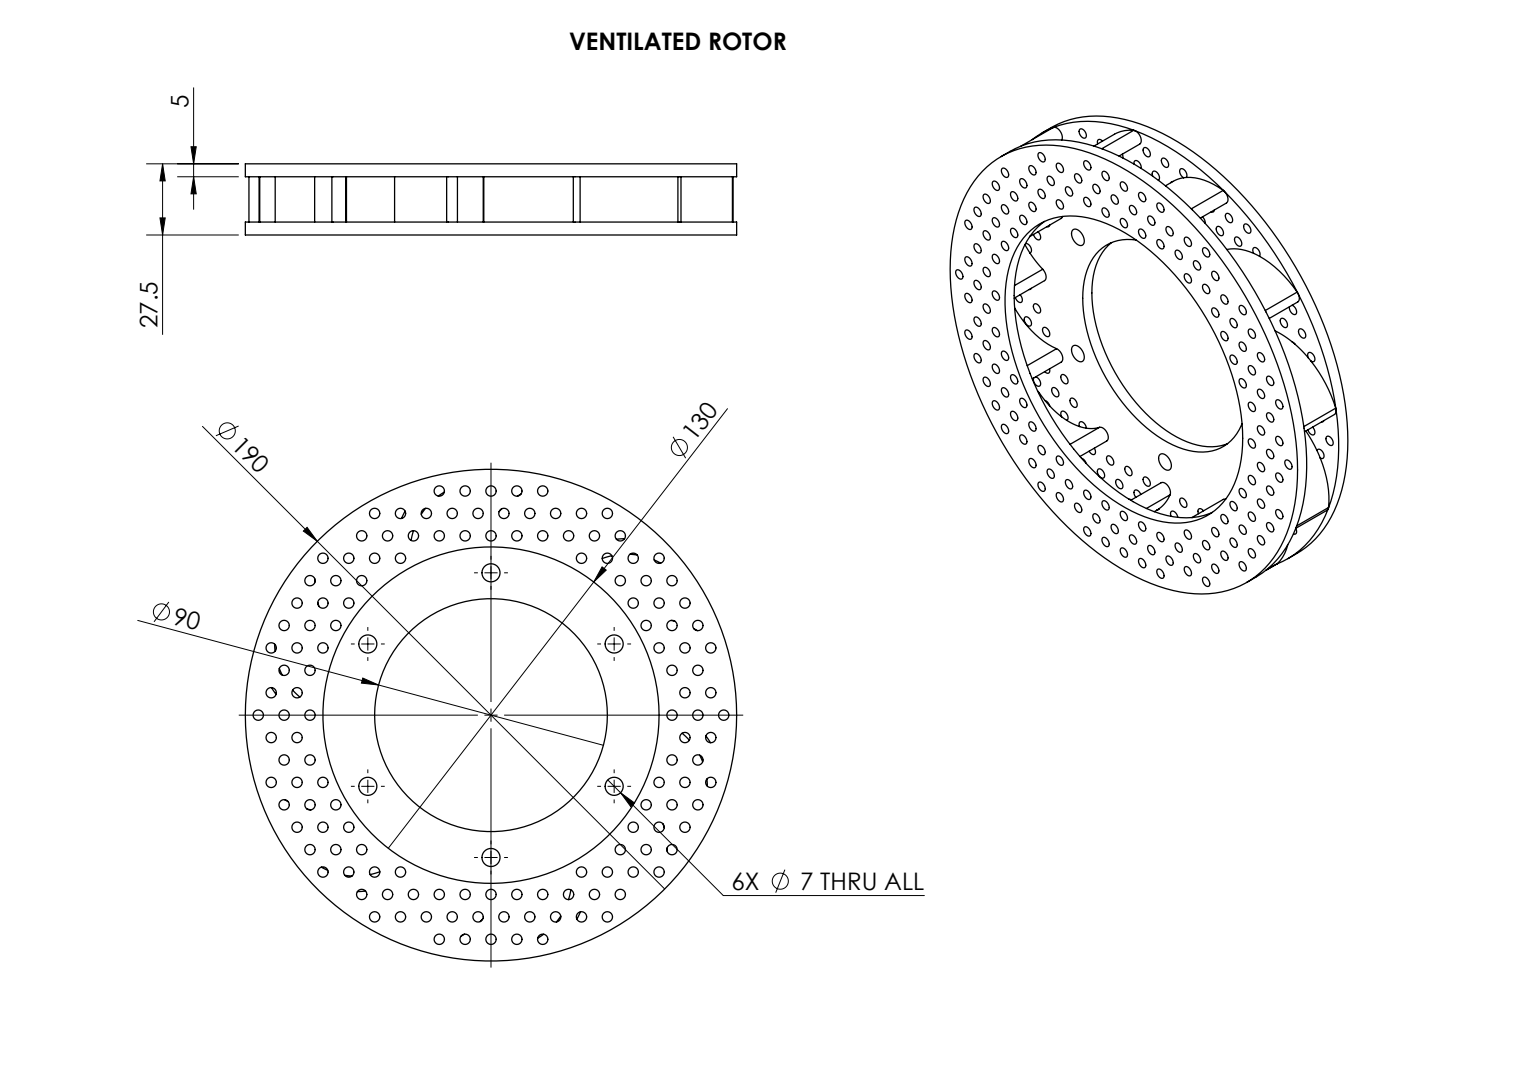
ISO-10303-21;
HEADER;
FILE_DESCRIPTION (('STEP AP214'),
    '1' );
FILE_NAME ('ventilated rotor.step',
    '2026-09-21T15:58:29',
    ( '' ),
    ( '' ),
    'SwSTEP 2.0',
    'SolidWorks 2026',
    '' );
FILE_SCHEMA (( 'AUTOMOTIVE_DESIGN' ));
ENDSEC;

DATA;
#1=ORIENTED_EDGE ( 'NONE', *, *, #25263, .F. ) ;
#2=EDGE_CURVE ( 'NONE', #26836, #23671, #14788, .T. ) ;
#4=VERTEX_POINT ( 'NONE', #16752 ) ;
#5=DIRECTION ( 'NONE',  ( 0.000000000000000000, 0.000000000000000000, 1.000000000000000000 ) ) ;
#7=CARTESIAN_POINT ( 'NONE',  ( 73.47608876694671665, 59.13646009116074964, -4.999999999999997335 ) ) ;
#9=AXIS2_PLACEMENT_3D ( 'NONE', #11158, #31391, #28593 ) ;
#10=DIRECTION ( 'NONE',  ( -1.000000000000000000, 0.000000000000000000, 0.000000000000000000 ) ) ;
#11=DIRECTION ( 'NONE',  ( 0.000000000000000000, 0.000000000000000000, 1.000000000000000000 ) ) ;
#12=FACE_OUTER_BOUND ( 'NONE', #34219, .T. ) ;
#14=ORIENTED_EDGE ( 'NONE', *, *, #31079, .F. ) ;
#15=DIRECTION ( 'NONE',  ( 0.000000000000000000, 0.000000000000000000, 1.000000000000000000 ) ) ;
#17=DIRECTION ( 'NONE',  ( 1.000000000000000000, 0.000000000000000000, 0.000000000000000000 ) ) ;
#19=AXIS2_PLACEMENT_3D ( 'NONE', #6620, #12200, #4183 ) ;
#20=FACE_OUTER_BOUND ( 'NONE', #1538, .T. ) ;
#21=CARTESIAN_POINT ( 'NONE',  ( -85.00000337463092137, -25.98076211353322051, -9.999999999999998224 ) ) ;
#24=EDGE_CURVE ( 'NONE', #14526, #29968, #7006, .T. ) ;
#25=ORIENTED_EDGE ( 'NONE', *, *, #3813, .F. ) ;
#27=EDGE_CURVE ( 'NONE', #13680, #28909, #27960, .T. ) ;
#28=CARTESIAN_POINT ( 'NONE',  ( 31.46585318596250502, 86.45172111230321832, 12.49999999999999822 ) ) ;
#29=AXIS2_PLACEMENT_3D ( 'NONE', #25718, #14617, #11988 ) ;
#30=DIRECTION ( 'NONE',  ( 0.000000000000000000, 0.000000000000000000, 1.000000000000000000 ) ) ;
#31=EDGE_CURVE ( 'NONE', #24795, #10704, #408, .T. ) ;
#32=DIRECTION ( 'NONE',  ( 0.000000000000000000, 0.000000000000000000, -1.000000000000000000 ) ) ;
#33=VERTEX_POINT ( 'NONE', #15201 ) ;
#34=ORIENTED_EDGE ( 'NONE', *, *, #16794, .F. ) ;
#35=AXIS2_PLACEMENT_3D ( 'NONE', #3567, #23609, #24168 ) ;
#36=DIRECTION ( 'NONE',  ( 0.000000000000000000, 0.000000000000000000, 1.000000000000000000 ) ) ;
#38=ORIENTED_EDGE ( 'NONE', *, *, #10995, .T. ) ;
#39=DIRECTION ( 'NONE',  ( 0.000000000000000000, 0.000000000000000000, -1.000000000000000000 ) ) ;
#44=EDGE_CURVE ( 'NONE', #12727, #16632, #5220, .T. ) ;
#45=DIRECTION ( 'NONE',  ( 0.000000000000000000, 0.000000000000000000, 1.000000000000000000 ) ) ;
#47=ORIENTED_EDGE ( 'NONE', *, *, #25069, .T. ) ;
#48=DIRECTION ( 'NONE',  ( 0.000000000000000000, 0.000000000000000000, 1.000000000000000000 ) ) ;
#49=LINE ( 'NONE', #17110, #26195 ) ;
#50=DIRECTION ( 'NONE',  ( 1.000000000000000000, 0.000000000000000000, 0.000000000000000000 ) ) ;
#51=ORIENTED_EDGE ( 'NONE', *, *, #17262, .T. ) ;
#52=CARTESIAN_POINT ( 'NONE',  ( 7.122621931239992550E-13, 68.00000000000000000, -49.86348611802629449 ) ) ;
#53=AXIS2_PLACEMENT_3D ( 'NONE', #21369, #24177, #27163 ) ;
#54=FACE_BOUND ( 'NONE', #30415, .T. ) ;
#55=EDGE_CURVE ( 'NONE', #24891, #6532, #23685, .T. ) ;
#57=CARTESIAN_POINT ( 'NONE',  ( 9.999996625368625658, 86.60254037844397601, 12.50000000000000000 ) ) ;
#58=DIRECTION ( 'NONE',  ( 1.000000000000000000, 0.000000000000000000, 0.000000000000000000 ) ) ;
#59=CYLINDRICAL_SURFACE ( 'NONE', #323, 2.000000000000001776 ) ;
#60=CARTESIAN_POINT ( 'NONE',  ( 89.99999662536828282, 0.000000000000000000, 17.49999999999999645 ) ) ;
#63=CARTESIAN_POINT ( 'NONE',  ( 34.00000000000068923, 58.88972745734143643, 12.49999999999999822 ) ) ;
#64=DIRECTION ( 'NONE',  ( 0.000000000000000000, 0.000000000000000000, -1.000000000000000000 ) ) ;
#66=EDGE_LOOP ( 'NONE', ( #17669, #12617 ) ) ;
#67=EDGE_CURVE ( 'NONE', #35240, #2856, #17838, .T. ) ;
#68=VERTEX_POINT ( 'NONE', #26089 ) ;
#69=ORIENTED_EDGE ( 'NONE', *, *, #4639, .T. ) ;
#70=EDGE_CURVE ( 'NONE', #12832, #7029, #18901, .T. ) ;
#71=EDGE_CURVE ( 'NONE', #553, #16094, #23467, .T. ) ;
#72=DIRECTION ( 'NONE',  ( 0.000000000000000000, 0.000000000000000000, 1.000000000000000000 ) ) ;
#73=FACE_OUTER_BOUND ( 'NONE', #6428, .T. ) ;
#75=EDGE_LOOP ( 'NONE', ( #16524, #10873, #23457, #7165 ) ) ;
#76=CIRCLE ( 'NONE', #28807, 2.000000000000001776 ) ;
#77=DIRECTION ( 'NONE',  ( 1.000000000000000000, 0.000000000000000000, 0.000000000000000000 ) ) ;
#78=ORIENTED_EDGE ( 'NONE', *, *, #9389, .F. ) ;
#80=EDGE_LOOP ( 'NONE', ( #13593, #3847 ) ) ;
#81=CYLINDRICAL_SURFACE ( 'NONE', #36890, 3.000000000000002665 ) ;
#82=ORIENTED_EDGE ( 'NONE', *, *, #8215, .F. ) ;
#83=ORIENTED_EDGE ( 'NONE', *, *, #27457, .T. ) ;
#85=DIRECTION ( 'NONE',  ( 1.000000000000000000, 0.000000000000000000, 0.000000000000000000 ) ) ;
#86=DIRECTION ( 'NONE',  ( 0.000000000000000000, 0.000000000000000000, 1.000000000000000000 ) ) ;
#87=ORIENTED_EDGE ( 'NONE', *, *, #14475, .T. ) ;
#88=DIRECTION ( 'NONE',  ( 0.000000000000000000, 0.000000000000000000, 1.000000000000000000 ) ) ;
#89=EDGE_CURVE ( 'NONE', #15444, #13344, #33274, .T. ) ;
#92=EDGE_LOOP ( 'NONE', ( #21704, #496, #2169, #36469 ) ) ;
#93=CYLINDRICAL_SURFACE ( 'NONE', #7565, 2.000000000000001776 ) ;
#94=DIRECTION ( 'NONE',  ( 0.000000000000000000, 0.000000000000000000, 1.000000000000000000 ) ) ;
#95=CIRCLE ( 'NONE', #3102, 2.000000000000001776 ) ;
#96=ORIENTED_EDGE ( 'NONE', *, *, #17102, .T. ) ;
#97=DIRECTION ( 'NONE',  ( 1.000000000000000000, 0.000000000000000000, 0.000000000000000000 ) ) ;
#98=CIRCLE ( 'NONE', #10881, 2.000000000000001776 ) ;
#99=FACE_OUTER_BOUND ( 'NONE', #4741, .T. ) ;
#100=CYLINDRICAL_SURFACE ( 'NONE', #2791, 2.000000000000001776 ) ;
#101=CARTESIAN_POINT ( 'NONE',  ( 77.99999662536832545, -34.64101615137759183, -9.999999999999998224 ) ) ;
#102=ORIENTED_EDGE ( 'NONE', *, *, #25257, .T. ) ;
#103=DIRECTION ( 'NONE',  ( 1.000000000000000000, 0.000000000000000000, 0.000000000000000000 ) ) ;
#104=FACE_OUTER_BOUND ( 'NONE', #24735, .T. ) ;
#106=ORIENTED_EDGE ( 'NONE', *, *, #23165, .T. ) ;
#107=EDGE_CURVE ( 'NONE', #34831, #10183, #17101, .T. ) ;
#108=FACE_OUTER_BOUND ( 'NONE', #27387, .T. ) ;
#109=CARTESIAN_POINT ( 'NONE',  ( 7.999996625368656744, -69.28203230275519786, 17.49999999999999645 ) ) ;
#110=DIRECTION ( 'NONE',  ( -1.000000000000000000, -4.625929269271482956E-15, 0.000000000000000000 ) ) ;
#111=VERTEX_POINT ( 'NONE', #9201 ) ;
#112=CIRCLE ( 'NONE', #7327, 33.00000000000002132 ) ;
#113=DIRECTION ( 'NONE',  ( 0.000000000000000000, 0.000000000000000000, 1.000000000000000000 ) ) ;
#115=CYLINDRICAL_SURFACE ( 'NONE', #8938, 2.000000000000001776 ) ;
#116=ORIENTED_EDGE ( 'NONE', *, *, #4433, .F. ) ;
#117=DIRECTION ( 'NONE',  ( 1.000000000000000000, 0.000000000000000000, 0.000000000000000000 ) ) ;
#119=CARTESIAN_POINT ( 'NONE',  ( 0.000000000000000000, 0.000000000000000000, 12.49999999999999822 ) ) ;
#121=EDGE_CURVE ( 'NONE', #28672, #5777, #21894, .T. ) ;
#123=CARTESIAN_POINT ( 'NONE',  ( -65.00000337463106348, -60.62177826491083010, -9.999999999999998224 ) ) ;
#124=DIRECTION ( 'NONE',  ( -1.000000000000000000, 0.000000000000000000, 0.000000000000000000 ) ) ;
#125=DIRECTION ( 'NONE',  ( -1.000000000000000000, 0.000000000000000000, 0.000000000000000000 ) ) ;
#126=VERTEX_POINT ( 'NONE', #20628 ) ;
#127=CARTESIAN_POINT ( 'NONE',  ( -56.67878100130369035, 27.78182860042797131, 12.49999999999999822 ) ) ;
#128=DIRECTION ( 'NONE',  ( 0.000000000000000000, 0.000000000000000000, -1.000000000000000000 ) ) ;
#129=DIRECTION ( 'NONE',  ( -1.000000000000000000, 0.000000000000000000, 0.000000000000000000 ) ) ;
#131=EDGE_CURVE ( 'NONE', #32452, #18237, #7927, .T. ) ;
#133=CIRCLE ( 'NONE', #36688, 33.00000000000001421 ) ;
#136=CARTESIAN_POINT ( 'NONE',  ( -20.00000337463123756, -86.60254037844400443, -9.999999999999998224 ) ) ;
#137=EDGE_CURVE ( 'NONE', #22617, #21874, #32058, .T. ) ;
#138=CARTESIAN_POINT ( 'NONE',  ( 71.99999662536838230, -34.64101615137759183, -9.999999999999998224 ) ) ;
#140=DIRECTION ( 'NONE',  ( -1.000000000000000000, -9.765850679573131385E-15, 0.000000000000000000 ) ) ;
#142=ORIENTED_EDGE ( 'NONE', *, *, #26390, .F. ) ;
#145=FACE_OUTER_BOUND ( 'NONE', #19323, .T. ) ;
#147=DIRECTION ( 'NONE',  ( 0.000000000000000000, 0.000000000000000000, 1.000000000000000000 ) ) ;
#148=VERTEX_POINT ( 'NONE', #32628 ) ;
#150=EDGE_CURVE ( 'NONE', #5895, #27049, #26455, .T. ) ;
#151=FACE_BOUND ( 'NONE', #17768, .T. ) ;
#153=CIRCLE ( 'NONE', #7373, 2.000000000000001776 ) ;
#154=ORIENTED_EDGE ( 'NONE', *, *, #13664, .T. ) ;
#155=EDGE_CURVE ( 'NONE', #32663, #9761, #30082, .T. ) ;
#157=CARTESIAN_POINT ( 'NONE',  ( 81.99999662536832545, -17.32050807568879591, -9.999999999999998224 ) ) ;
#158=ORIENTED_EDGE ( 'NONE', *, *, #26934, .T. ) ;
#159=ADVANCED_FACE ( 'NONE', ( #762 ), #32267, .F. ) ;
#161=CARTESIAN_POINT ( 'NONE',  ( 47.99999662536846756, 51.96152422706637708, -5.000000000000000000 ) ) ;
#163=ORIENTED_EDGE ( 'NONE', *, *, #28659, .F. ) ;
#164=ORIENTED_EDGE ( 'NONE', *, *, #35718, .T. ) ;
#165=EDGE_CURVE ( 'NONE', #35067, #9776, #18024, .T. ) ;
#166=AXIS2_PLACEMENT_3D ( 'NONE', #2144, #21659, #19396 ) ;
#167=VERTEX_POINT ( 'NONE', #9594 ) ;
#168=ORIENTED_EDGE ( 'NONE', *, *, #20538, .F. ) ;
#169=AXIS2_PLACEMENT_3D ( 'NONE', #10141, #18184, #29613 ) ;
#171=ORIENTED_EDGE ( 'NONE', *, *, #5884, .T. ) ;
#172=DIRECTION ( 'NONE',  ( 0.000000000000000000, 0.000000000000000000, 1.000000000000000000 ) ) ;
#174=DIRECTION ( 'NONE',  ( 0.000000000000000000, 0.000000000000000000, 1.000000000000000000 ) ) ;
#176=DIRECTION ( 'NONE',  ( 0.000000000000000000, 0.000000000000000000, 1.000000000000000000 ) ) ;
#177=ORIENTED_EDGE ( 'NONE', *, *, #12686, .T. ) ;
#179=CARTESIAN_POINT ( 'NONE',  ( 76.99999662536836809, -8.660254037844401509, -5.000000000000000000 ) ) ;
#180=AXIS2_PLACEMENT_3D ( 'NONE', #17663, #11656, #14493 ) ;
#181=CARTESIAN_POINT ( 'NONE',  ( -87.00000337463093558, 25.98076211353317433, -9.999999999999998224 ) ) ;
#182=VERTEX_POINT ( 'NONE', #6760 ) ;
#184=CARTESIAN_POINT ( 'NONE',  ( -67.00000337463102085, 43.30127018922198801, -9.999999999999998224 ) ) ;
#185=ORIENTED_EDGE ( 'NONE', *, *, #1729, .T. ) ;
#186=EDGE_LOOP ( 'NONE', ( #37032, #34199, #35351 ) ) ;
#189=DIRECTION ( 'NONE',  ( -1.000000000000000000, 0.000000000000000000, 0.000000000000000000 ) ) ;
#190=DIRECTION ( 'NONE',  ( 0.000000000000000000, 0.000000000000000000, 1.000000000000000000 ) ) ;
#191=FACE_OUTER_BOUND ( 'NONE', #12059, .T. ) ;
#192=ORIENTED_EDGE ( 'NONE', *, *, #24443, .F. ) ;
#193=ORIENTED_EDGE ( 'NONE', *, *, #28677, .F. ) ;
#195=FACE_OUTER_BOUND ( 'NONE', #26488, .T. ) ;
#196=EDGE_CURVE ( 'NONE', #666, #24271, #33682, .T. ) ;
#198=CYLINDRICAL_SURFACE ( 'NONE', #3922, 2.000000000000001776 ) ;
#199=CIRCLE ( 'NONE', #27130, 2.000000000000001776 ) ;
#200=VERTEX_POINT ( 'NONE', #18959 ) ;
#203=VERTEX_POINT ( 'NONE', #33394 ) ;
#204=ORIENTED_EDGE ( 'NONE', *, *, #23510, .F. ) ;
#205=CIRCLE ( 'NONE', #19978, 1.999999999999998224 ) ;
#206=CARTESIAN_POINT ( 'NONE',  ( -55.00000337463107059, 43.30127018922197379, -9.999999999999998224 ) ) ;
#207=AXIS2_PLACEMENT_3D ( 'NONE', #7351, #10726, #24618 ) ;
#208=LINE ( 'NONE', #6596, #28035 ) ;
#210=VERTEX_POINT ( 'NONE', #1504 ) ;
#211=FACE_OUTER_BOUND ( 'NONE', #12219, .T. ) ;
#213=DIRECTION ( 'NONE',  ( 0.000000000000000000, 0.000000000000000000, 1.000000000000000000 ) ) ;
#214=DIRECTION ( 'NONE',  ( -1.000000000000000000, 0.000000000000000000, 0.000000000000000000 ) ) ;
#215=EDGE_CURVE ( 'NONE', #20361, #36249, #4334, .T. ) ;
#217=CARTESIAN_POINT ( 'NONE',  ( 54.99999662536846046, -43.30127018922200222, -9.999999999999998224 ) ) ;
#218=FACE_BOUND ( 'NONE', #809, .T. ) ;
#220=DIRECTION ( 'NONE',  ( 1.000000000000000000, 0.000000000000000000, 0.000000000000000000 ) ) ;
#221=CARTESIAN_POINT ( 'NONE',  ( -13.00000337463126066, 77.94228634059957983, 17.49999999999999645 ) ) ;
#222=DIRECTION ( 'NONE',  ( 1.000000000000000000, 0.000000000000000000, 0.000000000000000000 ) ) ;
#223=CIRCLE ( 'NONE', #20559, 2.000000000000000000 ) ;
#224=DIRECTION ( 'NONE',  ( 0.000000000000000000, 0.000000000000000000, 1.000000000000000000 ) ) ;
#225=DIRECTION ( 'NONE',  ( 0.000000000000000000, 0.000000000000000000, -1.000000000000000000 ) ) ;
#226=ORIENTED_EDGE ( 'NONE', *, *, #20326, .F. ) ;
#227=CARTESIAN_POINT ( 'NONE',  ( -60.00000337463108480, -51.96152422706641971, -9.999999999999998224 ) ) ;
#228=DIRECTION ( 'NONE',  ( 0.000000000000000000, 0.000000000000000000, -1.000000000000000000 ) ) ;
#230=VECTOR ( 'NONE', #24200, 1000.000000000000000 ) ;
#232=EDGE_LOOP ( 'NONE', ( #6616, #28930, #1676, #8816 ) ) ;
#233=EDGE_CURVE ( 'NONE', #35279, #34770, #16155, .T. ) ;
#234=ORIENTED_EDGE ( 'NONE', *, *, #11721, .F. ) ;
#235=CIRCLE ( 'NONE', #13432, 1.999999999999998224 ) ;
#236=DIRECTION ( 'NONE',  ( -1.000000000000000000, 0.000000000000000000, 0.000000000000000000 ) ) ;
#237=CYLINDRICAL_SURFACE ( 'NONE', #14553, 2.000000000000001776 ) ;
#238=EDGE_CURVE ( 'NONE', #20810, #35505, #23500, .T. ) ;
#239=CARTESIAN_POINT ( 'NONE',  ( 79.99999662536833966, 34.64101615137759183, -5.000000000000000000 ) ) ;
#240=EDGE_LOOP ( 'NONE', ( #25593, #21234, #28289, #3164 ) ) ;
#241=EDGE_CURVE ( 'NONE', #35128, #3947, #28283, .T. ) ;
#242=DIRECTION ( 'NONE',  ( 0.8660254037844418162, 0.4999999999999946709, 0.000000000000000000 ) ) ;
#243=ORIENTED_EDGE ( 'NONE', *, *, #24473, .T. ) ;
#244=CARTESIAN_POINT ( 'NONE',  ( -70.00000337463099243, 51.96152422706637708, -5.000000000000000000 ) ) ;
#245=VERTEX_POINT ( 'NONE', #21754 ) ;
#246=EDGE_CURVE ( 'NONE', #24313, #6247, #31847, .T. ) ;
#249=EDGE_CURVE ( 'NONE', #20086, #13680, #36679, .T. ) ;
#251=CIRCLE ( 'NONE', #9840, 27.00000000000001421 ) ;
#253=CARTESIAN_POINT ( 'NONE',  ( -31.00000000000027356, -58.88972745734168512, -4.999999999999997335 ) ) ;
#254=CARTESIAN_POINT ( 'NONE',  ( -3.374631303565411855E-06, -86.60254037844400443, -9.999999999999998224 ) ) ;
#255=ORIENTED_EDGE ( 'NONE', *, *, #21076, .T. ) ;
#256=DIRECTION ( 'NONE',  ( 1.000000000000000000, 0.000000000000000000, 0.000000000000000000 ) ) ;
#257=EDGE_CURVE ( 'NONE', #28630, #6061, #8948, .T. ) ;
#258=AXIS2_PLACEMENT_3D ( 'NONE', #28130, #2453, #13872 ) ;
#259=CARTESIAN_POINT ( 'NONE',  ( 0.000000000000000000, 0.000000000000000000, 12.49999999999999822 ) ) ;
#260=AXIS2_PLACEMENT_3D ( 'NONE', #12321, #32216, #32783 ) ;
#262=DIRECTION ( 'NONE',  ( -1.000000000000000000, 0.000000000000000000, 0.000000000000000000 ) ) ;
#263=ADVANCED_FACE ( 'NONE', ( #24402 ), #10505, .F. ) ;
#264=EDGE_LOOP ( 'NONE', ( #8446, #2459 ) ) ;
#266=CARTESIAN_POINT ( 'NONE',  ( 51.99999662536848888, -51.96152422706640550, 12.50000000000000000 ) ) ;
#268=EDGE_CURVE ( 'NONE', #8353, #34330, #5962, .T. ) ;
#269=ORIENTED_EDGE ( 'NONE', *, *, #4961, .F. ) ;
#270=CARTESIAN_POINT ( 'NONE',  ( -40.00000337463113453, 69.28203230275516944, -9.999999999999998224 ) ) ;
#271=CARTESIAN_POINT ( 'NONE',  ( 68.00000000000000000, 0.000000000000000000, -49.86348611802629449 ) ) ;
#272=FACE_OUTER_BOUND ( 'NONE', #19222, .T. ) ;
#274=DIRECTION ( 'NONE',  ( 1.000000000000000000, 0.000000000000000000, 0.000000000000000000 ) ) ;
#275=AXIS2_PLACEMENT_3D ( 'NONE', #18372, #12551, #4489 ) ;
#279=DIRECTION ( 'NONE',  ( 0.000000000000000000, 0.000000000000000000, 1.000000000000000000 ) ) ;
#281=VERTEX_POINT ( 'NONE', #22145 ) ;
#282=CIRCLE ( 'NONE', #23627, 2.000000000000001776 ) ;
#286=DIRECTION ( 'NONE',  ( 0.000000000000000000, 0.000000000000000000, 1.000000000000000000 ) ) ;
#287=DIRECTION ( 'NONE',  ( -1.000000000000000000, 0.000000000000000000, 0.000000000000000000 ) ) ;
#288=AXIS2_PLACEMENT_3D ( 'NONE', #11552, #26000, #31627 ) ;
#289=CIRCLE ( 'NONE', #2710, 2.000000000000001776 ) ;
#290=DIRECTION ( 'NONE',  ( 0.000000000000000000, 0.000000000000000000, -1.000000000000000000 ) ) ;
#291=ORIENTED_EDGE ( 'NONE', *, *, #20174, .T. ) ;
#293=ORIENTED_EDGE ( 'NONE', *, *, #27242, .F. ) ;
#294=FACE_BOUND ( 'NONE', #33628, .T. ) ;
#295=DIRECTION ( 'NONE',  ( 1.000000000000000000, 0.000000000000000000, 0.000000000000000000 ) ) ;
#296=CIRCLE ( 'NONE', #6888, 2.000000000000001776 ) ;
#297=CARTESIAN_POINT ( 'NONE',  ( -60.00000337463104216, 34.64101615137757051, -9.999999999999998224 ) ) ;
#298=CIRCLE ( 'NONE', #6279, 95.00000000000001421 ) ;
#299=DIRECTION ( 'NONE',  ( 0.000000000000000000, 0.000000000000000000, 1.000000000000000000 ) ) ;
#301=VECTOR ( 'NONE', #9104, 1000.000000000000000 ) ;
#302=AXIS2_PLACEMENT_3D ( 'NONE', #13859, #25139, #31280 ) ;
#304=CARTESIAN_POINT ( 'NONE',  ( 64.99999662536839651, -43.30127018922199511, -9.999999999999998224 ) ) ;
#305=DIRECTION ( 'NONE',  ( 0.000000000000000000, 0.000000000000000000, 1.000000000000000000 ) ) ;
#306=EDGE_CURVE ( 'NONE', #32244, #30221, #25138, .T. ) ;
#308=CARTESIAN_POINT ( 'NONE',  ( -40.00000337463113453, -69.28203230275519786, 17.49999999999999645 ) ) ;
#309=CYLINDRICAL_SURFACE ( 'NONE', #34030, 2.000000000000001776 ) ;
#310=VECTOR ( 'NONE', #20718, 1000.000000000000000 ) ;
#311=CARTESIAN_POINT ( 'NONE',  ( -48.49679504533954599, -67.96280346788670101, 12.50000000000000000 ) ) ;
#312=AXIS2_PLACEMENT_3D ( 'NONE', #1612, #13051, #12846 ) ;
#313=CIRCLE ( 'NONE', #17111, 33.00000000000001421 ) ;
#314=EDGE_LOOP ( 'NONE', ( #13805, #27625, #5618, #19237 ) ) ;
#317=ORIENTED_EDGE ( 'NONE', *, *, #23310, .F. ) ;
#318=CYLINDRICAL_SURFACE ( 'NONE', #26736, 2.000000000000001776 ) ;
#320=VECTOR ( 'NONE', #25378, 1000.000000000000000 ) ;
#321=LINE ( 'NONE', #703, #22374 ) ;
#323=AXIS2_PLACEMENT_3D ( 'NONE', #34020, #22562, #31540 ) ;
#324=CARTESIAN_POINT ( 'NONE',  ( 34.99999662536855283, -77.94228634059960825, -9.999999999999998224 ) ) ;
#325=VECTOR ( 'NONE', #1638, 1000.000000000000000 ) ;
#326=EDGE_CURVE ( 'NONE', #14473, #5023, #12520, .T. ) ;
#327=AXIS2_PLACEMENT_3D ( 'NONE', #16910, #9026, #2860 ) ;
#328=DIRECTION ( 'NONE',  ( 1.000000000000000000, 0.000000000000000000, 0.000000000000000000 ) ) ;
#329=EDGE_CURVE ( 'NONE', #27070, #4355, #10750, .T. ) ;
#330=ORIENTED_EDGE ( 'NONE', *, *, #17401, .T. ) ;
#331=ORIENTED_EDGE ( 'NONE', *, *, #15606, .T. ) ;
#332=DIRECTION ( 'NONE',  ( 1.000000000000000000, 0.000000000000000000, 0.000000000000000000 ) ) ;
#333=DIRECTION ( 'NONE',  ( 0.000000000000000000, 0.000000000000000000, 1.000000000000000000 ) ) ;
#334=LINE ( 'NONE', #8600, #4130 ) ;
#336=AXIS2_PLACEMENT_3D ( 'NONE', #30480, #30096, #21491 ) ;
#337=EDGE_CURVE ( 'NONE', #3085, #32118, #36511, .T. ) ;
#338=FACE_BOUND ( 'NONE', #19821, .T. ) ;
#339=EDGE_LOOP ( 'NONE', ( #32117, #28572, #22647 ) ) ;
#340=ORIENTED_EDGE ( 'NONE', *, *, #13858, .F. ) ;
#341=CARTESIAN_POINT ( 'NONE',  ( 31.99999662536857770, -69.28203230275519786, 17.49999999999999645 ) ) ;
#342=ORIENTED_EDGE ( 'NONE', *, *, #22958, .F. ) ;
#344=DIRECTION ( 'NONE',  ( 1.000000000000000000, 0.000000000000000000, 0.000000000000000000 ) ) ;
#347=EDGE_CURVE ( 'NONE', #5750, #19941, #18596, .T. ) ;
#348=ORIENTED_EDGE ( 'NONE', *, *, #23113, .F. ) ;
#349=ORIENTED_EDGE ( 'NONE', *, *, #15856, .F. ) ;
#351=CIRCLE ( 'NONE', #30901, 27.00000000000001421 ) ;
#352=ORIENTED_EDGE ( 'NONE', *, *, #4867, .T. ) ;
#353=VECTOR ( 'NONE', #6522, 1000.000000000000000 ) ;
#354=AXIS2_PLACEMENT_3D ( 'NONE', #1393, #4597, #16033 ) ;
#355=EDGE_LOOP ( 'NONE', ( #5631, #10944 ) ) ;
#356=CIRCLE ( 'NONE', #29106, 2.000000000000001776 ) ;
#357=VERTEX_POINT ( 'NONE', #11426 ) ;
#358=CARTESIAN_POINT ( 'NONE',  ( 64.99999662536839651, -60.62177826491080168, 12.50000000000000000 ) ) ;
#359=DIRECTION ( 'NONE',  ( 0.000000000000000000, 0.000000000000000000, 1.000000000000000000 ) ) ;
#360=CARTESIAN_POINT ( 'NONE',  ( 61.99999662536842493, 51.96152422706639129, -9.999999999999998224 ) ) ;
#362=DIRECTION ( 'NONE',  ( 0.000000000000000000, 0.000000000000000000, 1.000000000000000000 ) ) ;
#363=ORIENTED_EDGE ( 'NONE', *, *, #17772, .T. ) ;
#364=DIRECTION ( 'NONE',  ( 4.625929269271481378E-15, 1.000000000000000000, 0.000000000000000000 ) ) ;
#365=VECTOR ( 'NONE', #5528, 1000.000000000000000 ) ;
#366=CARTESIAN_POINT ( 'NONE',  ( -3.374631289687624047E-06, -69.28203230275519786, 17.49999999999999645 ) ) ;
#367=EDGE_CURVE ( 'NONE', #31278, #23804, #18545, .T. ) ;
#369=ORIENTED_EDGE ( 'NONE', *, *, #22241, .T. ) ;
#370=DIRECTION ( 'NONE',  ( 1.000000000000000000, 0.000000000000000000, 0.000000000000000000 ) ) ;
#371=CARTESIAN_POINT ( 'NONE',  ( -50.00000337463112032, -51.96152422706641971, -9.999999999999998224 ) ) ;
#372=ORIENTED_EDGE ( 'NONE', *, *, #6789, .F. ) ;
#373=AXIS2_PLACEMENT_3D ( 'NONE', #34364, #17849, #12387 ) ;
#376=CIRCLE ( 'NONE', #15948, 2.000000000000001776 ) ;
#377=PRODUCT_DEFINITION ( 'UNKNOWN', '', #6977, #25310 ) ;
#378=DIRECTION ( 'NONE',  ( -1.000000000000000000, 0.000000000000000000, 0.000000000000000000 ) ) ;
#379=DIRECTION ( 'NONE',  ( 1.000000000000000000, 0.000000000000000000, 0.000000000000000000 ) ) ;
#380=DIRECTION ( 'NONE',  ( 0.000000000000000000, 0.000000000000000000, -1.000000000000000000 ) ) ;
#381=EDGE_CURVE ( 'NONE', #31393, #2483, #23330, .T. ) ;
#383=ORIENTED_EDGE ( 'NONE', *, *, #2638, .F. ) ;
#384=AXIS2_PLACEMENT_3D ( 'NONE', #15641, #24247, #35700 ) ;
#386=CARTESIAN_POINT ( 'NONE',  ( 44.99999662536851019, 77.94228634059959404, -9.999999999999998224 ) ) ;
#387=CARTESIAN_POINT ( 'NONE',  ( 46.99999662536849598, 60.62177826491077326, -9.999999999999998224 ) ) ;
#389=AXIS2_PLACEMENT_3D ( 'NONE', #3869, #35759, #30111 ) ;
#390=ADVANCED_FACE ( 'NONE', ( #34309 ), #8442, .F. ) ;
#393=VERTEX_POINT ( 'NONE', #19504 ) ;
#395=CIRCLE ( 'NONE', #5209, 2.000000000000001776 ) ;
#396=DIRECTION ( 'NONE',  ( 0.000000000000000000, 0.000000000000000000, 1.000000000000000000 ) ) ;
#397=CARTESIAN_POINT ( 'NONE',  ( -8.000003374631278419, -69.28203230275519786, -9.999999999999998224 ) ) ;
#398=ORIENTED_EDGE ( 'NONE', *, *, #9596, .T. ) ;
#399=ORIENTED_EDGE ( 'NONE', *, *, #27886, .T. ) ;
#402=CARTESIAN_POINT ( 'NONE',  ( 54.99999662536846046, -43.30127018922200222, -5.000000000000000000 ) ) ;
#403=FACE_OUTER_BOUND ( 'NONE', #1715, .T. ) ;
#405=CIRCLE ( 'NONE', #23176, 2.000000000000001776 ) ;
#406=VERTEX_POINT ( 'NONE', #31295 ) ;
#407=CARTESIAN_POINT ( 'NONE',  ( -75.00000337463097821, -8.660254037844422825, -5.000000000000000000 ) ) ;
#408=CIRCLE ( 'NONE', #21379, 95.00000000000000000 ) ;
#409=FACE_BOUND ( 'NONE', #25954, .T. ) ;
#410=DIRECTION ( 'NONE',  ( 0.000000000000000000, 0.000000000000000000, 1.000000000000000000 ) ) ;
#411=CARTESIAN_POINT ( 'NONE',  ( 84.99999662536832545, 25.98076211353319565, -5.000000000000000000 ) ) ;
#414=CYLINDRICAL_SURFACE ( 'NONE', #5727, 2.000000000000001776 ) ;
#415=EDGE_CURVE ( 'NONE', #9776, #6234, #17336, .T. ) ;
#416=AXIS2_PLACEMENT_3D ( 'NONE', #33124, #10826, #22083 ) ;
#417=CIRCLE ( 'NONE', #24987, 2.000000000000001776 ) ;
#418=CARTESIAN_POINT ( 'NONE',  ( -72.00000337463100664, 34.64101615137758472, -9.999999999999998224 ) ) ;
#419=EDGE_CURVE ( 'NONE', #33801, #10648, #30929, .T. ) ;
#422=DIRECTION ( 'NONE',  ( -1.000000000000000000, 0.000000000000000000, 0.000000000000000000 ) ) ;
#425=AXIS2_PLACEMENT_3D ( 'NONE', #16423, #2545, #16814 ) ;
#426=ORIENTED_EDGE ( 'NONE', *, *, #31754, .T. ) ;
#427=AXIS2_PLACEMENT_3D ( 'NONE', #36028, #27183, #30185 ) ;
#429=EDGE_LOOP ( 'NONE', ( #21064, #7984 ) ) ;
#432=CARTESIAN_POINT ( 'NONE',  ( -30.00000337463118427, 69.28203230275516944, -9.999999999999998224 ) ) ;
#433=ORIENTED_EDGE ( 'NONE', *, *, #32932, .F. ) ;
#435=CIRCLE ( 'NONE', #1059, 2.000000000000001776 ) ;
#437=EDGE_CURVE ( 'NONE', #14230, #21660, #8801, .T. ) ;
#438=AXIS2_PLACEMENT_3D ( 'NONE', #22022, #2338, #36089 ) ;
#439=ORIENTED_EDGE ( 'NONE', *, *, #25001, .T. ) ;
#442=LINE ( 'NONE', #35143, #33928 ) ;
#443=ORIENTED_EDGE ( 'NONE', *, *, #11812, .T. ) ;
#444=ORIENTED_EDGE ( 'NONE', *, *, #10489, .T. ) ;
#445=CIRCLE ( 'NONE', #21413, 2.000000000000001776 ) ;
#446=AXIS2_PLACEMENT_3D ( 'NONE', #13189, #27434, #32882 ) ;
#447=CARTESIAN_POINT ( 'NONE',  ( -65.00000337463104927, -43.30127018922202353, -9.999999999999998224 ) ) ;
#448=LINE ( 'NONE', #18241, #25630 ) ;
#449=DIRECTION ( 'NONE',  ( 0.000000000000000000, 0.000000000000000000, 1.000000000000000000 ) ) ;
#450=ORIENTED_EDGE ( 'NONE', *, *, #35879, .F. ) ;
#452=AXIS2_PLACEMENT_3D ( 'NONE', #7985, #34244, #8372 ) ;
#453=DIRECTION ( 'NONE',  ( -0.000000000000000000, 0.000000000000000000, -1.000000000000000000 ) ) ;
#454=CARTESIAN_POINT ( 'NONE',  ( 35.19434990244975126, -52.39915983220758022, 12.49999999999999822 ) ) ;
#455=EDGE_CURVE ( 'NONE', #28642, #34166, #20183, .T. ) ;
#456=ORIENTED_EDGE ( 'NONE', *, *, #33462, .T. ) ;
#457=FACE_OUTER_BOUND ( 'NONE', #6118, .T. ) ;
#458=AXIS2_PLACEMENT_3D ( 'NONE', #31556, #28758, #23130 ) ;
#459=CARTESIAN_POINT ( 'NONE',  ( -55.00000337463107059, 60.62177826491078747, -9.999999999999998224 ) ) ;
#461=EDGE_CURVE ( 'NONE', #15417, #12117, #25697, .T. ) ;
#462=CARTESIAN_POINT ( 'NONE',  ( 79.83584911142594365, 32.64776363509508883, 12.50000000000000000 ) ) ;
#463=AXIS2_PLACEMENT_3D ( 'NONE', #20717, #23541, #16991 ) ;
#464=VECTOR ( 'NONE', #22327, 1000.000000000000000 ) ;
#465=DIRECTION ( 'NONE',  ( 1.000000000000000000, 0.000000000000000000, 0.000000000000000000 ) ) ;
#466=DIRECTION ( 'NONE',  ( 0.000000000000000000, 0.000000000000000000, -1.000000000000000000 ) ) ;
#467=CARTESIAN_POINT ( 'NONE',  ( 59.99999662536845335, 34.64101615137759893, -5.000000000000000000 ) ) ;
#468=VECTOR ( 'NONE', #869, 1000.000000000000000 ) ;
#470=LINE ( 'NONE', #31594, #559 ) ;
#471=CIRCLE ( 'NONE', #6443, 2.000000000000001776 ) ;
#472=CARTESIAN_POINT ( 'NONE',  ( -37.00000337463116296, 60.62177826491077326, -5.000000000000000000 ) ) ;
#473=ORIENTED_EDGE ( 'NONE', *, *, #22699, .T. ) ;
#474=DIRECTION ( 'NONE',  ( 0.000000000000000000, 0.000000000000000000, 1.000000000000000000 ) ) ;
#475=EDGE_CURVE ( 'NONE', #21726, #32663, #25496, .T. ) ;
#476=DIRECTION ( 'NONE',  ( -1.000000000000000000, 0.000000000000000000, 0.000000000000000000 ) ) ;
#477=DIRECTION ( 'NONE',  ( -0.000000000000000000, -0.000000000000000000, 1.000000000000000000 ) ) ;
#478=ADVANCED_FACE ( 'NONE', ( #16501 ), #22494, .F. ) ;
#479=ORIENTED_EDGE ( 'NONE', *, *, #28678, .T. ) ;
#480=ORIENTED_EDGE ( 'NONE', *, *, #7602, .T. ) ;
#481=ORIENTED_EDGE ( 'NONE', *, *, #15113, .F. ) ;
#482=DIRECTION ( 'NONE',  ( 0.8660254037844347108, -0.5000000000000067724, 0.000000000000000000 ) ) ;
#484=DIRECTION ( 'NONE',  ( 0.000000000000000000, 0.000000000000000000, 1.000000000000000000 ) ) ;
#485=CIRCLE ( 'NONE', #14278, 2.000000000000001776 ) ;
#487=EDGE_CURVE ( 'NONE', #18803, #9986, #30966, .T. ) ;
#489=EDGE_CURVE ( 'NONE', #8845, #17624, #29750, .T. ) ;
#490=AXIS2_PLACEMENT_3D ( 'NONE', #34543, #3216, #9032 ) ;
#494=EDGE_CURVE ( 'NONE', #22235, #8449, #26177, .T. ) ;
#495=DIRECTION ( 'NONE',  ( 0.000000000000000000, 0.000000000000000000, 1.000000000000000000 ) ) ;
#496=ORIENTED_EDGE ( 'NONE', *, *, #6778, .F. ) ;
#497=CIRCLE ( 'NONE', #16671, 2.000000000000001776 ) ;
#498=AXIS2_PLACEMENT_3D ( 'NONE', #15560, #26807, #26606 ) ;
#499=FACE_BOUND ( 'NONE', #23878, .T. ) ;
#500=AXIS2_PLACEMENT_3D ( 'NONE', #24873, #22243, #28401 ) ;
#501=VECTOR ( 'NONE', #13470, 1000.000000000000000 ) ;
#503=CARTESIAN_POINT ( 'NONE',  ( 49.99999662536848177, -51.96152422706640550, -5.000000000000000000 ) ) ;
#504=ORIENTED_EDGE ( 'NONE', *, *, #24797, .F. ) ;
#507=AXIS2_PLACEMENT_3D ( 'NONE', #23833, #9582, #9188 ) ;
#508=DIRECTION ( 'NONE',  ( 0.000000000000000000, 0.000000000000000000, 1.000000000000000000 ) ) ;
#509=CIRCLE ( 'NONE', #25684, 33.00000000000001421 ) ;
#510=CARTESIAN_POINT ( 'NONE',  ( -65.00000337463106348, -60.62177826491083010, -5.000000000000000000 ) ) ;
#512=ORIENTED_EDGE ( 'NONE', *, *, #1242, .T. ) ;
#513=CARTESIAN_POINT ( 'NONE',  ( 46.99999662536851019, 77.94228634059959404, -9.999999999999998224 ) ) ;
#514=CARTESIAN_POINT ( 'NONE',  ( 79.99999662536833966, 34.64101615137759183, 12.50000000000000000 ) ) ;
#515=AXIS2_PLACEMENT_3D ( 'NONE', #34654, #34457, #12285 ) ;
#516=CARTESIAN_POINT ( 'NONE',  ( -77.00000337463097821, 43.30127018922197379, -9.999999999999998224 ) ) ;
#517=ORIENTED_EDGE ( 'NONE', *, *, #24288, .F. ) ;
#518=EDGE_LOOP ( 'NONE', ( #20740, #16897, #25527, #2907, #12930 ) ) ;
#519=VECTOR ( 'NONE', #3730, 1000.000000000000000 ) ;
#520=VERTEX_POINT ( 'NONE', #10263 ) ;
#522=LINE ( 'NONE', #18315, #353 ) ;
#523=FACE_OUTER_BOUND ( 'NONE', #3503, .T. ) ;
#528=CIRCLE ( 'NONE', #2341, 27.00000000000001421 ) ;
#529=CYLINDRICAL_SURFACE ( 'NONE', #4228, 2.000000000000000000 ) ;
#531=EDGE_CURVE ( 'NONE', #35883, #4900, #15393, .T. ) ;
#532=ORIENTED_EDGE ( 'NONE', *, *, #24422, .F. ) ;
#533=LINE ( 'NONE', #26023, #19487 ) ;
#534=VECTOR ( 'NONE', #24717, 1000.000000000000000 ) ;
#538=VERTEX_POINT ( 'NONE', #33526 ) ;
#539=CARTESIAN_POINT ( 'NONE',  ( -3.374631303565411855E-06, -86.60254037844400443, 12.50000000000000000 ) ) ;
#541=ORIENTED_EDGE ( 'NONE', *, *, #11291, .F. ) ;
#542=ORIENTED_EDGE ( 'NONE', *, *, #25215, .T. ) ;
#543=AXIS2_PLACEMENT_3D ( 'NONE', #29779, #32409, #21345 ) ;
#545=VERTEX_POINT ( 'NONE', #15886 ) ;
#546=CARTESIAN_POINT ( 'NONE',  ( -15.00000337463126066, 77.94228634059957983, 12.50000000000000000 ) ) ;
#547=CARTESIAN_POINT ( 'NONE',  ( -25.00000337463120914, 77.94228634059957983, -5.000000000000000000 ) ) ;
#549=AXIS2_PLACEMENT_3D ( 'NONE', #29523, #28026, #13587 ) ;
#550=VERTEX_POINT ( 'NONE', #27865 ) ;
#551=ORIENTED_EDGE ( 'NONE', *, *, #18723, .F. ) ;
#552=AXIS2_PLACEMENT_3D ( 'NONE', #10097, #4282, #15895 ) ;
#553=VERTEX_POINT ( 'NONE', #35970 ) ;
#555=ORIENTED_EDGE ( 'NONE', *, *, #20326, .T. ) ;
#556=VECTOR ( 'NONE', #15858, 1000.000000000000000 ) ;
#559=VECTOR ( 'NONE', #17364, 1000.000000000000000 ) ;
#560=ORIENTED_EDGE ( 'NONE', *, *, #23769, .T. ) ;
#561=DIRECTION ( 'NONE',  ( 0.000000000000000000, 0.000000000000000000, 1.000000000000000000 ) ) ;
#564=ORIENTED_EDGE ( 'NONE', *, *, #32404, .T. ) ;
#565=DIRECTION ( 'NONE',  ( 1.000000000000000000, 0.000000000000000000, 0.000000000000000000 ) ) ;
#567=CARTESIAN_POINT ( 'NONE',  ( 31.46585318596250502, 86.45172111230321832, -4.999999999999997335 ) ) ;
#568=VECTOR ( 'NONE', #23561, 1000.000000000000000 ) ;
#569=DIRECTION ( 'NONE',  ( 0.000000000000000000, 0.000000000000000000, 1.000000000000000000 ) ) ;
#570=EDGE_LOOP ( 'NONE', ( #30471, #6213, #2466, #12851 ) ) ;
#571=FACE_OUTER_BOUND ( 'NONE', #12516, .T. ) ;
#572=CIRCLE ( 'NONE', #33545, 2.000000000000000000 ) ;
#575=VERTEX_POINT ( 'NONE', #13630 ) ;
#577=DIRECTION ( 'NONE',  ( -0.000000000000000000, -0.000000000000000000, 1.000000000000000000 ) ) ;
#578=EDGE_CURVE ( 'NONE', #33610, #19047, #7627, .T. ) ;
#581=ORIENTED_EDGE ( 'NONE', *, *, #7822, .T. ) ;
#582=CIRCLE ( 'NONE', #23347, 2.000000000000001776 ) ;
#583=DIRECTION ( 'NONE',  ( 1.000000000000000000, 0.000000000000000000, 0.000000000000000000 ) ) ;
#584=CARTESIAN_POINT ( 'NONE',  ( -85.00000337463092137, 25.98076211353317433, -9.999999999999998224 ) ) ;
#586=AXIS2_PLACEMENT_3D ( 'NONE', #7498, #4888, #30917 ) ;
#587=ORIENTED_EDGE ( 'NONE', *, *, #4431, .F. ) ;
#590=CIRCLE ( 'NONE', #1189, 2.000000000000001776 ) ;
#592=DIRECTION ( 'NONE',  ( 1.000000000000000000, 0.000000000000000000, 0.000000000000000000 ) ) ;
#594=AXIS2_PLACEMENT_3D ( 'NONE', #28395, #2721, #11351 ) ;
#596=CARTESIAN_POINT ( 'NONE',  ( 4.279621169095998212, -62.97617850287780072, -4.999999999999997335 ) ) ;
#597=ORIENTED_EDGE ( 'NONE', *, *, #25808, .T. ) ;
#598=VERTEX_POINT ( 'NONE', #27124 ) ;
#601=DIRECTION ( 'NONE',  ( 0.000000000000000000, 0.000000000000000000, 1.000000000000000000 ) ) ;
#602=CARTESIAN_POINT ( 'NONE',  ( -5.000003374631307729, 77.94228634059957983, -5.000000000000000000 ) ) ;
#603=VERTEX_POINT ( 'NONE', #27313 ) ;
#604=CARTESIAN_POINT ( 'NONE',  ( -10.00000337463125000, -86.60254037844400443, -9.999999999999998224 ) ) ;
#605=FACE_BOUND ( 'NONE', #24109, .T. ) ;
#606=CIRCLE ( 'NONE', #19787, 27.00000000000001421 ) ;
#607=EDGE_CURVE ( 'NONE', #27018, #35698, #9402, .T. ) ;
#609=LINE ( 'NONE', #1339, #13284 ) ;
#610=DIRECTION ( 'NONE',  ( -0.000000000000000000, -0.000000000000000000, 1.000000000000000000 ) ) ;
#611=CIRCLE ( 'NONE', #14987, 2.000000000000000000 ) ;
#612=EDGE_LOOP ( 'NONE', ( #26487, #9451, #450, #4104, #36029, #18289 ) ) ;
#616=AXIS2_PLACEMENT_3D ( 'NONE', #20434, #3187, #26434 ) ;
#618=ORIENTED_EDGE ( 'NONE', *, *, #36591, .T. ) ;
#619=CARTESIAN_POINT ( 'NONE',  ( 1.999996625368710257, -69.28203230275519786, -9.999999999999998224 ) ) ;
#621=AXIS2_PLACEMENT_3D ( 'NONE', #34504, #28693, #34320 ) ;
#622=DIRECTION ( 'NONE',  ( 0.000000000000000000, 0.000000000000000000, 1.000000000000000000 ) ) ;
#624=ORIENTED_EDGE ( 'NONE', *, *, #18049, .F. ) ;
#625=VERTEX_POINT ( 'NONE', #19092 ) ;
#628=DIRECTION ( 'NONE',  ( -1.000000000000000000, 0.000000000000000000, 0.000000000000000000 ) ) ;
#629=DIRECTION ( 'NONE',  ( -0.000000000000000000, 0.000000000000000000, -1.000000000000000000 ) ) ;
#630=VERTEX_POINT ( 'NONE', #10639 ) ;
#631=EDGE_LOOP ( 'NONE', ( #37043, #1357 ) ) ;
#632=DIRECTION ( 'NONE',  ( -0.000000000000000000, -0.000000000000000000, 1.000000000000000000 ) ) ;
#633=EDGE_LOOP ( 'NONE', ( #17490, #25632, #16229, #1140, #21792 ) ) ;
#634=CYLINDRICAL_SURFACE ( 'NONE', #1798, 2.000000000000001776 ) ;
#635=ORIENTED_EDGE ( 'NONE', *, *, #13792, .F. ) ;
#636=CARTESIAN_POINT ( 'NONE',  ( 52.39915983220795681, 35.19434990244919703, 12.49999999999999822 ) ) ;
#637=ORIENTED_EDGE ( 'NONE', *, *, #2357, .T. ) ;
#638=ORIENTED_EDGE ( 'NONE', *, *, #3699, .F. ) ;
#639=EDGE_CURVE ( 'NONE', #14986, #12253, #2835, .T. ) ;
#640=FACE_OUTER_BOUND ( 'NONE', #21210, .T. ) ;
#642=EDGE_CURVE ( 'NONE', #7415, #15541, #36961, .T. ) ;
#644=CIRCLE ( 'NONE', #15017, 3.000000000000006661 ) ;
#645=ORIENTED_EDGE ( 'NONE', *, *, #31138, .F. ) ;
#647=FACE_OUTER_BOUND ( 'NONE', #33083, .T. ) ;
#649=ORIENTED_EDGE ( 'NONE', *, *, #1353, .F. ) ;
#650=CARTESIAN_POINT ( 'NONE',  ( 82.99999662536831124, -25.98076211353319565, -9.999999999999998224 ) ) ;
#652=ORIENTED_EDGE ( 'NONE', *, *, #5571, .T. ) ;
#655=CARTESIAN_POINT ( 'NONE',  ( 14.99999662536859901, 77.94228634059957983, -9.999999999999998224 ) ) ;
#656=DIRECTION ( 'NONE',  ( 0.000000000000000000, 0.000000000000000000, 1.000000000000000000 ) ) ;
#658=DIRECTION ( 'NONE',  ( -0.000000000000000000, -0.000000000000000000, 1.000000000000000000 ) ) ;
#659=EDGE_CURVE ( 'NONE', #25006, #4037, #16002, .T. ) ;
#660=LINE ( 'NONE', #31939, #34328 ) ;
#662=FACE_OUTER_BOUND ( 'NONE', #1246, .T. ) ;
#663=CARTESIAN_POINT ( 'NONE',  ( 62.99999662536841072, 25.98076211353318854, 17.49999999999999645 ) ) ;
#664=DIRECTION ( 'NONE',  ( 1.000000000000000000, 0.000000000000000000, 0.000000000000000000 ) ) ;
#665=ORIENTED_EDGE ( 'NONE', *, *, #34374, .T. ) ;
#666=VERTEX_POINT ( 'NONE', #28244 ) ;
#667=ORIENTED_EDGE ( 'NONE', *, *, #30676, .T. ) ;
#668=CIRCLE ( 'NONE', #30002, 2.000000000000000000 ) ;
#670=CARTESIAN_POINT ( 'NONE',  ( 0.000000000000000000, 0.000000000000000000, 12.49999999999999822 ) ) ;
#671=CARTESIAN_POINT ( 'NONE',  ( -78.00000337463094979, 17.32050807568878525, -5.000000000000000000 ) ) ;
#672=CARTESIAN_POINT ( 'NONE',  ( 67.99999662536836809, -51.96152422706639840, 12.50000000000000000 ) ) ;
#673=EDGE_CURVE ( 'NONE', #16100, #33530, #36691, .T. ) ;
#675=ORIENTED_EDGE ( 'NONE', *, *, #18137, .F. ) ;
#676=DIRECTION ( 'NONE',  ( 1.000000000000000000, 0.000000000000000000, 0.000000000000000000 ) ) ;
#678=FACE_BOUND ( 'NONE', #26621, .T. ) ;
#682=DIRECTION ( 'NONE',  ( 1.000000000000000000, 0.000000000000000000, 0.000000000000000000 ) ) ;
#683=EDGE_CURVE ( 'NONE', #26110, #31910, #34436, .T. ) ;
#686=CIRCLE ( 'NONE', #33621, 3.000000000000007550 ) ;
#688=CARTESIAN_POINT ( 'NONE',  ( 29.99999662536857770, -69.28203230275519786, 12.50000000000000000 ) ) ;
#690=DIRECTION ( 'NONE',  ( 0.000000000000000000, 0.000000000000000000, -1.000000000000000000 ) ) ;
#691=VERTEX_POINT ( 'NONE', #5196 ) ;
#693=DIRECTION ( 'NONE',  ( -1.000000000000000000, 0.000000000000000000, 0.000000000000000000 ) ) ;
#695=VERTEX_POINT ( 'NONE', #8386 ) ;
#696=ORIENTED_EDGE ( 'NONE', *, *, #22729, .F. ) ;
#697=EDGE_CURVE ( 'NONE', #34083, #21168, #25636, .T. ) ;
#698=VERTEX_POINT ( 'NONE', #11372 ) ;
#699=DIRECTION ( 'NONE',  ( -0.000000000000000000, -0.000000000000000000, -1.000000000000000000 ) ) ;
#700=PLANE ( 'NONE',  #28473 ) ;
#701=ORIENTED_EDGE ( 'NONE', *, *, #12852, .F. ) ;
#702=CIRCLE ( 'NONE', #28823, 2.000000000000001776 ) ;
#703=CARTESIAN_POINT ( 'NONE',  ( -83.00000337463092137, -25.98076211353322051, -9.999999999999998224 ) ) ;
#704=DIRECTION ( 'NONE',  ( -1.000000000000000000, 0.000000000000000000, 0.000000000000000000 ) ) ;
#706=EDGE_LOOP ( 'NONE', ( #6808, #12784, #32734, #8007 ) ) ;
#707=ORIENTED_EDGE ( 'NONE', *, *, #14675, .T. ) ;
#708=CARTESIAN_POINT ( 'NONE',  ( -45.00000337463112743, -60.62177826491080168, 12.50000000000000000 ) ) ;
#709=EDGE_CURVE ( 'NONE', #31147, #12977, #28614, .T. ) ;
#710=FACE_OUTER_BOUND ( 'NONE', #35150, .T. ) ;
#712=DIRECTION ( 'NONE',  ( 0.000000000000000000, 0.000000000000000000, 1.000000000000000000 ) ) ;
#713=ORIENTED_EDGE ( 'NONE', *, *, #26824, .T. ) ;
#714=FACE_BOUND ( 'NONE', #20933, .T. ) ;
#715=EDGE_LOOP ( 'NONE', ( #3359, #25390, #2714, #32200 ) ) ;
#716=VERTEX_POINT ( 'NONE', #23179 ) ;
#717=EDGE_CURVE ( 'NONE', #28135, #24339, #28066, .T. ) ;
#718=CARTESIAN_POINT ( 'NONE',  ( -65.00000337463102085, 25.98076211353317433, -9.999999999999998224 ) ) ;
#719=VERTEX_POINT ( 'NONE', #31606 ) ;
#722=CIRCLE ( 'NONE', #22285, 27.00000000000001776 ) ;
#723=CYLINDRICAL_SURFACE ( 'NONE', #543, 2.000000000000001776 ) ;
#725=VERTEX_POINT ( 'NONE', #2743 ) ;
#726=ORIENTED_EDGE ( 'NONE', *, *, #70, .F. ) ;
#728=ORIENTED_EDGE ( 'NONE', *, *, #34251, .T. ) ;
#729=EDGE_CURVE ( 'NONE', #6234, #9776, #26632, .T. ) ;
#730=ORIENTED_EDGE ( 'NONE', *, *, #12828, .F. ) ;
#731=VERTEX_POINT ( 'NONE', #2393 ) ;
#732=EDGE_CURVE ( 'NONE', #13981, #15311, #19439, .T. ) ;
#733=DIRECTION ( 'NONE',  ( -1.000000000000000000, 0.000000000000000000, -0.000000000000000000 ) ) ;
#734=EDGE_CURVE ( 'NONE', #35238, #6394, #7477, .T. ) ;
#736=ORIENTED_EDGE ( 'NONE', *, *, #15630, .T. ) ;
#740=ORIENTED_EDGE ( 'NONE', *, *, #13061, .T. ) ;
#741=CARTESIAN_POINT ( 'NONE',  ( -22.00000337463124112, 69.28203230275516944, -9.999999999999998224 ) ) ;
#742=AXIS2_PLACEMENT_3D ( 'NONE', #35133, #6623, #15055 ) ;
#744=PLANE ( 'NONE',  #1446 ) ;
#745=VERTEX_POINT ( 'NONE', #8736 ) ;
#746=CARTESIAN_POINT ( 'NONE',  ( 13.89091430021463935, 62.33939050065170306, 12.49999999999999822 ) ) ;
#747=CYLINDRICAL_SURFACE ( 'NONE', #18394, 2.000000000000001776 ) ;
#748=ORIENTED_EDGE ( 'NONE', *, *, #21903, .T. ) ;
#749=EDGE_LOOP ( 'NONE', ( #27988, #21421, #30787, #25803 ) ) ;
#751=FACE_OUTER_BOUND ( 'NONE', #21916, .T. ) ;
#752=DIRECTION ( 'NONE',  ( 0.000000000000000000, 0.000000000000000000, 1.000000000000000000 ) ) ;
#753=AXIS2_PLACEMENT_3D ( 'NONE', #3835, #26714, #32706 ) ;
#756=ADVANCED_FACE ( 'NONE', ( #5558 ), #5945, .F. ) ;
#757=CARTESIAN_POINT ( 'NONE',  ( -62.00000337463104927, 34.64101615137757051, 12.50000000000000000 ) ) ;
#758=DIRECTION ( 'NONE',  ( 1.000000000000000000, 0.000000000000000000, 0.000000000000000000 ) ) ;
#759=ORIENTED_EDGE ( 'NONE', *, *, #20397, .T. ) ;
#760=CARTESIAN_POINT ( 'NONE',  ( -68.00000337463099243, 34.64101615137758472, 17.49999999999999645 ) ) ;
#761=ORIENTED_EDGE ( 'NONE', *, *, #12359, .F. ) ;
#762=FACE_OUTER_BOUND ( 'NONE', #15936, .T. ) ;
#763=DIRECTION ( 'NONE',  ( 1.000000000000000000, 0.000000000000000000, 0.000000000000000000 ) ) ;
#766=ORIENTED_EDGE ( 'NONE', *, *, #35554, .F. ) ;
#767=LINE ( 'NONE', #10464, #5296 ) ;
#768=DIRECTION ( 'NONE',  ( 0.000000000000000000, 0.000000000000000000, 1.000000000000000000 ) ) ;
#769=LINE ( 'NONE', #35993, #5932 ) ;
#770=ORIENTED_EDGE ( 'NONE', *, *, #3390, .F. ) ;
#771=CARTESIAN_POINT ( 'NONE',  ( -72.00000337463100664, -17.32050807568882078, 17.49999999999999645 ) ) ;
#772=CIRCLE ( 'NONE', #2581, 3.000000000000002665 ) ;
#773=ADVANCED_FACE ( 'NONE', ( #14178 ), #33878, .F. ) ;
#775=FACE_BOUND ( 'NONE', #29543, .T. ) ;
#776=DIRECTION ( 'NONE',  ( 0.000000000000000000, 0.000000000000000000, 1.000000000000000000 ) ) ;
#778=DIRECTION ( 'NONE',  ( 0.000000000000000000, 0.000000000000000000, 1.000000000000000000 ) ) ;
#779=ORIENTED_EDGE ( 'NONE', *, *, #8998, .T. ) ;
#780=CARTESIAN_POINT ( 'NONE',  ( 62.99999662536839651, -43.30127018922199511, -5.000000000000000000 ) ) ;
#783=CARTESIAN_POINT ( 'NONE',  ( -32.00000337463119848, -69.28203230275522628, -9.999999999999998224 ) ) ;
#784=ORIENTED_EDGE ( 'NONE', *, *, #3551, .F. ) ;
#786=CARTESIAN_POINT ( 'NONE',  ( 36.97203788309026606, -58.48108235278833433, -4.999999999999997335 ) ) ;
#787=AXIS2_PLACEMENT_3D ( 'NONE', #34385, #9057, #8687 ) ;
#788=CARTESIAN_POINT ( 'NONE',  ( -60.00000337463108480, -51.96152422706641971, -9.999999999999998224 ) ) ;
#790=AXIS2_PLACEMENT_3D ( 'NONE', #20031, #32206, #6536 ) ;
#791=EDGE_LOOP ( 'NONE', ( #7696, #29616, #13253, #10658 ) ) ;
#792=VERTEX_POINT ( 'NONE', #3121 ) ;
#794=DIRECTION ( 'NONE',  ( 1.000000000000000000, 0.000000000000000000, 0.000000000000000000 ) ) ;
#795=DIRECTION ( 'NONE',  ( -1.000000000000000000, 0.000000000000000000, 0.000000000000000000 ) ) ;
#796=ORIENTED_EDGE ( 'NONE', *, *, #30510, .T. ) ;
#797=ORIENTED_EDGE ( 'NONE', *, *, #31619, .F. ) ;
#798=EDGE_LOOP ( 'NONE', ( #23448, #6697, #696, #2063 ) ) ;
#799=EDGE_CURVE ( 'NONE', #33595, #36282, #8557, .T. ) ;
#800=EDGE_CURVE ( 'NONE', #167, #22384, #5680, .T. ) ;
#801=AXIS2_PLACEMENT_3D ( 'NONE', #454, #8709, #11888 ) ;
#802=LINE ( 'NONE', #10191, #24500 ) ;
#803=CIRCLE ( 'NONE', #9770, 2.000000000000001776 ) ;
#804=ORIENTED_EDGE ( 'NONE', *, *, #25973, .T. ) ;
#807=VERTEX_POINT ( 'NONE', #1041 ) ;
#808=CYLINDRICAL_SURFACE ( 'NONE', #12350, 2.000000000000000000 ) ;
#809=EDGE_LOOP ( 'NONE', ( #29970, #18235 ) ) ;
#810=AXIS2_PLACEMENT_3D ( 'NONE', #9275, #29702, #32516 ) ;
#814=FACE_BOUND ( 'NONE', #2745, .T. ) ;
#817=ORIENTED_EDGE ( 'NONE', *, *, #3496, .F. ) ;
#818=CARTESIAN_POINT ( 'NONE',  ( 84.99999662536831124, -25.98076211353319565, 12.50000000000000000 ) ) ;
#819=DIRECTION ( 'NONE',  ( 0.000000000000000000, 0.000000000000000000, 1.000000000000000000 ) ) ;
#820=CARTESIAN_POINT ( 'NONE',  ( -45.00000337463111322, 60.62177826491077326, -5.000000000000000000 ) ) ;
#821=CIRCLE ( 'NONE', #26565, 2.000000000000001776 ) ;
#822=ORIENTED_EDGE ( 'NONE', *, *, #12407, .F. ) ;
#823=CARTESIAN_POINT ( 'NONE',  ( -70.00000337463102085, -51.96152422706641971, 12.50000000000000000 ) ) ;
#825=ORIENTED_EDGE ( 'NONE', *, *, #23189, .T. ) ;
#826=EDGE_CURVE ( 'NONE', #5699, #16797, #15258, .T. ) ;
#827=DIRECTION ( 'NONE',  ( 1.000000000000000000, 0.000000000000000000, 0.000000000000000000 ) ) ;
#828=LINE ( 'NONE', #12240, #30455 ) ;
#829=DIRECTION ( 'NONE',  ( 0.000000000000000000, 0.000000000000000000, -1.000000000000000000 ) ) ;
#830=CARTESIAN_POINT ( 'NONE',  ( -8.000003374631278419, -69.28203230275519786, 17.49999999999999645 ) ) ;
#831=AXIS2_PLACEMENT_3D ( 'NONE', #34408, #28226, #31762 ) ;
#832=DIRECTION ( 'NONE',  ( 1.000000000000000000, 0.000000000000000000, 0.000000000000000000 ) ) ;
#833=AXIS2_PLACEMENT_3D ( 'NONE', #2841, #5634, #5469 ) ;
#835=EDGE_LOOP ( 'NONE', ( #25371, #30049 ) ) ;
#836=CARTESIAN_POINT ( 'NONE',  ( 74.99999662536836809, -8.660254037844401509, -5.000000000000000000 ) ) ;
#837=CARTESIAN_POINT ( 'NONE',  ( -68.00000337463102085, -34.64101615137762025, -5.000000000000000000 ) ) ;
#840=EDGE_LOOP ( 'NONE', ( #9665, #15054 ) ) ;
#841=ORIENTED_EDGE ( 'NONE', *, *, #18335, .T. ) ;
#842=ADVANCED_FACE ( 'NONE', ( #26365 ), #3674, .F. ) ;
#846=AXIS2_PLACEMENT_3D ( 'NONE', #8926, #5744, #482 ) ;
#847=CARTESIAN_POINT ( 'NONE',  ( 29.99999662536856349, 69.28203230275518365, 17.49999999999999645 ) ) ;
#848=CARTESIAN_POINT ( 'NONE',  ( -72.00000337463100664, -2.404119930384582903E-14, -9.999999999999998224 ) ) ;
#849=ORIENTED_EDGE ( 'NONE', *, *, #6512, .F. ) ;
#850=CARTESIAN_POINT ( 'NONE',  ( -83.00000337463092137, -8.660254037844422825, -9.999999999999998224 ) ) ;
#851=EDGE_CURVE ( 'NONE', #36107, #18101, #12892, .T. ) ;
#852=ORIENTED_EDGE ( 'NONE', *, *, #32604, .T. ) ;
#853=FACE_BOUND ( 'NONE', #31139, .T. ) ;
#857=CIRCLE ( 'NONE', #21821, 2.000000000000001776 ) ;
#858=CARTESIAN_POINT ( 'NONE',  ( 0.000000000000000000, 0.000000000000000000, -5.000000000000000000 ) ) ;
#859=VERTEX_POINT ( 'NONE', #6113 ) ;
#860=LINE ( 'NONE', #3858, #22442 ) ;
#862=DIRECTION ( 'NONE',  ( -1.000000000000000000, 0.000000000000000000, 0.000000000000000000 ) ) ;
#863=AXIS2_PLACEMENT_3D ( 'NONE', #5084, #16525, #22516 ) ;
#864=FACE_OUTER_BOUND ( 'NONE', #1884, .T. ) ;
#865=DIRECTION ( 'NONE',  ( 1.000000000000000000, 0.000000000000000000, 0.000000000000000000 ) ) ;
#866=ORIENTED_EDGE ( 'NONE', *, *, #31804, .F. ) ;
#867=CARTESIAN_POINT ( 'NONE',  ( 51.67316999614278217, 68.18636315956837279, 12.50000000000000000 ) ) ;
#869=DIRECTION ( 'NONE',  ( 0.000000000000000000, 0.000000000000000000, 1.000000000000000000 ) ) ;
#870=CARTESIAN_POINT ( 'NONE',  ( 69.99999662536839651, -3.469446951953614189E-15, 12.50000000000000000 ) ) ;
#871=ORIENTED_EDGE ( 'NONE', *, *, #36928, .T. ) ;
#872=AXIS2_PLACEMENT_3D ( 'NONE', #12562, #12163, #34891 ) ;
#873=EDGE_CURVE ( 'NONE', #24444, #18009, #21278, .T. ) ;
#874=ORIENTED_EDGE ( 'NONE', *, *, #19101, .F. ) ;
#875=VERTEX_POINT ( 'NONE', #6840 ) ;
#876=CARTESIAN_POINT ( 'NONE',  ( 9.999996625368655856, -86.60254037844400443, -5.000000000000000000 ) ) ;
#878=VECTOR ( 'NONE', #28436, 1000.000000000000000 ) ;
#879=EDGE_CURVE ( 'NONE', #21303, #29936, #13484, .T. ) ;
#880=AXIS2_PLACEMENT_3D ( 'NONE', #11968, #17424, #28839 ) ;
#881=AXIS2_PLACEMENT_3D ( 'NONE', #8194, #34259, #31066 ) ;
#883=AXIS2_PLACEMENT_3D ( 'NONE', #35948, #19415, #7250 ) ;
#884=EDGE_CURVE ( 'NONE', #12035, #22989, #33869, .T. ) ;
#885=CARTESIAN_POINT ( 'NONE',  ( -77.00000337463097821, 43.30127018922197379, -9.999999999999998224 ) ) ;
#886=CARTESIAN_POINT ( 'NONE',  ( 57.99999662536842493, -51.96152422706639840, 12.50000000000000000 ) ) ;
#887=DIRECTION ( 'NONE',  ( 0.000000000000000000, 0.000000000000000000, 1.000000000000000000 ) ) ;
#889=ORIENTED_EDGE ( 'NONE', *, *, #8422, .F. ) ;
#892=ORIENTED_EDGE ( 'NONE', *, *, #31404, .F. ) ;
#894=ORIENTED_EDGE ( 'NONE', *, *, #9878, .T. ) ;
#896=VECTOR ( 'NONE', #1089, 1000.000000000000000 ) ;
#897=EDGE_CURVE ( 'NONE', #17193, #19877, #2112, .T. ) ;
#898=FACE_BOUND ( 'NONE', #36335, .T. ) ;
#899=ORIENTED_EDGE ( 'NONE', *, *, #233, .T. ) ;
#900=ORIENTED_EDGE ( 'NONE', *, *, #13295, .F. ) ;
#902=VERTEX_POINT ( 'NONE', #671 ) ;
#903=CARTESIAN_POINT ( 'NONE',  ( -63.10544949267008974, -59.98094631475026262, -5.000000000000000000 ) ) ;
#904=DIRECTION ( 'NONE',  ( 1.000000000000000000, 0.000000000000000000, 0.000000000000000000 ) ) ;
#905=DIRECTION ( 'NONE',  ( 0.000000000000000000, 0.000000000000000000, 1.000000000000000000 ) ) ;
#906=EDGE_LOOP ( 'NONE', ( #34279, #5541, #36794 ) ) ;
#907=ORIENTED_EDGE ( 'NONE', *, *, #26589, .T. ) ;
#908=ORIENTED_EDGE ( 'NONE', *, *, #1147, .T. ) ;
#909=EDGE_LOOP ( 'NONE', ( #21439, #34161, #11256, #12333, #4938 ) ) ;
#910=EDGE_CURVE ( 'NONE', #8144, #9228, #21096, .T. ) ;
#911=VERTEX_POINT ( 'NONE', #18278 ) ;
#912=AXIS2_PLACEMENT_3D ( 'NONE', #18681, #29729, #36300 ) ;
#913=DIRECTION ( 'NONE',  ( 0.000000000000000000, 0.000000000000000000, 1.000000000000000000 ) ) ;
#914=DIRECTION ( 'NONE',  ( 0.000000000000000000, 0.000000000000000000, 1.000000000000000000 ) ) ;
#915=EDGE_CURVE ( 'NONE', #21808, #7036, #34459, .T. ) ;
#917=AXIS2_PLACEMENT_3D ( 'NONE', #8500, #13762, #25212 ) ;
#918=CARTESIAN_POINT ( 'NONE',  ( -35.00000337463116296, 60.62177826491077326, -9.999999999999998224 ) ) ;
#919=DIRECTION ( 'NONE',  ( 0.000000000000000000, 0.000000000000000000, -1.000000000000000000 ) ) ;
#921=CIRCLE ( 'NONE', #14715, 27.00000000000001066 ) ;
#922=EDGE_LOOP ( 'NONE', ( #32769, #22190, #15278, #22129 ) ) ;
#923=AXIS2_PLACEMENT_3D ( 'NONE', #31422, #14380, #8742 ) ;
#924=FACE_OUTER_BOUND ( 'NONE', #20592, .T. ) ;
#925=EDGE_CURVE ( 'NONE', #25902, #22136, #23069, .T. ) ;
#926=AXIS2_PLACEMENT_3D ( 'NONE', #28788, #28957, #26356 ) ;
#928=AXIS2_PLACEMENT_3D ( 'NONE', #26837, #26283, #3955 ) ;
#929=CARTESIAN_POINT ( 'NONE',  ( 37.99999662536853151, -69.28203230275519786, 12.50000000000000000 ) ) ;
#930=ORIENTED_EDGE ( 'NONE', *, *, #5467, .F. ) ;
#931=PLANE ( 'NONE',  #1685 ) ;
#932=EDGE_CURVE ( 'NONE', #8794, #23016, #6904, .T. ) ;
#933=DIRECTION ( 'NONE',  ( 1.000000000000000000, 0.000000000000000000, 0.000000000000000000 ) ) ;
#934=EDGE_CURVE ( 'NONE', #953, #6746, #26534, .T. ) ;
#936=AXIS2_PLACEMENT_3D ( 'NONE', #30512, #16262, #33521 ) ;
#937=ORIENTED_EDGE ( 'NONE', *, *, #24324, .F. ) ;
#939=LINE ( 'NONE', #6031, #30693 ) ;
#940=DIRECTION ( 'NONE',  ( 0.000000000000000000, 0.000000000000000000, 1.000000000000000000 ) ) ;
#942=VERTEX_POINT ( 'NONE', #35187 ) ;
#943=EDGE_CURVE ( 'NONE', #36107, #2483, #9102, .T. ) ;
#944=DIRECTION ( 'NONE',  ( 0.000000000000000000, 0.000000000000000000, 1.000000000000000000 ) ) ;
#945=EDGE_CURVE ( 'NONE', #2623, #23562, #30850, .T. ) ;
#946=CARTESIAN_POINT ( 'NONE',  ( 64.99999662536839651, -60.62177826491080168, 17.49999999999999645 ) ) ;
#947=ADVANCED_FACE ( 'NONE', ( #26919 ), #20364, .F. ) ;
#948=ORIENTED_EDGE ( 'NONE', *, *, #26845, .F. ) ;
#949=EDGE_CURVE ( 'NONE', #34902, #24063, #3319, .T. ) ;
#951=CIRCLE ( 'NONE', #25501, 65.00000000000000000 ) ;
#952=CARTESIAN_POINT ( 'NONE',  ( -62.97617850287781494, -4.279621169095772615, 12.49999999999999822 ) ) ;
#953=VERTEX_POINT ( 'NONE', #16261 ) ;
#954=AXIS2_PLACEMENT_3D ( 'NONE', #30315, #18885, #12300 ) ;
#955=AXIS2_PLACEMENT_3D ( 'NONE', #4511, #24395, #36023 ) ;
#956=CIRCLE ( 'NONE', #34476, 2.000000000000000000 ) ;
#957=DIRECTION ( 'NONE',  ( 0.000000000000000000, 0.000000000000000000, 1.000000000000000000 ) ) ;
#959=CARTESIAN_POINT ( 'NONE',  ( -3.374631327851540519E-06, 86.60254037844397601, -5.000000000000000000 ) ) ;
#960=AXIS2_PLACEMENT_3D ( 'NONE', #19464, #27895, #25458 ) ;
#961=CARTESIAN_POINT ( 'NONE',  ( -75.00000337463097821, 8.660254037844374864, 12.50000000000000000 ) ) ;
#962=ORIENTED_EDGE ( 'NONE', *, *, #11615, .T. ) ;
#964=CIRCLE ( 'NONE', #30303, 2.000000000000001776 ) ;
#965=CIRCLE ( 'NONE', #3965, 2.000000000000001776 ) ;
#966=DIRECTION ( 'NONE',  ( 1.000000000000000000, 0.000000000000000000, 0.000000000000000000 ) ) ;
#967=EDGE_LOOP ( 'NONE', ( #28944, #3441 ) ) ;
#968=CARTESIAN_POINT ( 'NONE',  ( -68.00000337463100664, -17.32050807568882078, 17.49999999999999645 ) ) ;
#969=CARTESIAN_POINT ( 'NONE',  ( -50.00000337463110611, -69.28203230275519786, -9.999999999999998224 ) ) ;
#970=CARTESIAN_POINT ( 'NONE',  ( 17.99999662536861678, -69.28203230275519786, -5.000000000000000000 ) ) ;
#972=CYLINDRICAL_SURFACE ( 'NONE', #26727, 2.000000000000001776 ) ;
#973=ORIENTED_EDGE ( 'NONE', *, *, #22437, .F. ) ;
#974=DIRECTION ( 'NONE',  ( 0.000000000000000000, 0.000000000000000000, 1.000000000000000000 ) ) ;
#975=AXIS2_PLACEMENT_3D ( 'NONE', #823, #1018, #3654 ) ;
#977=DIRECTION ( 'NONE',  ( 0.000000000000000000, 0.000000000000000000, 1.000000000000000000 ) ) ;
#978=ORIENTED_EDGE ( 'NONE', *, *, #16782, .T. ) ;
#981=DIRECTION ( 'NONE',  ( 0.000000000000000000, 0.000000000000000000, 1.000000000000000000 ) ) ;
#982=AXIS2_PLACEMENT_3D ( 'NONE', #6069, #26123, #12207 ) ;
#984=CIRCLE ( 'NONE', #23122, 2.000000000000001776 ) ;
#985=VERTEX_POINT ( 'NONE', #2388 ) ;
#987=ORIENTED_EDGE ( 'NONE', *, *, #34811, .T. ) ;
#988=CIRCLE ( 'NONE', #389, 2.000000000000001776 ) ;
#989=CARTESIAN_POINT ( 'NONE',  ( -50.00000337463112032, -51.96152422706641971, -5.000000000000000000 ) ) ;
#990=CARTESIAN_POINT ( 'NONE',  ( 49.99999662536846756, 51.96152422706637708, -9.999999999999998224 ) ) ;
#992=ORIENTED_EDGE ( 'NONE', *, *, #21226, .F. ) ;
#993=ORIENTED_EDGE ( 'NONE', *, *, #35591, .T. ) ;
#994=ORIENTED_EDGE ( 'NONE', *, *, #17122, .F. ) ;
#995=VECTOR ( 'NONE', #19238, 1000.000000000000000 ) ;
#996=FACE_OUTER_BOUND ( 'NONE', #23548, .T. ) ;
#997=EDGE_LOOP ( 'NONE', ( #28170, #14819 ) ) ;
#999=FACE_OUTER_BOUND ( 'NONE', #16357, .T. ) ;
#1001=DIRECTION ( 'NONE',  ( -1.000000000000000000, 0.000000000000000000, 0.000000000000000000 ) ) ;
#1003=CIRCLE ( 'NONE', #23764, 2.000000000000001776 ) ;
#1004=EDGE_LOOP ( 'NONE', ( #26799, #907, #2975, #34427 ) ) ;
#1005=( NAMED_UNIT ( * ) SI_UNIT ( $, .STERADIAN. ) SOLID_ANGLE_UNIT ( ) );
#1006=FACE_OUTER_BOUND ( 'NONE', #8509, .T. ) ;
#1007=CIRCLE ( 'NONE', #6381, 2.000000000000001776 ) ;
#1008=CARTESIAN_POINT ( 'NONE',  ( 93.55673653615997409, 16.49657687835710362, 12.49999999999999822 ) ) ;
#1010=ORIENTED_EDGE ( 'NONE', *, *, #2395, .T. ) ;
#1014=CARTESIAN_POINT ( 'NONE',  ( 21.99999662536862033, -69.28203230275519786, -9.999999999999998224 ) ) ;
#1016=AXIS2_PLACEMENT_3D ( 'NONE', #1384, #21079, #21258 ) ;
#1017=ORIENTED_EDGE ( 'NONE', *, *, #32627, .F. ) ;
#1018=DIRECTION ( 'NONE',  ( 0.000000000000000000, 0.000000000000000000, 1.000000000000000000 ) ) ;
#1019=DIRECTION ( 'NONE',  ( 1.000000000000000000, 0.000000000000000000, 0.000000000000000000 ) ) ;
#1020=ORIENTED_EDGE ( 'NONE', *, *, #1892, .T. ) ;
#1021=DIRECTION ( 'NONE',  ( 0.000000000000000000, 0.000000000000000000, 1.000000000000000000 ) ) ;
#1022=CARTESIAN_POINT ( 'NONE',  ( -53.00000337463106348, 43.30127018922197379, -9.999999999999998224 ) ) ;
#1023=DIRECTION ( 'NONE',  ( 0.000000000000000000, 0.000000000000000000, 1.000000000000000000 ) ) ;
#1024=EDGE_CURVE ( 'NONE', #2754, #11413, #27298, .T. ) ;
#1025=CARTESIAN_POINT ( 'NONE',  ( -48.00000337463110611, -69.28203230275519786, -9.999999999999998224 ) ) ;
#1028=CARTESIAN_POINT ( 'NONE',  ( 9.999996625368655856, -69.28203230275519786, 17.49999999999999645 ) ) ;
#1029=ORIENTED_EDGE ( 'NONE', *, *, #11490, .T. ) ;
#1030=CARTESIAN_POINT ( 'NONE',  ( 77.99999662536833966, 17.32050807568879236, -9.999999999999998224 ) ) ;
#1031=CIRCLE ( 'NONE', #24408, 3.000000000000002665 ) ;
#1032=CARTESIAN_POINT ( 'NONE',  ( -56.67878100130369035, 27.78182860042797131, -4.999999999999997335 ) ) ;
#1034=CIRCLE ( 'NONE', #21993, 2.000000000000001776 ) ;
#1036=ORIENTED_EDGE ( 'NONE', *, *, #15845, .T. ) ;
#1037=ORIENTED_EDGE ( 'NONE', *, *, #29724, .T. ) ;
#1038=CIRCLE ( 'NONE', #14201, 2.000000000000001776 ) ;
#1039=FACE_OUTER_BOUND ( 'NONE', #15280, .T. ) ;
#1041=CARTESIAN_POINT ( 'NONE',  ( -23.00000337463121980, -77.94228634059963667, -9.999999999999998224 ) ) ;
#1042=CIRCLE ( 'NONE', #36971, 2.000000000000001776 ) ;
#1043=AXIS2_PLACEMENT_3D ( 'NONE', #27055, #12989, #4375 ) ;
#1044=DIRECTION ( 'NONE',  ( 1.000000000000000000, 0.000000000000000000, 0.000000000000000000 ) ) ;
#1045=CARTESIAN_POINT ( 'NONE',  ( 69.99999662536838230, -34.64101615137759183, 17.49999999999999645 ) ) ;
#1046=EDGE_LOOP ( 'NONE', ( #22360, #11853, #18757, #7790, #2460, #9786 ) ) ;
#1047=EDGE_CURVE ( 'NONE', #27815, #5261, #964, .T. ) ;
#1048=CARTESIAN_POINT ( 'NONE',  ( 44.99999662536851019, 77.94228634059959404, -9.999999999999998224 ) ) ;
#1049=ORIENTED_EDGE ( 'NONE', *, *, #165, .T. ) ;
#1050=FACE_BOUND ( 'NONE', #27215, .T. ) ;
#1051=CIRCLE ( 'NONE', #5850, 2.000000000000001776 ) ;
#1053=CIRCLE ( 'NONE', #33994, 95.00000000000001421 ) ;
#1054=VERTEX_POINT ( 'NONE', #13816 ) ;
#1055=CARTESIAN_POINT ( 'NONE',  ( -60.93295298010992411, -19.13981058454771755, 12.49999999999999822 ) ) ;
#1056=CIRCLE ( 'NONE', #24436, 2.000000000000001776 ) ;
#1057=AXIS2_PLACEMENT_3D ( 'NONE', #1167, #24039, #35484 ) ;
#1059=AXIS2_PLACEMENT_3D ( 'NONE', #21546, #35806, #33152 ) ;
#1060=DIRECTION ( 'NONE',  ( 0.000000000000000000, 0.000000000000000000, 1.000000000000000000 ) ) ;
#1061=AXIS2_PLACEMENT_3D ( 'NONE', #22379, #8133, #22771 ) ;
#1062=CARTESIAN_POINT ( 'NONE',  ( 47.63139720814418610, 27.49999999999988987, -10.00000000000000000 ) ) ;
#1063=CARTESIAN_POINT ( 'NONE',  ( -40.00000337463113453, -69.28203230275519786, -5.000000000000000000 ) ) ;
#1064=ADVANCED_FACE ( 'NONE', ( #19431 ), #5188, .F. ) ;
#1065=ORIENTED_EDGE ( 'NONE', *, *, #33685, .T. ) ;
#1066=CARTESIAN_POINT ( 'NONE',  ( 0.000000000000000000, 0.000000000000000000, -5.000000000000000000 ) ) ;
#1067=CYLINDRICAL_SURFACE ( 'NONE', #23786, 2.000000000000001776 ) ;
#1068=FACE_OUTER_BOUND ( 'NONE', #28300, .T. ) ;
#1069=EDGE_CURVE ( 'NONE', #7812, #13352, #36887, .T. ) ;
#1071=CIRCLE ( 'NONE', #5871, 2.000000000000001776 ) ;
#1072=VERTEX_POINT ( 'NONE', #27856 ) ;
#1074=EDGE_CURVE ( 'NONE', #17068, #21597, #33308, .T. ) ;
#1075=CARTESIAN_POINT ( 'NONE',  ( 0.000000000000000000, 55.00000000000000000, -10.00000000000000178 ) ) ;
#1076=AXIS2_PLACEMENT_3D ( 'NONE', #7946, #19931, #31356 ) ;
#1077=CARTESIAN_POINT ( 'NONE',  ( -27.00000337463120914, 77.94228634059957983, -9.999999999999998224 ) ) ;
#1079=EDGE_CURVE ( 'NONE', #21959, #18966, #18933, .T. ) ;
#1081=CARTESIAN_POINT ( 'NONE',  ( 70.47608876694671665, 59.13646009116074964, 12.49999999999999822 ) ) ;
#1083=AXIS2_PLACEMENT_3D ( 'NONE', #4604, #30814, #13385 ) ;
#1084=AXIS2_PLACEMENT_3D ( 'NONE', #2463, #36213, #13884 ) ;
#1085=DIRECTION ( 'NONE',  ( 0.000000000000000000, 0.000000000000000000, 1.000000000000000000 ) ) ;
#1086=EDGE_LOOP ( 'NONE', ( #35105, #22460, #36309, #3044 ) ) ;
#1087=AXIS2_PLACEMENT_3D ( 'NONE', #24691, #35407, #10071 ) ;
#1088=ORIENTED_EDGE ( 'NONE', *, *, #5950, .F. ) ;
#1089=DIRECTION ( 'NONE',  ( 0.000000000000000000, 0.000000000000000000, 1.000000000000000000 ) ) ;
#1090=AXIS2_PLACEMENT_3D ( 'NONE', #23449, #35457, #14620 ) ;
#1091=DIRECTION ( 'NONE',  ( 0.000000000000000000, 0.000000000000000000, -1.000000000000000000 ) ) ;
#1092=VERTEX_POINT ( 'NONE', #7438 ) ;
#1093=DIRECTION ( 'NONE',  ( -1.000000000000000000, 0.000000000000000000, 0.000000000000000000 ) ) ;
#1094=VERTEX_POINT ( 'NONE', #10981 ) ;
#1095=AXIS2_PLACEMENT_3D ( 'NONE', #24644, #4937, #10373 ) ;
#1096=ADVANCED_FACE ( 'NONE', ( #4641 ), #16081, .F. ) ;
#1099=ORIENTED_EDGE ( 'NONE', *, *, #3575, .F. ) ;
#1101=ORIENTED_EDGE ( 'NONE', *, *, #5950, .T. ) ;
#1102=AXIS2_PLACEMENT_3D ( 'NONE', #22107, #13103, #24557 ) ;
#1103=EDGE_CURVE ( 'NONE', #35240, #21723, #21928, .T. ) ;
#1105=DIRECTION ( 'NONE',  ( 0.000000000000000000, 0.000000000000000000, 1.000000000000000000 ) ) ;
#1108=DIRECTION ( 'NONE',  ( 1.000000000000000000, 0.000000000000000000, 0.000000000000000000 ) ) ;
#1109=EDGE_CURVE ( 'NONE', #15541, #7415, #6337, .T. ) ;
#1110=VERTEX_POINT ( 'NONE', #16626 ) ;
#1111=ORIENTED_EDGE ( 'NONE', *, *, #5859, .T. ) ;
#1112=AXIS2_PLACEMENT_3D ( 'NONE', #7901, #19336, #19521 ) ;
#1113=ORIENTED_EDGE ( 'NONE', *, *, #12601, .F. ) ;
#1114=CIRCLE ( 'NONE', #35845, 2.000000000000000000 ) ;
#1115=ORIENTED_EDGE ( 'NONE', *, *, #14379, .F. ) ;
#1116=VECTOR ( 'NONE', #33369, 1000.000000000000000 ) ;
#1117=ORIENTED_EDGE ( 'NONE', *, *, #28870, .T. ) ;
#1118=DIRECTION ( 'NONE',  ( 1.000000000000000000, 0.000000000000000000, 0.000000000000000000 ) ) ;
#1120=ORIENTED_EDGE ( 'NONE', *, *, #709, .T. ) ;
#1121=DIRECTION ( 'NONE',  ( -1.000000000000000000, 0.000000000000000000, 0.000000000000000000 ) ) ;
#1123=DIRECTION ( 'NONE',  ( 0.000000000000000000, 0.000000000000000000, 1.000000000000000000 ) ) ;
#1125=VERTEX_POINT ( 'NONE', #36130 ) ;
#1127=AXIS2_PLACEMENT_3D ( 'NONE', #25556, #11105, #22757 ) ;
#1128=CARTESIAN_POINT ( 'NONE',  ( 2.999996625368645198, 77.94228634059957983, 12.50000000000000000 ) ) ;
#1129=EDGE_CURVE ( 'NONE', #35481, #15444, #20708, .T. ) ;
#1130=DIRECTION ( 'NONE',  ( 0.000000000000000000, 0.000000000000000000, 1.000000000000000000 ) ) ;
#1131=ORIENTED_EDGE ( 'NONE', *, *, #27826, .T. ) ;
#1132=DIRECTION ( 'NONE',  ( 0.000000000000000000, 0.000000000000000000, 1.000000000000000000 ) ) ;
#1133=CARTESIAN_POINT ( 'NONE',  ( 21.99999662536859191, 69.28203230275516944, -9.999999999999998224 ) ) ;
#1134=ORIENTED_EDGE ( 'NONE', *, *, #35531, .T. ) ;
#1135=VERTEX_POINT ( 'NONE', #28239 ) ;
#1137=VECTOR ( 'NONE', #19117, 1000.000000000000000 ) ;
#1138=LINE ( 'NONE', #32821, #11547 ) ;
#1139=DIRECTION ( 'NONE',  ( 0.000000000000000000, 0.000000000000000000, 1.000000000000000000 ) ) ;
#1140=ORIENTED_EDGE ( 'NONE', *, *, #5610, .F. ) ;
#1141=CIRCLE ( 'NONE', #14312, 2.000000000000001776 ) ;
#1142=DIRECTION ( 'NONE',  ( 0.000000000000000000, 0.000000000000000000, 1.000000000000000000 ) ) ;
#1143=DIRECTION ( 'NONE',  ( 1.000000000000000000, 0.000000000000000000, 0.000000000000000000 ) ) ;
#1144=ADVANCED_FACE ( 'NONE', ( #2556 ), #28058, .F. ) ;
#1145=ORIENTED_EDGE ( 'NONE', *, *, #27137, .T. ) ;
#1146=AXIS2_PLACEMENT_3D ( 'NONE', #33482, #1791, #19048 ) ;
#1147=EDGE_CURVE ( 'NONE', #8445, #4612, #10257, .T. ) ;
#1148=LINE ( 'NONE', #15588, #32767 ) ;
#1149=ORIENTED_EDGE ( 'NONE', *, *, #2072, .F. ) ;
#1150=AXIS2_PLACEMENT_3D ( 'NONE', #16145, #35836, #30371 ) ;
#1151=DIRECTION ( 'NONE',  ( 1.000000000000000000, 0.000000000000000000, 0.000000000000000000 ) ) ;
#1152=EDGE_CURVE ( 'NONE', #3514, #5093, #3808, .T. ) ;
#1153=DIRECTION ( 'NONE',  ( -0.000000000000000000, -0.000000000000000000, 1.000000000000000000 ) ) ;
#1154=AXIS2_PLACEMENT_3D ( 'NONE', #29769, #23981, #32780 ) ;
#1155=DIRECTION ( 'NONE',  ( 1.000000000000000000, 0.000000000000000000, 0.000000000000000000 ) ) ;
#1156=EDGE_CURVE ( 'NONE', #30650, #21828, #6105, .T. ) ;
#1157=ORIENTED_EDGE ( 'NONE', *, *, #34773, .T. ) ;
#1158=AXIS2_PLACEMENT_3D ( 'NONE', #18655, #15470, #18473 ) ;
#1159=ORIENTED_EDGE ( 'NONE', *, *, #12376, .F. ) ;
#1160=ADVANCED_FACE ( 'NONE', ( #104 ), #36862, .F. ) ;
#1161=ADVANCED_FACE ( 'NONE', ( #2940 ), #9094, .F. ) ;
#1162=AXIS2_PLACEMENT_3D ( 'NONE', #27745, #7331, #35846 ) ;
#1165=VECTOR ( 'NONE', #23204, 1000.000000000000000 ) ;
#1167=CARTESIAN_POINT ( 'NONE',  ( 64.99999662536841072, -25.98076211353320275, 17.49999999999999645 ) ) ;
#1168=CARTESIAN_POINT ( 'NONE',  ( -73.00000337463097821, -8.660254037844422825, -5.000000000000000000 ) ) ;
#1169=CARTESIAN_POINT ( 'NONE',  ( -8.000003374631249997, -86.60254037844400443, -9.999999999999998224 ) ) ;
#1170=EDGE_CURVE ( 'NONE', #9726, #1919, #14589, .T. ) ;
#1171=ORIENTED_EDGE ( 'NONE', *, *, #26583, .T. ) ;
#1173=EDGE_CURVE ( 'NONE', #17720, #12612, #31236, .T. ) ;
#1175=EDGE_CURVE ( 'NONE', #30254, #25902, #5739, .T. ) ;
#1176=LINE ( 'NONE', #20856, #10978 ) ;
#1177=ORIENTED_EDGE ( 'NONE', *, *, #12201, .T. ) ;
#1178=CARTESIAN_POINT ( 'NONE',  ( -34.00000000000027711, -58.88972745734168512, -4.999999999999997335 ) ) ;
#1180=DIRECTION ( 'NONE',  ( -0.000000000000000000, -0.000000000000000000, 1.000000000000000000 ) ) ;
#1181=AXIS2_PLACEMENT_3D ( 'NONE', #26923, #11728, #23741 ) ;
#1182=EDGE_LOOP ( 'NONE', ( #19164, #37024 ) ) ;
#1183=ORIENTED_EDGE ( 'NONE', *, *, #215, .F. ) ;
#1184=DIRECTION ( 'NONE',  ( 1.000000000000000000, 0.000000000000000000, 0.000000000000000000 ) ) ;
#1185=CARTESIAN_POINT ( 'NONE',  ( 69.99999662536839651, 34.64101615137758472, 12.50000000000000000 ) ) ;
#1186=CARTESIAN_POINT ( 'NONE',  ( -53.00000337463109190, -60.62177826491083010, -9.999999999999998224 ) ) ;
#1189=AXIS2_PLACEMENT_3D ( 'NONE', #28308, #7717, #13883 ) ;
#1191=CARTESIAN_POINT ( 'NONE',  ( -50.00000337463109190, 69.28203230275518365, -9.999999999999998224 ) ) ;
#1192=EDGE_CURVE ( 'NONE', #12047, #25810, #10398, .T. ) ;
#1193=ORIENTED_EDGE ( 'NONE', *, *, #196, .T. ) ;
#1194=ADVANCED_FACE ( 'NONE', ( #37063 ), #17719, .F. ) ;
#1195=VERTEX_POINT ( 'NONE', #20169 ) ;
#1197=ORIENTED_EDGE ( 'NONE', *, *, #18865, .T. ) ;
#1198=ORIENTED_EDGE ( 'NONE', *, *, #21038, .T. ) ;
#1199=DIRECTION ( 'NONE',  ( 0.000000000000000000, 0.000000000000000000, 1.000000000000000000 ) ) ;
#1200=DIRECTION ( 'NONE',  ( -0.000000000000000000, -0.000000000000000000, 1.000000000000000000 ) ) ;
#1201=ORIENTED_EDGE ( 'NONE', *, *, #3906, .T. ) ;
#1202=ORIENTED_EDGE ( 'NONE', *, *, #22250, .T. ) ;
#1203=EDGE_CURVE ( 'NONE', #14529, #21657, #26559, .T. ) ;
#1205=DIRECTION ( 'NONE',  ( 1.000000000000000000, 0.000000000000000000, 0.000000000000000000 ) ) ;
#1207=CYLINDRICAL_SURFACE ( 'NONE', #4899, 95.00000000000000000 ) ;
#1210=CARTESIAN_POINT ( 'NONE',  ( -23.00000337463120559, 77.94228634059957983, -5.000000000000000000 ) ) ;
#1211=ORIENTED_EDGE ( 'NONE', *, *, #22703, .F. ) ;
#1212=AXIS2_PLACEMENT_3D ( 'NONE', #6059, #25767, #35115 ) ;
#1213=DIRECTION ( 'NONE',  ( 0.000000000000000000, 0.000000000000000000, -1.000000000000000000 ) ) ;
#1216=CYLINDRICAL_SURFACE ( 'NONE', #1016, 2.000000000000001776 ) ;
#1218=DIRECTION ( 'NONE',  ( 0.000000000000000000, 0.000000000000000000, 1.000000000000000000 ) ) ;
#1219=EDGE_CURVE ( 'NONE', #26696, #14320, #21772, .T. ) ;
#1220=CARTESIAN_POINT ( 'NONE',  ( 69.99999662536839651, -17.32050807568879947, -9.999999999999998224 ) ) ;
#1221=EDGE_CURVE ( 'NONE', #29589, #29318, #16985, .T. ) ;
#1222=EDGE_CURVE ( 'NONE', #29771, #34151, #3222, .T. ) ;
#1223=DIRECTION ( 'NONE',  ( -1.000000000000000000, 0.000000000000000000, 0.000000000000000000 ) ) ;
#1225=DIRECTION ( 'NONE',  ( 0.000000000000000000, 0.000000000000000000, 1.000000000000000000 ) ) ;
#1226=DIRECTION ( 'NONE',  ( 0.8660254037844344888, -0.5000000000000069944, 0.000000000000000000 ) ) ;
#1227=CARTESIAN_POINT ( 'NONE',  ( 82.99999662536831124, -25.98076211353319565, -5.000000000000000000 ) ) ;
#1230=ORIENTED_EDGE ( 'NONE', *, *, #7457, .F. ) ;
#1231=DIRECTION ( 'NONE',  ( -1.000000000000000000, 0.000000000000000000, 0.000000000000000000 ) ) ;
#1234=AXIS2_PLACEMENT_3D ( 'NONE', #35121, #9785, #9429 ) ;
#1235=DIRECTION ( 'NONE',  ( 1.000000000000000000, 0.000000000000000000, 0.000000000000000000 ) ) ;
#1236=FACE_OUTER_BOUND ( 'NONE', #31327, .T. ) ;
#1237=CARTESIAN_POINT ( 'NONE',  ( -75.00000337463097821, 43.30127018922197379, 17.49999999999999645 ) ) ;
#1239=FACE_OUTER_BOUND ( 'NONE', #35151, .T. ) ;
#1240=ORIENTED_EDGE ( 'NONE', *, *, #2218, .T. ) ;
#1241=FACE_BOUND ( 'NONE', #25011, .T. ) ;
#1242=EDGE_CURVE ( 'NONE', #8606, #35191, #24182, .T. ) ;
#1246=EDGE_LOOP ( 'NONE', ( #23678, #30155, #171, #5798 ) ) ;
#1247=DIRECTION ( 'NONE',  ( -0.000000000000000000, -0.000000000000000000, 1.000000000000000000 ) ) ;
#1249=DIRECTION ( 'NONE',  ( 0.000000000000000000, 0.000000000000000000, 1.000000000000000000 ) ) ;
#1250=DIRECTION ( 'NONE',  ( -1.000000000000000000, 0.000000000000000000, 0.000000000000000000 ) ) ;
#1251=DIRECTION ( 'NONE',  ( 1.000000000000000000, 0.000000000000000000, 0.000000000000000000 ) ) ;
#1252=ORIENTED_EDGE ( 'NONE', *, *, #7122, .T. ) ;
#1253=DIRECTION ( 'NONE',  ( 0.000000000000000000, 0.000000000000000000, 1.000000000000000000 ) ) ;
#1254=CARTESIAN_POINT ( 'NONE',  ( 54.99999662536844625, 60.62177826491077326, -9.999999999999998224 ) ) ;
#1255=DIRECTION ( 'NONE',  ( 0.000000000000000000, 0.000000000000000000, 1.000000000000000000 ) ) ;
#1256=ORIENTED_EDGE ( 'NONE', *, *, #13954, .F. ) ;
#1257=ORIENTED_EDGE ( 'NONE', *, *, #6342, .T. ) ;
#1258=AXIS2_PLACEMENT_3D ( 'NONE', #15742, #21175, #12552 ) ;
#1259=EDGE_CURVE ( 'NONE', #36782, #30643, #4413, .T. ) ;
#1260=ORIENTED_EDGE ( 'NONE', *, *, #23433, .T. ) ;
#1261=DIRECTION ( 'NONE',  ( 1.000000000000000000, 0.000000000000000000, 0.000000000000000000 ) ) ;
#1264=CARTESIAN_POINT ( 'NONE',  ( 0.000000000000000000, 0.000000000000000000, -5.000000000000000000 ) ) ;
#1265=CARTESIAN_POINT ( 'NONE',  ( 59.99999662536842493, -51.96152422706639840, -5.000000000000000000 ) ) ;
#1266=APPLICATION_CONTEXT ( 'automotive_design' ) ;
#1267=FACE_OUTER_BOUND ( 'NONE', #16876, .T. ) ;
#1268=EDGE_LOOP ( 'NONE', ( #35515, #24367, #17572, #340 ) ) ;
#1270=DIRECTION ( 'NONE',  ( 0.000000000000000000, 0.000000000000000000, 1.000000000000000000 ) ) ;
#1271=CARTESIAN_POINT ( 'NONE',  ( -56.29165124598871017, -32.49999999999966604, 12.49999999999999822 ) ) ;
#1272=EDGE_LOOP ( 'NONE', ( #23070, #25854, #7139 ) ) ;
#1273=DIRECTION ( 'NONE',  ( 1.000000000000000000, 0.000000000000000000, 0.000000000000000000 ) ) ;
#1274=ORIENTED_EDGE ( 'NONE', *, *, #34814, .F. ) ;
#1275=AXIS2_PLACEMENT_3D ( 'NONE', #35835, #10142, #4887 ) ;
#1276=CARTESIAN_POINT ( 'NONE',  ( 4.279621169095998212, -62.97617850287780072, -4.999999999999997335 ) ) ;
#1277=EDGE_CURVE ( 'NONE', #32298, #9210, #18783, .T. ) ;
#1278=CARTESIAN_POINT ( 'NONE',  ( 49.99999662536846756, -69.28203230275519786, 12.50000000000000000 ) ) ;
#1279=ORIENTED_EDGE ( 'NONE', *, *, #8302, .F. ) ;
#1280=ORIENTED_EDGE ( 'NONE', *, *, #25146, .F. ) ;
#1281=EDGE_CURVE ( 'NONE', #28577, #28380, #32553, .T. ) ;
#1282=DIRECTION ( 'NONE',  ( 1.000000000000000000, 0.000000000000000000, 0.000000000000000000 ) ) ;
#1286=ADVANCED_FACE ( 'NONE', ( #10030 ), #17919, .T. ) ;
#1287=DIRECTION ( 'NONE',  ( -1.000000000000000000, 0.000000000000000000, 0.000000000000000000 ) ) ;
#1288=DIRECTION ( 'NONE',  ( 0.000000000000000000, 0.000000000000000000, 1.000000000000000000 ) ) ;
#1289=ORIENTED_EDGE ( 'NONE', *, *, #35342, .F. ) ;
#1290=ORIENTED_EDGE ( 'NONE', *, *, #13014, .F. ) ;
#1291=ORIENTED_EDGE ( 'NONE', *, *, #35469, .T. ) ;
#1292=ORIENTED_EDGE ( 'NONE', *, *, #28666, .T. ) ;
#1295=EDGE_CURVE ( 'NONE', #4453, #33934, #25980, .T. ) ;
#1296=LINE ( 'NONE', #9915, #16803 ) ;
#1298=VECTOR ( 'NONE', #940, 1000.000000000000000 ) ;
#1299=CARTESIAN_POINT ( 'NONE',  ( -56.56139351304917540, -61.87160258682602176, 12.50000000000000000 ) ) ;
#1300=DIRECTION ( 'NONE',  ( 1.000000000000000000, 0.000000000000000000, 0.000000000000000000 ) ) ;
#1301=CARTESIAN_POINT ( 'NONE',  ( -80.00000337463094979, 34.64101615137757051, -9.999999999999998224 ) ) ;
#1302=ORIENTED_EDGE ( 'NONE', *, *, #17801, .T. ) ;
#1303=CARTESIAN_POINT ( 'NONE',  ( 69.99999662536841072, 51.96152422706640550, -9.999999999999998224 ) ) ;
#1304=CARTESIAN_POINT ( 'NONE',  ( 26.97173338359068850, -77.60724282659606388, 12.50000000000000000 ) ) ;
#1306=ORIENTED_EDGE ( 'NONE', *, *, #5534, .F. ) ;
#1309=ORIENTED_EDGE ( 'NONE', *, *, #28870, .F. ) ;
#1310=EDGE_CURVE ( 'NONE', #14745, #34871, #16401, .T. ) ;
#1312=DIRECTION ( 'NONE',  ( 0.000000000000000000, 0.000000000000000000, 1.000000000000000000 ) ) ;
#1313=EDGE_CURVE ( 'NONE', #11967, #18936, #28347, .T. ) ;
#1314=CARTESIAN_POINT ( 'NONE',  ( -68.19171733629717380, 52.81598405851951838, -5.000000000000000000 ) ) ;
#1315=DIRECTION ( 'NONE',  ( -0.000000000000000000, -0.000000000000000000, 1.000000000000000000 ) ) ;
#1316=DIRECTION ( 'NONE',  ( 1.000000000000000000, 0.000000000000000000, 0.000000000000000000 ) ) ;
#1317=EDGE_LOOP ( 'NONE', ( #22354, #5648 ) ) ;
#1319=EDGE_CURVE ( 'NONE', #11639, #9216, #27762, .T. ) ;
#1320=CARTESIAN_POINT ( 'NONE',  ( 56.67878100130369035, -27.78182860042797131, -4.999999999999997335 ) ) ;
#1321=DIRECTION ( 'NONE',  ( 1.000000000000000000, 0.000000000000000000, 0.000000000000000000 ) ) ;
#1322=ORIENTED_EDGE ( 'NONE', *, *, #27528, .T. ) ;
#1324=ADVANCED_FACE ( 'NONE', ( #29903 ), #23727, .F. ) ;
#1325=CARTESIAN_POINT ( 'NONE',  ( 71.99999662536841072, 51.96152422706640550, -9.999999999999998224 ) ) ;
#1326=ORIENTED_EDGE ( 'NONE', *, *, #5342, .F. ) ;
#1328=LINE ( 'NONE', #27392, #230 ) ;
#1330=DIRECTION ( 'NONE',  ( 1.000000000000000000, 0.000000000000000000, 0.000000000000000000 ) ) ;
#1331=ORIENTED_EDGE ( 'NONE', *, *, #33702, .F. ) ;
#1332=EDGE_LOOP ( 'NONE', ( #26969, #10374, #12947, #269 ) ) ;
#1333=VECTOR ( 'NONE', #12576, 1000.000000000000000 ) ;
#1334=VECTOR ( 'NONE', #7184, 1000.000000000000000 ) ;
#1335=EDGE_LOOP ( 'NONE', ( #28851, #36850, #26335, #27471 ) ) ;
#1336=CARTESIAN_POINT ( 'NONE',  ( -35.00000337463116296, -60.62177826491080168, 17.49999999999999645 ) ) ;
#1337=CARTESIAN_POINT ( 'NONE',  ( 0.000000000000000000, 0.000000000000000000, -10.00000000000000000 ) ) ;
#1338=CARTESIAN_POINT ( 'NONE',  ( -75.00000337463097821, 8.660254037844374864, -9.999999999999998224 ) ) ;
#1339=CARTESIAN_POINT ( 'NONE',  ( -53.00000337463109190, -60.62177826491083010, -9.999999999999998224 ) ) ;
#1340=CARTESIAN_POINT ( 'NONE',  ( -3.374631327851540519E-06, 86.60254037844397601, -9.999999999999998224 ) ) ;
#1341=EDGE_LOOP ( 'NONE', ( #33053, #4985, #34509, #5482 ) ) ;
#1342=CARTESIAN_POINT ( 'NONE',  ( 0.000000000000000000, 0.000000000000000000, -10.00000000000000000 ) ) ;
#1343=ADVANCED_FACE ( 'NONE', ( #20710 ), #12251, .F. ) ;
#1344=DIRECTION ( 'NONE',  ( 0.8660254037844415942, 0.4999999999999949485, 0.000000000000000000 ) ) ;
#1346=FACE_OUTER_BOUND ( 'NONE', #19597, .T. ) ;
#1347=ORIENTED_EDGE ( 'NONE', *, *, #9423, .F. ) ;
#1348=CARTESIAN_POINT ( 'NONE',  ( -30.99999999999944933, 58.88972745734214698, -4.999999999999997335 ) ) ;
#1349=CARTESIAN_POINT ( 'NONE',  ( -60.00000337463107059, -34.64101615137762025, 17.49999999999999645 ) ) ;
#1350=ORIENTED_EDGE ( 'NONE', *, *, #33790, .T. ) ;
#1351=ADVANCED_FACE ( 'NONE', ( #35723 ), #29348, .F. ) ;
#1352=ORIENTED_EDGE ( 'NONE', *, *, #28011, .F. ) ;
#1353=EDGE_CURVE ( 'NONE', #7436, #25823, #3667, .T. ) ;
#1354=CARTESIAN_POINT ( 'NONE',  ( -65.00000337463104927, -43.30127018922202353, 17.49999999999999645 ) ) ;
#1356=DIRECTION ( 'NONE',  ( 1.000000000000000000, 0.000000000000000000, 0.000000000000000000 ) ) ;
#1357=ORIENTED_EDGE ( 'NONE', *, *, #14392, .T. ) ;
#1359=EDGE_LOOP ( 'NONE', ( #6598, #23396 ) ) ;
#1360=CARTESIAN_POINT ( 'NONE',  ( 74.99999662536836809, -8.660254037844401509, -9.999999999999998224 ) ) ;
#1361=AXIS2_PLACEMENT_3D ( 'NONE', #16489, #36922, #30568 ) ;
#1362=VERTEX_POINT ( 'NONE', #9664 ) ;
#1364=DIRECTION ( 'NONE',  ( 0.000000000000000000, 0.000000000000000000, -1.000000000000000000 ) ) ;
#1365=ORIENTED_EDGE ( 'NONE', *, *, #257, .T. ) ;
#1366=ORIENTED_EDGE ( 'NONE', *, *, #25560, .T. ) ;
#1367=CARTESIAN_POINT ( 'NONE',  ( -3.108944973436880588, -78.59336093177338967, 12.50000000000000000 ) ) ;
#1369=VECTOR ( 'NONE', #22116, 1000.000000000000000 ) ;
#1370=CARTESIAN_POINT ( 'NONE',  ( 57.99999662536843914, -34.64101615137759893, -9.999999999999998224 ) ) ;
#1372=CIRCLE ( 'NONE', #19925, 2.000000000000001776 ) ;
#1373=VERTEX_POINT ( 'NONE', #20919 ) ;
#1376=FACE_OUTER_BOUND ( 'NONE', #29442, .T. ) ;
#1377=LINE ( 'NONE', #23349, #6509 ) ;
#1378=ORIENTED_EDGE ( 'NONE', *, *, #31, .F. ) ;
#1379=DIRECTION ( 'NONE',  ( 0.000000000000000000, 0.000000000000000000, 1.000000000000000000 ) ) ;
#1380=ORIENTED_EDGE ( 'NONE', *, *, #29534, .T. ) ;
#1382=CYLINDRICAL_SURFACE ( 'NONE', #34584, 2.000000000000001776 ) ;
#1384=CARTESIAN_POINT ( 'NONE',  ( 64.99999662536841072, -25.98076211353320275, -9.999999999999998224 ) ) ;
#1385=CARTESIAN_POINT ( 'NONE',  ( -85.00000337463092137, -8.660254037844422825, -9.999999999999998224 ) ) ;
#1386=DIRECTION ( 'NONE',  ( 0.000000000000000000, 0.000000000000000000, 1.000000000000000000 ) ) ;
#1387=EDGE_CURVE ( 'NONE', #4724, #15870, #6159, .T. ) ;
#1392=DIRECTION ( 'NONE',  ( 0.000000000000000000, 0.000000000000000000, -1.000000000000000000 ) ) ;
#1393=CARTESIAN_POINT ( 'NONE',  ( 74.99999662536836809, 25.98076211353319565, -9.999999999999998224 ) ) ;
#1394=DIRECTION ( 'NONE',  ( 0.000000000000000000, 0.000000000000000000, 1.000000000000000000 ) ) ;
#1395=VERTEX_POINT ( 'NONE', #24094 ) ;
#1396=EDGE_CURVE ( 'NONE', #24986, #6951, #24134, .T. ) ;
#1397=EDGE_LOOP ( 'NONE', ( #635, #19656 ) ) ;
#1399=AXIS2_PLACEMENT_3D ( 'NONE', #7948, #21648, #16029 ) ;
#1401=CARTESIAN_POINT ( 'NONE',  ( 57.99999662536842493, 51.96152422706639129, -5.000000000000000000 ) ) ;
#1404=ORIENTED_EDGE ( 'NONE', *, *, #31414, .F. ) ;
#1405=EDGE_CURVE ( 'NONE', #5493, #24286, #18269, .T. ) ;
#1406=CARTESIAN_POINT ( 'NONE',  ( -2.000003374631289521, -69.28203230275519786, -5.000000000000000000 ) ) ;
#1407=DIRECTION ( 'NONE',  ( 0.000000000000000000, 0.000000000000000000, 1.000000000000000000 ) ) ;
#1409=DIRECTION ( 'NONE',  ( 1.000000000000000000, 0.000000000000000000, 0.000000000000000000 ) ) ;
#1410=VERTEX_POINT ( 'NONE', #1227 ) ;
#1411=FACE_BOUND ( 'NONE', #34304, .T. ) ;
#1412=EDGE_CURVE ( 'NONE', #17343, #8449, #18127, .T. ) ;
#1414=CIRCLE ( 'NONE', #27771, 2.000000000000001776 ) ;
#1415=DIRECTION ( 'NONE',  ( 1.000000000000000000, 0.000000000000000000, 0.000000000000000000 ) ) ;
#1416=CARTESIAN_POINT ( 'NONE',  ( -20.00000337463123756, -69.28203230275522628, -9.999999999999998224 ) ) ;
#1417=ADVANCED_FACE ( 'NONE', ( #10941 ), #24478, .F. ) ;
#1418=ADVANCED_FACE ( 'NONE', ( #4952 ), #35918, .F. ) ;
#1421=CARTESIAN_POINT ( 'NONE',  ( 56.67878100130369035, -27.78182860042797131, -4.999999999999997335 ) ) ;
#1423=CARTESIAN_POINT ( 'NONE',  ( 42.99999662536850309, -60.62177826491080168, -9.999999999999998224 ) ) ;
#1426=DIRECTION ( 'NONE',  ( 1.000000000000000000, 0.000000000000000000, 0.000000000000000000 ) ) ;
#1427=EDGE_LOOP ( 'NONE', ( #9390, #29158 ) ) ;
#1428=DIRECTION ( 'NONE',  ( 0.000000000000000000, 0.000000000000000000, 1.000000000000000000 ) ) ;
#1431=ORIENTED_EDGE ( 'NONE', *, *, #16531, .F. ) ;
#1433=DIRECTION ( 'NONE',  ( 0.000000000000000000, 0.000000000000000000, 1.000000000000000000 ) ) ;
#1434=CARTESIAN_POINT ( 'NONE',  ( -12.97563234535667753, 90.60231327712331506, 12.49999999999999822 ) ) ;
#1435=CIRCLE ( 'NONE', #13418, 1.999999999999998224 ) ;
#1436=DIRECTION ( 'NONE',  ( -1.000000000000000000, 0.000000000000000000, 0.000000000000000000 ) ) ;
#1437=ORIENTED_EDGE ( 'NONE', *, *, #3221, .F. ) ;
#1438=DIRECTION ( 'NONE',  ( 0.000000000000000000, 0.000000000000000000, 1.000000000000000000 ) ) ;
#1439=DIRECTION ( 'NONE',  ( 0.000000000000000000, 0.000000000000000000, -1.000000000000000000 ) ) ;
#1441=DIRECTION ( 'NONE',  ( 1.000000000000000000, 0.000000000000000000, 0.000000000000000000 ) ) ;
#1443=VECTOR ( 'NONE', #18597, 1000.000000000000000 ) ;
#1444=EDGE_LOOP ( 'NONE', ( #13748, #34243, #10343, #4834 ) ) ;
#1445=CARTESIAN_POINT ( 'NONE',  ( -67.00000337463102085, 43.30127018922198801, -5.000000000000000000 ) ) ;
#1446=AXIS2_PLACEMENT_3D ( 'NONE', #12156, #3929, #12722 ) ;
#1447=CARTESIAN_POINT ( 'NONE',  ( -47.00000337463112743, -60.62177826491080168, -5.000000000000000000 ) ) ;
#1448=ORIENTED_EDGE ( 'NONE', *, *, #31242, .F. ) ;
#1449=DIRECTION ( 'NONE',  ( 1.000000000000000000, 0.000000000000000000, 0.000000000000000000 ) ) ;
#1450=VERTEX_POINT ( 'NONE', #33079 ) ;
#1451=DIRECTION ( 'NONE',  ( 0.000000000000000000, 0.000000000000000000, -1.000000000000000000 ) ) ;
#1452=FACE_BOUND ( 'NONE', #19243, .T. ) ;
#1453=EDGE_LOOP ( 'NONE', ( #36341, #23972 ) ) ;
#1454=EDGE_LOOP ( 'NONE', ( #18816, #5074, #35697, #7195 ) ) ;
#1455=ADVANCED_FACE ( 'NONE', ( #1583 ), #7952, .F. ) ;
#1457=DIRECTION ( 'NONE',  ( -1.000000000000000000, 0.000000000000000000, -0.000000000000000000 ) ) ;
#1460=DIRECTION ( 'NONE',  ( 0.000000000000000000, 0.000000000000000000, 1.000000000000000000 ) ) ;
#1461=CARTESIAN_POINT ( 'NONE',  ( 49.99999662536848177, -51.96152422706640550, -9.999999999999998224 ) ) ;
#1462=DIRECTION ( 'NONE',  ( -0.000000000000000000, -0.000000000000000000, 1.000000000000000000 ) ) ;
#1463=ORIENTED_EDGE ( 'NONE', *, *, #22294, .F. ) ;
#1464=CARTESIAN_POINT ( 'NONE',  ( -70.00000337463099243, -2.428612866367529932E-14, -5.000000000000000000 ) ) ;
#1465=CYLINDRICAL_SURFACE ( 'NONE', #16620, 2.000000000000001776 ) ;
#1466=EDGE_LOOP ( 'NONE', ( #1037, #34759 ) ) ;
#1467=CIRCLE ( 'NONE', #8064, 27.00000000000001776 ) ;
#1469=ORIENTED_EDGE ( 'NONE', *, *, #25869, .F. ) ;
#1470=DIRECTION ( 'NONE',  ( -1.000000000000000000, 0.000000000000000000, -0.000000000000000000 ) ) ;
#1471=CIRCLE ( 'NONE', #801, 33.00000000000001421 ) ;
#1472=DIRECTION ( 'NONE',  ( 0.000000000000000000, 0.000000000000000000, 1.000000000000000000 ) ) ;
#1473=VERTEX_POINT ( 'NONE', #30259 ) ;
#1474=CARTESIAN_POINT ( 'NONE',  ( 21.99999662536862033, -86.60254037844400443, -9.999999999999998224 ) ) ;
#1475=DIRECTION ( 'NONE',  ( 1.000000000000000000, 0.000000000000000000, 0.000000000000000000 ) ) ;
#1476=EDGE_CURVE ( 'NONE', #7505, #6635, #33092, .T. ) ;
#1477=ORIENTED_EDGE ( 'NONE', *, *, #35526, .F. ) ;
#1478=FACE_OUTER_BOUND ( 'NONE', #30171, .T. ) ;
#1479=EDGE_CURVE ( 'NONE', #4566, #16555, #10953, .T. ) ;
#1480=CARTESIAN_POINT ( 'NONE',  ( 47.99999662536846756, 51.96152422706637708, -9.999999999999998224 ) ) ;
#1481=AXIS2_PLACEMENT_3D ( 'NONE', #17552, #6123, #28977 ) ;
#1482=DIRECTION ( 'NONE',  ( 0.000000000000000000, 0.000000000000000000, 1.000000000000000000 ) ) ;
#1483=DIRECTION ( 'NONE',  ( 0.000000000000000000, 0.000000000000000000, 1.000000000000000000 ) ) ;
#1486=CARTESIAN_POINT ( 'NONE',  ( -63.00000337463102085, 43.30127018922198801, -9.999999999999998224 ) ) ;
#1489=ORIENTED_EDGE ( 'NONE', *, *, #31945, .T. ) ;
#1491=CARTESIAN_POINT ( 'NONE',  ( -71.20512444582767841, -36.23716251175871861, 12.50000000000000000 ) ) ;
#1492=DIRECTION ( 'NONE',  ( -1.000000000000000000, 0.000000000000000000, 0.000000000000000000 ) ) ;
#1493=DIRECTION ( 'NONE',  ( 0.000000000000000000, 0.000000000000000000, 1.000000000000000000 ) ) ;
#1494=CARTESIAN_POINT ( 'NONE',  ( 62.97617850287784336, 4.279621169095339184, -4.999999999999997335 ) ) ;
#1495=ORIENTED_EDGE ( 'NONE', *, *, #19939, .T. ) ;
#1496=CIRCLE ( 'NONE', #21248, 2.000000000000001776 ) ;
#1497=DIRECTION ( 'NONE',  ( 1.000000000000000000, 0.000000000000000000, 0.000000000000000000 ) ) ;
#1499=FACE_OUTER_BOUND ( 'NONE', #31519, .T. ) ;
#1500=VERTEX_POINT ( 'NONE', #33651 ) ;
#1501=ADVANCED_FACE ( 'NONE', ( #13578 ), #30806, .F. ) ;
#1502=DIRECTION ( 'NONE',  ( 0.8660254037844415942, 0.4999999999999949485, 0.000000000000000000 ) ) ;
#1503=ORIENTED_EDGE ( 'NONE', *, *, #8246, .T. ) ;
#1504=CARTESIAN_POINT ( 'NONE',  ( -63.00000337463102085, 60.62177826491077326, -5.000000000000000000 ) ) ;
#1506=DIRECTION ( 'NONE',  ( 0.000000000000000000, 0.000000000000000000, -1.000000000000000000 ) ) ;
#1507=ORIENTED_EDGE ( 'NONE', *, *, #7577, .F. ) ;
#1508=CIRCLE ( 'NONE', #3918, 2.000000000000001776 ) ;
#1510=CIRCLE ( 'NONE', #18899, 2.000000000000001776 ) ;
#1511=AXIS2_PLACEMENT_3D ( 'NONE', #14031, #5250, #11415 ) ;
#1514=EDGE_CURVE ( 'NONE', #5475, #15339, #27261, .T. ) ;
#1515=DIRECTION ( 'NONE',  ( 1.000000000000000000, 0.000000000000000000, 0.000000000000000000 ) ) ;
#1516=FACE_OUTER_BOUND ( 'NONE', #15122, .T. ) ;
#1517=DIRECTION ( 'NONE',  ( 0.000000000000000000, 0.000000000000000000, 1.000000000000000000 ) ) ;
#1519=EDGE_CURVE ( 'NONE', #19586, #29300, #15755, .T. ) ;
#1520=ORIENTED_EDGE ( 'NONE', *, *, #19030, .F. ) ;
#1524=DIRECTION ( 'NONE',  ( 1.000000000000000000, 0.000000000000000000, 0.000000000000000000 ) ) ;
#1525=ORIENTED_EDGE ( 'NONE', *, *, #24071, .F. ) ;
#1527=PLANE ( 'NONE',  #22645 ) ;
#1528=EDGE_CURVE ( 'NONE', #18637, #8974, #28017, .T. ) ;
#1529=CARTESIAN_POINT ( 'NONE',  ( 74.99999662536836809, -8.660254037844401509, -5.000000000000000000 ) ) ;
#1530=ORIENTED_EDGE ( 'NONE', *, *, #26753, .T. ) ;
#1532=EDGE_CURVE ( 'NONE', #203, #14513, #36712, .T. ) ;
#1533=AXIS2_PLACEMENT_3D ( 'NONE', #19025, #1573, #24260 ) ;
#1534=CARTESIAN_POINT ( 'NONE',  ( -33.21453780030408609, 78.84345928898012801, 12.50000000000000000 ) ) ;
#1535=DIRECTION ( 'NONE',  ( 0.8660254037844418162, 0.4999999999999946709, 0.000000000000000000 ) ) ;
#1536=CIRCLE ( 'NONE', #20030, 2.000000000000001776 ) ;
#1537=CARTESIAN_POINT ( 'NONE',  ( -3.374631303565411855E-06, -86.60254037844400443, -9.999999999999998224 ) ) ;
#1538=EDGE_LOOP ( 'NONE', ( #27083, #20318, #20390, #7384 ) ) ;
#1539=VERTEX_POINT ( 'NONE', #15834 ) ;
#1541=ORIENTED_EDGE ( 'NONE', *, *, #26643, .F. ) ;
#1542=AXIS2_PLACEMENT_3D ( 'NONE', #17829, #32260, #1321 ) ;
#1543=CIRCLE ( 'NONE', #22505, 2.000000000000001776 ) ;
#1544=VECTOR ( 'NONE', #1270, 1000.000000000000000 ) ;
#1545=DIRECTION ( 'NONE',  ( 0.000000000000000000, 0.000000000000000000, -1.000000000000000000 ) ) ;
#1547=ORIENTED_EDGE ( 'NONE', *, *, #35364, .T. ) ;
#1548=LINE ( 'NONE', #7553, #15964 ) ;
#1549=AXIS2_PLACEMENT_3D ( 'NONE', #1991, #5387, #13621 ) ;
#1550=ORIENTED_EDGE ( 'NONE', *, *, #8819, .T. ) ;
#1551=ORIENTED_EDGE ( 'NONE', *, *, #3941, .F. ) ;
#1552=CIRCLE ( 'NONE', #14725, 2.000000000000001776 ) ;
#1553=EDGE_CURVE ( 'NONE', #22833, #3127, #13021, .T. ) ;
#1554=DIRECTION ( 'NONE',  ( 0.000000000000000000, 0.000000000000000000, -1.000000000000000000 ) ) ;
#1555=DIRECTION ( 'NONE',  ( 0.000000000000000000, 0.000000000000000000, 1.000000000000000000 ) ) ;
#1557=ORIENTED_EDGE ( 'NONE', *, *, #9070, .F. ) ;
#1558=CYLINDRICAL_SURFACE ( 'NONE', #1759, 2.000000000000001776 ) ;
#1560=CIRCLE ( 'NONE', #34490, 33.00000000000001421 ) ;
#1561=EDGE_CURVE ( 'NONE', #14131, #20810, #27705, .T. ) ;
#1562=LINE ( 'NONE', #1014, #26450 ) ;
#1563=CARTESIAN_POINT ( 'NONE',  ( 35.19434990244975126, -52.39915983220758022, -4.999999999999997335 ) ) ;
#1564=AXIS2_PLACEMENT_3D ( 'NONE', #35486, #21209, #31310 ) ;
#1565=ORIENTED_EDGE ( 'NONE', *, *, #10566, .T. ) ;
#1566=DIRECTION ( 'NONE',  ( 1.000000000000000000, 0.000000000000000000, 0.000000000000000000 ) ) ;
#1568=ORIENTED_EDGE ( 'NONE', *, *, #6656, .T. ) ;
#1569=CARTESIAN_POINT ( 'NONE',  ( 1.999996625368665182, 69.28203230275516944, 12.50000000000000000 ) ) ;
#1571=CARTESIAN_POINT ( 'NONE',  ( 56.99999662536844625, 60.62177826491077326, -9.999999999999998224 ) ) ;
#1572=CIRCLE ( 'NONE', #34528, 2.000000000000001776 ) ;
#1573=DIRECTION ( 'NONE',  ( 0.000000000000000000, 0.000000000000000000, 1.000000000000000000 ) ) ;
#1574=AXIS2_PLACEMENT_3D ( 'NONE', #3758, #12169, #9192 ) ;
#1575=CARTESIAN_POINT ( 'NONE',  ( 57.99999662536842493, 51.96152422706639129, -9.999999999999998224 ) ) ;
#1576=AXIS2_PLACEMENT_3D ( 'NONE', #33824, #8134, #28196 ) ;
#1577=CIRCLE ( 'NONE', #9955, 2.000000000000001776 ) ;
#1580=EDGE_LOOP ( 'NONE', ( #25200, #16709 ) ) ;
#1581=DIRECTION ( 'NONE',  ( 1.000000000000000000, 0.000000000000000000, 0.000000000000000000 ) ) ;
#1582=DIRECTION ( 'NONE',  ( 1.000000000000000000, 0.000000000000000000, 0.000000000000000000 ) ) ;
#1583=FACE_OUTER_BOUND ( 'NONE', #16361, .T. ) ;
#1584=VERTEX_POINT ( 'NONE', #1949 ) ;
#1585=AXIS2_PLACEMENT_3D ( 'NONE', #25400, #37035, #11339 ) ;
#1586=ORIENTED_EDGE ( 'NONE', *, *, #29687, .F. ) ;
#1587=ORIENTED_EDGE ( 'NONE', *, *, #4704, .F. ) ;
#1588=EDGE_CURVE ( 'NONE', #27568, #6775, #22026, .T. ) ;
#1590=FACE_OUTER_BOUND ( 'NONE', #36859, .T. ) ;
#1592=AXIS2_PLACEMENT_3D ( 'NONE', #7939, #13558, #22759 ) ;
#1593=CARTESIAN_POINT ( 'NONE',  ( 76.99999662536836809, -8.660254037844401509, -9.999999999999998224 ) ) ;
#1594=VECTOR ( 'NONE', #36557, 1000.000000000000000 ) ;
#1595=DIRECTION ( 'NONE',  ( -1.000000000000000000, 0.000000000000000000, 0.000000000000000000 ) ) ;
#1596=ORIENTED_EDGE ( 'NONE', *, *, #13699, .T. ) ;
#1597=DIRECTION ( 'NONE',  ( 0.000000000000000000, 0.000000000000000000, 1.000000000000000000 ) ) ;
#1600=CARTESIAN_POINT ( 'NONE',  ( 4.999996625368676284, -77.94228634059960825, -9.999999999999998224 ) ) ;
#1602=VECTOR ( 'NONE', #7826, 1000.000000000000000 ) ;
#1603=ADVANCED_FACE ( 'NONE', ( #17489 ), #31735, .F. ) ;
#1606=LINE ( 'NONE', #24292, #33163 ) ;
#1608=EDGE_LOOP ( 'NONE', ( #5690, #20874 ) ) ;
#1610=AXIS2_PLACEMENT_3D ( 'NONE', #2864, #34538, #23465 ) ;
#1611=EDGE_CURVE ( 'NONE', #18695, #36878, #1372, .T. ) ;
#1612=CARTESIAN_POINT ( 'NONE',  ( -4.279621169095561228, 62.97617850287782915, 12.49999999999999822 ) ) ;
#1615=DIRECTION ( 'NONE',  ( 0.000000000000000000, 0.000000000000000000, 1.000000000000000000 ) ) ;
#1616=ORIENTED_EDGE ( 'NONE', *, *, #35479, .T. ) ;
#1618=EDGE_CURVE ( 'NONE', #32403, #22417, #8507, .T. ) ;
#1623=AXIS2_PLACEMENT_3D ( 'NONE', #31306, #2630, #17062 ) ;
#1625=AXIS2_PLACEMENT_3D ( 'NONE', #33468, #10027, #21825 ) ;
#1626=VERTEX_POINT ( 'NONE', #11859 ) ;
#1627=CARTESIAN_POINT ( 'NONE',  ( -65.63757354697304436, -58.72612421542294925, -5.000000000000000000 ) ) ;
#1628=LINE ( 'NONE', #1077, #31477 ) ;
#1629=EDGE_CURVE ( 'NONE', #17931, #34610, #34305, .T. ) ;
#1632=EDGE_CURVE ( 'NONE', #26415, #8015, #1965, .T. ) ;
#1633=DIRECTION ( 'NONE',  ( -0.000000000000000000, -0.000000000000000000, 1.000000000000000000 ) ) ;
#1634=AXIS2_PLACEMENT_3D ( 'NONE', #15649, #9822, #29692 ) ;
#1635=ORIENTED_EDGE ( 'NONE', *, *, #29591, .F. ) ;
#1637=CARTESIAN_POINT ( 'NONE',  ( 89.42901512340354486, -31.83425564451495404, -5.000000000000011546 ) ) ;
#1638=DIRECTION ( 'NONE',  ( 0.000000000000000000, 0.000000000000000000, 1.000000000000000000 ) ) ;
#1639=EDGE_CURVE ( 'NONE', #33094, #3043, #8408, .T. ) ;
#1640=DIRECTION ( 'NONE',  ( 0.000000000000000000, 0.000000000000000000, 1.000000000000000000 ) ) ;
#1642=DIRECTION ( 'NONE',  ( -1.000000000000000000, 0.000000000000000000, 0.000000000000000000 ) ) ;
#1644=CIRCLE ( 'NONE', #32165, 2.000000000000001776 ) ;
#1645=ORIENTED_EDGE ( 'NONE', *, *, #24791, .T. ) ;
#1646=CARTESIAN_POINT ( 'NONE',  ( -3.374631334790434423E-06, 69.28203230275516944, 17.49999999999999645 ) ) ;
#1647=AXIS2_PLACEMENT_3D ( 'NONE', #239, #23496, #11502 ) ;
#1648=DIRECTION ( 'NONE',  ( 1.000000000000000000, 0.000000000000000000, 0.000000000000000000 ) ) ;
#1649=EDGE_LOOP ( 'NONE', ( #22777, #456 ) ) ;
#1653=CARTESIAN_POINT ( 'NONE',  ( -87.00000337463093558, -25.98076211353322051, -9.999999999999998224 ) ) ;
#1655=AXIS2_PLACEMENT_3D ( 'NONE', #22166, #9973, #21972 ) ;
#1658=DIRECTION ( 'NONE',  ( 0.000000000000000000, 0.000000000000000000, 1.000000000000000000 ) ) ;
#1659=VERTEX_POINT ( 'NONE', #19776 ) ;
#1662=AXIS2_PLACEMENT_3D ( 'NONE', #10916, #2869, #19363 ) ;
#1663=DIRECTION ( 'NONE',  ( 1.000000000000000000, 0.000000000000000000, 0.000000000000000000 ) ) ;
#1664=DIRECTION ( 'NONE',  ( 0.000000000000000000, 0.000000000000000000, 1.000000000000000000 ) ) ;
#1665=ORIENTED_EDGE ( 'NONE', *, *, #11193, .F. ) ;
#1666=DIRECTION ( 'NONE',  ( 1.000000000000000000, 0.000000000000000000, 0.000000000000000000 ) ) ;
#1668=CIRCLE ( 'NONE', #11246, 2.000000000000001776 ) ;
#1669=CARTESIAN_POINT ( 'NONE',  ( 7.999996625368656744, -86.60254037844400443, -9.999999999999998224 ) ) ;
#1670=VERTEX_POINT ( 'NONE', #11496 ) ;
#1671=ORIENTED_EDGE ( 'NONE', *, *, #5157, .F. ) ;
#1672=ORIENTED_EDGE ( 'NONE', *, *, #4969, .F. ) ;
#1675=DIRECTION ( 'NONE',  ( 0.000000000000000000, 0.000000000000000000, 1.000000000000000000 ) ) ;
#1676=ORIENTED_EDGE ( 'NONE', *, *, #34306, .F. ) ;
#1678=AXIS2_PLACEMENT_3D ( 'NONE', #15413, #32459, #12757 ) ;
#1680=DIRECTION ( 'NONE',  ( 0.000000000000000000, 0.000000000000000000, 1.000000000000000000 ) ) ;
#1681=DIRECTION ( 'NONE',  ( 1.000000000000000000, 0.000000000000000000, 0.000000000000000000 ) ) ;
#1682=AXIS2_PLACEMENT_3D ( 'NONE', #32550, #32944, #19074 ) ;
#1683=EDGE_CURVE ( 'NONE', #28818, #26555, #34167, .T. ) ;
#1684=FACE_OUTER_BOUND ( 'NONE', #25442, .T. ) ;
#1685=AXIS2_PLACEMENT_3D ( 'NONE', #746, #20437, #6574 ) ;
#1686=ADVANCED_FACE ( 'NONE', ( #13938 ), #31198, .F. ) ;
#1687=ADVANCED_FACE ( 'NONE', ( #14121 ), #16779, .T. ) ;
#1688=DIRECTION ( 'NONE',  ( -0.000000000000000000, -0.000000000000000000, 1.000000000000000000 ) ) ;
#1689=FACE_OUTER_BOUND ( 'NONE', #12212, .T. ) ;
#1691=DIRECTION ( 'NONE',  ( -1.000000000000000000, 0.000000000000000000, -0.000000000000000000 ) ) ;
#1693=EDGE_LOOP ( 'NONE', ( #15183, #32670 ) ) ;
#1694=CIRCLE ( 'NONE', #8856, 33.00000000000001421 ) ;
#1695=DIRECTION ( 'NONE',  ( 0.5000000000000038858, 0.8660254037844363761, 0.000000000000000000 ) ) ;
#1696=DIRECTION ( 'NONE',  ( 0.000000000000000000, 0.000000000000000000, -1.000000000000000000 ) ) ;
#1697=DIRECTION ( 'NONE',  ( 0.000000000000000000, 0.000000000000000000, 1.000000000000000000 ) ) ;
#1698=CARTESIAN_POINT ( 'NONE',  ( -78.00000337463094979, 34.64101615137757051, 12.50000000000000000 ) ) ;
#1699=ORIENTED_EDGE ( 'NONE', *, *, #20552, .T. ) ;
#1700=CIRCLE ( 'NONE', #22657, 3.000000000000003997 ) ;
#1702=DIRECTION ( 'NONE',  ( 0.000000000000000000, 0.000000000000000000, 1.000000000000000000 ) ) ;
#1704=AXIS2_PLACEMENT_3D ( 'NONE', #36443, #2108, #22189 ) ;
#1705=ORIENTED_EDGE ( 'NONE', *, *, #11357, .F. ) ;
#1708=ORIENTED_EDGE ( 'NONE', *, *, #31388, .F. ) ;
#1709=EDGE_CURVE ( 'NONE', #6799, #27465, #31362, .T. ) ;
#1710=AXIS2_PLACEMENT_3D ( 'NONE', #11524, #12065, #25969 ) ;
#1711=CARTESIAN_POINT ( 'NONE',  ( -65.00000337463104927, -43.30127018922202353, 12.50000000000000000 ) ) ;
#1713=CIRCLE ( 'NONE', #31355, 2.000000000000000000 ) ;
#1714=CARTESIAN_POINT ( 'NONE',  ( -42.00000337463114164, -69.28203230275519786, -9.999999999999998224 ) ) ;
#1715=EDGE_LOOP ( 'NONE', ( #15994, #30159, #25758, #23139 ) ) ;
#1716=ORIENTED_EDGE ( 'NONE', *, *, #3941, .T. ) ;
#1717=VECTOR ( 'NONE', #5646, 1000.000000000000000 ) ;
#1718=CYLINDRICAL_SURFACE ( 'NONE', #25165, 2.000000000000001776 ) ;
#1719=CIRCLE ( 'NONE', #23887, 2.000000000000001776 ) ;
#1720=ORIENTED_EDGE ( 'NONE', *, *, #15375, .T. ) ;
#1721=CARTESIAN_POINT ( 'NONE',  ( -3.374631303565411855E-06, -86.60254037844400443, -9.999999999999998224 ) ) ;
#1722=FACE_BOUND ( 'NONE', #31894, .T. ) ;
#1723=DIRECTION ( 'NONE',  ( 0.000000000000000000, 0.000000000000000000, 1.000000000000000000 ) ) ;
#1724=CARTESIAN_POINT ( 'NONE',  ( 84.99999662536832545, 8.660254037844394404, 17.49999999999999645 ) ) ;
#1725=DIRECTION ( 'NONE',  ( 1.000000000000000000, 0.000000000000000000, 0.000000000000000000 ) ) ;
#1726=ORIENTED_EDGE ( 'NONE', *, *, #4042, .F. ) ;
#1728=CARTESIAN_POINT ( 'NONE',  ( 69.99999662536839651, -17.32050807568879947, 12.50000000000000000 ) ) ;
#1729=EDGE_CURVE ( 'NONE', #1410, #9726, #21578, .T. ) ;
#1730=SURFACE_STYLE_USAGE ( .BOTH. , #15979 ) ;
#1731=ORIENTED_EDGE ( 'NONE', *, *, #30960, .T. ) ;
#1732=CYLINDRICAL_SURFACE ( 'NONE', #20808, 2.000000000000001776 ) ;
#1733=AXIS2_PLACEMENT_3D ( 'NONE', #24641, #18643, #30236 ) ;
#1734=CARTESIAN_POINT ( 'NONE',  ( -14.80603122773057478, 87.83969979969877784, 12.49999999999999645 ) ) ;
#1735=ORIENTED_EDGE ( 'NONE', *, *, #31425, .F. ) ;
#1736=ORIENTED_EDGE ( 'NONE', *, *, #27714, .T. ) ;
#1737=FACE_OUTER_BOUND ( 'NONE', #10885, .T. ) ;
#1738=DIRECTION ( 'NONE',  ( 0.000000000000000000, 0.000000000000000000, 1.000000000000000000 ) ) ;
#1740=ORIENTED_EDGE ( 'NONE', *, *, #24255, .T. ) ;
#1741=ORIENTED_EDGE ( 'NONE', *, *, #33937, .F. ) ;
#1742=ORIENTED_EDGE ( 'NONE', *, *, #2060, .T. ) ;
#1743=CARTESIAN_POINT ( 'NONE',  ( 74.99999662536836809, 8.660254037844394404, 17.49999999999999645 ) ) ;
#1744=AXIS2_PLACEMENT_3D ( 'NONE', #22096, #25105, #7848 ) ;
#1745=ORIENTED_EDGE ( 'NONE', *, *, #4190, .T. ) ;
#1746=EDGE_CURVE ( 'NONE', #22366, #13981, #15602, .T. ) ;
#1747=AXIS2_PLACEMENT_3D ( 'NONE', #10474, #33910, #8230 ) ;
#1748=DIRECTION ( 'NONE',  ( -0.000000000000000000, -0.000000000000000000, 1.000000000000000000 ) ) ;
#1751=ORIENTED_EDGE ( 'NONE', *, *, #1412, .F. ) ;
#1752=DIRECTION ( 'NONE',  ( 0.8660254037844344888, -0.5000000000000071054, 0.000000000000000000 ) ) ;
#1753=AXIS2_PLACEMENT_3D ( 'NONE', #4859, #27890, #2214 ) ;
#1754=CARTESIAN_POINT ( 'NONE',  ( -32.00000337463118427, 69.28203230275516944, -9.999999999999998224 ) ) ;
#1755=VERTEX_POINT ( 'NONE', #34763 ) ;
#1756=ADVANCED_FACE ( 'NONE', ( #31013 ), #5349, .F. ) ;
#1757=VERTEX_POINT ( 'NONE', #29099 ) ;
#1758=CARTESIAN_POINT ( 'NONE',  ( 24.99999662536857059, 77.94228634059957983, -9.999999999999998224 ) ) ;
#1759=AXIS2_PLACEMENT_3D ( 'NONE', #27439, #21803, #33242 ) ;
#1761=CARTESIAN_POINT ( 'NONE',  ( -48.00000337463109190, 69.28203230275518365, -9.999999999999998224 ) ) ;
#1762=DIRECTION ( 'NONE',  ( 1.000000000000000000, 0.000000000000000000, 0.000000000000000000 ) ) ;
#1763=ADVANCED_FACE ( 'NONE', ( #15051 ), #6979, .F. ) ;
#1764=VERTEX_POINT ( 'NONE', #29856 ) ;
#1765=CARTESIAN_POINT ( 'NONE',  ( 26.99999662536856704, 77.94228634059957983, 12.50000000000000000 ) ) ;
#1766=CIRCLE ( 'NONE', #27510, 2.000000000000001776 ) ;
#1769=DIRECTION ( 'NONE',  ( 0.000000000000000000, 0.000000000000000000, 1.000000000000000000 ) ) ;
#1770=FACE_BOUND ( 'NONE', #14736, .T. ) ;
#1772=VECTOR ( 'NONE', #14188, 1000.000000000000000 ) ;
#1773=CARTESIAN_POINT ( 'NONE',  ( 62.99999662536839651, 60.62177826491078747, -9.999999999999998224 ) ) ;
#1774=AXIS2_PLACEMENT_3D ( 'NONE', #3510, #28973, #6503 ) ;
#1775=CARTESIAN_POINT ( 'NONE',  ( 77.99999662536832545, -34.64101615137759183, -9.999999999999998224 ) ) ;
#1776=EDGE_CURVE ( 'NONE', #36972, #30139, #36572, .T. ) ;
#1778=ORIENTED_EDGE ( 'NONE', *, *, #9161, .F. ) ;
#1779=LINE ( 'NONE', #24835, #26780 ) ;
#1780=LINE ( 'NONE', #21267, #16549 ) ;
#1781=DIRECTION ( 'NONE',  ( -0.000000000000000000, -0.000000000000000000, 1.000000000000000000 ) ) ;
#1782=EDGE_LOOP ( 'NONE', ( #26880, #23235, #33783, #15243, #18109 ) ) ;
#1785=CIRCLE ( 'NONE', #17947, 33.00000000000001421 ) ;
#1788=CIRCLE ( 'NONE', #22754, 3.000000000000002665 ) ;
#1790=EDGE_CURVE ( 'NONE', #17529, #13754, #14396, .T. ) ;
#1791=DIRECTION ( 'NONE',  ( 0.000000000000000000, 0.000000000000000000, -1.000000000000000000 ) ) ;
#1792=CARTESIAN_POINT ( 'NONE',  ( -10.00000337463125000, -86.60254037844400443, 12.50000000000000000 ) ) ;
#1794=EDGE_CURVE ( 'NONE', #2651, #8103, #20385, .T. ) ;
#1795=DIRECTION ( 'NONE',  ( 0.000000000000000000, 0.000000000000000000, 1.000000000000000000 ) ) ;
#1796=EDGE_LOOP ( 'NONE', ( #35672, #5088 ) ) ;
#1797=DIRECTION ( 'NONE',  ( 0.000000000000000000, 0.000000000000000000, 1.000000000000000000 ) ) ;
#1798=AXIS2_PLACEMENT_3D ( 'NONE', #12044, #3087, #23504 ) ;
#1799=CARTESIAN_POINT ( 'NONE',  ( 52.99999662536844625, -60.62177826491080168, -9.999999999999998224 ) ) ;
#1800=FACE_OUTER_BOUND ( 'NONE', #612, .T. ) ;
#1802=VECTOR ( 'NONE', #24216, 1000.000000000000000 ) ;
#1804=ORIENTED_EDGE ( 'NONE', *, *, #487, .T. ) ;
#1806=AXIS2_PLACEMENT_3D ( 'NONE', #8453, #14806, #25710 ) ;
#1808=DIRECTION ( 'NONE',  ( 0.000000000000000000, 0.000000000000000000, -1.000000000000000000 ) ) ;
#1812=ORIENTED_EDGE ( 'NONE', *, *, #16207, .T. ) ;
#1813=DIRECTION ( 'NONE',  ( -0.4999999999999980016, 0.8660254037844398178, 0.000000000000000000 ) ) ;
#1815=EDGE_LOOP ( 'NONE', ( #19953, #7949 ) ) ;
#1816=CARTESIAN_POINT ( 'NONE',  ( 34.99999662536855283, 60.62177826491078747, -9.999999999999998224 ) ) ;
#1818=CARTESIAN_POINT ( 'NONE',  ( 24.99999662536857059, 77.94228634059957983, -9.999999999999998224 ) ) ;
#1819=VERTEX_POINT ( 'NONE', #26310 ) ;
#1821=AXIS2_PLACEMENT_3D ( 'NONE', #788, #12032, #17866 ) ;
#1822=DIRECTION ( 'NONE',  ( 0.000000000000000000, 0.000000000000000000, 1.000000000000000000 ) ) ;
#1823=CARTESIAN_POINT ( 'NONE',  ( 59.99999662536842493, 51.96152422706639129, -9.999999999999998224 ) ) ;
#1824=DIRECTION ( 'NONE',  ( 1.000000000000000000, 0.000000000000000000, 0.000000000000000000 ) ) ;
#1825=EDGE_CURVE ( 'NONE', #6458, #10369, #18046, .T. ) ;
#1826=ORIENTED_EDGE ( 'NONE', *, *, #3894, .T. ) ;
#1828=FACE_OUTER_BOUND ( 'NONE', #3973, .T. ) ;
#1829=CARTESIAN_POINT ( 'NONE',  ( 11.99999662536865763, -86.60254037844400443, -9.999999999999998224 ) ) ;
#1832=EDGE_LOOP ( 'NONE', ( #22224, #2825 ) ) ;
#1833=EDGE_CURVE ( 'NONE', #34764, #68, #34928, .T. ) ;
#1834=EDGE_LOOP ( 'NONE', ( #17146, #25800, #28090, #24674 ) ) ;
#1835=DIRECTION ( 'NONE',  ( 1.000000000000000000, 0.000000000000000000, 0.000000000000000000 ) ) ;
#1836=FACE_OUTER_BOUND ( 'NONE', #32214, .T. ) ;
#1837=ORIENTED_EDGE ( 'NONE', *, *, #25740, .T. ) ;
#1838=ADVANCED_FACE ( 'NONE', ( #6231 ), #35497, .F. ) ;
#1839=CARTESIAN_POINT ( 'NONE',  ( 65.63757102168601421, 58.72612563608866765, -5.000000000000000000 ) ) ;
#1841=ORIENTED_EDGE ( 'NONE', *, *, #25449, .F. ) ;
#1842=CARTESIAN_POINT ( 'NONE',  ( 17.99999662536858125, 86.60254037844397601, 12.50000000000000000 ) ) ;
#1843=DIRECTION ( 'NONE',  ( 1.000000000000000000, 0.000000000000000000, 0.000000000000000000 ) ) ;
#1844=EDGE_LOOP ( 'NONE', ( #2809, #20964 ) ) ;
#1845=CARTESIAN_POINT ( 'NONE',  ( 32.99999662536855283, -60.62177826491080168, -5.000000000000000000 ) ) ;
#1846=ORIENTED_EDGE ( 'NONE', *, *, #30808, .F. ) ;
#1847=CARTESIAN_POINT ( 'NONE',  ( 67.99999662536838230, -17.32050807568879947, 17.49999999999999645 ) ) ;
#1848=EDGE_CURVE ( 'NONE', #9530, #25810, #9620, .T. ) ;
#1849=CARTESIAN_POINT ( 'NONE',  ( 62.99999662536839651, -43.30127018922199511, 17.49999999999999645 ) ) ;
#1850=DIRECTION ( 'NONE',  ( 1.000000000000000000, 0.000000000000000000, 0.000000000000000000 ) ) ;
#1851=AXIS2_PLACEMENT_3D ( 'NONE', #19848, #31269, #22848 ) ;
#1852=ORIENTED_EDGE ( 'NONE', *, *, #31081, .T. ) ;
#1853=DIRECTION ( 'NONE',  ( 0.000000000000000000, 0.000000000000000000, 1.000000000000000000 ) ) ;
#1855=DIRECTION ( 'NONE',  ( 0.000000000000000000, 0.000000000000000000, 1.000000000000000000 ) ) ;
#1856=CARTESIAN_POINT ( 'NONE',  ( -85.00000337463092137, 8.660254037844389075, -5.000000000000000000 ) ) ;
#1857=VERTEX_POINT ( 'NONE', #12403 ) ;
#1858=ORIENTED_EDGE ( 'NONE', *, *, #25066, .F. ) ;
#1859=ORIENTED_EDGE ( 'NONE', *, *, #14978, .F. ) ;
#1860=DIRECTION ( 'NONE',  ( 1.000000000000000000, 0.000000000000000000, 0.000000000000000000 ) ) ;
#1861=VERTEX_POINT ( 'NONE', #20657 ) ;
#1863=CARTESIAN_POINT ( 'NONE',  ( -3.374631327851540519E-06, 86.60254037844397601, 12.50000000000000000 ) ) ;
#1865=EDGE_CURVE ( 'NONE', #33610, #4180, #32091, .T. ) ;
#1866=CARTESIAN_POINT ( 'NONE',  ( -65.00000337463102085, 60.62177826491077326, -5.000000000000000000 ) ) ;
#1867=FACE_OUTER_BOUND ( 'NONE', #31906, .T. ) ;
#1869=EDGE_CURVE ( 'NONE', #14564, #13541, #16791, .T. ) ;
#1873=EDGE_CURVE ( 'NONE', #17871, #18749, #33578, .T. ) ;
#1875=DIRECTION ( 'NONE',  ( 0.000000000000000000, 0.000000000000000000, 1.000000000000000000 ) ) ;
#1876=CARTESIAN_POINT ( 'NONE',  ( -70.00000337463099243, 51.96152422706637708, 12.50000000000000000 ) ) ;
#1877=DIRECTION ( 'NONE',  ( 1.000000000000000000, 0.000000000000000000, 0.000000000000000000 ) ) ;
#1878=CARTESIAN_POINT ( 'NONE',  ( -67.00000337463106348, -60.62177826491083010, -5.000000000000000000 ) ) ;
#1879=EDGE_CURVE ( 'NONE', #29900, #36497, #18429, .T. ) ;
#1881=EDGE_CURVE ( 'NONE', #2266, #18182, #29650, .T. ) ;
#1882=CARTESIAN_POINT ( 'NONE',  ( -20.00000337463122690, 86.60254037844397601, -5.000000000000000000 ) ) ;
#1884=EDGE_LOOP ( 'NONE', ( #8577, #25517, #19032, #6250 ) ) ;
#1885=FACE_OUTER_BOUND ( 'NONE', #26315, .T. ) ;
#1886=ORIENTED_EDGE ( 'NONE', *, *, #1790, .F. ) ;
#1887=EDGE_CURVE ( 'NONE', #36225, #13221, #24051, .T. ) ;
#1889=DIRECTION ( 'NONE',  ( -1.051347561198064495E-14, -1.000000000000000000, 0.000000000000000000 ) ) ;
#1891=LINE ( 'NONE', #13317, #14018 ) ;
#1892=EDGE_CURVE ( 'NONE', #20137, #32311, #13852, .T. ) ;
#1893=AXIS2_PLACEMENT_3D ( 'NONE', #34009, #27796, #1934 ) ;
#1894=LINE ( 'NONE', #1714, #7701 ) ;
#1895=ADVANCED_FACE ( 'NONE', ( #7875 ), #13471, .F. ) ;
#1896=EDGE_LOOP ( 'NONE', ( #31675, #26615, #30467, #15596, #25576, #31376 ) ) ;
#1897=EDGE_LOOP ( 'NONE', ( #34890, #7758 ) ) ;
#1898=AXIS2_PLACEMENT_3D ( 'NONE', #15578, #12732, #35077 ) ;
#1899=CARTESIAN_POINT ( 'NONE',  ( -70.00000337463100664, -17.32050807568882078, -9.999999999999998224 ) ) ;
#1900=ORIENTED_EDGE ( 'NONE', *, *, #22499, .F. ) ;
#1902=CYLINDRICAL_SURFACE ( 'NONE', #14361, 33.00000000000001421 ) ;
#1903=CARTESIAN_POINT ( 'NONE',  ( -7.000003374631307729, 77.94228634059957983, -9.999999999999998224 ) ) ;
#1905=CARTESIAN_POINT ( 'NONE',  ( -29.97040610772328861, 71.28181329121154874, -5.000000000000000000 ) ) ;
#1906=ORIENTED_EDGE ( 'NONE', *, *, #11864, .T. ) ;
#1910=ORIENTED_EDGE ( 'NONE', *, *, #925, .T. ) ;
#1912=CARTESIAN_POINT ( 'NONE',  ( -5.000003374631269537, -77.94228634059960825, -9.999999999999998224 ) ) ;
#1913=EDGE_CURVE ( 'NONE', #33336, #3159, #606, .T. ) ;
#1914=ORIENTED_EDGE ( 'NONE', *, *, #21623, .F. ) ;
#1915=ORIENTED_EDGE ( 'NONE', *, *, #4297, .T. ) ;
#1919=VERTEX_POINT ( 'NONE', #33740 ) ;
#1921=EDGE_LOOP ( 'NONE', ( #6368, #1910 ) ) ;
#1922=DIRECTION ( 'NONE',  ( 0.000000000000000000, 0.000000000000000000, -1.000000000000000000 ) ) ;
#1923=ORIENTED_EDGE ( 'NONE', *, *, #30008, .F. ) ;
#1926=VERTEX_POINT ( 'NONE', #24935 ) ;
#1927=CARTESIAN_POINT ( 'NONE',  ( -85.00000337463092137, 8.660254037844389075, -9.999999999999998224 ) ) ;
#1930=ORIENTED_EDGE ( 'NONE', *, *, #25063, .F. ) ;
#1931=ORIENTED_EDGE ( 'NONE', *, *, #19432, .F. ) ;
#1933=CARTESIAN_POINT ( 'NONE',  ( -8.000003374631281972, 86.60254037844397601, -9.999999999999998224 ) ) ;
#1934=DIRECTION ( 'NONE',  ( 1.000000000000000000, 0.000000000000000000, 0.000000000000000000 ) ) ;
#1935=LINE ( 'NONE', #21637, #12460 ) ;
#1936=ORIENTED_EDGE ( 'NONE', *, *, #27644, .F. ) ;
#1937=DIRECTION ( 'NONE',  ( 0.000000000000000000, 0.000000000000000000, 1.000000000000000000 ) ) ;
#1938=AXIS2_PLACEMENT_3D ( 'NONE', #13117, #19130, #30160 ) ;
#1939=FACE_BOUND ( 'NONE', #20725, .T. ) ;
#1940=DIRECTION ( 'NONE',  ( 1.000000000000000000, 0.000000000000000000, 0.000000000000000000 ) ) ;
#1941=CARTESIAN_POINT ( 'NONE',  ( -43.19957991610399972, -47.04203867989563292, 12.49999999999999822 ) ) ;
#1942=DIRECTION ( 'NONE',  ( -0.000000000000000000, -0.000000000000000000, 1.000000000000000000 ) ) ;
#1943=DIRECTION ( 'NONE',  ( 0.000000000000000000, 0.000000000000000000, 1.000000000000000000 ) ) ;
#1947=LINE ( 'NONE', #30460, #25008 ) ;
#1948=PLANE ( 'NONE',  #15930 ) ;
#1949=CARTESIAN_POINT ( 'NONE',  ( -78.00000337463096400, -34.64101615137762025, -9.999999999999998224 ) ) ;
#1951=EDGE_CURVE ( 'NONE', #1659, #19499, #14122, .T. ) ;
#1953=AXIS2_PLACEMENT_3D ( 'NONE', #1354, #33045, #1184 ) ;
#1954=ORIENTED_EDGE ( 'NONE', *, *, #10337, .T. ) ;
#1955=VERTEX_POINT ( 'NONE', #11031 ) ;
#1956=DIRECTION ( 'NONE',  ( 0.000000000000000000, 0.000000000000000000, 1.000000000000000000 ) ) ;
#1958=ADVANCED_FACE ( 'NONE', ( #10682 ), #30722, .F. ) ;
#1960=CARTESIAN_POINT ( 'NONE',  ( 67.99999662536839651, 51.96152422706640550, 12.50000000000000000 ) ) ;
#1964=ORIENTED_EDGE ( 'NONE', *, *, #11063, .T. ) ;
#1965=CIRCLE ( 'NONE', #30706, 2.000000000000001776 ) ;
#1966=CYLINDRICAL_SURFACE ( 'NONE', #19181, 2.000000000000001776 ) ;
#1967=EDGE_LOOP ( 'NONE', ( #24734, #28848 ) ) ;
#1968=DIRECTION ( 'NONE',  ( 0.000000000000000000, 0.000000000000000000, 1.000000000000000000 ) ) ;
#1969=DIRECTION ( 'NONE',  ( 1.000000000000000000, 0.000000000000000000, 0.000000000000000000 ) ) ;
#1971=CARTESIAN_POINT ( 'NONE',  ( -95.00000000000000000, 0.000000000000000000, 12.49999999999999822 ) ) ;
#1976=CYLINDRICAL_SURFACE ( 'NONE', #2114, 2.000000000000001776 ) ;
#1977=LINE ( 'NONE', #2167, #12153 ) ;
#1978=AXIS2_PLACEMENT_3D ( 'NONE', #31503, #11620, #5845 ) ;
#1979=ORIENTED_EDGE ( 'NONE', *, *, #12058, .F. ) ;
#1980=LINE ( 'NONE', #13054, #7198 ) ;
#1981=DIRECTION ( 'NONE',  ( 0.000000000000000000, 0.000000000000000000, 1.000000000000000000 ) ) ;
#1982=ORIENTED_EDGE ( 'NONE', *, *, #20359, .F. ) ;
#1984=PLANE ( 'NONE',  #28039 ) ;
#1985=CARTESIAN_POINT ( 'NONE',  ( -27.00000337463120914, 77.94228634059957983, -9.999999999999998224 ) ) ;
#1986=EDGE_LOOP ( 'NONE', ( #6166, #34350 ) ) ;
#1987=AXIS2_PLACEMENT_3D ( 'NONE', #4028, #35719, #9658 ) ;
#1988=EDGE_CURVE ( 'NONE', #32887, #4892, #14714, .T. ) ;
#1989=ORIENTED_EDGE ( 'NONE', *, *, #35364, .F. ) ;
#1990=DIRECTION ( 'NONE',  ( -1.000000000000000000, 0.000000000000000000, -0.000000000000000000 ) ) ;
#1991=CARTESIAN_POINT ( 'NONE',  ( -75.00000337463100664, -43.30127018922202353, 17.49999999999999645 ) ) ;
#1993=EDGE_LOOP ( 'NONE', ( #30566, #3036, #34482, #12581 ) ) ;
#1994=EDGE_LOOP ( 'NONE', ( #28535, #32707 ) ) ;
#1996=DIRECTION ( 'NONE',  ( -1.000000000000000000, 0.000000000000000000, 0.000000000000000000 ) ) ;
#2000=AXIS2_PLACEMENT_3D ( 'NONE', #11669, #31369, #22945 ) ;
#2001=DIRECTION ( 'NONE',  ( 0.000000000000000000, 0.000000000000000000, 1.000000000000000000 ) ) ;
#2002=VERTEX_POINT ( 'NONE', #23408 ) ;
#2004=AXIS2_PLACEMENT_3D ( 'NONE', #18333, #33131, #12878 ) ;
#2005=DIRECTION ( 'NONE',  ( -1.000000000000000000, 0.000000000000000000, 0.000000000000000000 ) ) ;
#2007=DIRECTION ( 'NONE',  ( 1.000000000000000000, 0.000000000000000000, 0.000000000000000000 ) ) ;
#2008=ORIENTED_EDGE ( 'NONE', *, *, #30972, .F. ) ;
#2010=EDGE_LOOP ( 'NONE', ( #24036, #35965 ) ) ;
#2012=AXIS2_PLACEMENT_3D ( 'NONE', #30484, #2659, #25747 ) ;
#2014=DIRECTION ( 'NONE',  ( 1.000000000000000000, 0.000000000000000000, 0.000000000000000000 ) ) ;
#2015=ORIENTED_EDGE ( 'NONE', *, *, #33020, .T. ) ;
#2016=AXIS2_PLACEMENT_3D ( 'NONE', #14169, #25627, #34622 ) ;
#2019=EDGE_CURVE ( 'NONE', #12329, #33284, #26215, .T. ) ;
#2020=CARTESIAN_POINT ( 'NONE',  ( -52.39915983220772233, -35.19434990244957362, -4.999999999999997335 ) ) ;
#2022=EDGE_LOOP ( 'NONE', ( #21195, #20127, #11544, #36205 ) ) ;
#2023=DIRECTION ( 'NONE',  ( 0.000000000000000000, 0.000000000000000000, -1.000000000000000000 ) ) ;
#2024=DIRECTION ( 'NONE',  ( 0.000000000000000000, 0.000000000000000000, 1.000000000000000000 ) ) ;
#2026=VERTEX_POINT ( 'NONE', #15136 ) ;
#2027=EDGE_CURVE ( 'NONE', #25889, #26458, #28653, .T. ) ;
#2028=VERTEX_POINT ( 'NONE', #11954 ) ;
#2029=CIRCLE ( 'NONE', #11590, 2.000000000000001776 ) ;
#2032=DIRECTION ( 'NONE',  ( 1.000000000000000000, 0.000000000000000000, 0.000000000000000000 ) ) ;
#2035=CARTESIAN_POINT ( 'NONE',  ( 51.99999662536847467, -69.28203230275519786, -9.999999999999998224 ) ) ;
#2036=CYLINDRICAL_SURFACE ( 'NONE', #2448, 2.000000000000001776 ) ;
#2037=AXIS2_PLACEMENT_3D ( 'NONE', #21970, #35864, #33606 ) ;
#2038=CARTESIAN_POINT ( 'NONE',  ( -35.00000337463116296, 60.62177826491077326, -9.999999999999998224 ) ) ;
#2039=LINE ( 'NONE', #15744, #1116 ) ;
#2041=DIRECTION ( 'NONE',  ( 0.000000000000000000, 0.000000000000000000, 1.000000000000000000 ) ) ;
#2042=DIRECTION ( 'NONE',  ( 0.000000000000000000, 0.000000000000000000, 1.000000000000000000 ) ) ;
#2043=ORIENTED_EDGE ( 'NONE', *, *, #25784, .F. ) ;
#2044=ORIENTED_EDGE ( 'NONE', *, *, #19742, .F. ) ;
#2045=EDGE_CURVE ( 'NONE', #9593, #30829, #2134, .T. ) ;
#2046=CARTESIAN_POINT ( 'NONE',  ( 71.99999662536838230, -34.64101615137759183, -9.999999999999998224 ) ) ;
#2047=CARTESIAN_POINT ( 'NONE',  ( -35.00000337463116296, 77.94228634059957983, -9.999999999999998224 ) ) ;
#2048=CARTESIAN_POINT ( 'NONE',  ( 44.99999662536849598, -77.94228634059960825, 17.49999999999999645 ) ) ;
#2050=DIRECTION ( 'NONE',  ( 0.000000000000000000, 0.000000000000000000, 1.000000000000000000 ) ) ;
#2052=DIRECTION ( 'NONE',  ( 1.000000000000000000, 0.000000000000000000, 0.000000000000000000 ) ) ;
#2053=VERTEX_POINT ( 'NONE', #29200 ) ;
#2054=DIRECTION ( 'NONE',  ( 0.000000000000000000, 0.000000000000000000, 1.000000000000000000 ) ) ;
#2055=VERTEX_POINT ( 'NONE', #26402 ) ;
#2056=DIRECTION ( 'NONE',  ( 1.000000000000000000, 0.000000000000000000, 0.000000000000000000 ) ) ;
#2057=AXIS2_PLACEMENT_3D ( 'NONE', #4110, #12703, #4471 ) ;
#2058=AXIS2_PLACEMENT_3D ( 'NONE', #23236, #20239, #31827 ) ;
#2059=CARTESIAN_POINT ( 'NONE',  ( 72.99999662536835388, -43.30127018922199511, -5.000000000000000000 ) ) ;
#2060=EDGE_CURVE ( 'NONE', #30710, #7161, #18298, .T. ) ;
#2061=AXIS2_PLACEMENT_3D ( 'NONE', #29994, #36007, #10300 ) ;
#2062=DIRECTION ( 'NONE',  ( 0.000000000000000000, 0.000000000000000000, -1.000000000000000000 ) ) ;
#2063=ORIENTED_EDGE ( 'NONE', *, *, #18585, .F. ) ;
#2064=EDGE_CURVE ( 'NONE', #20328, #26329, #9919, .T. ) ;
#2065=ORIENTED_EDGE ( 'NONE', *, *, #4297, .F. ) ;
#2066=ADVANCED_FACE ( 'NONE', ( #20396 ), #20024, .T. ) ;
#2067=EDGE_LOOP ( 'NONE', ( #25119, #14983, #24161 ) ) ;
#2068=AXIS2_PLACEMENT_3D ( 'NONE', #32426, #29601, #1681 ) ;
#2069=DIRECTION ( 'NONE',  ( 1.000000000000000000, 0.000000000000000000, 0.000000000000000000 ) ) ;
#2071=AXIS2_PLACEMENT_3D ( 'NONE', #35052, #22883, #6173 ) ;
#2072=EDGE_CURVE ( 'NONE', #23588, #15633, #12303, .T. ) ;
#2073=CARTESIAN_POINT ( 'NONE',  ( -10.00000337463125000, -86.60254037844400443, -9.999999999999998224 ) ) ;
#2075=FACE_OUTER_BOUND ( 'NONE', #18889, .T. ) ;
#2076=ADVANCED_FACE ( 'NONE', ( #17574 ), #5793, .F. ) ;
#2077=ORIENTED_EDGE ( 'NONE', *, *, #14938, .T. ) ;
#2078=DIRECTION ( 'NONE',  ( 1.000000000000000000, 0.000000000000000000, 0.000000000000000000 ) ) ;
#2079=CIRCLE ( 'NONE', #21836, 2.000000000000001776 ) ;
#2080=FACE_OUTER_BOUND ( 'NONE', #27709, .T. ) ;
#2081=DIRECTION ( 'NONE',  ( 0.000000000000000000, 0.000000000000000000, 1.000000000000000000 ) ) ;
#2082=ORIENTED_EDGE ( 'NONE', *, *, #25421, .T. ) ;
#2083=LINE ( 'NONE', #27414, #13053 ) ;
#2084=DIRECTION ( 'NONE',  ( -0.000000000000000000, -0.000000000000000000, 1.000000000000000000 ) ) ;
#2087=ORIENTED_EDGE ( 'NONE', *, *, #21136, .T. ) ;
#2088=EDGE_CURVE ( 'NONE', #26833, #15434, #35682, .T. ) ;
#2089=VERTEX_POINT ( 'NONE', #26018 ) ;
#2090=DIRECTION ( 'NONE',  ( 1.000000000000000000, 0.000000000000000000, 0.000000000000000000 ) ) ;
#2094=EDGE_CURVE ( 'NONE', #27785, #30348, #7546, .T. ) ;
#2095=CARTESIAN_POINT ( 'NONE',  ( 69.99999662536839651, 17.32050807568879236, 17.49999999999999645 ) ) ;
#2097=ORIENTED_EDGE ( 'NONE', *, *, #13664, .F. ) ;
#2098=DIRECTION ( 'NONE',  ( 0.000000000000000000, 0.000000000000000000, -1.000000000000000000 ) ) ;
#2099=CIRCLE ( 'NONE', #31993, 2.000000000000000000 ) ;
#2100=VERTEX_POINT ( 'NONE', #886 ) ;
#2102=FACE_BOUND ( 'NONE', #27319, .T. ) ;
#2105=ORIENTED_EDGE ( 'NONE', *, *, #29918, .T. ) ;
#2106=CIRCLE ( 'NONE', #5114, 2.000000000000001776 ) ;
#2107=CYLINDRICAL_SURFACE ( 'NONE', #27997, 27.00000000000001421 ) ;
#2108=DIRECTION ( 'NONE',  ( 0.000000000000000000, 0.000000000000000000, 1.000000000000000000 ) ) ;
#2109=ORIENTED_EDGE ( 'NONE', *, *, #26290, .T. ) ;
#2110=ORIENTED_EDGE ( 'NONE', *, *, #799, .F. ) ;
#2111=FACE_OUTER_BOUND ( 'NONE', #35952, .T. ) ;
#2112=CIRCLE ( 'NONE', #14688, 1.999999999999998224 ) ;
#2114=AXIS2_PLACEMENT_3D ( 'NONE', #13605, #30833, #5539 ) ;
#2115=CARTESIAN_POINT ( 'NONE',  ( -47.00000337463112743, -60.62177826491080168, -9.999999999999998224 ) ) ;
#2116=AXIS2_PLACEMENT_3D ( 'NONE', #1276, #15536, #34179 ) ;
#2117=DIRECTION ( 'NONE',  ( -1.000000000000000000, 0.000000000000000000, 0.000000000000000000 ) ) ;
#2120=FACE_BOUND ( 'NONE', #34435, .T. ) ;
#2122=CARTESIAN_POINT ( 'NONE',  ( 47.04203867989577503, -43.19957991610382919, 12.49999999999999822 ) ) ;
#2123=FACE_OUTER_BOUND ( 'NONE', #19915, .T. ) ;
#2124=CARTESIAN_POINT ( 'NONE',  ( -70.00000337463099243, 34.64101615137758472, -9.999999999999998224 ) ) ;
#2125=CARTESIAN_POINT ( 'NONE',  ( 29.99999662536857770, -69.28203230275519786, 12.50000000000000000 ) ) ;
#2127=LINE ( 'NONE', #13767, #11576 ) ;
#2128=EDGE_CURVE ( 'NONE', #8511, #6351, #19510, .T. ) ;
#2129=ORIENTED_EDGE ( 'NONE', *, *, #31840, .F. ) ;
#2130=FACE_OUTER_BOUND ( 'NONE', #32941, .T. ) ;
#2131=AXIS2_PLACEMENT_3D ( 'NONE', #33816, #5677, #19380 ) ;
#2132=DIRECTION ( 'NONE',  ( 0.000000000000000000, 0.000000000000000000, 1.000000000000000000 ) ) ;
#2134=CIRCLE ( 'NONE', #29070, 27.00000000000001421 ) ;
#2135=AXIS2_PLACEMENT_3D ( 'NONE', #29869, #17883, #35337 ) ;
#2136=CIRCLE ( 'NONE', #31455, 2.000000000000000000 ) ;
#2138=CIRCLE ( 'NONE', #33893, 2.000000000000001776 ) ;
#2139=EDGE_CURVE ( 'NONE', #28708, #13783, #17130, .T. ) ;
#2140=ORIENTED_EDGE ( 'NONE', *, *, #5981, .F. ) ;
#2141=EDGE_LOOP ( 'NONE', ( #82, #30005, #22727, #24066 ) ) ;
#2142=EDGE_CURVE ( 'NONE', #5127, #11641, #23776, .T. ) ;
#2144=CARTESIAN_POINT ( 'NONE',  ( 34.99999662536853862, 77.94228634059959404, -9.999999999999998224 ) ) ;
#2145=ORIENTED_EDGE ( 'NONE', *, *, #1881, .T. ) ;
#2146=CIRCLE ( 'NONE', #23099, 2.000000000000001776 ) ;
#2147=CARTESIAN_POINT ( 'NONE',  ( 77.99999662536833966, -3.224517592124143893E-15, -5.000000000000000000 ) ) ;
#2148=DIRECTION ( 'NONE',  ( 0.000000000000000000, 0.000000000000000000, 1.000000000000000000 ) ) ;
#2149=ORIENTED_EDGE ( 'NONE', *, *, #3807, .F. ) ;
#2151=ORIENTED_EDGE ( 'NONE', *, *, #16537, .T. ) ;
#2152=CARTESIAN_POINT ( 'NONE',  ( 89.99999662536828282, 0.000000000000000000, 12.50000000000000000 ) ) ;
#2153=AXIS2_PLACEMENT_3D ( 'NONE', #23156, #6817, #9259 ) ;
#2154=CYLINDRICAL_SURFACE ( 'NONE', #9416, 2.000000000000001776 ) ;
#2156=AXIS2_PLACEMENT_3D ( 'NONE', #16768, #14489, #13760 ) ;
#2157=CIRCLE ( 'NONE', #15323, 2.000000000000001776 ) ;
#2158=ORIENTED_EDGE ( 'NONE', *, *, #27351, .F. ) ;
#2161=AXIS2_PLACEMENT_3D ( 'NONE', #15520, #17959, #12680 ) ;
#2163=AXIS2_PLACEMENT_3D ( 'NONE', #18128, #17759, #29196 ) ;
#2164=EDGE_CURVE ( 'NONE', #32910, #5560, #32664, .T. ) ;
#2165=CIRCLE ( 'NONE', #18926, 2.000000000000001776 ) ;
#2167=CARTESIAN_POINT ( 'NONE',  ( -67.00000337463104927, -25.98076211353322051, -9.999999999999998224 ) ) ;
#2168=AXIS2_PLACEMENT_3D ( 'NONE', #17752, #23565, #8412 ) ;
#2169=ORIENTED_EDGE ( 'NONE', *, *, #8510, .T. ) ;
#2172=VERTEX_POINT ( 'NONE', #35969 ) ;
#2173=DIRECTION ( 'NONE',  ( 0.000000000000000000, 0.000000000000000000, 1.000000000000000000 ) ) ;
#2174=DIRECTION ( 'NONE',  ( 0.000000000000000000, 0.000000000000000000, -1.000000000000000000 ) ) ;
#2175=DIRECTION ( 'NONE',  ( 1.000000000000000000, 0.000000000000000000, 0.000000000000000000 ) ) ;
#2176=EDGE_CURVE ( 'NONE', #9542, #29900, #16510, .T. ) ;
#2177=VERTEX_POINT ( 'NONE', #4646 ) ;
#2178=ORIENTED_EDGE ( 'NONE', *, *, #29139, .T. ) ;
#2179=LINE ( 'NONE', #36861, #9385 ) ;
#2181=AXIS2_PLACEMENT_3D ( 'NONE', #2673, #2879, #25023 ) ;
#2182=FACE_OUTER_BOUND ( 'NONE', #27550, .T. ) ;
#2183=EDGE_LOOP ( 'NONE', ( #36867, #15554, #36057, #31956 ) ) ;
#2186=EDGE_CURVE ( 'NONE', #14320, #21597, #15885, .T. ) ;
#2188=CARTESIAN_POINT ( 'NONE',  ( -38.00000337463113453, -69.28203230275519786, -9.999999999999998224 ) ) ;
#2191=AXIS2_PLACEMENT_3D ( 'NONE', #6241, #3249, #23880 ) ;
#2192=AXIS2_PLACEMENT_3D ( 'NONE', #9463, #20894, #16562 ) ;
#2195=EDGE_LOOP ( 'NONE', ( #5622, #36339, #21023, #6317 ) ) ;
#2196=CIRCLE ( 'NONE', #26147, 2.000000000000001776 ) ;
#2197=ORIENTED_EDGE ( 'NONE', *, *, #18735, .T. ) ;
#2198=FACE_OUTER_BOUND ( 'NONE', #28753, .T. ) ;
#2199=AXIS2_PLACEMENT_3D ( 'NONE', #36677, #16425, #22244 ) ;
#2200=CARTESIAN_POINT ( 'NONE',  ( -20.39230267490738768, 84.64139243425341874, -5.000000000000000000 ) ) ;
#2201=VERTEX_POINT ( 'NONE', #24139 ) ;
#2204=FACE_BOUND ( 'NONE', #6962, .T. ) ;
#2205=CIRCLE ( 'NONE', #23754, 2.000000000000001776 ) ;
#2206=CARTESIAN_POINT ( 'NONE',  ( -50.00000337463109190, 69.28203230275518365, -9.999999999999998224 ) ) ;
#2208=DIRECTION ( 'NONE',  ( -1.000000000000000000, 0.000000000000000000, 0.000000000000000000 ) ) ;
#2209=ORIENTED_EDGE ( 'NONE', *, *, #20485, .T. ) ;
#2210=EDGE_CURVE ( 'NONE', #8614, #18736, #24297, .T. ) ;
#2211=CARTESIAN_POINT ( 'NONE',  ( 67.99999662536838230, -17.32050807568879947, 12.50000000000000000 ) ) ;
#2213=CARTESIAN_POINT ( 'NONE',  ( -2.000003374631327713, 86.60254037844397601, -9.999999999999998224 ) ) ;
#2214=DIRECTION ( 'NONE',  ( 1.000000000000000000, 0.000000000000000000, 0.000000000000000000 ) ) ;
#2216=ORIENTED_EDGE ( 'NONE', *, *, #36204, .T. ) ;
#2217=CARTESIAN_POINT ( 'NONE',  ( 44.99999662536849598, 60.62177826491077326, 12.50000000000000000 ) ) ;
#2218=EDGE_CURVE ( 'NONE', #13427, #1092, #31010, .T. ) ;
#2220=CYLINDRICAL_SURFACE ( 'NONE', #20250, 2.000000000000001776 ) ;
#2221=FACE_OUTER_BOUND ( 'NONE', #3395, .T. ) ;
#2223=CIRCLE ( 'NONE', #4616, 2.000000000000001776 ) ;
#2224=EDGE_LOOP ( 'NONE', ( #6573, #23462 ) ) ;
#2225=AXIS2_PLACEMENT_3D ( 'NONE', #19870, #5267, #34141 ) ;
#2226=AXIS2_PLACEMENT_3D ( 'NONE', #13009, #30247, #28002 ) ;
#2230=ORIENTED_EDGE ( 'NONE', *, *, #23922, .T. ) ;
#2231=CARTESIAN_POINT ( 'NONE',  ( -70.00000337463102085, -51.96152422706641971, -5.000000000000000000 ) ) ;
#2232=AXIS2_PLACEMENT_3D ( 'NONE', #31970, #17750, #3522 ) ;
#2233=DIRECTION ( 'NONE',  ( 0.000000000000000000, 0.000000000000000000, 1.000000000000000000 ) ) ;
#2234=AXIS2_PLACEMENT_3D ( 'NONE', #6999, #18448, #27229 ) ;
#2236=DIRECTION ( 'NONE',  ( 0.000000000000000000, 0.000000000000000000, -1.000000000000000000 ) ) ;
#2237=DIRECTION ( 'NONE',  ( 0.000000000000000000, 0.000000000000000000, 1.000000000000000000 ) ) ;
#2240=CIRCLE ( 'NONE', #29180, 3.499999999999989342 ) ;
#2241=CARTESIAN_POINT ( 'NONE',  ( -55.00000337463107059, 43.30127018922197379, -9.999999999999998224 ) ) ;
#2242=ORIENTED_EDGE ( 'NONE', *, *, #33594, .T. ) ;
#2245=EDGE_CURVE ( 'NONE', #5952, #8794, #36404, .T. ) ;
#2247=DIRECTION ( 'NONE',  ( -1.000000000000000000, 0.000000000000000000, 0.000000000000000000 ) ) ;
#2248=DIRECTION ( 'NONE',  ( 0.000000000000000000, 0.000000000000000000, 1.000000000000000000 ) ) ;
#2249=DIRECTION ( 'NONE',  ( 1.000000000000000000, 0.000000000000000000, 0.000000000000000000 ) ) ;
#2250=ORIENTED_EDGE ( 'NONE', *, *, #306, .T. ) ;
#2253=AXIS2_PLACEMENT_3D ( 'NONE', #34288, #17766, #2795 ) ;
#2254=AXIS2_PLACEMENT_3D ( 'NONE', #33238, #4930, #18452 ) ;
#2255=CYLINDRICAL_SURFACE ( 'NONE', #8989, 2.000000000000001776 ) ;
#2257=EDGE_LOOP ( 'NONE', ( #14402, #32970 ) ) ;
#2258=EDGE_CURVE ( 'NONE', #20554, #12415, #35201, .T. ) ;
#2259=CARTESIAN_POINT ( 'NONE',  ( 61.99999662536845335, 34.64101615137759893, -5.000000000000000000 ) ) ;
#2260=VERTEX_POINT ( 'NONE', #9706 ) ;
#2261=CARTESIAN_POINT ( 'NONE',  ( 62.99999662536841072, 25.98076211353318854, -9.999999999999998224 ) ) ;
#2263=AXIS2_PLACEMENT_3D ( 'NONE', #11868, #6071, #29112 ) ;
#2264=DIRECTION ( 'NONE',  ( 0.000000000000000000, 0.000000000000000000, 1.000000000000000000 ) ) ;
#2265=ORIENTED_EDGE ( 'NONE', *, *, #13282, .T. ) ;
#2266=VERTEX_POINT ( 'NONE', #30121 ) ;
#2267=AXIS2_PLACEMENT_3D ( 'NONE', #28414, #22991, #34430 ) ;
#2269=ORIENTED_EDGE ( 'NONE', *, *, #12176, .F. ) ;
#2270=AXIS2_PLACEMENT_3D ( 'NONE', #29545, #11559, #20743 ) ;
#2272=AXIS2_PLACEMENT_3D ( 'NONE', #6781, #6424, #17863 ) ;
#2273=VERTEX_POINT ( 'NONE', #24887 ) ;
#2274=CARTESIAN_POINT ( 'NONE',  ( 52.99999662536844625, 43.30127018922198801, -9.999999999999998224 ) ) ;
#2275=CARTESIAN_POINT ( 'NONE',  ( -51.67317684408315870, -68.18636331025710717, 12.50000000000000000 ) ) ;
#2277=CARTESIAN_POINT ( 'NONE',  ( -70.00000337463102085, -34.64101615137762025, 12.50000000000000000 ) ) ;
#2279=ORIENTED_EDGE ( 'NONE', *, *, #2915, .F. ) ;
#2281=AXIS2_PLACEMENT_3D ( 'NONE', #36376, #7313, #10685 ) ;
#2282=DIRECTION ( 'NONE',  ( 0.000000000000000000, 0.000000000000000000, 1.000000000000000000 ) ) ;
#2284=VERTEX_POINT ( 'NONE', #25089 ) ;
#2285=CARTESIAN_POINT ( 'NONE',  ( 51.99999662536847467, 51.96152422706637708, -9.999999999999998224 ) ) ;
#2287=AXIS2_PLACEMENT_3D ( 'NONE', #11204, #36548, #17213 ) ;
#2288=ORIENTED_EDGE ( 'NONE', *, *, #12048, .F. ) ;
#2289=EDGE_LOOP ( 'NONE', ( #27948, #25590, #25487, #24034, #12444 ) ) ;
#2290=EDGE_CURVE ( 'NONE', #36088, #1094, #22627, .T. ) ;
#2291=CARTESIAN_POINT ( 'NONE',  ( -56.67878100130369035, 27.78182860042797131, 12.49999999999999822 ) ) ;
#2292=CARTESIAN_POINT ( 'NONE',  ( 35.19434990244975126, -52.39915983220758022, 12.49999999999999822 ) ) ;
#2295=LINE ( 'NONE', #24801, #13171 ) ;
#2297=ORIENTED_EDGE ( 'NONE', *, *, #13007, .F. ) ;
#2300=CIRCLE ( 'NONE', #30426, 2.000000000000001776 ) ;
#2301=EDGE_CURVE ( 'NONE', #19227, #13708, #19035, .T. ) ;
#2302=CARTESIAN_POINT ( 'NONE',  ( 82.99999662536831124, -8.660254037844397956, 17.49999999999999645 ) ) ;
#2304=EDGE_LOOP ( 'NONE', ( #36745, #23293, #34724, #3964 ) ) ;
#2306=EDGE_CURVE ( 'NONE', #18101, #36107, #1056, .T. ) ;
#2307=DIRECTION ( 'NONE',  ( 0.000000000000000000, 0.000000000000000000, -1.000000000000000000 ) ) ;
#2308=ORIENTED_EDGE ( 'NONE', *, *, #5946, .T. ) ;
#2309=CIRCLE ( 'NONE', #32845, 2.000000000000001776 ) ;
#2310=VERTEX_POINT ( 'NONE', #10437 ) ;
#2311=AXIS2_PLACEMENT_3D ( 'NONE', #30995, #16924, #8121 ) ;
#2312=CARTESIAN_POINT ( 'NONE',  ( -70.00000337463099243, 17.32050807568877460, 12.50000000000000000 ) ) ;
#2313=FACE_OUTER_BOUND ( 'NONE', #36206, .T. ) ;
#2314=VERTEX_POINT ( 'NONE', #19819 ) ;
#2315=ORIENTED_EDGE ( 'NONE', *, *, #25346, .T. ) ;
#2316=FACE_OUTER_BOUND ( 'NONE', #27302, .T. ) ;
#2317=CIRCLE ( 'NONE', #18458, 2.000000000000001776 ) ;
#2318=CARTESIAN_POINT ( 'NONE',  ( -48.00000337463109190, 51.96152422706637708, 12.50000000000000000 ) ) ;
#2319=EDGE_CURVE ( 'NONE', #34031, #34954, #15436, .T. ) ;
#2320=DIRECTION ( 'NONE',  ( 1.000000000000000000, 0.000000000000000000, 0.000000000000000000 ) ) ;
#2321=EDGE_CURVE ( 'NONE', #35319, #3063, #13048, .T. ) ;
#2322=LINE ( 'NONE', #2670, #35852 ) ;
#2324=VERTEX_POINT ( 'NONE', #19090 ) ;
#2325=CARTESIAN_POINT ( 'NONE',  ( -30.00000337463118427, 69.28203230275516944, -9.999999999999998224 ) ) ;
#2326=AXIS2_PLACEMENT_3D ( 'NONE', #24768, #9598, #21022 ) ;
#2327=FACE_BOUND ( 'NONE', #35983, .T. ) ;
#2328=CIRCLE ( 'NONE', #7113, 2.000000000000001776 ) ;
#2329=FACE_OUTER_BOUND ( 'NONE', #1335, .T. ) ;
#2330=FACE_BOUND ( 'NONE', #30307, .T. ) ;
#2331=CARTESIAN_POINT ( 'NONE',  ( 4.279621169095998212, -62.97617850287780072, 12.49999999999999822 ) ) ;
#2332=CARTESIAN_POINT ( 'NONE',  ( 95.00000000000001421, 0.000000000000000000, -10.00000000000000000 ) ) ;
#2333=DIRECTION ( 'NONE',  ( 0.000000000000000000, 0.000000000000000000, 1.000000000000000000 ) ) ;
#2335=AXIS2_PLACEMENT_3D ( 'NONE', #1191, #15236, #29478 ) ;
#2336=FACE_OUTER_BOUND ( 'NONE', #9314, .T. ) ;
#2337=ORIENTED_EDGE ( 'NONE', *, *, #17534, .F. ) ;
#2338=DIRECTION ( 'NONE',  ( 0.000000000000000000, 0.000000000000000000, -1.000000000000000000 ) ) ;
#2339=DIRECTION ( 'NONE',  ( 0.000000000000000000, 0.000000000000000000, -1.000000000000000000 ) ) ;
#2340=DIRECTION ( 'NONE',  ( 1.000000000000000000, 0.000000000000000000, 0.000000000000000000 ) ) ;
#2341=AXIS2_PLACEMENT_3D ( 'NONE', #34131, #36741, #8788 ) ;
#2342=ORIENTED_EDGE ( 'NONE', *, *, #14576, .F. ) ;
#2343=CIRCLE ( 'NONE', #34680, 2.000000000000001776 ) ;
#2344=VERTEX_POINT ( 'NONE', #13256 ) ;
#2345=ADVANCED_FACE ( 'NONE', ( #30859 ), #13424, .F. ) ;
#2346=VERTEX_POINT ( 'NONE', #8191 ) ;
#2347=CARTESIAN_POINT ( 'NONE',  ( -75.00000337463097821, -8.660254037844422825, -5.000000000000000000 ) ) ;
#2348=DIRECTION ( 'NONE',  ( 1.000000000000000000, 0.000000000000000000, 0.000000000000000000 ) ) ;
#2350=ORIENTED_EDGE ( 'NONE', *, *, #36591, .F. ) ;
#2352=AXIS2_PLACEMENT_3D ( 'NONE', #2770, #20383, #34652 ) ;
#2353=CARTESIAN_POINT ( 'NONE',  ( 24.99999662536857059, 77.94228634059957983, -9.999999999999998224 ) ) ;
#2354=VERTEX_POINT ( 'NONE', #2188 ) ;
#2355=CARTESIAN_POINT ( 'NONE',  ( 37.27962116909601065, -62.97617850287780072, 12.49999999999999822 ) ) ;
#2356=ORIENTED_EDGE ( 'NONE', *, *, #23989, .T. ) ;
#2357=EDGE_CURVE ( 'NONE', #7889, #2089, #16435, .T. ) ;
#2358=VECTOR ( 'NONE', #23598, 1000.000000000000000 ) ;
#2359=CARTESIAN_POINT ( 'NONE',  ( 15.97563234535730814, -90.60231327712320137, -49.86561046011506448 ) ) ;
#2361=DIRECTION ( 'NONE',  ( 0.000000000000000000, 0.000000000000000000, 1.000000000000000000 ) ) ;
#2362=VECTOR ( 'NONE', #35553, 1000.000000000000000 ) ;
#2363=VERTEX_POINT ( 'NONE', #7836 ) ;
#2365=VECTOR ( 'NONE', #28251, 1000.000000000000000 ) ;
#2367=DIRECTION ( 'NONE',  ( 0.000000000000000000, 0.000000000000000000, 1.000000000000000000 ) ) ;
#2369=CARTESIAN_POINT ( 'NONE',  ( 74.99999662536835388, -25.98076211353319565, -9.999999999999998224 ) ) ;
#2370=CIRCLE ( 'NONE', #36502, 2.000000000000001776 ) ;
#2371=ADVANCED_FACE ( 'NONE', ( #17540 ), #28613, .F. ) ;
#2373=DIRECTION ( 'NONE',  ( 0.000000000000000000, 0.000000000000000000, 1.000000000000000000 ) ) ;
#2376=ORIENTED_EDGE ( 'NONE', *, *, #15078, .F. ) ;
#2377=AXIS2_PLACEMENT_3D ( 'NONE', #18920, #27554, #1860 ) ;
#2378=CARTESIAN_POINT ( 'NONE',  ( 69.99999662536838230, -34.64101615137759183, -9.999999999999998224 ) ) ;
#2379=DIRECTION ( 'NONE',  ( -1.000000000000000000, 0.000000000000000000, 0.000000000000000000 ) ) ;
#2380=CARTESIAN_POINT ( 'NONE',  ( 4.999996625368676284, -77.94228634059960825, 17.49999999999999645 ) ) ;
#2381=CARTESIAN_POINT ( 'NONE',  ( -50.00000337463110611, -69.28203230275519786, -9.999999999999998224 ) ) ;
#2382=AXIS2_PLACEMENT_3D ( 'NONE', #1711, #32836, #7157 ) ;
#2383=ORIENTED_EDGE ( 'NONE', *, *, #14978, .T. ) ;
#2384=VECTOR ( 'NONE', #13407, 1000.000000000000000 ) ;
#2385=ORIENTED_EDGE ( 'NONE', *, *, #9349, .F. ) ;
#2388=CARTESIAN_POINT ( 'NONE',  ( -13.00000337463126066, 77.94228634059957983, -9.999999999999998224 ) ) ;
#2389=ORIENTED_EDGE ( 'NONE', *, *, #22724, .F. ) ;
#2390=ORIENTED_EDGE ( 'NONE', *, *, #26400, .T. ) ;
#2391=CARTESIAN_POINT ( 'NONE',  ( -70.00000337463102085, -51.96152422706641971, -9.999999999999998224 ) ) ;
#2392=DIRECTION ( 'NONE',  ( 1.000000000000000000, 0.000000000000000000, 0.000000000000000000 ) ) ;
#2393=CARTESIAN_POINT ( 'NONE',  ( 52.99999662536844625, 43.30127018922198801, 12.50000000000000000 ) ) ;
#2394=CIRCLE ( 'NONE', #7180, 2.000000000000001776 ) ;
#2395=EDGE_CURVE ( 'NONE', #24063, #34902, #11255, .T. ) ;
#2396=ORIENTED_EDGE ( 'NONE', *, *, #7192, .T. ) ;
#2400=VERTEX_POINT ( 'NONE', #109 ) ;
#2401=AXIS2_PLACEMENT_3D ( 'NONE', #5882, #34567, #28907 ) ;
#2402=CARTESIAN_POINT ( 'NONE',  ( 54.99999662536844625, 60.62177826491077326, -5.000000000000000000 ) ) ;
#2403=VERTEX_POINT ( 'NONE', #3120 ) ;
#2404=FACE_BOUND ( 'NONE', #33236, .T. ) ;
#2406=DIRECTION ( 'NONE',  ( 0.000000000000000000, 0.000000000000000000, 1.000000000000000000 ) ) ;
#2407=VECTOR ( 'NONE', #30394, 1000.000000000000000 ) ;
#2408=CIRCLE ( 'NONE', #22784, 2.000000000000001776 ) ;
#2409=ORIENTED_EDGE ( 'NONE', *, *, #19176, .T. ) ;
#2411=CARTESIAN_POINT ( 'NONE',  ( -75.00000337463097821, -8.660254037844422825, -9.999999999999998224 ) ) ;
#2412=CARTESIAN_POINT ( 'NONE',  ( 56.67878100130369035, -27.78182860042797131, 12.49999999999999822 ) ) ;
#2413=CARTESIAN_POINT ( 'NONE',  ( -3.374631303565411855E-06, -86.60254037844400443, -9.999999999999998224 ) ) ;
#2414=EDGE_CURVE ( 'NONE', #2314, #31389, #9440, .T. ) ;
#2415=ORIENTED_EDGE ( 'NONE', *, *, #25215, .F. ) ;
#2416=CYLINDRICAL_SURFACE ( 'NONE', #11876, 2.000000000000001776 ) ;
#2417=DIRECTION ( 'NONE',  ( -1.000000000000000000, 0.000000000000000000, 0.000000000000000000 ) ) ;
#2418=CARTESIAN_POINT ( 'NONE',  ( 39.99999662536853151, -69.28203230275519786, -9.999999999999998224 ) ) ;
#2419=AXIS2_PLACEMENT_3D ( 'NONE', #5260, #22139, #15949 ) ;
#2421=ORIENTED_EDGE ( 'NONE', *, *, #16207, .F. ) ;
#2422=VECTOR ( 'NONE', #3576, 1000.000000000000000 ) ;
#2423=CARTESIAN_POINT ( 'NONE',  ( -89.27079897466126113, 32.49191361593859284, 12.49999999999999822 ) ) ;
#2424=ORIENTED_EDGE ( 'NONE', *, *, #9001, .T. ) ;
#2426=CIRCLE ( 'NONE', #7217, 2.000000000000001776 ) ;
#2428=DIRECTION ( 'NONE',  ( -0.000000000000000000, 0.000000000000000000, -1.000000000000000000 ) ) ;
#2431=CARTESIAN_POINT ( 'NONE',  ( 84.99999662536831124, -8.660254037844397956, -9.999999999999998224 ) ) ;
#2433=EDGE_CURVE ( 'NONE', #666, #5093, #11536, .T. ) ;
#2434=DIRECTION ( 'NONE',  ( 0.000000000000000000, 0.000000000000000000, 1.000000000000000000 ) ) ;
#2435=EDGE_LOOP ( 'NONE', ( #16819, #36767, #30220, #22143 ) ) ;
#2436=EDGE_LOOP ( 'NONE', ( #3625, #23425, #29411, #17365 ) ) ;
#2438=DIRECTION ( 'NONE',  ( -1.000000000000000000, 1.516276816038986019E-14, 0.000000000000000000 ) ) ;
#2442=ORIENTED_EDGE ( 'NONE', *, *, #35938, .T. ) ;
#2444=EDGE_CURVE ( 'NONE', #17808, #17256, #28598, .T. ) ;
#2445=CARTESIAN_POINT ( 'NONE',  ( 71.99999662536839651, -17.32050807568879947, -5.000000000000000000 ) ) ;
#2446=ORIENTED_EDGE ( 'NONE', *, *, #26140, .F. ) ;
#2447=VERTEX_POINT ( 'NONE', #20363 ) ;
#2448=AXIS2_PLACEMENT_3D ( 'NONE', #13467, #24931, #36371 ) ;
#2449=FACE_OUTER_BOUND ( 'NONE', #11683, .T. ) ;
#2450=ORIENTED_EDGE ( 'NONE', *, *, #25367, .F. ) ;
#2452=CARTESIAN_POINT ( 'NONE',  ( 54.99999662536846046, -43.30127018922200222, 17.49999999999999645 ) ) ;
#2453=DIRECTION ( 'NONE',  ( 0.000000000000000000, 0.000000000000000000, 1.000000000000000000 ) ) ;
#2455=EDGE_CURVE ( 'NONE', #27413, #25343, #26217, .T. ) ;
#2456=ORIENTED_EDGE ( 'NONE', *, *, #19213, .T. ) ;
#2457=ORIENTED_EDGE ( 'NONE', *, *, #32987, .T. ) ;
#2458=ORIENTED_EDGE ( 'NONE', *, *, #19080, .T. ) ;
#2459=ORIENTED_EDGE ( 'NONE', *, *, #28810, .T. ) ;
#2460=ORIENTED_EDGE ( 'NONE', *, *, #20527, .F. ) ;
#2461=DIRECTION ( 'NONE',  ( 0.000000000000000000, 0.000000000000000000, 1.000000000000000000 ) ) ;
#2462=CARTESIAN_POINT ( 'NONE',  ( 17.99999662536858835, 69.28203230275516944, 17.49999999999999645 ) ) ;
#2463=CARTESIAN_POINT ( 'NONE',  ( -80.00000337463096400, -34.64101615137762025, 12.50000000000000000 ) ) ;
#2466=ORIENTED_EDGE ( 'NONE', *, *, #20204, .T. ) ;
#2467=CARTESIAN_POINT ( 'NONE',  ( -62.00000337463104927, 51.96152422706639129, -9.999999999999998224 ) ) ;
#2468=EDGE_CURVE ( 'NONE', #12792, #26170, #32196, .T. ) ;
#2469=CARTESIAN_POINT ( 'NONE',  ( 59.99999662536845335, 34.64101615137759893, -9.999999999999998224 ) ) ;
#2470=EDGE_CURVE ( 'NONE', #19796, #2978, #10651, .T. ) ;
#2471=AXIS2_PLACEMENT_3D ( 'NONE', #8965, #28996, #3328 ) ;
#2472=CARTESIAN_POINT ( 'NONE',  ( 19.99999662536861678, -69.28203230275519786, -9.999999999999998224 ) ) ;
#2473=ORIENTED_EDGE ( 'NONE', *, *, #24422, .T. ) ;
#2474=FACE_OUTER_BOUND ( 'NONE', #32412, .T. ) ;
#2475=CYLINDRICAL_SURFACE ( 'NONE', #28523, 2.000000000000001776 ) ;
#2476=ORIENTED_EDGE ( 'NONE', *, *, #20416, .T. ) ;
#2477=EDGE_LOOP ( 'NONE', ( #15614, #4466 ) ) ;
#2482=EDGE_CURVE ( 'NONE', #30643, #32298, #37016, .T. ) ;
#2483=VERTEX_POINT ( 'NONE', #12079 ) ;
#2484=EDGE_LOOP ( 'NONE', ( #18047, #14457, #8542, #28271, #14081, #24475, #26306, #6737, #29059, #9151, #32316, #1437, #12204, #12891, #28177, #23491 ) ) ;
#2485=DIRECTION ( 'NONE',  ( -1.000000000000000000, 0.000000000000000000, 0.000000000000000000 ) ) ;
#2486=ADVANCED_FACE ( 'NONE', ( #3495 ), #26172, .F. ) ;
#2487=EDGE_LOOP ( 'NONE', ( #32209, #3344, #1157, #21393 ) ) ;
#2488=CIRCLE ( 'NONE', #34245, 2.000000000000001776 ) ;
#2489=CARTESIAN_POINT ( 'NONE',  ( -86.45172111230354517, 31.46585318596159553, 12.49999999999999822 ) ) ;
#2490=ORIENTED_EDGE ( 'NONE', *, *, #30442, .F. ) ;
#2493=CARTESIAN_POINT ( 'NONE',  ( -12.00000337463125000, -86.60254037844400443, -9.999999999999998224 ) ) ;
#2494=ORIENTED_EDGE ( 'NONE', *, *, #4463, .T. ) ;
#2496=CARTESIAN_POINT ( 'NONE',  ( 52.39915983220795681, 35.19434990244919703, -49.22241343995293761 ) ) ;
#2498=DIRECTION ( 'NONE',  ( 0.000000000000000000, 0.000000000000000000, 1.000000000000000000 ) ) ;
#2499=CARTESIAN_POINT ( 'NONE',  ( 62.99999662536839651, -43.30127018922199511, -9.999999999999998224 ) ) ;
#2500=ADVANCED_FACE ( 'NONE', ( #26363 ), #5557, .F. ) ;
#2501=ORIENTED_EDGE ( 'NONE', *, *, #19297, .F. ) ;
#2502=DIRECTION ( 'NONE',  ( 0.000000000000000000, 0.000000000000000000, 1.000000000000000000 ) ) ;
#2503=FACE_BOUND ( 'NONE', #7547, .T. ) ;
#2504=CARTESIAN_POINT ( 'NONE',  ( -72.28378166042018904, -61.53067111003240797, 12.49999999999999822 ) ) ;
#2505=DIRECTION ( 'NONE',  ( -1.000000000000000000, 0.000000000000000000, 0.000000000000000000 ) ) ;
#2507=CYLINDRICAL_SURFACE ( 'NONE', #11702, 3.000000000000002665 ) ;
#2508=EDGE_CURVE ( 'NONE', #6746, #22301, #29793, .T. ) ;
#2509=FACE_OUTER_BOUND ( 'NONE', #29914, .T. ) ;
#2510=VECTOR ( 'NONE', #7380, 1000.000000000000000 ) ;
#2511=EDGE_CURVE ( 'NONE', #15438, #20259, #18440, .T. ) ;
#2513=ORIENTED_EDGE ( 'NONE', *, *, #6238, .F. ) ;
#2514=CARTESIAN_POINT ( 'NONE',  ( 32.99999662536855283, 60.62177826491078747, -9.999999999999998224 ) ) ;
#2515=VECTOR ( 'NONE', #19728, 1000.000000000000000 ) ;
#2517=DIRECTION ( 'NONE',  ( -0.000000000000000000, -0.000000000000000000, 1.000000000000000000 ) ) ;
#2518=ORIENTED_EDGE ( 'NONE', *, *, #4874, .T. ) ;
#2520=ORIENTED_EDGE ( 'NONE', *, *, #3027, .F. ) ;
#2521=DIRECTION ( 'NONE',  ( 0.000000000000000000, 0.000000000000000000, 1.000000000000000000 ) ) ;
#2523=ORIENTED_EDGE ( 'NONE', *, *, #6441, .T. ) ;
#2524=CARTESIAN_POINT ( 'NONE',  ( 14.99999662536859901, 77.94228634059957983, -9.999999999999998224 ) ) ;
#2525=EDGE_CURVE ( 'NONE', #18182, #17536, #4688, .T. ) ;
#2527=DIRECTION ( 'NONE',  ( 1.000000000000000000, 0.000000000000000000, 0.000000000000000000 ) ) ;
#2528=EDGE_LOOP ( 'NONE', ( #22457, #26208 ) ) ;
#2529=DIRECTION ( 'NONE',  ( -0.000000000000000000, 0.000000000000000000, -1.000000000000000000 ) ) ;
#2531=CARTESIAN_POINT ( 'NONE',  ( 44.99999662536849598, 60.62177826491077326, -9.999999999999998224 ) ) ;
#2532=DIRECTION ( 'NONE',  ( 0.000000000000000000, 0.000000000000000000, 1.000000000000000000 ) ) ;
#2533=AXIS2_PLACEMENT_3D ( 'NONE', #35485, #23660, #31889 ) ;
#2534=ORIENTED_EDGE ( 'NONE', *, *, #28079, .F. ) ;
#2535=DIRECTION ( 'NONE',  ( 1.000000000000000000, 0.000000000000000000, 0.000000000000000000 ) ) ;
#2538=LINE ( 'NONE', #5920, #10414 ) ;
#2540=VERTEX_POINT ( 'NONE', #10039 ) ;
#2541=CARTESIAN_POINT ( 'NONE',  ( -70.00000337463099243, -2.428612866367529932E-14, -9.999999999999998224 ) ) ;
#2542=DIRECTION ( 'NONE',  ( 0.000000000000000000, 0.000000000000000000, 1.000000000000000000 ) ) ;
#2543=EDGE_LOOP ( 'NONE', ( #6067, #35259 ) ) ;
#2544=EDGE_CURVE ( 'NONE', #30363, #26529, #11826, .T. ) ;
#2545=DIRECTION ( 'NONE',  ( 0.000000000000000000, 0.000000000000000000, 1.000000000000000000 ) ) ;
#2546=CARTESIAN_POINT ( 'NONE',  ( -45.00000337463111322, 60.62177826491077326, -9.999999999999998224 ) ) ;
#2547=CYLINDRICAL_SURFACE ( 'NONE', #9388, 2.000000000000001776 ) ;
#2548=DIRECTION ( 'NONE',  ( 1.000000000000000000, 0.000000000000000000, 0.000000000000000000 ) ) ;
#2549=ADVANCED_FACE ( 'NONE', ( #1590 ), #4041, .F. ) ;
#2550=AXIS2_PLACEMENT_3D ( 'NONE', #23646, #20453, #1151 ) ;
#2552=ORIENTED_EDGE ( 'NONE', *, *, #28307, .T. ) ;
#2553=VERTEX_POINT ( 'NONE', #3841 ) ;
#2554=ADVANCED_FACE ( 'NONE', ( #35548 ), #18277, .T. ) ;
#2555=DIRECTION ( 'NONE',  ( 1.000000000000000000, 0.000000000000000000, 0.000000000000000000 ) ) ;
#2556=FACE_OUTER_BOUND ( 'NONE', #35426, .T. ) ;
#2559=EDGE_LOOP ( 'NONE', ( #23582, #8615, #5048, #3963 ) ) ;
#2560=CIRCLE ( 'NONE', #10341, 1.999999999999998224 ) ;
#2561=CARTESIAN_POINT ( 'NONE',  ( -59.29837256189559724, -31.02796211690927564, -4.999999999999997335 ) ) ;
#2563=CARTESIAN_POINT ( 'NONE',  ( -92.00000337463090716, -1.016341149603137227E-14, -9.999999999999998224 ) ) ;
#2564=EDGE_CURVE ( 'NONE', #16038, #35244, #25061, .T. ) ;
#2567=VERTEX_POINT ( 'NONE', #24278 ) ;
#2568=DIRECTION ( 'NONE',  ( 0.000000000000000000, 0.000000000000000000, 1.000000000000000000 ) ) ;
#2572=EDGE_CURVE ( 'NONE', #32411, #25244, #497, .T. ) ;
#2573=DIRECTION ( 'NONE',  ( 1.000000000000000000, 0.000000000000000000, 0.000000000000000000 ) ) ;
#2574=ORIENTED_EDGE ( 'NONE', *, *, #8150, .F. ) ;
#2575=FACE_BOUND ( 'NONE', #2672, .T. ) ;
#2576=CIRCLE ( 'NONE', #16967, 27.00000000000001421 ) ;
#2577=CARTESIAN_POINT ( 'NONE',  ( 81.99999662536832545, -17.32050807568879591, 17.49999999999999645 ) ) ;
#2578=ORIENTED_EDGE ( 'NONE', *, *, #24390, .T. ) ;
#2580=FACE_OUTER_BOUND ( 'NONE', #23319, .T. ) ;
#2581=AXIS2_PLACEMENT_3D ( 'NONE', #3831, #20705, #15829 ) ;
#2583=CARTESIAN_POINT ( 'NONE',  ( 54.99999662536844625, 43.30127018922198801, 12.50000000000000000 ) ) ;
#2584=ORIENTED_EDGE ( 'NONE', *, *, #20644, .F. ) ;
#2585=DIRECTION ( 'NONE',  ( 0.000000000000000000, 0.000000000000000000, 1.000000000000000000 ) ) ;
#2586=DIRECTION ( 'NONE',  ( -0.000000000000000000, -0.000000000000000000, 1.000000000000000000 ) ) ;
#2587=FACE_OUTER_BOUND ( 'NONE', #8879, .T. ) ;
#2588=ORIENTED_EDGE ( 'NONE', *, *, #34596, .T. ) ;
#2589=VERTEX_POINT ( 'NONE', #7233 ) ;
#2590=ORIENTED_EDGE ( 'NONE', *, *, #3746, .F. ) ;
#2592=CIRCLE ( 'NONE', #30123, 2.000000000000001776 ) ;
#2593=DIRECTION ( 'NONE',  ( -0.4999999999999980571, 0.8660254037844399289, 0.000000000000000000 ) ) ;
#2594=CIRCLE ( 'NONE', #19381, 27.00000000000001421 ) ;
#2595=CARTESIAN_POINT ( 'NONE',  ( 66.99999662536841072, 25.98076211353318854, 12.50000000000000000 ) ) ;
#2596=CARTESIAN_POINT ( 'NONE',  ( -65.00000337463106348, -60.62177826491083010, -9.999999999999998224 ) ) ;
#2600=LINE ( 'NONE', #11033, #29215 ) ;
#2601=ORIENTED_EDGE ( 'NONE', *, *, #32048, .T. ) ;
#2603=ORIENTED_EDGE ( 'NONE', *, *, #35793, .F. ) ;
#2604=CARTESIAN_POINT ( 'NONE',  ( -35.00000337463117717, -77.94228634059963667, -9.999999999999998224 ) ) ;
#2608=CARTESIAN_POINT ( 'NONE',  ( -72.77422209630326222, -61.06482292022084835, -5.000000000000000000 ) ) ;
#2609=DIRECTION ( 'NONE',  ( 1.000000000000000000, 0.000000000000000000, 0.000000000000000000 ) ) ;
#2611=AXIS2_PLACEMENT_3D ( 'NONE', #8921, #25425, #22619 ) ;
#2612=FACE_BOUND ( 'NONE', #23037, .T. ) ;
#2613=ORIENTED_EDGE ( 'NONE', *, *, #8439, .F. ) ;
#2615=DIRECTION ( 'NONE',  ( 1.000000000000000000, 0.000000000000000000, 0.000000000000000000 ) ) ;
#2616=CIRCLE ( 'NONE', #25961, 2.000000000000001776 ) ;
#2617=ORIENTED_EDGE ( 'NONE', *, *, #16998, .F. ) ;
#2618=CARTESIAN_POINT ( 'NONE',  ( -75.00000337463100664, -43.30127018922202353, -5.000000000000000000 ) ) ;
#2619=VECTOR ( 'NONE', #11370, 1000.000000000000000 ) ;
#2621=CARTESIAN_POINT ( 'NONE',  ( 34.00000000000068923, 58.88972745734143643, 12.49999999999999822 ) ) ;
#2622=ORIENTED_EDGE ( 'NONE', *, *, #35748, .T. ) ;
#2623=VERTEX_POINT ( 'NONE', #12651 ) ;
#2624=EDGE_CURVE ( 'NONE', #26555, #28818, #25647, .T. ) ;
#2625=ORIENTED_EDGE ( 'NONE', *, *, #20397, .F. ) ;
#2626=EDGE_CURVE ( 'NONE', #34851, #23895, #19062, .T. ) ;
#2628=ORIENTED_EDGE ( 'NONE', *, *, #21755, .F. ) ;
#2629=ORIENTED_EDGE ( 'NONE', *, *, #36873, .F. ) ;
#2630=DIRECTION ( 'NONE',  ( 0.000000000000000000, 0.000000000000000000, -1.000000000000000000 ) ) ;
#2631=CARTESIAN_POINT ( 'NONE',  ( -10.00000337463127842, -69.28203230275519786, -9.999999999999998224 ) ) ;
#2632=DIRECTION ( 'NONE',  ( 0.000000000000000000, 0.000000000000000000, 1.000000000000000000 ) ) ;
#2634=DIRECTION ( 'NONE',  ( -0.000000000000000000, -0.000000000000000000, 1.000000000000000000 ) ) ;
#2637=CYLINDRICAL_SURFACE ( 'NONE', #22796, 2.000000000000001776 ) ;
#2638=EDGE_CURVE ( 'NONE', #29503, #29624, #18467, .T. ) ;
#2640=ORIENTED_EDGE ( 'NONE', *, *, #7808, .T. ) ;
#2641=CARTESIAN_POINT ( 'NONE',  ( 17.99999662536861678, -86.60254037844400443, -9.999999999999998224 ) ) ;
#2643=EDGE_LOOP ( 'NONE', ( #29990, #31165, #7832, #12203 ) ) ;
#2644=AXIS2_PLACEMENT_3D ( 'NONE', #25344, #19725, #20271 ) ;
#2645=ORIENTED_EDGE ( 'NONE', *, *, #29562, .T. ) ;
#2650=DIRECTION ( 'NONE',  ( 1.000000000000000000, 0.000000000000000000, 0.000000000000000000 ) ) ;
#2651=VERTEX_POINT ( 'NONE', #12465 ) ;
#2652=ORIENTED_EDGE ( 'NONE', *, *, #14446, .T. ) ;
#2653=AXIS2_PLACEMENT_3D ( 'NONE', #15028, #26456, #763 ) ;
#2655=VERTEX_POINT ( 'NONE', #21095 ) ;
#2656=DIRECTION ( 'NONE',  ( 0.000000000000000000, 0.000000000000000000, 1.000000000000000000 ) ) ;
#2657=ORIENTED_EDGE ( 'NONE', *, *, #5667, .F. ) ;
#2659=DIRECTION ( 'NONE',  ( 0.000000000000000000, 0.000000000000000000, -1.000000000000000000 ) ) ;
#2660=DIRECTION ( 'NONE',  ( 0.000000000000000000, 0.000000000000000000, 1.000000000000000000 ) ) ;
#2663=ORIENTED_EDGE ( 'NONE', *, *, #27147, .F. ) ;
#2664=CIRCLE ( 'NONE', #23622, 2.000000000000001776 ) ;
#2665=ORIENTED_EDGE ( 'NONE', *, *, #5511, .F. ) ;
#2666=CARTESIAN_POINT ( 'NONE',  ( 9.999996625368655856, -86.60254037844400443, 12.50000000000000000 ) ) ;
#2667=DIRECTION ( 'NONE',  ( 1.000000000000000000, 0.000000000000000000, 0.000000000000000000 ) ) ;
#2668=EDGE_CURVE ( 'NONE', #26530, #21698, #11856, .T. ) ;
#2669=DIRECTION ( 'NONE',  ( 1.000000000000000000, 0.000000000000000000, 0.000000000000000000 ) ) ;
#2670=CARTESIAN_POINT ( 'NONE',  ( -48.00000337463110611, -69.28203230275519786, -9.999999999999998224 ) ) ;
#2671=AXIS2_PLACEMENT_3D ( 'NONE', #5844, #5299, #36976 ) ;
#2672=EDGE_LOOP ( 'NONE', ( #25843, #32072 ) ) ;
#2673=CARTESIAN_POINT ( 'NONE',  ( -35.00000337463116296, 77.94228634059957983, 12.50000000000000000 ) ) ;
#2675=DIRECTION ( 'NONE',  ( 0.000000000000000000, 0.000000000000000000, 1.000000000000000000 ) ) ;
#2676=EDGE_CURVE ( 'NONE', #31828, #15574, #7788, .T. ) ;
#2677=DIRECTION ( 'NONE',  ( -1.000000000000000000, 0.000000000000000000, 0.000000000000000000 ) ) ;
#2679=CARTESIAN_POINT ( 'NONE',  ( -47.00000337463112743, -60.62177826491080168, -9.999999999999998224 ) ) ;
#2680=FACE_OUTER_BOUND ( 'NONE', #35498, .T. ) ;
#2681=AXIS2_PLACEMENT_3D ( 'NONE', #6004, #6721, #17426 ) ;
#2685=AXIS2_PLACEMENT_3D ( 'NONE', #8365, #25963, #262 ) ;
#2686=DIRECTION ( 'NONE',  ( -1.000000000000000000, 0.000000000000000000, 0.000000000000000000 ) ) ;
#2691=VERTEX_POINT ( 'NONE', #22388 ) ;
#2693=ORIENTED_EDGE ( 'NONE', *, *, #1222, .F. ) ;
#2694=CIRCLE ( 'NONE', #12244, 3.000000000000002665 ) ;
#2695=DIRECTION ( 'NONE',  ( 0.000000000000000000, 0.000000000000000000, -1.000000000000000000 ) ) ;
#2696=DIRECTION ( 'NONE',  ( 1.000000000000000000, 0.000000000000000000, 0.000000000000000000 ) ) ;
#2697=AXIS2_PLACEMENT_3D ( 'NONE', #13812, #14164, #5182 ) ;
#2698=VERTEX_POINT ( 'NONE', #16228 ) ;
#2700=DIRECTION ( 'NONE',  ( 0.000000000000000000, 0.000000000000000000, -1.000000000000000000 ) ) ;
#2701=ADVANCED_FACE ( 'NONE', ( #5355 ), #36653, .F. ) ;
#2704=EDGE_LOOP ( 'NONE', ( #3407, #26222, #4553, #31576 ) ) ;
#2705=FACE_OUTER_BOUND ( 'NONE', #36826, .T. ) ;
#2706=EDGE_LOOP ( 'NONE', ( #16258, #7473, #35621, #6717 ) ) ;
#2708=ORIENTED_EDGE ( 'NONE', *, *, #24153, .F. ) ;
#2710=AXIS2_PLACEMENT_3D ( 'NONE', #3464, #20496, #29321 ) ;
#2711=DIRECTION ( 'NONE',  ( 0.000000000000000000, 0.000000000000000000, 1.000000000000000000 ) ) ;
#2712=DIRECTION ( 'NONE',  ( 0.000000000000000000, 0.000000000000000000, -1.000000000000000000 ) ) ;
#2713=ADVANCED_FACE ( 'NONE', ( #16589 ), #33086, .F. ) ;
#2714=ORIENTED_EDGE ( 'NONE', *, *, #25915, .T. ) ;
#2719=ORIENTED_EDGE ( 'NONE', *, *, #8887, .T. ) ;
#2721=DIRECTION ( 'NONE',  ( 0.000000000000000000, 0.000000000000000000, -1.000000000000000000 ) ) ;
#2723=CARTESIAN_POINT ( 'NONE',  ( -53.00000337463106348, 60.62177826491078747, -9.999999999999998224 ) ) ;
#2724=AXIS2_PLACEMENT_3D ( 'NONE', #7391, #16216, #33460 ) ;
#2725=CARTESIAN_POINT ( 'NONE',  ( 67.99999662536839651, 51.96152422706640550, 17.49999999999999645 ) ) ;
#2726=LINE ( 'NONE', #16976, #33360 ) ;
#2727=AXIS2_PLACEMENT_3D ( 'NONE', #35506, #12421, #9444 ) ;
#2729=CARTESIAN_POINT ( 'NONE',  ( 86.99999662536832545, 8.660254037844394404, -9.999999999999998224 ) ) ;
#2731=ORIENTED_EDGE ( 'NONE', *, *, #4905, .T. ) ;
#2732=ADVANCED_FACE ( 'NONE', ( #19230 ), #13584, .F. ) ;
#2733=AXIS2_PLACEMENT_3D ( 'NONE', #9394, #3598, #23287 ) ;
#2736=DIRECTION ( 'NONE',  ( 0.000000000000000000, 0.000000000000000000, 1.000000000000000000 ) ) ;
#2737=AXIS2_PLACEMENT_3D ( 'NONE', #7617, #13803, #30491 ) ;
#2739=ORIENTED_EDGE ( 'NONE', *, *, #29944, .T. ) ;
#2742=CARTESIAN_POINT ( 'NONE',  ( -10.00000337463128197, 86.60254037844397601, -9.999999999999998224 ) ) ;
#2743=CARTESIAN_POINT ( 'NONE',  ( -68.00000337463102085, -51.96152422706641971, -5.000000000000000000 ) ) ;
#2744=ORIENTED_EDGE ( 'NONE', *, *, #25381, .F. ) ;
#2745=EDGE_LOOP ( 'NONE', ( #11047, #12714 ) ) ;
#2746=LINE ( 'NONE', #25640, #9925 ) ;
#2747=EDGE_CURVE ( 'NONE', #35934, #20160, #25045, .T. ) ;
#2748=CIRCLE ( 'NONE', #19506, 2.000000000000001776 ) ;
#2749=DIRECTION ( 'NONE',  ( 1.000000000000000000, 0.000000000000000000, 0.000000000000000000 ) ) ;
#2750=ORIENTED_EDGE ( 'NONE', *, *, #7367, .F. ) ;
#2751=EDGE_CURVE ( 'NONE', #2567, #26082, #13667, .T. ) ;
#2752=CIRCLE ( 'NONE', #31475, 2.000000000000001776 ) ;
#2753=DIRECTION ( 'NONE',  ( -1.000000000000000000, 0.000000000000000000, 0.000000000000000000 ) ) ;
#2754=VERTEX_POINT ( 'NONE', #28203 ) ;
#2755=LINE ( 'NONE', #22830, #30881 ) ;
#2756=AXIS2_PLACEMENT_3D ( 'NONE', #30561, #19675, #13676 ) ;
#2757=CIRCLE ( 'NONE', #17132, 2.000000000000001776 ) ;
#2759=CIRCLE ( 'NONE', #23124, 2.000000000000001776 ) ;
#2760=CIRCLE ( 'NONE', #36305, 2.000000000000001776 ) ;
#2761=DIRECTION ( 'NONE',  ( 0.000000000000000000, 0.000000000000000000, 1.000000000000000000 ) ) ;
#2762=ADVANCED_FACE ( 'NONE', ( #30268 ), #22034, .F. ) ;
#2763=AXIS2_PLACEMENT_3D ( 'NONE', #13417, #10818, #21870 ) ;
#2764=ORIENTED_EDGE ( 'NONE', *, *, #2904, .T. ) ;
#2765=EDGE_CURVE ( 'NONE', #10183, #18228, #28331, .T. ) ;
#2767=AXIS2_PLACEMENT_3D ( 'NONE', #1600, #2911, #28576 ) ;
#2768=CARTESIAN_POINT ( 'NONE',  ( -67.00000337463102085, 43.30127018922198801, 17.49999999999999645 ) ) ;
#2769=CARTESIAN_POINT ( 'NONE',  ( 86.45172111230354517, -31.46585318596159553, 12.49999999999999822 ) ) ;
#2770=CARTESIAN_POINT ( 'NONE',  ( 0.000000000000000000, 0.000000000000000000, -5.000000000000000000 ) ) ;
#2771=ORIENTED_EDGE ( 'NONE', *, *, #17662, .T. ) ;
#2772=LINE ( 'NONE', #5024, #32218 ) ;
#2773=DIRECTION ( 'NONE',  ( 0.000000000000000000, 0.000000000000000000, 1.000000000000000000 ) ) ;
#2774=DIRECTION ( 'NONE',  ( 0.000000000000000000, 0.000000000000000000, -1.000000000000000000 ) ) ;
#2775=ADVANCED_FACE ( 'NONE', ( #4959 ), #21833, .F. ) ;
#2776=CIRCLE ( 'NONE', #25526, 3.000000000000006661 ) ;
#2777=ADVANCED_FACE ( 'NONE', ( #19046 ), #27819, .F. ) ;
#2778=ORIENTED_EDGE ( 'NONE', *, *, #32946, .T. ) ;
#2779=EDGE_LOOP ( 'NONE', ( #10001, #7376, #20857, #5494 ) ) ;
#2780=EDGE_CURVE ( 'NONE', #15508, #36358, #4977, .T. ) ;
#2781=CIRCLE ( 'NONE', #23737, 2.000000000000001776 ) ;
#2787=AXIS2_PLACEMENT_3D ( 'NONE', #19013, #34008, #30619 ) ;
#2789=AXIS2_PLACEMENT_3D ( 'NONE', #11858, #34927, #20475 ) ;
#2790=CARTESIAN_POINT ( 'NONE',  ( 78.38501592334911550, 33.46125459406803060, 12.50000000000000000 ) ) ;
#2791=AXIS2_PLACEMENT_3D ( 'NONE', #20164, #34063, #34615 ) ;
#2792=CARTESIAN_POINT ( 'NONE',  ( 71.99999662536839651, 34.64101615137758472, -9.999999999999998224 ) ) ;
#2795=DIRECTION ( 'NONE',  ( 1.000000000000000000, 0.000000000000000000, 0.000000000000000000 ) ) ;
#2796=DIRECTION ( 'NONE',  ( 0.000000000000000000, 0.000000000000000000, 1.000000000000000000 ) ) ;
#2797=EDGE_LOOP ( 'NONE', ( #7959, #33060, #6471, #16756 ) ) ;
#2798=CIRCLE ( 'NONE', #23164, 33.00000000000001421 ) ;
#2799=ORIENTED_EDGE ( 'NONE', *, *, #27985, .T. ) ;
#2801=EDGE_CURVE ( 'NONE', #18680, #7314, #7387, .T. ) ;
#2802=CARTESIAN_POINT ( 'NONE',  ( 66.99999662536841072, -25.98076211353320275, 17.49999999999999645 ) ) ;
#2803=LINE ( 'NONE', #3675, #25247 ) ;
#2805=ORIENTED_EDGE ( 'NONE', *, *, #7890, .T. ) ;
#2806=AXIS2_PLACEMENT_3D ( 'NONE', #27999, #16764, #28352 ) ;
#2807=AXIS2_PLACEMENT_3D ( 'NONE', #1863, #15924, #18924 ) ;
#2808=FACE_BOUND ( 'NONE', #9716, .T. ) ;
#2809=ORIENTED_EDGE ( 'NONE', *, *, #3813, .T. ) ;
#2810=EDGE_LOOP ( 'NONE', ( #29669, #1915, #18969, #23575 ) ) ;
#2812=VERTEX_POINT ( 'NONE', #28581 ) ;
#2815=AXIS2_PLACEMENT_3D ( 'NONE', #33287, #18291, #27280 ) ;
#2816=CARTESIAN_POINT ( 'NONE',  ( -20.00000337463123756, -86.60254037844400443, -5.000000000000000000 ) ) ;
#2817=CARTESIAN_POINT ( 'NONE',  ( -82.00000337463094979, 34.64101615137757051, -9.999999999999998224 ) ) ;
#2819=CARTESIAN_POINT ( 'NONE',  ( 72.99999662536835388, -25.98076211353319565, -9.999999999999998224 ) ) ;
#2824=EDGE_CURVE ( 'NONE', #16319, #10634, #31897, .T. ) ;
#2825=ORIENTED_EDGE ( 'NONE', *, *, #28978, .T. ) ;
#2827=EDGE_CURVE ( 'NONE', #22214, #19789, #29530, .T. ) ;
#2828=LINE ( 'NONE', #3016, #25423 ) ;
#2829=EDGE_CURVE ( 'NONE', #953, #23803, #15162, .T. ) ;
#2830=DIRECTION ( 'NONE',  ( 1.000000000000000000, 0.000000000000000000, 0.000000000000000000 ) ) ;
#2831=CARTESIAN_POINT ( 'NONE',  ( 11.99999662536865763, -69.28203230275519786, 17.49999999999999645 ) ) ;
#2832=CIRCLE ( 'NONE', #33461, 2.000000000000001776 ) ;
#2834=CARTESIAN_POINT ( 'NONE',  ( 67.99999662536839651, 51.96152422706640550, -9.999999999999998224 ) ) ;
#2835=CIRCLE ( 'NONE', #30361, 2.000000000000000000 ) ;
#2836=EDGE_LOOP ( 'NONE', ( #8618, #2442, #9985, #20484 ) ) ;
#2837=CARTESIAN_POINT ( 'NONE',  ( 34.46585318596250858, 86.45172111230321832, -49.86348611802629449 ) ) ;
#2838=CIRCLE ( 'NONE', #9995, 95.00000000000001421 ) ;
#2839=DIRECTION ( 'NONE',  ( 0.000000000000000000, 0.000000000000000000, 1.000000000000000000 ) ) ;
#2840=VECTOR ( 'NONE', #31547, 1000.000000000000000 ) ;
#2841=CARTESIAN_POINT ( 'NONE',  ( -4.279621169095561228, 62.97617850287782915, 12.49999999999999822 ) ) ;
#2842=VERTEX_POINT ( 'NONE', #5898 ) ;
#2843=CARTESIAN_POINT ( 'NONE',  ( -28.00000337463119493, -69.28203230275522628, -9.999999999999998224 ) ) ;
#2844=CIRCLE ( 'NONE', #23992, 2.000000000000001776 ) ;
#2845=DIRECTION ( 'NONE',  ( 0.000000000000000000, 0.000000000000000000, 1.000000000000000000 ) ) ;
#2847=ORIENTED_EDGE ( 'NONE', *, *, #326, .F. ) ;
#2848=CIRCLE ( 'NONE', #20814, 3.499999999999987566 ) ;
#2849=EDGE_LOOP ( 'NONE', ( #5620, #4658 ) ) ;
#2850=AXIS2_PLACEMENT_3D ( 'NONE', #4208, #10365, #13354 ) ;
#2851=DIRECTION ( 'NONE',  ( 0.000000000000000000, 0.000000000000000000, 1.000000000000000000 ) ) ;
#2852=DIRECTION ( 'NONE',  ( 0.000000000000000000, 0.000000000000000000, 1.000000000000000000 ) ) ;
#2854=DIRECTION ( 'NONE',  ( 0.000000000000000000, 0.000000000000000000, 1.000000000000000000 ) ) ;
#2855=ORIENTED_EDGE ( 'NONE', *, *, #19948, .T. ) ;
#2856=VERTEX_POINT ( 'NONE', #23324 ) ;
#2857=CIRCLE ( 'NONE', #14800, 1.999999999999998224 ) ;
#2859=DIRECTION ( 'NONE',  ( -0.000000000000000000, -0.000000000000000000, 1.000000000000000000 ) ) ;
#2860=DIRECTION ( 'NONE',  ( 1.000000000000000000, 0.000000000000000000, 0.000000000000000000 ) ) ;
#2862=ORIENTED_EDGE ( 'NONE', *, *, #24667, .F. ) ;
#2864=CARTESIAN_POINT ( 'NONE',  ( 19.99999662536861678, -69.28203230275519786, 12.50000000000000000 ) ) ;
#2866=CIRCLE ( 'NONE', #22613, 27.00000000000000711 ) ;
#2867=EDGE_LOOP ( 'NONE', ( #31463, #3366, #20490, #19599, #8376 ) ) ;
#2868=DIRECTION ( 'NONE',  ( 0.000000000000000000, 0.000000000000000000, 1.000000000000000000 ) ) ;
#2869=DIRECTION ( 'NONE',  ( 0.000000000000000000, 0.000000000000000000, -1.000000000000000000 ) ) ;
#2870=AXIS2_PLACEMENT_3D ( 'NONE', #4353, #4543, #27767 ) ;
#2871=FACE_BOUND ( 'NONE', #17915, .T. ) ;
#2872=ORIENTED_EDGE ( 'NONE', *, *, #5946, .F. ) ;
#2873=ORIENTED_EDGE ( 'NONE', *, *, #24308, .T. ) ;
#2874=DIRECTION ( 'NONE',  ( 1.000000000000000000, 0.000000000000000000, 0.000000000000000000 ) ) ;
#2875=CARTESIAN_POINT ( 'NONE',  ( 31.99999662536856704, 69.28203230275518365, -9.999999999999998224 ) ) ;
#2876=DIRECTION ( 'NONE',  ( -0.000000000000000000, 0.000000000000000000, -1.000000000000000000 ) ) ;
#2877=CYLINDRICAL_SURFACE ( 'NONE', #1127, 2.000000000000000000 ) ;
#2878=VERTEX_POINT ( 'NONE', #3444 ) ;
#2879=DIRECTION ( 'NONE',  ( 0.000000000000000000, 0.000000000000000000, 1.000000000000000000 ) ) ;
#2881=FACE_BOUND ( 'NONE', #3641, .T. ) ;
#2882=CARTESIAN_POINT ( 'NONE',  ( -70.00000337463099243, 34.64101615137758472, 12.50000000000000000 ) ) ;
#2883=CYLINDRICAL_SURFACE ( 'NONE', #27068, 3.000000000000002665 ) ;
#2886=CARTESIAN_POINT ( 'NONE',  ( 0.000000000000000000, 0.000000000000000000, -5.000000000000000000 ) ) ;
#2887=CYLINDRICAL_SURFACE ( 'NONE', #20958, 2.000000000000001776 ) ;
#2889=EDGE_LOOP ( 'NONE', ( #10879, #4992, #27135, #13817, #15532 ) ) ;
#2890=LINE ( 'NONE', #19580, #10066 ) ;
#2892=AXIS2_PLACEMENT_3D ( 'NONE', #35312, #27404, #9607 ) ;
#2893=DIRECTION ( 'NONE',  ( 1.000000000000000000, 0.000000000000000000, 0.000000000000000000 ) ) ;
#2894=CARTESIAN_POINT ( 'NONE',  ( 49.99999662536846756, -69.28203230275519786, 17.49999999999999645 ) ) ;
#2895=CIRCLE ( 'NONE', #20833, 2.000000000000001776 ) ;
#2896=ORIENTED_EDGE ( 'NONE', *, *, #8998, .F. ) ;
#2897=EDGE_LOOP ( 'NONE', ( #32096, #34103, #27596, #30792, #11181 ) ) ;
#2899=AXIS2_PLACEMENT_3D ( 'NONE', #22721, #22893, #31317 ) ;
#2900=DIRECTION ( 'NONE',  ( 0.000000000000000000, 0.000000000000000000, 1.000000000000000000 ) ) ;
#2901=DIRECTION ( 'NONE',  ( -1.000000000000000000, 0.000000000000000000, 0.000000000000000000 ) ) ;
#2902=CARTESIAN_POINT ( 'NONE',  ( 60.93295298011005201, 19.13981058454729123, 12.49999999999999822 ) ) ;
#2903=ORIENTED_EDGE ( 'NONE', *, *, #15040, .T. ) ;
#2904=EDGE_CURVE ( 'NONE', #2026, #29492, #34343, .T. ) ;
#2905=AXIS2_PLACEMENT_3D ( 'NONE', #19556, #10751, #22355 ) ;
#2906=CARTESIAN_POINT ( 'NONE',  ( 59.99999662536842493, -51.96152422706639840, -9.999999999999998224 ) ) ;
#2907=ORIENTED_EDGE ( 'NONE', *, *, #18493, .F. ) ;
#2908=DIRECTION ( 'NONE',  ( 0.000000000000000000, 0.000000000000000000, 1.000000000000000000 ) ) ;
#2909=EDGE_CURVE ( 'NONE', #37038, #23091, #21134, .T. ) ;
#2910=ORIENTED_EDGE ( 'NONE', *, *, #5531, .F. ) ;
#2911=DIRECTION ( 'NONE',  ( 0.000000000000000000, 0.000000000000000000, 1.000000000000000000 ) ) ;
#2912=VECTOR ( 'NONE', #17474, 1000.000000000000000 ) ;
#2913=ORIENTED_EDGE ( 'NONE', *, *, #33665, .T. ) ;
#2914=ORIENTED_EDGE ( 'NONE', *, *, #4748, .T. ) ;
#2915=EDGE_CURVE ( 'NONE', #34742, #20792, #18159, .T. ) ;
#2916=CARTESIAN_POINT ( 'NONE',  ( 44.99999662536849598, 60.62177826491077326, 17.49999999999999645 ) ) ;
#2918=AXIS2_PLACEMENT_3D ( 'NONE', #32451, #18407, #30015 ) ;
#2919=DIRECTION ( 'NONE',  ( 1.000000000000000000, 0.000000000000000000, 0.000000000000000000 ) ) ;
#2920=ORIENTED_EDGE ( 'NONE', *, *, #20416, .F. ) ;
#2921=CARTESIAN_POINT ( 'NONE',  ( 31.83425564451589196, 89.42901512340320380, -49.86348611802629449 ) ) ;
#2922=CIRCLE ( 'NONE', #23246, 2.000000000000001776 ) ;
#2925=VECTOR ( 'NONE', #4879, 1000.000000000000000 ) ;
#2926=ORIENTED_EDGE ( 'NONE', *, *, #15793, .F. ) ;
#2928=DIRECTION ( 'NONE',  ( 1.000000000000000000, 0.000000000000000000, 0.000000000000000000 ) ) ;
#2929=ORIENTED_EDGE ( 'NONE', *, *, #20759, .T. ) ;
#2931=CYLINDRICAL_SURFACE ( 'NONE', #37007, 1.999999999999998224 ) ;
#2932=DIRECTION ( 'NONE',  ( 1.000000000000000000, 0.000000000000000000, 0.000000000000000000 ) ) ;
#2933=DIRECTION ( 'NONE',  ( 1.000000000000000000, 0.000000000000000000, 0.000000000000000000 ) ) ;
#2934=AXIS2_PLACEMENT_3D ( 'NONE', #32823, #26625, #18389 ) ;
#2935=CARTESIAN_POINT ( 'NONE',  ( -78.00000337463094979, 17.32050807568878525, -9.999999999999998224 ) ) ;
#2936=CIRCLE ( 'NONE', #17882, 2.000000000000001776 ) ;
#2938=ORIENTED_EDGE ( 'NONE', *, *, #17116, .T. ) ;
#2940=FACE_OUTER_BOUND ( 'NONE', #24265, .T. ) ;
#2942=VERTEX_POINT ( 'NONE', #22578 ) ;
#2943=ORIENTED_EDGE ( 'NONE', *, *, #29143, .F. ) ;
#2944=AXIS2_PLACEMENT_3D ( 'NONE', #18355, #4294, #4113 ) ;
#2946=DIRECTION ( 'NONE',  ( 0.000000000000000000, 0.000000000000000000, 1.000000000000000000 ) ) ;
#2948=DIRECTION ( 'NONE',  ( 0.000000000000000000, 0.000000000000000000, 1.000000000000000000 ) ) ;
#2949=EDGE_CURVE ( 'NONE', #9993, #30809, #31328, .T. ) ;
#2951=FACE_OUTER_BOUND ( 'NONE', #7690, .T. ) ;
#2952=ORIENTED_EDGE ( 'NONE', *, *, #16444, .F. ) ;
#2953=CARTESIAN_POINT ( 'NONE',  ( -43.00331345287344931, -60.50675932581249583, -5.000000000000000000 ) ) ;
#2954=EDGE_CURVE ( 'NONE', #18222, #5353, #24761, .T. ) ;
#2955=ORIENTED_EDGE ( 'NONE', *, *, #5766, .F. ) ;
#2956=CYLINDRICAL_SURFACE ( 'NONE', #17141, 2.000000000000001776 ) ;
#2957=AXIS2_PLACEMENT_3D ( 'NONE', #2997, #5991, #17417 ) ;
#2958=EDGE_CURVE ( 'NONE', #29981, #15962, #16358, .T. ) ;
#2959=LINE ( 'NONE', #36703, #14914 ) ;
#2960=DIRECTION ( 'NONE',  ( 0.000000000000000000, 0.000000000000000000, 1.000000000000000000 ) ) ;
#2961=ORIENTED_EDGE ( 'NONE', *, *, #30807, .F. ) ;
#2963=DIRECTION ( 'NONE',  ( -1.000000000000000000, 0.000000000000000000, 0.000000000000000000 ) ) ;
#2964=AXIS2_PLACEMENT_3D ( 'NONE', #5614, #8063, #14045 ) ;
#2965=CIRCLE ( 'NONE', #32913, 2.000000000000001776 ) ;
#2966=LINE ( 'NONE', #19460, #28732 ) ;
#2968=ORIENTED_EDGE ( 'NONE', *, *, #873, .F. ) ;
#2969=DIRECTION ( 'NONE',  ( 0.000000000000000000, 0.000000000000000000, 1.000000000000000000 ) ) ;
#2970=CIRCLE ( 'NONE', #13721, 2.000000000000001776 ) ;
#2971=CARTESIAN_POINT ( 'NONE',  ( -48.00000337463109190, 69.28203230275518365, 17.49999999999999645 ) ) ;
#2973=VERTEX_POINT ( 'NONE', #31904 ) ;
#2974=EDGE_CURVE ( 'NONE', #14063, #14131, #30715, .T. ) ;
#2975=ORIENTED_EDGE ( 'NONE', *, *, #8019, .F. ) ;
#2978=VERTEX_POINT ( 'NONE', #14331 ) ;
#2979=AXIS2_PLACEMENT_3D ( 'NONE', #16101, #4460, #24340 ) ;
#2980=EDGE_CURVE ( 'NONE', #27460, #32112, #2592, .T. ) ;
#2981=DIRECTION ( 'NONE',  ( 0.000000000000000000, 0.000000000000000000, 1.000000000000000000 ) ) ;
#2983=CARTESIAN_POINT ( 'NONE',  ( -65.00000337463106348, -60.62177826491083010, 12.50000000000000000 ) ) ;
#2984=ADVANCED_FACE ( 'NONE', ( #73 ), #237, .F. ) ;
#2986=CARTESIAN_POINT ( 'NONE',  ( -14.80603122773056768, 87.83969979969874942, -49.86561046011506448 ) ) ;
#2988=CARTESIAN_POINT ( 'NONE',  ( 0.000000000000000000, 55.00000000000000000, -10.00000000000000178 ) ) ;
#2989=CIRCLE ( 'NONE', #31135, 2.000000000000001776 ) ;
#2993=AXIS2_PLACEMENT_3D ( 'NONE', #459, #94, #2928 ) ;
#2994=PLANE ( 'NONE',  #29532 ) ;
#2995=CARTESIAN_POINT ( 'NONE',  ( -90.00000337463090716, -1.040834085586084257E-14, 12.50000000000000000 ) ) ;
#2997=CARTESIAN_POINT ( 'NONE',  ( 27.78182860042856461, 56.67878100130339902, -4.999999999999997335 ) ) ;
#2998=EDGE_LOOP ( 'NONE', ( #2043, #15950, #27792, #21738 ) ) ;
#2999=ADVANCED_FACE ( 'NONE', ( #20869 ), #9983, .F. ) ;
#3000=FACE_BOUND ( 'NONE', #18631, .T. ) ;
#3002=VERTEX_POINT ( 'NONE', #4359 ) ;
#3003=LINE ( 'NONE', #5809, #36811 ) ;
#3004=ORIENTED_EDGE ( 'NONE', *, *, #249, .F. ) ;
#3006=DIRECTION ( 'NONE',  ( 0.000000000000000000, 0.000000000000000000, 1.000000000000000000 ) ) ;
#3008=CIRCLE ( 'NONE', #36531, 2.000000000000001776 ) ;
#3009=EDGE_LOOP ( 'NONE', ( #33677, #13074 ) ) ;
#3010=ORIENTED_EDGE ( 'NONE', *, *, #27990, .F. ) ;
#3011=CIRCLE ( 'NONE', #13205, 2.000000000000001776 ) ;
#3012=ORIENTED_EDGE ( 'NONE', *, *, #31052, .F. ) ;
#3014=ADVANCED_FACE ( 'NONE', ( #26672 ), #23675, .F. ) ;
#3015=EDGE_LOOP ( 'NONE', ( #9068, #21045 ) ) ;
#3016=CARTESIAN_POINT ( 'NONE',  ( 82.99999662536831124, -8.660254037844397956, -9.999999999999998224 ) ) ;
#3017=AXIS2_PLACEMENT_3D ( 'NONE', #29391, #6883, #12114 ) ;
#3018=CYLINDRICAL_SURFACE ( 'NONE', #17385, 3.000000000000006217 ) ;
#3021=DIRECTION ( 'NONE',  ( 1.000000000000000000, 0.000000000000000000, 0.000000000000000000 ) ) ;
#3022=CARTESIAN_POINT ( 'NONE',  ( -3.499999999999991562, -55.00000000000000000, -10.00000000000000000 ) ) ;
#3023=DIRECTION ( 'NONE',  ( 1.000000000000000000, 0.000000000000000000, 0.000000000000000000 ) ) ;
#3024=ORIENTED_EDGE ( 'NONE', *, *, #1396, .T. ) ;
#3027=EDGE_CURVE ( 'NONE', #8351, #15508, #29304, .T. ) ;
#3028=DIRECTION ( 'NONE',  ( -1.000000000000000000, 0.000000000000000000, 0.000000000000000000 ) ) ;
#3030=EDGE_LOOP ( 'NONE', ( #30592, #21771, #3521, #11712 ) ) ;
#3031=VECTOR ( 'NONE', #32655, 1000.000000000000000 ) ;
#3032=CYLINDRICAL_SURFACE ( 'NONE', #31620, 2.000000000000001776 ) ;
#3033=EDGE_CURVE ( 'NONE', #29904, #18462, #28912, .T. ) ;
#3036=ORIENTED_EDGE ( 'NONE', *, *, #10642, .F. ) ;
#3038=CARTESIAN_POINT ( 'NONE',  ( 59.99999662536843914, -34.64101615137759893, 17.49999999999999645 ) ) ;
#3039=CARTESIAN_POINT ( 'NONE',  ( 21.99999662536857770, 86.60254037844397601, 12.50000000000000000 ) ) ;
#3040=CIRCLE ( 'NONE', #6032, 2.000000000000001776 ) ;
#3042=DIRECTION ( 'NONE',  ( 0.000000000000000000, 0.000000000000000000, 1.000000000000000000 ) ) ;
#3043=VERTEX_POINT ( 'NONE', #12775 ) ;
#3044=ORIENTED_EDGE ( 'NONE', *, *, #31062, .F. ) ;
#3045=EDGE_CURVE ( 'NONE', #6546, #20763, #32868, .T. ) ;
#3046=DIRECTION ( 'NONE',  ( 0.000000000000000000, 0.000000000000000000, 1.000000000000000000 ) ) ;
#3048=EDGE_CURVE ( 'NONE', #26912, #20671, #22370, .T. ) ;
#3050=ADVANCED_FACE ( 'NONE', ( #9231 ), #32303, .F. ) ;
#3051=VERTEX_POINT ( 'NONE', #30039 ) ;
#3052=EDGE_CURVE ( 'NONE', #30350, #1819, #6197, .T. ) ;
#3054=EDGE_LOOP ( 'NONE', ( #116, #12528, #22839, #23482 ) ) ;
#3055=ORIENTED_EDGE ( 'NONE', *, *, #32137, .F. ) ;
#3056=CARTESIAN_POINT ( 'NONE',  ( -25.00000337463121980, -77.94228634059963667, 12.50000000000000000 ) ) ;
#3058=ORIENTED_EDGE ( 'NONE', *, *, #16911, .T. ) ;
#3060=CARTESIAN_POINT ( 'NONE',  ( -2.000003374631289521, -69.28203230275519786, -9.999999999999998224 ) ) ;
#3061=CARTESIAN_POINT ( 'NONE',  ( 49.99999662536846756, -69.28203230275519786, 17.49999999999999645 ) ) ;
#3063=VERTEX_POINT ( 'NONE', #15229 ) ;
#3064=CARTESIAN_POINT ( 'NONE',  ( 79.99999662536833966, 17.32050807568879236, 12.50000000000000000 ) ) ;
#3065=AXIS2_PLACEMENT_3D ( 'NONE', #7485, #8034, #33919 ) ;
#3066=FACE_BOUND ( 'NONE', #20042, .T. ) ;
#3068=FACE_OUTER_BOUND ( 'NONE', #29152, .T. ) ;
#3069=CARTESIAN_POINT ( 'NONE',  ( 44.99999662536849598, -77.94228634059960825, -9.999999999999998224 ) ) ;
#3071=DIRECTION ( 'NONE',  ( 1.000000000000000000, 0.000000000000000000, 0.000000000000000000 ) ) ;
#3072=CARTESIAN_POINT ( 'NONE',  ( -58.48108235278846934, -36.97203788309006001, 12.49999999999999645 ) ) ;
#3073=EDGE_LOOP ( 'NONE', ( #17456, #12380, #2145, #18604 ) ) ;
#3074=DIRECTION ( 'NONE',  ( 0.000000000000000000, 0.000000000000000000, 1.000000000000000000 ) ) ;
#3076=DIRECTION ( 'NONE',  ( 0.000000000000000000, 0.000000000000000000, 1.000000000000000000 ) ) ;
#3077=ORIENTED_EDGE ( 'NONE', *, *, #30519, .F. ) ;
#3079=ORIENTED_EDGE ( 'NONE', *, *, #4809, .T. ) ;
#3080=CARTESIAN_POINT ( 'NONE',  ( 9.999996625368625658, 86.60254037844397601, -9.999999999999998224 ) ) ;
#3081=DIRECTION ( 'NONE',  ( 1.000000000000000000, 0.000000000000000000, 0.000000000000000000 ) ) ;
#3082=DIRECTION ( 'NONE',  ( 1.000000000000000000, 0.000000000000000000, 0.000000000000000000 ) ) ;
#3083=ORIENTED_EDGE ( 'NONE', *, *, #14865, .T. ) ;
#3084=DIRECTION ( 'NONE',  ( -1.000000000000000000, 0.000000000000000000, 0.000000000000000000 ) ) ;
#3085=VERTEX_POINT ( 'NONE', #12037 ) ;
#3086=ADVANCED_FACE ( 'NONE', ( #23495 ), #32100, .F. ) ;
#3087=DIRECTION ( 'NONE',  ( 0.000000000000000000, 0.000000000000000000, 1.000000000000000000 ) ) ;
#3088=ORIENTED_EDGE ( 'NONE', *, *, #20087, .F. ) ;
#3090=EDGE_LOOP ( 'NONE', ( #28997, #6446, #27276, #35613 ) ) ;
#3091=ORIENTED_EDGE ( 'NONE', *, *, #22663, .F. ) ;
#3092=DIRECTION ( 'NONE',  ( 0.000000000000000000, 0.000000000000000000, 1.000000000000000000 ) ) ;
#3093=CARTESIAN_POINT ( 'NONE',  ( 19.99999662536858835, 69.28203230275516944, -9.999999999999998224 ) ) ;
#3095=VERTEX_POINT ( 'NONE', #17875 ) ;
#3096=CARTESIAN_POINT ( 'NONE',  ( 21.99999662536862033, -86.60254037844400443, -9.999999999999998224 ) ) ;
#3097=DIRECTION ( 'NONE',  ( 0.000000000000000000, 0.000000000000000000, 1.000000000000000000 ) ) ;
#3099=ORIENTED_EDGE ( 'NONE', *, *, #14997, .F. ) ;
#3100=LINE ( 'NONE', #650, #5161 ) ;
#3102=AXIS2_PLACEMENT_3D ( 'NONE', #35158, #6644, #12626 ) ;
#3103=ORIENTED_EDGE ( 'NONE', *, *, #2827, .T. ) ;
#3104=CYLINDRICAL_SURFACE ( 'NONE', #24427, 2.000000000000000000 ) ;
#3105=DIRECTION ( 'NONE',  ( 0.000000000000000000, 0.000000000000000000, 1.000000000000000000 ) ) ;
#3107=EDGE_CURVE ( 'NONE', #17753, #29194, #9784, .T. ) ;
#3108=EDGE_CURVE ( 'NONE', #9038, #22407, #2616, .T. ) ;
#3109=CARTESIAN_POINT ( 'NONE',  ( 72.99999662536836809, 25.98076211353319565, -9.999999999999998224 ) ) ;
#3111=LINE ( 'NONE', #12452, #34095 ) ;
#3112=EDGE_LOOP ( 'NONE', ( #16665, #3669, #14434, #31474, #12126 ) ) ;
#3113=CARTESIAN_POINT ( 'NONE',  ( 79.99999662536833966, -3.469446951953614189E-15, -9.999999999999998224 ) ) ;
#3114=DIRECTION ( 'NONE',  ( 0.000000000000000000, 0.000000000000000000, 1.000000000000000000 ) ) ;
#3115=ORIENTED_EDGE ( 'NONE', *, *, #3137, .T. ) ;
#3116=ADVANCED_FACE ( 'NONE', ( #24058 ), #35501, .F. ) ;
#3117=EDGE_LOOP ( 'NONE', ( #1931, #25655, #439, #24884, #18028 ) ) ;
#3118=VERTEX_POINT ( 'NONE', #16354 ) ;
#3120=CARTESIAN_POINT ( 'NONE',  ( 46.99999662536849598, 60.62177826491077326, -5.000000000000000000 ) ) ;
#3121=CARTESIAN_POINT ( 'NONE',  ( -22.00000337463124112, 69.28203230275516944, -9.999999999999998224 ) ) ;
#3122=AXIS2_PLACEMENT_3D ( 'NONE', #13159, #35858, #21408 ) ;
#3123=CARTESIAN_POINT ( 'NONE',  ( -10.21421600225141724, -84.61404523131187716, -5.000000000000000000 ) ) ;
#3126=CARTESIAN_POINT ( 'NONE',  ( -82.00000337463094979, 17.32050807568878525, -9.999999999999998224 ) ) ;
#3127=VERTEX_POINT ( 'NONE', #13730 ) ;
#3128=FACE_BOUND ( 'NONE', #6857, .T. ) ;
#3129=CARTESIAN_POINT ( 'NONE',  ( -75.00000337463100664, -43.30127018922202353, 12.50000000000000000 ) ) ;
#3131=CARTESIAN_POINT ( 'NONE',  ( 74.99999662536835388, -43.30127018922199511, 12.50000000000000000 ) ) ;
#3133=DIRECTION ( 'NONE',  ( 1.000000000000000000, 0.000000000000000000, 0.000000000000000000 ) ) ;
#3134=CIRCLE ( 'NONE', #22915, 2.000000000000001776 ) ;
#3135=CARTESIAN_POINT ( 'NONE',  ( -53.00000337463106348, 43.30127018922197379, -9.999999999999998224 ) ) ;
#3136=CARTESIAN_POINT ( 'NONE',  ( 61.06482292022109704, -72.77422209630303485, -5.000000000000000000 ) ) ;
#3137=EDGE_CURVE ( 'NONE', #36216, #9400, #12770, .T. ) ;
#3140=DIRECTION ( 'NONE',  ( 0.000000000000000000, 0.000000000000000000, -1.000000000000000000 ) ) ;
#3141=DIRECTION ( 'NONE',  ( 1.000000000000000000, 0.000000000000000000, 0.000000000000000000 ) ) ;
#3143=EDGE_LOOP ( 'NONE', ( #16788, #5054 ) ) ;
#3144=VECTOR ( 'NONE', #23613, 1000.000000000000000 ) ;
#3145=ORIENTED_EDGE ( 'NONE', *, *, #15609, .T. ) ;
#3146=EDGE_CURVE ( 'NONE', #695, #17257, #27150, .T. ) ;
#3147=DIRECTION ( 'NONE',  ( 3.491481338843133355E-15, 1.000000000000000000, 0.000000000000000000 ) ) ;
#3148=ADVANCED_FACE ( 'NONE', ( #36055 ), #16184, .T. ) ;
#3149=DIRECTION ( 'NONE',  ( -1.000000000000000000, 0.000000000000000000, 0.000000000000000000 ) ) ;
#3150=DIRECTION ( 'NONE',  ( 0.000000000000000000, 0.000000000000000000, 1.000000000000000000 ) ) ;
#3151=DIRECTION ( 'NONE',  ( 0.000000000000000000, 0.000000000000000000, -1.000000000000000000 ) ) ;
#3152=CARTESIAN_POINT ( 'NONE',  ( -37.00000337463116296, 60.62177826491077326, -9.999999999999998224 ) ) ;
#3153=ORIENTED_EDGE ( 'NONE', *, *, #22779, .F. ) ;
#3155=CIRCLE ( 'NONE', #15140, 2.000000000000001776 ) ;
#3156=CARTESIAN_POINT ( 'NONE',  ( 47.99999662536848177, -51.96152422706640550, 17.49999999999999645 ) ) ;
#3158=FACE_OUTER_BOUND ( 'NONE', #23959, .T. ) ;
#3159=VERTEX_POINT ( 'NONE', #10186 ) ;
#3162=EDGE_LOOP ( 'NONE', ( #10503, #25222, #32784, #8227 ) ) ;
#3163=CIRCLE ( 'NONE', #31885, 3.000000000000008882 ) ;
#3164=ORIENTED_EDGE ( 'NONE', *, *, #31640, .F. ) ;
#3166=CARTESIAN_POINT ( 'NONE',  ( -77.00000337463097821, 43.30127018922197379, 12.50000000000000000 ) ) ;
#3169=ADVANCED_FACE ( 'NONE', ( #8097 ), #18991, .F. ) ;
#3170=CARTESIAN_POINT ( 'NONE',  ( 44.99999662536851019, -60.62177826491080168, -9.999999999999998224 ) ) ;
#3171=CYLINDRICAL_SURFACE ( 'NONE', #4713, 2.000000000000001776 ) ;
#3173=ORIENTED_EDGE ( 'NONE', *, *, #3048, .T. ) ;
#3175=ORIENTED_EDGE ( 'NONE', *, *, #18253, .T. ) ;
#3177=ORIENTED_EDGE ( 'NONE', *, *, #36558, .F. ) ;
#3179=ORIENTED_EDGE ( 'NONE', *, *, #31846, .F. ) ;
#3180=DIRECTION ( 'NONE',  ( 0.000000000000000000, 0.000000000000000000, 1.000000000000000000 ) ) ;
#3182=CYLINDRICAL_SURFACE ( 'NONE', #11857, 2.000000000000000000 ) ;
#3183=DIRECTION ( 'NONE',  ( 0.000000000000000000, 0.000000000000000000, -1.000000000000000000 ) ) ;
#3184=DIRECTION ( 'NONE',  ( 0.000000000000000000, 0.000000000000000000, -1.000000000000000000 ) ) ;
#3185=ORIENTED_EDGE ( 'NONE', *, *, #20789, .F. ) ;
#3187=DIRECTION ( 'NONE',  ( 0.000000000000000000, 0.000000000000000000, 1.000000000000000000 ) ) ;
#3189=AXIS2_PLACEMENT_3D ( 'NONE', #5345, #28192, #10773 ) ;
#3192=DIRECTION ( 'NONE',  ( 0.000000000000000000, 0.000000000000000000, 1.000000000000000000 ) ) ;
#3193=DIRECTION ( 'NONE',  ( 1.000000000000000000, 0.000000000000000000, 0.000000000000000000 ) ) ;
#3194=EDGE_LOOP ( 'NONE', ( #2337, #34005, #15980, #817 ) ) ;
#3195=ORIENTED_EDGE ( 'NONE', *, *, #4704, .T. ) ;
#3197=DIRECTION ( 'NONE',  ( -1.000000000000000000, 0.000000000000000000, 0.000000000000000000 ) ) ;
#3199=CARTESIAN_POINT ( 'NONE',  ( 0.000000000000000000, 0.000000000000000000, -5.000000000000000000 ) ) ;
#3200=ORIENTED_EDGE ( 'NONE', *, *, #18319, .T. ) ;
#3201=AXIS2_PLACEMENT_3D ( 'NONE', #27421, #11082, #25730 ) ;
#3202=DIRECTION ( 'NONE',  ( 1.000000000000000000, 0.000000000000000000, 0.000000000000000000 ) ) ;
#3203=LINE ( 'NONE', #387, #28521 ) ;
#3204=CARTESIAN_POINT ( 'NONE',  ( -55.88972745734202618, -33.99999999999965894, 12.49999999999999822 ) ) ;
#3205=AXIS2_PLACEMENT_3D ( 'NONE', #13860, #7882, #24943 ) ;
#3209=CARTESIAN_POINT ( 'NONE',  ( 62.99999662536839651, -60.62177826491080168, -9.999999999999998224 ) ) ;
#3212=VECTOR ( 'NONE', #18504, 1000.000000000000000 ) ;
#3213=EDGE_CURVE ( 'NONE', #36127, #20281, #24432, .T. ) ;
#3214=LINE ( 'NONE', #23289, #29559 ) ;
#3215=AXIS2_PLACEMENT_3D ( 'NONE', #33415, #7908, #1524 ) ;
#3216=DIRECTION ( 'NONE',  ( 0.000000000000000000, 0.000000000000000000, 1.000000000000000000 ) ) ;
#3219=EDGE_CURVE ( 'NONE', #23390, #21452, #21160, .T. ) ;
#3220=DIRECTION ( 'NONE',  ( 0.000000000000000000, 0.000000000000000000, -1.000000000000000000 ) ) ;
#3221=EDGE_CURVE ( 'NONE', #20810, #14063, #5003, .T. ) ;
#3222=CIRCLE ( 'NONE', #18180, 2.000000000000001776 ) ;
#3223=DIRECTION ( 'NONE',  ( 1.000000000000000000, 0.000000000000000000, 0.000000000000000000 ) ) ;
#3224=DIRECTION ( 'NONE',  ( 1.000000000000000000, 0.000000000000000000, 0.000000000000000000 ) ) ;
#3225=EDGE_LOOP ( 'NONE', ( #35673, #24923, #9340, #11117 ) ) ;
#3226=DIRECTION ( 'NONE',  ( 0.000000000000000000, 0.000000000000000000, 1.000000000000000000 ) ) ;
#3227=FACE_BOUND ( 'NONE', #35804, .T. ) ;
#3228=DIRECTION ( 'NONE',  ( 1.000000000000000000, 0.000000000000000000, 0.000000000000000000 ) ) ;
#3230=FACE_OUTER_BOUND ( 'NONE', #22273, .T. ) ;
#3231=EDGE_CURVE ( 'NONE', #3360, #29817, #17084, .T. ) ;
#3232=CARTESIAN_POINT ( 'NONE',  ( 7.999996625368656744, -86.60254037844400443, -5.000000000000000000 ) ) ;
#3234=AXIS2_PLACEMENT_3D ( 'NONE', #1081, #12507, #21693 ) ;
#3235=FACE_OUTER_BOUND ( 'NONE', #14571, .T. ) ;
#3236=EDGE_CURVE ( 'NONE', #29323, #29299, #28826, .T. ) ;
#3237=EDGE_CURVE ( 'NONE', #24381, #26240, #35447, .T. ) ;
#3238=CARTESIAN_POINT ( 'NONE',  ( 69.99999662536838230, -51.96152422706639840, 17.49999999999999645 ) ) ;
#3239=EDGE_LOOP ( 'NONE', ( #14781, #30688 ) ) ;
#3240=EDGE_CURVE ( 'NONE', #33684, #32017, #11282, .T. ) ;
#3243=DIRECTION ( 'NONE',  ( 0.000000000000000000, 0.000000000000000000, 1.000000000000000000 ) ) ;
#3244=AXIS2_PLACEMENT_3D ( 'NONE', #36753, #36584, #7892 ) ;
#3245=ORIENTED_EDGE ( 'NONE', *, *, #27611, .T. ) ;
#3247=ORIENTED_EDGE ( 'NONE', *, *, #32470, .F. ) ;
#3249=DIRECTION ( 'NONE',  ( 0.000000000000000000, 0.000000000000000000, -1.000000000000000000 ) ) ;
#3251=CYLINDRICAL_SURFACE ( 'NONE', #25031, 2.000000000000001776 ) ;
#3252=VERTEX_POINT ( 'NONE', #20442 ) ;
#3257=ORIENTED_EDGE ( 'NONE', *, *, #28542, .T. ) ;
#3259=EDGE_LOOP ( 'NONE', ( #28821, #10348 ) ) ;
#3260=ORIENTED_EDGE ( 'NONE', *, *, #35132, .F. ) ;
#3261=AXIS2_PLACEMENT_3D ( 'NONE', #29911, #13726, #27773 ) ;
#3263=CARTESIAN_POINT ( 'NONE',  ( 59.99999662536842493, 51.96152422706639129, 17.49999999999999645 ) ) ;
#3264=ORIENTED_EDGE ( 'NONE', *, *, #26845, .T. ) ;
#3265=CARTESIAN_POINT ( 'NONE',  ( 49.99999662536848177, -51.96152422706640550, -9.999999999999998224 ) ) ;
#3266=CIRCLE ( 'NONE', #24221, 2.000000000000000000 ) ;
#3268=DIRECTION ( 'NONE',  ( 0.000000000000000000, 0.000000000000000000, 1.000000000000000000 ) ) ;
#3270=AXIS2_PLACEMENT_3D ( 'NONE', #27491, #33299, #24685 ) ;
#3271=DIRECTION ( 'NONE',  ( 0.000000000000000000, 0.000000000000000000, 1.000000000000000000 ) ) ;
#3272=LINE ( 'NONE', #14707, #20967 ) ;
#3273=ORIENTED_EDGE ( 'NONE', *, *, #3350, .T. ) ;
#3274=CYLINDRICAL_SURFACE ( 'NONE', #34601, 2.000000000000001776 ) ;
#3275=CARTESIAN_POINT ( 'NONE',  ( 51.99999662536848888, -51.96152422706640550, -5.000000000000000000 ) ) ;
#3276=CYLINDRICAL_SURFACE ( 'NONE', #18962, 3.000000000000002665 ) ;
#3277=CARTESIAN_POINT ( 'NONE',  ( -56.52018970185233826, 35.83991598322119643, -4.999999999999997335 ) ) ;
#3278=EDGE_CURVE ( 'NONE', #23804, #31278, #34841, .T. ) ;
#3279=DIRECTION ( 'NONE',  ( 1.000000000000000000, 0.000000000000000000, 0.000000000000000000 ) ) ;
#3280=AXIS2_PLACEMENT_3D ( 'NONE', #34999, #32373, #14557 ) ;
#3282=ORIENTED_EDGE ( 'NONE', *, *, #19239, .F. ) ;
#3283=CARTESIAN_POINT ( 'NONE',  ( -25.00000337463120914, 77.94228634059957983, -9.999999999999998224 ) ) ;
#3284=CIRCLE ( 'NONE', #24845, 2.000000000000000000 ) ;
#3285=DIRECTION ( 'NONE',  ( -0.8660254037844383745, 0.5000000000000005551, 0.000000000000000000 ) ) ;
#3286=DIRECTION ( 'NONE',  ( -0.000000000000000000, 0.000000000000000000, -1.000000000000000000 ) ) ;
#3287=VERTEX_POINT ( 'NONE', #34175 ) ;
#3288=VECTOR ( 'NONE', #18584, 1000.000000000000000 ) ;
#3289=ORIENTED_EDGE ( 'NONE', *, *, #20583, .F. ) ;
#3290=ORIENTED_EDGE ( 'NONE', *, *, #3240, .F. ) ;
#3292=DIRECTION ( 'NONE',  ( -1.000000000000000000, 0.000000000000000000, 0.000000000000000000 ) ) ;
#3293=DIRECTION ( 'NONE',  ( 0.000000000000000000, 0.000000000000000000, 1.000000000000000000 ) ) ;
#3294=CIRCLE ( 'NONE', #6290, 2.000000000000000000 ) ;
#3295=CIRCLE ( 'NONE', #4510, 65.00000000000000000 ) ;
#3296=DIRECTION ( 'NONE',  ( -0.000000000000000000, -0.000000000000000000, -1.000000000000000000 ) ) ;
#3297=ORIENTED_EDGE ( 'NONE', *, *, #35692, .F. ) ;
#3298=DIRECTION ( 'NONE',  ( 0.000000000000000000, 0.000000000000000000, 1.000000000000000000 ) ) ;
#3299=ORIENTED_EDGE ( 'NONE', *, *, #31791, .T. ) ;
#3300=FACE_BOUND ( 'NONE', #27954, .T. ) ;
#3301=EDGE_CURVE ( 'NONE', #15339, #11692, #31814, .T. ) ;
#3302=CARTESIAN_POINT ( 'NONE',  ( -27.00000337463121625, -77.94228634059963667, -9.999999999999998224 ) ) ;
#3303=CIRCLE ( 'NONE', #21882, 2.000000000000001776 ) ;
#3304=DIRECTION ( 'NONE',  ( 1.000000000000000000, 0.000000000000000000, 0.000000000000000000 ) ) ;
#3305=AXIS2_PLACEMENT_3D ( 'NONE', #3479, #23917, #15469 ) ;
#3307=DIRECTION ( 'NONE',  ( 0.000000000000000000, 0.000000000000000000, -1.000000000000000000 ) ) ;
#3308=AXIS2_PLACEMENT_3D ( 'NONE', #36235, #25352, #16359 ) ;
#3310=AXIS2_PLACEMENT_3D ( 'NONE', #28071, #5203, #30687 ) ;
#3311=CIRCLE ( 'NONE', #16485, 2.000000000000001776 ) ;
#3312=CARTESIAN_POINT ( 'NONE',  ( 66.99999662536841072, -25.98076211353320275, 12.50000000000000000 ) ) ;
#3315=DIRECTION ( 'NONE',  ( -1.051347561198064495E-14, -1.000000000000000000, 0.000000000000000000 ) ) ;
#3316=ORIENTED_EDGE ( 'NONE', *, *, #15234, .F. ) ;
#3317=DIRECTION ( 'NONE',  ( 1.000000000000000000, 0.000000000000000000, 0.000000000000000000 ) ) ;
#3319=CIRCLE ( 'NONE', #35099, 2.000000000000001776 ) ;
#3320=DIRECTION ( 'NONE',  ( 0.000000000000000000, 0.000000000000000000, 1.000000000000000000 ) ) ;
#3322=AXIS2_PLACEMENT_3D ( 'NONE', #14632, #5851, #3202 ) ;
#3323=ORIENTED_EDGE ( 'NONE', *, *, #437, .T. ) ;
#3325=EDGE_CURVE ( 'NONE', #10822, #16313, #6097, .T. ) ;
#3326=ORIENTED_EDGE ( 'NONE', *, *, #12201, .F. ) ;
#3327=CARTESIAN_POINT ( 'NONE',  ( 69.13212189986965939, 2.778182860042805125, -4.999999999999997335 ) ) ;
#3328=DIRECTION ( 'NONE',  ( 1.000000000000000000, 0.000000000000000000, -0.000000000000000000 ) ) ;
#3329=CIRCLE ( 'NONE', #18919, 2.000000000000001776 ) ;
#3330=CARTESIAN_POINT ( 'NONE',  ( -22.00000337463122690, 86.60254037844397601, -9.999999999999998224 ) ) ;
#3332=AXIS2_PLACEMENT_3D ( 'NONE', #23108, #29461, #15045 ) ;
#3333=DIRECTION ( 'NONE',  ( 1.000000000000000000, 0.000000000000000000, 0.000000000000000000 ) ) ;
#3334=AXIS2_PLACEMENT_3D ( 'NONE', #18322, #35589, #21133 ) ;
#3336=CARTESIAN_POINT ( 'NONE',  ( -56.67878100130369035, 27.78182860042797131, 12.49999999999999822 ) ) ;
#3339=VERTEX_POINT ( 'NONE', #26075 ) ;
#3340=CARTESIAN_POINT ( 'NONE',  ( -5.000003374631307729, 77.94228634059957983, -9.999999999999998224 ) ) ;
#3341=EDGE_CURVE ( 'NONE', #792, #36127, #4902, .T. ) ;
#3342=DIRECTION ( 'NONE',  ( 0.000000000000000000, 0.000000000000000000, -1.000000000000000000 ) ) ;
#3343=DIRECTION ( 'NONE',  ( -1.000000000000000000, 0.000000000000000000, 0.000000000000000000 ) ) ;
#3344=ORIENTED_EDGE ( 'NONE', *, *, #14200, .F. ) ;
#3345=EDGE_CURVE ( 'NONE', #33803, #22230, #5645, .T. ) ;
#3346=AXIS2_PLACEMENT_3D ( 'NONE', #27136, #36342, #36149 ) ;
#3347=FACE_OUTER_BOUND ( 'NONE', #20210, .T. ) ;
#3348=ORIENTED_EDGE ( 'NONE', *, *, #1825, .F. ) ;
#3349=ORIENTED_EDGE ( 'NONE', *, *, #21588, .F. ) ;
#3350=EDGE_CURVE ( 'NONE', #14947, #35287, #13877, .T. ) ;
#3351=CARTESIAN_POINT ( 'NONE',  ( -25.00000337463120914, 77.94228634059957983, 12.50000000000000000 ) ) ;
#3352=ORIENTED_EDGE ( 'NONE', *, *, #14752, .T. ) ;
#3354=AXIS2_PLACEMENT_3D ( 'NONE', #13364, #22009, #18827 ) ;
#3357=VECTOR ( 'NONE', #17271, 1000.000000000000000 ) ;
#3359=ORIENTED_EDGE ( 'NONE', *, *, #36714, .F. ) ;
#3360=VERTEX_POINT ( 'NONE', #34339 ) ;
#3361=CIRCLE ( 'NONE', #15351, 2.000000000000001776 ) ;
#3363=EDGE_LOOP ( 'NONE', ( #25159, #14521, #17445, #32150 ) ) ;
#3364=AXIS2_PLACEMENT_3D ( 'NONE', #21386, #15946, #1497 ) ;
#3365=AXIS2_PLACEMENT_3D ( 'NONE', #24268, #21469, #32907 ) ;
#3366=ORIENTED_EDGE ( 'NONE', *, *, #1618, .T. ) ;
#3367=CIRCLE ( 'NONE', #960, 2.000000000000001776 ) ;
#3368=ORIENTED_EDGE ( 'NONE', *, *, #5978, .T. ) ;
#3369=DIRECTION ( 'NONE',  ( 1.000000000000000000, 0.000000000000000000, 0.000000000000000000 ) ) ;
#3371=CARTESIAN_POINT ( 'NONE',  ( 39.99999662536853151, -69.28203230275519786, 12.50000000000000000 ) ) ;
#3372=ORIENTED_EDGE ( 'NONE', *, *, #25765, .F. ) ;
#3373=CARTESIAN_POINT ( 'NONE',  ( -80.00000337463096400, -34.64101615137762025, -9.999999999999998224 ) ) ;
#3375=CARTESIAN_POINT ( 'NONE',  ( -45.00000337463111322, -77.94228634059960825, -9.999999999999998224 ) ) ;
#3376=EDGE_LOOP ( 'NONE', ( #9996, #17506 ) ) ;
#3377=LINE ( 'NONE', #6021, #17032 ) ;
#3379=ADVANCED_FACE ( 'NONE', ( #23832 ), #9186, .T. ) ;
#3380=CARTESIAN_POINT ( 'NONE',  ( 64.99999662536842493, 43.30127018922200222, 12.50000000000000000 ) ) ;
#3382=ORIENTED_EDGE ( 'NONE', *, *, #14250, .F. ) ;
#3383=CARTESIAN_POINT ( 'NONE',  ( -89.42901512340354486, 31.83425564451495404, 12.49999999999999822 ) ) ;
#3384=DIRECTION ( 'NONE',  ( 1.000000000000000000, 0.000000000000000000, 0.000000000000000000 ) ) ;
#3385=VERTEX_POINT ( 'NONE', #35636 ) ;
#3386=CIRCLE ( 'NONE', #24349, 95.00000000000000000 ) ;
#3387=EDGE_CURVE ( 'NONE', #34182, #4700, #23464, .T. ) ;
#3388=VERTEX_POINT ( 'NONE', #9938 ) ;
#3390=EDGE_CURVE ( 'NONE', #30431, #35240, #21051, .T. ) ;
#3391=CARTESIAN_POINT ( 'NONE',  ( -63.00000337463104927, -43.30127018922202353, -5.000000000000000000 ) ) ;
#3392=DIRECTION ( 'NONE',  ( 1.000000000000000000, 0.000000000000000000, 0.000000000000000000 ) ) ;
#3393=DIRECTION ( 'NONE',  ( 1.000000000000000000, 0.000000000000000000, 0.000000000000000000 ) ) ;
#3395=EDGE_LOOP ( 'NONE', ( #7115, #36322, #33273, #20770 ) ) ;
#3397=CIRCLE ( 'NONE', #35155, 2.000000000000001776 ) ;
#3398=CARTESIAN_POINT ( 'NONE',  ( -60.00000337463108480, -51.96152422706641971, -9.999999999999998224 ) ) ;
#3401=AXIS2_PLACEMENT_3D ( 'NONE', #10898, #33978, #11275 ) ;
#3402=DIRECTION ( 'NONE',  ( 1.000000000000000000, 0.000000000000000000, 0.000000000000000000 ) ) ;
#3403=CIRCLE ( 'NONE', #32126, 2.000000000000001776 ) ;
#3405=EDGE_CURVE ( 'NONE', #18237, #11435, #98, .T. ) ;
#3406=DIRECTION ( 'NONE',  ( 0.000000000000000000, 0.000000000000000000, 1.000000000000000000 ) ) ;
#3407=ORIENTED_EDGE ( 'NONE', *, *, #14229, .F. ) ;
#3408=DIRECTION ( 'NONE',  ( 1.000000000000000000, 0.000000000000000000, 0.000000000000000000 ) ) ;
#3409=DIRECTION ( 'NONE',  ( -1.000000000000000000, 0.000000000000000000, 0.000000000000000000 ) ) ;
#3410=EDGE_CURVE ( 'NONE', #17105, #7306, #20450, .T. ) ;
#3412=ORIENTED_EDGE ( 'NONE', *, *, #6554, .F. ) ;
#3413=ORIENTED_EDGE ( 'NONE', *, *, #6964, .T. ) ;
#3414=DIRECTION ( 'NONE',  ( 0.000000000000000000, 0.000000000000000000, 1.000000000000000000 ) ) ;
#3416=FACE_OUTER_BOUND ( 'NONE', #14902, .T. ) ;
#3418=VECTOR ( 'NONE', #15474, 1000.000000000000000 ) ;
#3419=EDGE_LOOP ( 'NONE', ( #4535, #9732 ) ) ;
#3420=DIRECTION ( 'NONE',  ( 0.000000000000000000, 0.000000000000000000, -1.000000000000000000 ) ) ;
#3422=FACE_BOUND ( 'NONE', #10202, .T. ) ;
#3424=CYLINDRICAL_SURFACE ( 'NONE', #35230, 2.000000000000000000 ) ;
#3426=CARTESIAN_POINT ( 'NONE',  ( -45.00000337463111322, -77.94228634059960825, -9.999999999999998224 ) ) ;
#3428=DIRECTION ( 'NONE',  ( 0.000000000000000000, 0.000000000000000000, -1.000000000000000000 ) ) ;
#3430=EDGE_CURVE ( 'NONE', #14001, #27785, #7303, .T. ) ;
#3433=CARTESIAN_POINT ( 'NONE',  ( 56.56138580058825482, 61.87160379013676703, -5.000000000000000000 ) ) ;
#3434=CARTESIAN_POINT ( 'NONE',  ( 32.99999662536855283, -60.62177826491080168, -9.999999999999998224 ) ) ;
#3435=CARTESIAN_POINT ( 'NONE',  ( 52.99999662536844625, -60.62177826491080168, -9.999999999999998224 ) ) ;
#3436=AXIS2_PLACEMENT_3D ( 'NONE', #32548, #33110, #10422 ) ;
#3437=ORIENTED_EDGE ( 'NONE', *, *, #34374, .F. ) ;
#3438=AXIS2_PLACEMENT_3D ( 'NONE', #19153, #22314, #2615 ) ;
#3439=EDGE_CURVE ( 'NONE', #29585, #11539, #32439, .T. ) ;
#3440=EDGE_LOOP ( 'NONE', ( #23350, #21801 ) ) ;
#3441=ORIENTED_EDGE ( 'NONE', *, *, #32369, .T. ) ;
#3442=ADVANCED_FACE ( 'NONE', ( #14829 ), #35285, .F. ) ;
#3444=CARTESIAN_POINT ( 'NONE',  ( 12.99999662536863632, -77.94228634059960825, 17.49999999999999645 ) ) ;
#3445=EDGE_CURVE ( 'NONE', #12415, #35643, #686, .T. ) ;
#3447=VERTEX_POINT ( 'NONE', #18185 ) ;
#3449=VECTOR ( 'NONE', #17851, 1000.000000000000000 ) ;
#3450=CIRCLE ( 'NONE', #10031, 2.000000000000001776 ) ;
#3451=DIRECTION ( 'NONE',  ( 0.000000000000000000, 0.000000000000000000, -1.000000000000000000 ) ) ;
#3452=CIRCLE ( 'NONE', #31019, 2.000000000000001776 ) ;
#3456=FACE_OUTER_BOUND ( 'NONE', #5639, .T. ) ;
#3458=ORIENTED_EDGE ( 'NONE', *, *, #4537, .F. ) ;
#3459=CIRCLE ( 'NONE', #9453, 2.000000000000000000 ) ;
#3460=VECTOR ( 'NONE', #2532, 1000.000000000000000 ) ;
#3463=ADVANCED_FACE ( 'NONE', ( #12564 ), #20616, .F. ) ;
#3464=CARTESIAN_POINT ( 'NONE',  ( 64.99999662536839651, -43.30127018922199511, 12.50000000000000000 ) ) ;
#3465=ORIENTED_EDGE ( 'NONE', *, *, #37075, .F. ) ;
#3466=CARTESIAN_POINT ( 'NONE',  ( 44.13139720814420031, 27.49999999999988987, -10.00000000000000178 ) ) ;
#3467=AXIS2_PLACEMENT_3D ( 'NONE', #270, #26516, #827 ) ;
#3469=DIRECTION ( 'NONE',  ( 0.4999999999999924505, -0.8660254037844429265, 0.000000000000000000 ) ) ;
#3470=VERTEX_POINT ( 'NONE', #29815 ) ;
#3471=CARTESIAN_POINT ( 'NONE',  ( 24.99999662536857059, 77.94228634059957983, -9.999999999999998224 ) ) ;
#3472=AXIS2_PLACEMENT_3D ( 'NONE', #24530, #10264, #21696 ) ;
#3473=CARTESIAN_POINT ( 'NONE',  ( 56.99999662536844625, -60.62177826491080168, 12.50000000000000000 ) ) ;
#3475=DIRECTION ( 'NONE',  ( -0.000000000000000000, -0.000000000000000000, 1.000000000000000000 ) ) ;
#3477=CARTESIAN_POINT ( 'NONE',  ( -18.00000337463123046, 86.60254037844397601, -9.999999999999998224 ) ) ;
#3478=LINE ( 'NONE', #26349, #22592 ) ;
#3479=CARTESIAN_POINT ( 'NONE',  ( -10.00000337463127842, -69.28203230275519786, 17.49999999999999645 ) ) ;
#3481=EDGE_CURVE ( 'NONE', #24271, #10050, #34822, .T. ) ;
#3482=DIRECTION ( 'NONE',  ( 1.000000000000000000, 0.000000000000000000, 0.000000000000000000 ) ) ;
#3483=AXIS2_PLACEMENT_3D ( 'NONE', #32431, #20607, #23825 ) ;
#3484=DIRECTION ( 'NONE',  ( 1.000000000000000000, 0.000000000000000000, 0.000000000000000000 ) ) ;
#3485=ORIENTED_EDGE ( 'NONE', *, *, #29941, .T. ) ;
#3489=DIRECTION ( 'NONE',  ( 0.000000000000000000, 0.000000000000000000, 1.000000000000000000 ) ) ;
#3490=EDGE_LOOP ( 'NONE', ( #31243, #21509, #9417, #11187 ) ) ;
#3493=ORIENTED_EDGE ( 'NONE', *, *, #8225, .F. ) ;
#3494=CARTESIAN_POINT ( 'NONE',  ( 67.99999662536838230, 34.64101615137758472, 12.50000000000000000 ) ) ;
#3495=FACE_OUTER_BOUND ( 'NONE', #19885, .T. ) ;
#3496=EDGE_CURVE ( 'NONE', #18808, #28322, #18055, .T. ) ;
#3497=CARTESIAN_POINT ( 'NONE',  ( 54.99999662536846046, -43.30127018922200222, 12.50000000000000000 ) ) ;
#3498=AXIS2_PLACEMENT_3D ( 'NONE', #6049, #3220, #14649 ) ;
#3499=CIRCLE ( 'NONE', #22050, 2.000000000000000000 ) ;
#3500=CARTESIAN_POINT ( 'NONE',  ( 32.99999662536853862, 77.94228634059959404, -9.999999999999998224 ) ) ;
#3502=DIRECTION ( 'NONE',  ( 0.000000000000000000, 0.000000000000000000, 1.000000000000000000 ) ) ;
#3503=EDGE_LOOP ( 'NONE', ( #19832, #16387, #30975, #20074, #33416, #34688, #17333, #26568, #26235, #1193, #10198, #1495, #16110, #25708, #16757, #13808, #27140, #16838, #31913, #3804, #10124, #19565, #36063, #26828 ) ) ;
#3504=AXIS2_PLACEMENT_3D ( 'NONE', #6565, #12148, #24002 ) ;
#3505=FACE_BOUND ( 'NONE', #35164, .T. ) ;
#3506=EDGE_CURVE ( 'NONE', #22424, #23506, #2488, .T. ) ;
#3507=AXIS2_PLACEMENT_3D ( 'NONE', #33679, #36853, #31396 ) ;
#3508=EDGE_CURVE ( 'NONE', #17720, #15986, #76, .T. ) ;
#3509=AXIS2_PLACEMENT_3D ( 'NONE', #17764, #29555, #35020 ) ;
#3510=CARTESIAN_POINT ( 'NONE',  ( -35.00000337463116296, 77.94228634059957983, -9.999999999999998224 ) ) ;
#3511=EDGE_CURVE ( 'NONE', #5353, #18222, #30609, .T. ) ;
#3512=ADVANCED_FACE ( 'NONE', ( #4322 ), #36383, .F. ) ;
#3513=CARTESIAN_POINT ( 'NONE',  ( -73.00000337463097821, 25.98076211353318854, 17.49999999999999645 ) ) ;
#3514=VERTEX_POINT ( 'NONE', #24944 ) ;
#3515=FACE_OUTER_BOUND ( 'NONE', #18788, .T. ) ;
#3517=AXIS2_PLACEMENT_3D ( 'NONE', #7695, #7884, #16491 ) ;
#3518=DIRECTION ( 'NONE',  ( -1.000000000000000000, 0.000000000000000000, 0.000000000000000000 ) ) ;
#3519=CARTESIAN_POINT ( 'NONE',  ( -50.00000337463109190, 51.96152422706637708, -9.999999999999998224 ) ) ;
#3520=LINE ( 'NONE', #12098, #568 ) ;
#3521=ORIENTED_EDGE ( 'NONE', *, *, #12132, .T. ) ;
#3522=DIRECTION ( 'NONE',  ( 1.000000000000000000, 0.000000000000000000, 0.000000000000000000 ) ) ;
#3523=DIRECTION ( 'NONE',  ( 1.000000000000000000, 0.000000000000000000, 0.000000000000000000 ) ) ;
#3524=DIRECTION ( 'NONE',  ( 1.000000000000000000, 0.000000000000000000, 0.000000000000000000 ) ) ;
#3526=ORIENTED_EDGE ( 'NONE', *, *, #1103, .T. ) ;
#3527=AXIS2_PLACEMENT_3D ( 'NONE', #29023, #34312, #20047 ) ;
#3529=AXIS2_PLACEMENT_3D ( 'NONE', #297, #2960, #14388 ) ;
#3530=DIRECTION ( 'NONE',  ( -0.000000000000000000, -0.000000000000000000, 1.000000000000000000 ) ) ;
#3531=EDGE_CURVE ( 'NONE', #6894, #10997, #10692, .T. ) ;
#3533=AXIS2_PLACEMENT_3D ( 'NONE', #25782, #31745, #14884 ) ;
#3534=DIRECTION ( 'NONE',  ( 0.000000000000000000, 0.000000000000000000, 1.000000000000000000 ) ) ;
#3537=AXIS2_PLACEMENT_3D ( 'NONE', #5802, #20034, #11040 ) ;
#3539=ORIENTED_EDGE ( 'NONE', *, *, #16911, .F. ) ;
#3540=ORIENTED_EDGE ( 'NONE', *, *, #26107, .F. ) ;
#3541=DIRECTION ( 'NONE',  ( 0.000000000000000000, 0.000000000000000000, 1.000000000000000000 ) ) ;
#3542=AXIS2_PLACEMENT_3D ( 'NONE', #14386, #17550, #31792 ) ;
#3543=DIRECTION ( 'NONE',  ( 1.000000000000000000, 0.000000000000000000, 0.000000000000000000 ) ) ;
#3544=AXIS2_PLACEMENT_3D ( 'NONE', #17912, #23920, #3279 ) ;
#3546=ORIENTED_EDGE ( 'NONE', *, *, #44, .T. ) ;
#3547=FACE_BOUND ( 'NONE', #29513, .T. ) ;
#3548=AXIS2_PLACEMENT_3D ( 'NONE', #25112, #4676, #5219 ) ;
#3549=ORIENTED_EDGE ( 'NONE', *, *, #31767, .T. ) ;
#3551=EDGE_CURVE ( 'NONE', #20954, #12074, #12643, .T. ) ;
#3552=CIRCLE ( 'NONE', #24519, 33.00000000000001421 ) ;
#3554=ORIENTED_EDGE ( 'NONE', *, *, #25836, .F. ) ;
#3555=CARTESIAN_POINT ( 'NONE',  ( -75.00000337463100664, -43.30127018922202353, -9.999999999999998224 ) ) ;
#3556=LINE ( 'NONE', #14990, #12526 ) ;
#3557=FACE_BOUND ( 'NONE', #264, .T. ) ;
#3561=VERTEX_POINT ( 'NONE', #22134 ) ;
#3564=ORIENTED_EDGE ( 'NONE', *, *, #6531, .T. ) ;
#3565=CARTESIAN_POINT ( 'NONE',  ( -45.00000337463111322, 77.94228634059959404, 17.49999999999999645 ) ) ;
#3566=CIRCLE ( 'NONE', #1076, 2.000000000000001776 ) ;
#3567=CARTESIAN_POINT ( 'NONE',  ( -86.45172111230354517, 31.46585318596159553, -49.86348611802629449 ) ) ;
#3568=ORIENTED_EDGE ( 'NONE', *, *, #23168, .T. ) ;
#3572=EDGE_CURVE ( 'NONE', #3470, #35481, #27638, .T. ) ;
#3573=ORIENTED_EDGE ( 'NONE', *, *, #3705, .F. ) ;
#3575=EDGE_CURVE ( 'NONE', #4901, #14195, #23440, .T. ) ;
#3576=DIRECTION ( 'NONE',  ( -0.000000000000000000, -0.000000000000000000, 1.000000000000000000 ) ) ;
#3577=DIRECTION ( 'NONE',  ( 1.000000000000000000, 0.000000000000000000, 0.000000000000000000 ) ) ;
#3578=ORIENTED_EDGE ( 'NONE', *, *, #8649, .T. ) ;
#3579=DIRECTION ( 'NONE',  ( 0.000000000000000000, 0.000000000000000000, 1.000000000000000000 ) ) ;
#3580=CIRCLE ( 'NONE', #7789, 2.000000000000001776 ) ;
#3581=DIRECTION ( 'NONE',  ( 0.000000000000000000, 0.000000000000000000, 1.000000000000000000 ) ) ;
#3582=VERTEX_POINT ( 'NONE', #27376 ) ;
#3583=ORIENTED_EDGE ( 'NONE', *, *, #20457, .T. ) ;
#3584=EDGE_CURVE ( 'NONE', #29631, #18343, #33577, .T. ) ;
#3586=DIRECTION ( 'NONE',  ( 1.000000000000000000, 0.000000000000000000, 0.000000000000000000 ) ) ;
#3589=ORIENTED_EDGE ( 'NONE', *, *, #33507, .F. ) ;
#3590=CARTESIAN_POINT ( 'NONE',  ( 77.99999662536833966, 17.32050807568879236, -9.999999999999998224 ) ) ;
#3591=CARTESIAN_POINT ( 'NONE',  ( 56.99999662536844625, 60.62177826491077326, -5.000000000000000000 ) ) ;
#3592=VERTEX_POINT ( 'NONE', #16490 ) ;
#3593=AXIS2_PLACEMENT_3D ( 'NONE', #60, #17317, #22933 ) ;
#3594=ADVANCED_FACE ( 'NONE', ( #7883 ), #30732, .F. ) ;
#3595=LINE ( 'NONE', #22912, #27362 ) ;
#3597=ORIENTED_EDGE ( 'NONE', *, *, #13848, .F. ) ;
#3598=DIRECTION ( 'NONE',  ( 0.000000000000000000, 0.000000000000000000, 1.000000000000000000 ) ) ;
#3600=AXIS2_PLACEMENT_3D ( 'NONE', #11159, #25613, #29142 ) ;
#3602=ORIENTED_EDGE ( 'NONE', *, *, #9371, .T. ) ;
#3603=EDGE_LOOP ( 'NONE', ( #13637, #908, #34139, #192 ) ) ;
#3605=DIRECTION ( 'NONE',  ( 0.000000000000000000, 0.000000000000000000, 1.000000000000000000 ) ) ;
#3606=CARTESIAN_POINT ( 'NONE',  ( -65.00000337463104927, -43.30127018922202353, 12.50000000000000000 ) ) ;
#3607=DIRECTION ( 'NONE',  ( 0.000000000000000000, 0.000000000000000000, 1.000000000000000000 ) ) ;
#3609=CYLINDRICAL_SURFACE ( 'NONE', #5189, 2.000000000000001776 ) ;
#3610=EDGE_CURVE ( 'NONE', #23016, #19957, #4881, .T. ) ;
#3611=FACE_BOUND ( 'NONE', #34955, .T. ) ;
#3612=FACE_OUTER_BOUND ( 'NONE', #9599, .T. ) ;
#3613=CARTESIAN_POINT ( 'NONE',  ( -75.00000337463097821, 8.660254037844374864, -5.000000000000000000 ) ) ;
#3614=CARTESIAN_POINT ( 'NONE',  ( -22.00000337463122690, 86.60254037844397601, -5.000000000000000000 ) ) ;
#3615=EDGE_LOOP ( 'NONE', ( #16192, #3857 ) ) ;
#3616=LINE ( 'NONE', #23308, #28459 ) ;
#3618=VECTOR ( 'NONE', #23063, 1000.000000000000000 ) ;
#3619=VERTEX_POINT ( 'NONE', #36188 ) ;
#3620=LINE ( 'NONE', #34760, #36407 ) ;
#3621=ADVANCED_FACE ( 'NONE', ( #10492 ), #16144, .F. ) ;
#3622=FACE_BOUND ( 'NONE', #25500, .T. ) ;
#3623=AXIS2_PLACEMENT_3D ( 'NONE', #8029, #33730, #28099 ) ;
#3624=DIRECTION ( 'NONE',  ( 0.000000000000000000, 0.000000000000000000, 1.000000000000000000 ) ) ;
#3625=ORIENTED_EDGE ( 'NONE', *, *, #8745, .F. ) ;
#3626=VERTEX_POINT ( 'NONE', #5052 ) ;
#3628=EDGE_CURVE ( 'NONE', #27334, #36171, #19253, .T. ) ;
#3629=CARTESIAN_POINT ( 'NONE',  ( -90.00000337463090716, -1.040834085586084257E-14, -5.000000000000000000 ) ) ;
#3632=ORIENTED_EDGE ( 'NONE', *, *, #9070, .T. ) ;
#3633=ORIENTED_EDGE ( 'NONE', *, *, #19962, .F. ) ;
#3634=ORIENTED_EDGE ( 'NONE', *, *, #17630, .T. ) ;
#3635=DIRECTION ( 'NONE',  ( 0.000000000000000000, 0.000000000000000000, 1.000000000000000000 ) ) ;
#3636=ORIENTED_EDGE ( 'NONE', *, *, #7763, .T. ) ;
#3638=EDGE_LOOP ( 'NONE', ( #22948, #34679 ) ) ;
#3639=DIRECTION ( 'NONE',  ( 1.000000000000000000, 0.000000000000000000, 0.000000000000000000 ) ) ;
#3641=EDGE_LOOP ( 'NONE', ( #7283, #7896 ) ) ;
#3642=ADVANCED_FACE ( 'NONE', ( #13303 ), #18755, .F. ) ;
#3643=CARTESIAN_POINT ( 'NONE',  ( -65.00000337463102085, 43.30127018922198801, -9.999999999999998224 ) ) ;
#3644=FACE_BOUND ( 'NONE', #12085, .T. ) ;
#3646=AXIS2_PLACEMENT_3D ( 'NONE', #15180, #26611, #12918 ) ;
#3647=ORIENTED_EDGE ( 'NONE', *, *, #24373, .F. ) ;
#3648=ORIENTED_EDGE ( 'NONE', *, *, #10882, .F. ) ;
#3649=CARTESIAN_POINT ( 'NONE',  ( 34.99999662536855283, -60.62177826491080168, -9.999999999999998224 ) ) ;
#3650=EDGE_CURVE ( 'NONE', #4700, #34182, #32420, .T. ) ;
#3652=DIRECTION ( 'NONE',  ( 1.000000000000000000, 0.000000000000000000, 0.000000000000000000 ) ) ;
#3653=ORIENTED_EDGE ( 'NONE', *, *, #33769, .F. ) ;
#3654=DIRECTION ( 'NONE',  ( 1.000000000000000000, 0.000000000000000000, 0.000000000000000000 ) ) ;
#3656=EDGE_CURVE ( 'NONE', #23102, #9991, #9662, .T. ) ;
#3657=EDGE_LOOP ( 'NONE', ( #3539, #19970 ) ) ;
#3660=CARTESIAN_POINT ( 'NONE',  ( 79.99999662536833966, 34.64101615137759183, 12.50000000000000000 ) ) ;
#3661=CARTESIAN_POINT ( 'NONE',  ( 7.999996625368656744, -86.60254037844400443, 12.50000000000000000 ) ) ;
#3662=CARTESIAN_POINT ( 'NONE',  ( -10.00000337463128730, 69.28203230275516944, -9.999999999999998224 ) ) ;
#3663=DIRECTION ( 'NONE',  ( 0.000000000000000000, 0.000000000000000000, 1.000000000000000000 ) ) ;
#3664=ORIENTED_EDGE ( 'NONE', *, *, #34211, .F. ) ;
#3665=CYLINDRICAL_SURFACE ( 'NONE', #7038, 3.000000000000002665 ) ;
#3666=DIRECTION ( 'NONE',  ( 1.000000000000000000, 0.000000000000000000, 0.000000000000000000 ) ) ;
#3667=LINE ( 'NONE', #23535, #34360 ) ;
#3668=ORIENTED_EDGE ( 'NONE', *, *, #26855, .T. ) ;
#3669=ORIENTED_EDGE ( 'NONE', *, *, #5032, .T. ) ;
#3670=VERTEX_POINT ( 'NONE', #18587 ) ;
#3671=EDGE_CURVE ( 'NONE', #13923, #18360, #21743, .T. ) ;
#3674=CYLINDRICAL_SURFACE ( 'NONE', #24280, 2.000000000000001776 ) ;
#3675=CARTESIAN_POINT ( 'NONE',  ( 72.99999662536835388, -43.30127018922199511, -9.999999999999998224 ) ) ;
#3676=CARTESIAN_POINT ( 'NONE',  ( 9.999996625368618552, 69.28203230275516944, -9.999999999999998224 ) ) ;
#3677=ORIENTED_EDGE ( 'NONE', *, *, #12616, .F. ) ;
#3679=FACE_OUTER_BOUND ( 'NONE', #21697, .T. ) ;
#3680=ORIENTED_EDGE ( 'NONE', *, *, #34602, .F. ) ;
#3681=FACE_BOUND ( 'NONE', #19890, .T. ) ;
#3682=ADVANCED_FACE ( 'NONE', ( #31115 ), #33748, .F. ) ;
#3683=DIRECTION ( 'NONE',  ( 1.000000000000000000, 0.000000000000000000, 0.000000000000000000 ) ) ;
#3685=EDGE_CURVE ( 'NONE', #12225, #19686, #9285, .T. ) ;
#3686=ORIENTED_EDGE ( 'NONE', *, *, #17001, .T. ) ;
#3688=VECTOR ( 'NONE', #7497, 1000.000000000000000 ) ;
#3690=EDGE_CURVE ( 'NONE', #18793, #15817, #11417, .T. ) ;
#3691=CARTESIAN_POINT ( 'NONE',  ( 29.99999662536856349, 69.28203230275518365, -9.999999999999998224 ) ) ;
#3693=CARTESIAN_POINT ( 'NONE',  ( -30.00000337463118427, 69.28203230275516944, -9.999999999999998224 ) ) ;
#3695=LINE ( 'NONE', #26386, #7025 ) ;
#3697=DIRECTION ( 'NONE',  ( -1.000000000000000000, 0.000000000000000000, 0.000000000000000000 ) ) ;
#3698=CARTESIAN_POINT ( 'NONE',  ( 26.99999662536856704, 77.94228634059957983, 17.49999999999999645 ) ) ;
#3699=EDGE_CURVE ( 'NONE', #31147, #31233, #15060, .T. ) ;
#3701=ORIENTED_EDGE ( 'NONE', *, *, #7925, .T. ) ;
#3702=ORIENTED_EDGE ( 'NONE', *, *, #23999, .T. ) ;
#3705=EDGE_CURVE ( 'NONE', #18803, #19499, #34987, .T. ) ;
#3706=EDGE_CURVE ( 'NONE', #8132, #8981, #22854, .T. ) ;
#3707=DIRECTION ( 'NONE',  ( 1.000000000000000000, 0.000000000000000000, 0.000000000000000000 ) ) ;
#3708=EDGE_CURVE ( 'NONE', #10163, #33312, #36618, .T. ) ;
#3709=AXIS2_PLACEMENT_3D ( 'NONE', #33632, #7935, #36074 ) ;
#3710=ADVANCED_FACE ( 'NONE', ( #36740 ), #28287, .F. ) ;
#3711=CARTESIAN_POINT ( 'NONE',  ( -3.374631327851540519E-06, 86.60254037844397601, -5.000000000000000000 ) ) ;
#3713=EDGE_CURVE ( 'NONE', #24720, #15837, #2803, .T. ) ;
#3714=CARTESIAN_POINT ( 'NONE',  ( 74.99999662536835388, -43.30127018922199511, -9.999999999999998224 ) ) ;
#3716=EDGE_LOOP ( 'NONE', ( #30677, #7672, #10091, #21475, #15396, #15031 ) ) ;
#3718=DIRECTION ( 'NONE',  ( 1.000000000000000000, 0.000000000000000000, 0.000000000000000000 ) ) ;
#3719=ORIENTED_EDGE ( 'NONE', *, *, #22834, .F. ) ;
#3720=CARTESIAN_POINT ( 'NONE',  ( 74.99999662536836809, 43.30127018922198801, 12.50000000000000000 ) ) ;
#3721=ORIENTED_EDGE ( 'NONE', *, *, #11363, .F. ) ;
#3722=FACE_BOUND ( 'NONE', #11433, .T. ) ;
#3723=ORIENTED_EDGE ( 'NONE', *, *, #31276, .T. ) ;
#3724=ORIENTED_EDGE ( 'NONE', *, *, #25866, .T. ) ;
#3726=ORIENTED_EDGE ( 'NONE', *, *, #24604, .F. ) ;
#3727=DIRECTION ( 'NONE',  ( 0.000000000000000000, 0.000000000000000000, -1.000000000000000000 ) ) ;
#3728=CIRCLE ( 'NONE', #34281, 2.000000000000001776 ) ;
#3730=DIRECTION ( 'NONE',  ( 0.000000000000000000, 0.000000000000000000, 1.000000000000000000 ) ) ;
#3731=ORIENTED_EDGE ( 'NONE', *, *, #16812, .F. ) ;
#3732=ORIENTED_EDGE ( 'NONE', *, *, #29115, .F. ) ;
#3733=VERTEX_POINT ( 'NONE', #15103 ) ;
#3734=ORIENTED_EDGE ( 'NONE', *, *, #934, .T. ) ;
#3735=VERTEX_POINT ( 'NONE', #2608 ) ;
#3736=CARTESIAN_POINT ( 'NONE',  ( -80.00000337463094979, -2.428612866367529932E-14, -5.000000000000000000 ) ) ;
#3737=CARTESIAN_POINT ( 'NONE',  ( 77.99999662536833966, 34.64101615137759183, -9.999999999999998224 ) ) ;
#3738=ORIENTED_EDGE ( 'NONE', *, *, #19930, .F. ) ;
#3741=LINE ( 'NONE', #6567, #6973 ) ;
#3742=ORIENTED_EDGE ( 'NONE', *, *, #18105, .F. ) ;
#3744=AXIS2_PLACEMENT_3D ( 'NONE', #2292, #5478, #8300 ) ;
#3745=CYLINDRICAL_SURFACE ( 'NONE', #36600, 2.000000000000001776 ) ;
#3746=EDGE_CURVE ( 'NONE', #716, #29611, #11438, .T. ) ;
#3747=CARTESIAN_POINT ( 'NONE',  ( 66.99999662536839651, 60.62177826491078747, -9.999999999999998224 ) ) ;
#3748=ORIENTED_EDGE ( 'NONE', *, *, #15092, .F. ) ;
#3750=CARTESIAN_POINT ( 'NONE',  ( 34.99999662536855283, -60.62177826491080168, 12.50000000000000000 ) ) ;
#3752=ORIENTED_EDGE ( 'NONE', *, *, #19894, .F. ) ;
#3753=CYLINDRICAL_SURFACE ( 'NONE', #31976, 2.000000000000001776 ) ;
#3754=DIRECTION ( 'NONE',  ( 0.000000000000000000, 0.000000000000000000, 1.000000000000000000 ) ) ;
#3755=DIRECTION ( 'NONE',  ( -1.000000000000000000, 0.000000000000000000, 0.000000000000000000 ) ) ;
#3758=CARTESIAN_POINT ( 'NONE',  ( -30.00000337463118427, 69.28203230275516944, 12.50000000000000000 ) ) ;
#3759=DIRECTION ( 'NONE',  ( 0.000000000000000000, 0.000000000000000000, 1.000000000000000000 ) ) ;
#3760=ORIENTED_EDGE ( 'NONE', *, *, #12376, .T. ) ;
#3761=DIRECTION ( 'NONE',  ( -0.000000000000000000, -0.000000000000000000, 1.000000000000000000 ) ) ;
#3762=EDGE_LOOP ( 'NONE', ( #8508, #22112 ) ) ;
#3764=DIRECTION ( 'NONE',  ( 0.000000000000000000, 0.000000000000000000, 1.000000000000000000 ) ) ;
#3765=CIRCLE ( 'NONE', #21140, 2.999999999999999556 ) ;
#3766=DIRECTION ( 'NONE',  ( -1.000000000000000000, 0.000000000000000000, 0.000000000000000000 ) ) ;
#3767=DIRECTION ( 'NONE',  ( 0.000000000000000000, 0.000000000000000000, 1.000000000000000000 ) ) ;
#3768=ORIENTED_EDGE ( 'NONE', *, *, #3231, .T. ) ;
#3771=VERTEX_POINT ( 'NONE', #672 ) ;
#3772=DIRECTION ( 'NONE',  ( 1.000000000000000000, 0.000000000000000000, 0.000000000000000000 ) ) ;
#3773=CIRCLE ( 'NONE', #1987, 2.000000000000001776 ) ;
#3774=CARTESIAN_POINT ( 'NONE',  ( 0.000000000000000000, 0.000000000000000000, 17.49999999999999645 ) ) ;
#3775=CARTESIAN_POINT ( 'NONE',  ( -31.09745072740852123, -83.47442710120346021, 12.49999999999999645 ) ) ;
#3777=CARTESIAN_POINT ( 'NONE',  ( -32.16008401677954254, -61.25926521283091830, -49.22241343995298024 ) ) ;
#3778=EDGE_LOOP ( 'NONE', ( #24758, #15893 ) ) ;
#3782=EDGE_CURVE ( 'NONE', #13768, #7831, #21651, .T. ) ;
#3784=ORIENTED_EDGE ( 'NONE', *, *, #6674, .T. ) ;
#3786=DIRECTION ( 'NONE',  ( 0.000000000000000000, 0.000000000000000000, 1.000000000000000000 ) ) ;
#3787=AXIS2_PLACEMENT_3D ( 'NONE', #33656, #7958, #36825 ) ;
#3788=DIRECTION ( 'NONE',  ( 1.000000000000000000, 0.000000000000000000, 0.000000000000000000 ) ) ;
#3790=AXIS2_PLACEMENT_3D ( 'NONE', #10491, #22133, #30731 ) ;
#3791=ORIENTED_EDGE ( 'NONE', *, *, #21551, .F. ) ;
#3793=CARTESIAN_POINT ( 'NONE',  ( -10.00000337463127842, -69.28203230275519786, -5.000000000000000000 ) ) ;
#3795=EDGE_LOOP ( 'NONE', ( #532, #22246 ) ) ;
#3798=AXIS2_PLACEMENT_3D ( 'NONE', #21850, #2868, #33290 ) ;
#3799=DIRECTION ( 'NONE',  ( -0.000000000000000000, -0.000000000000000000, 1.000000000000000000 ) ) ;
#3800=CIRCLE ( 'NONE', #4991, 2.000000000000001776 ) ;
#3801=EDGE_LOOP ( 'NONE', ( #16195, #9358 ) ) ;
#3802=EDGE_CURVE ( 'NONE', #2177, #8794, #20032, .T. ) ;
#3804=ORIENTED_EDGE ( 'NONE', *, *, #16288, .T. ) ;
#3805=DIRECTION ( 'NONE',  ( 1.000000000000000000, 0.000000000000000000, 0.000000000000000000 ) ) ;
#3807=EDGE_CURVE ( 'NONE', #21828, #12432, #26428, .T. ) ;
#3808=CIRCLE ( 'NONE', #25368, 2.000000000000001776 ) ;
#3809=ORIENTED_EDGE ( 'NONE', *, *, #15029, .F. ) ;
#3810=DIRECTION ( 'NONE',  ( -1.000000000000000000, 0.000000000000000000, 0.000000000000000000 ) ) ;
#3811=CARTESIAN_POINT ( 'NONE',  ( 66.99999662536839651, -60.62177826491080168, -9.999999999999998224 ) ) ;
#3813=EDGE_CURVE ( 'NONE', #14280, #12923, #31229, .T. ) ;
#3814=ORIENTED_EDGE ( 'NONE', *, *, #18805, .F. ) ;
#3815=CARTESIAN_POINT ( 'NONE',  ( 71.99999662536839651, -3.469446951953614189E-15, -9.999999999999998224 ) ) ;
#3817=DIRECTION ( 'NONE',  ( -0.000000000000000000, -0.000000000000000000, 1.000000000000000000 ) ) ;
#3818=DIRECTION ( 'NONE',  ( 0.000000000000000000, 0.000000000000000000, -1.000000000000000000 ) ) ;
#3820=ORIENTED_EDGE ( 'NONE', *, *, #13282, .F. ) ;
#3821=FACE_OUTER_BOUND ( 'NONE', #10290, .T. ) ;
#3823=EDGE_LOOP ( 'NONE', ( #19189, #13639, #4459, #25732, #19468 ) ) ;
#3826=PLANE ( 'NONE',  #21979 ) ;
#3830=VECTOR ( 'NONE', #20435, 1000.000000000000000 ) ;
#3831=CARTESIAN_POINT ( 'NONE',  ( -86.45172111230354517, 31.46585318596159553, -4.999999999999997335 ) ) ;
#3832=ORIENTED_EDGE ( 'NONE', *, *, #21506, .F. ) ;
#3833=DIRECTION ( 'NONE',  ( -1.000000000000000000, 0.000000000000000000, 0.000000000000000000 ) ) ;
#3834=DIRECTION ( 'NONE',  ( 0.000000000000000000, 0.000000000000000000, 1.000000000000000000 ) ) ;
#3835=CARTESIAN_POINT ( 'NONE',  ( -65.00000337463104927, -43.30127018922202353, 17.49999999999999645 ) ) ;
#3836=ORIENTED_EDGE ( 'NONE', *, *, #35591, .F. ) ;
#3837=EDGE_CURVE ( 'NONE', #7714, #8170, #23736, .T. ) ;
#3838=ORIENTED_EDGE ( 'NONE', *, *, #27411, .F. ) ;
#3839=VERTEX_POINT ( 'NONE', #1406 ) ;
#3841=CARTESIAN_POINT ( 'NONE',  ( 57.99999662536843914, -34.64101615137759893, 17.49999999999999645 ) ) ;
#3842=CARTESIAN_POINT ( 'NONE',  ( 84.99999662536831124, -8.660254037844397956, 12.50000000000000000 ) ) ;
#3843=EDGE_CURVE ( 'NONE', #21147, #5770, #23311, .T. ) ;
#3845=CARTESIAN_POINT ( 'NONE',  ( 79.99999662536833966, -3.469446951953614189E-15, 12.50000000000000000 ) ) ;
#3847=ORIENTED_EDGE ( 'NONE', *, *, #26135, .T. ) ;
#3848=ADVANCED_FACE ( 'NONE', ( #1236 ), #7235, .F. ) ;
#3850=EDGE_LOOP ( 'NONE', ( #26634, #10376, #24662, #5165, #17182, #35032, #5481, #168, #33522, #25667, #19228, #22128, #12935, #9351, #21001, #14227 ) ) ;
#3851=FACE_BOUND ( 'NONE', #26506, .T. ) ;
#3852=AXIS2_PLACEMENT_3D ( 'NONE', #28679, #25154, #8443 ) ;
#3853=VECTOR ( 'NONE', #8795, 1000.000000000000000 ) ;
#3855=AXIS2_PLACEMENT_3D ( 'NONE', #15743, #2236, #27166 ) ;
#3856=CARTESIAN_POINT ( 'NONE',  ( -59.13646009116099833, 70.47608876694653190, 12.49999999999999822 ) ) ;
#3857=ORIENTED_EDGE ( 'NONE', *, *, #3551, .T. ) ;
#3858=CARTESIAN_POINT ( 'NONE',  ( -78.00000337463094979, 34.64101615137757051, -9.999999999999998224 ) ) ;
#3860=CARTESIAN_POINT ( 'NONE',  ( -57.00000337463107059, 43.30127018922197379, 17.49999999999999645 ) ) ;
#3862=CIRCLE ( 'NONE', #863, 2.000000000000001776 ) ;
#3863=CARTESIAN_POINT ( 'NONE',  ( -72.00000337463100664, -2.404119930384582903E-14, 17.49999999999999645 ) ) ;
#3864=CARTESIAN_POINT ( 'NONE',  ( -50.00000337463112032, -51.96152422706641971, 17.49999999999999645 ) ) ;
#3865=ORIENTED_EDGE ( 'NONE', *, *, #16134, .T. ) ;
#3867=CIRCLE ( 'NONE', #18234, 2.000000000000001776 ) ;
#3869=CARTESIAN_POINT ( 'NONE',  ( 34.99999662536855283, -77.94228634059960825, 17.49999999999999645 ) ) ;
#3870=ORIENTED_EDGE ( 'NONE', *, *, #18751, .F. ) ;
#3872=VERTEX_POINT ( 'NONE', #12653 ) ;
#3873=ORIENTED_EDGE ( 'NONE', *, *, #16935, .T. ) ;
#3875=CYLINDRICAL_SURFACE ( 'NONE', #34529, 2.000000000000001776 ) ;
#3876=CIRCLE ( 'NONE', #258, 2.000000000000001776 ) ;
#3877=AXIS2_PLACEMENT_3D ( 'NONE', #33943, #31124, #25315 ) ;
#3879=EDGE_CURVE ( 'NONE', #30974, #985, #10151, .T. ) ;
#3880=DIRECTION ( 'NONE',  ( 1.000000000000000000, 0.000000000000000000, 0.000000000000000000 ) ) ;
#3884=ORIENTED_EDGE ( 'NONE', *, *, #5109, .T. ) ;
#3885=ADVANCED_FACE ( 'NONE', ( #18283 ), #35929, .F. ) ;
#3886=ORIENTED_EDGE ( 'NONE', *, *, #27351, .T. ) ;
#3887=DIRECTION ( 'NONE',  ( 1.000000000000000000, 0.000000000000000000, 0.000000000000000000 ) ) ;
#3891=CIRCLE ( 'NONE', #18267, 2.000000000000001776 ) ;
#3892=EDGE_CURVE ( 'NONE', #19957, #27668, #7152, .T. ) ;
#3894=EDGE_CURVE ( 'NONE', #23537, #9788, #17932, .T. ) ;
#3896=DIRECTION ( 'NONE',  ( 0.000000000000000000, 0.000000000000000000, 1.000000000000000000 ) ) ;
#3897=ORIENTED_EDGE ( 'NONE', *, *, #28920, .T. ) ;
#3898=ORIENTED_EDGE ( 'NONE', *, *, #12393, .T. ) ;
#3899=PLANE ( 'NONE',  #33818 ) ;
#3903=AXIS2_PLACEMENT_3D ( 'NONE', #6307, #14391, #3518 ) ;
#3904=EDGE_CURVE ( 'NONE', #21416, #30265, #32718, .T. ) ;
#3905=DIRECTION ( 'NONE',  ( 1.000000000000000000, 0.000000000000000000, 0.000000000000000000 ) ) ;
#3906=EDGE_CURVE ( 'NONE', #26494, #1764, #37102, .T. ) ;
#3907=FACE_OUTER_BOUND ( 'NONE', #34314, .T. ) ;
#3908=DIRECTION ( 'NONE',  ( 0.000000000000000000, 0.000000000000000000, 1.000000000000000000 ) ) ;
#3910=ORIENTED_EDGE ( 'NONE', *, *, #16650, .T. ) ;
#3911=ORIENTED_EDGE ( 'NONE', *, *, #21136, .F. ) ;
#3912=ORIENTED_EDGE ( 'NONE', *, *, #29505, .T. ) ;
#3913=ORIENTED_EDGE ( 'NONE', *, *, #13313, .T. ) ;
#3914=CIRCLE ( 'NONE', #28454, 2.000000000000001776 ) ;
#3915=DIRECTION ( 'NONE',  ( 0.000000000000000000, 0.000000000000000000, 1.000000000000000000 ) ) ;
#3917=VERTEX_POINT ( 'NONE', #4243 ) ;
#3918=AXIS2_PLACEMENT_3D ( 'NONE', #25029, #8331, #10934 ) ;
#3919=CARTESIAN_POINT ( 'NONE',  ( 81.99999662536833966, 17.32050807568879236, -9.999999999999998224 ) ) ;
#3921=CARTESIAN_POINT ( 'NONE',  ( 9.999996625368655856, -69.28203230275519786, 17.49999999999999645 ) ) ;
#3922=AXIS2_PLACEMENT_3D ( 'NONE', #14082, #17294, #11459 ) ;
#3924=VECTOR ( 'NONE', #26447, 1000.000000000000000 ) ;
#3926=AXIS2_PLACEMENT_3D ( 'NONE', #36875, #16997, #11184 ) ;
#3927=DIRECTION ( 'NONE',  ( 0.000000000000000000, 0.000000000000000000, 1.000000000000000000 ) ) ;
#3928=EDGE_CURVE ( 'NONE', #29624, #10165, #32920, .T. ) ;
#3929=DIRECTION ( 'NONE',  ( 0.000000000000000000, -0.000000000000000000, -1.000000000000000000 ) ) ;
#3931=DIRECTION ( 'NONE',  ( 0.000000000000000000, 0.000000000000000000, 1.000000000000000000 ) ) ;
#3932=EDGE_CURVE ( 'NONE', #35812, #19005, #32358, .T. ) ;
#3933=DIRECTION ( 'NONE',  ( 1.000000000000000000, 0.000000000000000000, 0.000000000000000000 ) ) ;
#3934=ORIENTED_EDGE ( 'NONE', *, *, #16860, .F. ) ;
#3935=CIRCLE ( 'NONE', #27272, 2.000000000000001776 ) ;
#3936=ORIENTED_EDGE ( 'NONE', *, *, #17223, .F. ) ;
#3937=CARTESIAN_POINT ( 'NONE',  ( -34.60911769017402406, 75.98085615278088767, -5.000000000000000000 ) ) ;
#3938=LINE ( 'NONE', #15382, #25940 ) ;
#3939=DIRECTION ( 'NONE',  ( -1.000000000000000000, 1.773272886554068598E-14, 0.000000000000000000 ) ) ;
#3940=DIRECTION ( 'NONE',  ( 0.000000000000000000, 0.000000000000000000, 1.000000000000000000 ) ) ;
#3941=EDGE_CURVE ( 'NONE', #12218, #22555, #1766, .T. ) ;
#3942=ORIENTED_EDGE ( 'NONE', *, *, #5104, .T. ) ;
#3943=VECTOR ( 'NONE', #19020, 1000.000000000000000 ) ;
#3944=DIRECTION ( 'NONE',  ( -0.000000000000000000, -0.000000000000000000, 1.000000000000000000 ) ) ;
#3946=AXIS2_PLACEMENT_3D ( 'NONE', #21461, #10217, #13564 ) ;
#3947=VERTEX_POINT ( 'NONE', #6673 ) ;
#3949=STYLED_ITEM ( 'NONE', ( #24763 ), #20178 ) ;
#3950=FACE_OUTER_BOUND ( 'NONE', #9162, .T. ) ;
#3951=ORIENTED_EDGE ( 'NONE', *, *, #31804, .T. ) ;
#3953=EDGE_CURVE ( 'NONE', #14173, #3447, #27472, .T. ) ;
#3955=DIRECTION ( 'NONE',  ( 1.000000000000000000, 0.000000000000000000, 0.000000000000000000 ) ) ;
#3957=EDGE_CURVE ( 'NONE', #18237, #20586, #14937, .T. ) ;
#3958=CARTESIAN_POINT ( 'NONE',  ( -70.00000337463102085, -34.64101615137762025, 12.50000000000000000 ) ) ;
#3960=EDGE_CURVE ( 'NONE', #11611, #2623, #8933, .T. ) ;
#3963=ORIENTED_EDGE ( 'NONE', *, *, #17637, .F. ) ;
#3964=ORIENTED_EDGE ( 'NONE', *, *, #23229, .F. ) ;
#3965=AXIS2_PLACEMENT_3D ( 'NONE', #13085, #24543, #35980 ) ;
#3966=CARTESIAN_POINT ( 'NONE',  ( -90.00000337463090716, -1.040834085586084257E-14, 12.50000000000000000 ) ) ;
#3967=ORIENTED_EDGE ( 'NONE', *, *, #16998, .T. ) ;
#3968=DIRECTION ( 'NONE',  ( -1.000000000000000000, 0.000000000000000000, 0.000000000000000000 ) ) ;
#3971=DIRECTION ( 'NONE',  ( 0.000000000000000000, 0.000000000000000000, 1.000000000000000000 ) ) ;
#3972=CARTESIAN_POINT ( 'NONE',  ( 67.99999662536836809, -34.64101615137759183, -9.999999999999998224 ) ) ;
#3973=EDGE_LOOP ( 'NONE', ( #10488, #18734 ) ) ;
#3974=DIRECTION ( 'NONE',  ( 0.000000000000000000, 0.000000000000000000, -1.000000000000000000 ) ) ;
#3976=DIRECTION ( 'NONE',  ( 0.000000000000000000, 0.000000000000000000, 1.000000000000000000 ) ) ;
#3977=ORIENTED_EDGE ( 'NONE', *, *, #915, .F. ) ;
#3981=CARTESIAN_POINT ( 'NONE',  ( -83.00000337463092137, -8.660254037844422825, -9.999999999999998224 ) ) ;
#3982=AXIS2_PLACEMENT_3D ( 'NONE', #12822, #10395, #12649 ) ;
#3983=AXIS2_PLACEMENT_3D ( 'NONE', #9317, #20752, #29552 ) ;
#3984=AXIS2_PLACEMENT_3D ( 'NONE', #35961, #24135, #24878 ) ;
#3985=EDGE_CURVE ( 'NONE', #9651, #7111, #5524, .T. ) ;
#3986=ORIENTED_EDGE ( 'NONE', *, *, #22968, .F. ) ;
#3989=CIRCLE ( 'NONE', #35745, 2.000000000000001776 ) ;
#3990=PLANE ( 'NONE',  #30670 ) ;
#3991=CARTESIAN_POINT ( 'NONE',  ( -68.00000337463099243, -2.428612866367529932E-14, -9.999999999999998224 ) ) ;
#3992=DIRECTION ( 'NONE',  ( 0.000000000000000000, 0.000000000000000000, 1.000000000000000000 ) ) ;
#3993=EDGE_LOOP ( 'NONE', ( #5322, #27054, #7552, #34599 ) ) ;
#3994=ORIENTED_EDGE ( 'NONE', *, *, #11003, .T. ) ;
#3995=ORIENTED_EDGE ( 'NONE', *, *, #28335, .F. ) ;
#3996=AXIS2_PLACEMENT_3D ( 'NONE', #7199, #4563, #12786 ) ;
#3997=LINE ( 'NONE', #19192, #21297 ) ;
#3998=EDGE_LOOP ( 'NONE', ( #32582, #34625, #5229, #2926 ) ) ;
#3999=ORIENTED_EDGE ( 'NONE', *, *, #10536, .T. ) ;
#4000=CARTESIAN_POINT ( 'NONE',  ( -82.00000337463094979, -17.32050807568882078, -9.999999999999998224 ) ) ;
#4001=VERTEX_POINT ( 'NONE', #28208 ) ;
#4003=ORIENTED_EDGE ( 'NONE', *, *, #37031, .T. ) ;
#4004=CARTESIAN_POINT ( 'NONE',  ( -52.00000337463112032, -51.96152422706641971, -9.999999999999998224 ) ) ;
#4005=AXIS2_PLACEMENT_3D ( 'NONE', #34878, #9169, #20601 ) ;
#4006=LINE ( 'NONE', #13190, #27831 ) ;
#4007=EDGE_CURVE ( 'NONE', #7029, #30130, #19726, .T. ) ;
#4008=ORIENTED_EDGE ( 'NONE', *, *, #19655, .F. ) ;
#4009=EDGE_LOOP ( 'NONE', ( #23883, #2603 ) ) ;
#4010=CYLINDRICAL_SURFACE ( 'NONE', #20893, 2.000000000000001776 ) ;
#4012=AXIS2_PLACEMENT_3D ( 'NONE', #11342, #12050, #12221 ) ;
#4013=AXIS2_PLACEMENT_3D ( 'NONE', #21973, #15012, #3384 ) ;
#4014=DIRECTION ( 'NONE',  ( 1.000000000000000000, 0.000000000000000000, 0.000000000000000000 ) ) ;
#4015=DIRECTION ( 'NONE',  ( -1.000000000000000000, 0.000000000000000000, 0.000000000000000000 ) ) ;
#4016=AXIS2_PLACEMENT_3D ( 'NONE', #28129, #31127, #7891 ) ;
#4017=VECTOR ( 'NONE', #17362, 1000.000000000000000 ) ;
#4018=ORIENTED_EDGE ( 'NONE', *, *, #19551, .F. ) ;
#4019=CYLINDRICAL_SURFACE ( 'NONE', #19534, 2.000000000000001776 ) ;
#4020=LINE ( 'NONE', #18077, #15568 ) ;
#4021=ORIENTED_EDGE ( 'NONE', *, *, #6713, .F. ) ;
#4022=CARTESIAN_POINT ( 'NONE',  ( 0.000000000000000000, 0.000000000000000000, 12.49999999999999822 ) ) ;
#4023=DIRECTION ( 'NONE',  ( 1.000000000000000000, 0.000000000000000000, 0.000000000000000000 ) ) ;
#4024=FACE_OUTER_BOUND ( 'NONE', #12787, .T. ) ;
#4026=AXIS2_PLACEMENT_3D ( 'NONE', #29668, #29873, #16194 ) ;
#4027=CARTESIAN_POINT ( 'NONE',  ( 2.999996625368676728, -77.94228634059960825, -5.000000000000000000 ) ) ;
#4028=CARTESIAN_POINT ( 'NONE',  ( -70.00000337463102085, -34.64101615137762025, -9.999999999999998224 ) ) ;
#4029=ORIENTED_EDGE ( 'NONE', *, *, #21897, .T. ) ;
#4030=CARTESIAN_POINT ( 'NONE',  ( -77.00000337463097821, 8.660254037844374864, 17.49999999999999645 ) ) ;
#4031=AXIS2_PLACEMENT_3D ( 'NONE', #25209, #33813, #28355 ) ;
#4032=CARTESIAN_POINT ( 'NONE',  ( -77.00000337463100664, -43.30127018922202353, -9.999999999999998224 ) ) ;
#4033=DIRECTION ( 'NONE',  ( 0.000000000000000000, 0.000000000000000000, 1.000000000000000000 ) ) ;
#4034=EDGE_CURVE ( 'NONE', #17256, #17808, #13702, .T. ) ;
#4035=AXIS2_PLACEMENT_3D ( 'NONE', #1336, #32456, #4168 ) ;
#4037=VERTEX_POINT ( 'NONE', #8349 ) ;
#4038=VERTEX_POINT ( 'NONE', #25048 ) ;
#4039=CIRCLE ( 'NONE', #33971, 2.000000000000001776 ) ;
#4040=CARTESIAN_POINT ( 'NONE',  ( -65.00000337463102085, 43.30127018922198801, 12.50000000000000000 ) ) ;
#4041=CYLINDRICAL_SURFACE ( 'NONE', #14840, 2.000000000000001776 ) ;
#4042=EDGE_CURVE ( 'NONE', #36464, #12455, #11136, .T. ) ;
#4043=DIRECTION ( 'NONE',  ( -0.000000000000000000, -0.000000000000000000, -1.000000000000000000 ) ) ;
#4044=AXIS2_PLACEMENT_3D ( 'NONE', #2531, #22227, #19408 ) ;
#4045=AXIS2_PLACEMENT_3D ( 'NONE', #10683, #5244, #4882 ) ;
#4046=VECTOR ( 'NONE', #13956, 1000.000000000000000 ) ;
#4047=CARTESIAN_POINT ( 'NONE',  ( -70.00000337463099243, 34.64101615137758472, -9.999999999999998224 ) ) ;
#4048=ADVANCED_FACE ( 'NONE', ( #24848 ), #34039, .F. ) ;
#4049=CYLINDRICAL_SURFACE ( 'NONE', #19513, 2.000000000000000000 ) ;
#4051=DIRECTION ( 'NONE',  ( 1.000000000000000000, 0.000000000000000000, 0.000000000000000000 ) ) ;
#4052=VERTEX_POINT ( 'NONE', #31207 ) ;
#4053=FACE_BOUND ( 'NONE', #15529, .T. ) ;
#4055=DIRECTION ( 'NONE',  ( 1.000000000000000000, 0.000000000000000000, 0.000000000000000000 ) ) ;
#4056=CARTESIAN_POINT ( 'NONE',  ( 34.99999662536855283, -77.94228634059960825, 12.50000000000000000 ) ) ;
#4057=AXIS2_PLACEMENT_3D ( 'NONE', #18053, #3992, #12209 ) ;
#4060=DIRECTION ( 'NONE',  ( 0.000000000000000000, 0.000000000000000000, -1.000000000000000000 ) ) ;
#4061=AXIS2_PLACEMENT_3D ( 'NONE', #8555, #20525, #25635 ) ;
#4062=AXIS2_PLACEMENT_3D ( 'NONE', #14487, #22762, #17480 ) ;
#4064=AXIS2_PLACEMENT_3D ( 'NONE', #3606, #35992, #19121 ) ;
#4066=VECTOR ( 'NONE', #8336, 1000.000000000000000 ) ;
#4067=CARTESIAN_POINT ( 'NONE',  ( 81.99999662536833966, 34.64101615137759183, -5.000000000000000000 ) ) ;
#4072=DIRECTION ( 'NONE',  ( 0.000000000000000000, 0.000000000000000000, 1.000000000000000000 ) ) ;
#4073=EDGE_CURVE ( 'NONE', #24141, #16030, #15523, .T. ) ;
#4074=ORIENTED_EDGE ( 'NONE', *, *, #20665, .T. ) ;
#4075=VECTOR ( 'NONE', #19744, 1000.000000000000000 ) ;
#4076=ORIENTED_EDGE ( 'NONE', *, *, #35356, .T. ) ;
#4078=ORIENTED_EDGE ( 'NONE', *, *, #19516, .T. ) ;
#4079=FACE_OUTER_BOUND ( 'NONE', #13353, .T. ) ;
#4080=AXIS2_PLACEMENT_3D ( 'NONE', #11523, #9262, #22977 ) ;
#4082=EDGE_CURVE ( 'NONE', #6394, #10047, #4746, .T. ) ;
#4083=DIRECTION ( 'NONE',  ( 1.000000000000000000, 0.000000000000000000, 0.000000000000000000 ) ) ;
#4085=CARTESIAN_POINT ( 'NONE',  ( -62.00000337463104927, 51.96152422706639129, -5.000000000000000000 ) ) ;
#4087=EDGE_CURVE ( 'NONE', #17344, #26458, #23911, .T. ) ;
#4088=AXIS2_PLACEMENT_3D ( 'NONE', #27269, #9491, #30088 ) ;
#4089=CIRCLE ( 'NONE', #22665, 2.000000000000001776 ) ;
#4090=DIRECTION ( 'NONE',  ( 0.000000000000000000, 0.000000000000000000, 1.000000000000000000 ) ) ;
#4091=ORIENTED_EDGE ( 'NONE', *, *, #3219, .T. ) ;
#4092=CIRCLE ( 'NONE', #12451, 2.000000000000001776 ) ;
#4093=EDGE_LOOP ( 'NONE', ( #26561, #1331, #11056, #6068 ) ) ;
#4095=EDGE_CURVE ( 'NONE', #27467, #15817, #27484, .T. ) ;
#4097=DIRECTION ( 'NONE',  ( 1.000000000000000000, 0.000000000000000000, 0.000000000000000000 ) ) ;
#4098=ORIENTED_EDGE ( 'NONE', *, *, #20113, .T. ) ;
#4101=LINE ( 'NONE', #19904, #14693 ) ;
#4102=VECTOR ( 'NONE', #19017, 1000.000000000000000 ) ;
#4103=FACE_BOUND ( 'NONE', #9350, .T. ) ;
#4104=ORIENTED_EDGE ( 'NONE', *, *, #30013, .F. ) ;
#4105=VERTEX_POINT ( 'NONE', #1960 ) ;
#4106=CARTESIAN_POINT ( 'NONE',  ( 0.000000000000000000, 0.000000000000000000, 12.49999999999999822 ) ) ;
#4107=EDGE_LOOP ( 'NONE', ( #33160, #16781 ) ) ;
#4108=AXIS2_PLACEMENT_3D ( 'NONE', #13451, #7293, #33149 ) ;
#4110=CARTESIAN_POINT ( 'NONE',  ( 56.67878100130369035, -27.78182860042797131, 12.49999999999999822 ) ) ;
#4112=DIRECTION ( 'NONE',  ( 0.000000000000000000, 0.000000000000000000, 1.000000000000000000 ) ) ;
#4113=DIRECTION ( 'NONE',  ( 1.000000000000000000, 0.000000000000000000, 0.000000000000000000 ) ) ;
#4114=ORIENTED_EDGE ( 'NONE', *, *, #35127, .T. ) ;
#4117=EDGE_LOOP ( 'NONE', ( #2456, #10368 ) ) ;
#4118=EDGE_CURVE ( 'NONE', #20117, #14572, #13114, .T. ) ;
#4119=VERTEX_POINT ( 'NONE', #2147 ) ;
#4120=AXIS2_PLACEMENT_3D ( 'NONE', #18135, #15135, #3149 ) ;
#4121=ORIENTED_EDGE ( 'NONE', *, *, #8848, .T. ) ;
#4122=CYLINDRICAL_SURFACE ( 'NONE', #11039, 2.000000000000001776 ) ;
#4123=CIRCLE ( 'NONE', #5949, 2.000000000000001776 ) ;
#4124=EDGE_CURVE ( 'NONE', #32298, #30643, #10735, .T. ) ;
#4125=CYLINDRICAL_SURFACE ( 'NONE', #20374, 2.000000000000001776 ) ;
#4126=ORIENTED_EDGE ( 'NONE', *, *, #697, .F. ) ;
#4127=FACE_OUTER_BOUND ( 'NONE', #10182, .T. ) ;
#4129=CARTESIAN_POINT ( 'NONE',  ( 4.279621169095998212, -62.97617850287780072, 12.49999999999999822 ) ) ;
#4130=VECTOR ( 'NONE', #31116, 1000.000000000000000 ) ;
#4134=DIRECTION ( 'NONE',  ( -0.000000000000000000, -0.000000000000000000, 1.000000000000000000 ) ) ;
#4135=CARTESIAN_POINT ( 'NONE',  ( 89.99999662536828282, 0.000000000000000000, 12.50000000000000000 ) ) ;
#4136=ORIENTED_EDGE ( 'NONE', *, *, #16973, .F. ) ;
#4138=DIRECTION ( 'NONE',  ( 0.000000000000000000, 0.000000000000000000, 1.000000000000000000 ) ) ;
#4140=ORIENTED_EDGE ( 'NONE', *, *, #4319, .T. ) ;
#4143=EDGE_CURVE ( 'NONE', #7742, #14131, #27649, .T. ) ;
#4144=AXIS2_PLACEMENT_3D ( 'NONE', #17594, #905, #7468 ) ;
#4145=CARTESIAN_POINT ( 'NONE',  ( -35.19434990244938888, 52.39915983220783602, -4.999999999999997335 ) ) ;
#4147=DIRECTION ( 'NONE',  ( 1.000000000000000000, 0.000000000000000000, 0.000000000000000000 ) ) ;
#4148=ORIENTED_EDGE ( 'NONE', *, *, #1310, .F. ) ;
#4150=DIRECTION ( 'NONE',  ( 0.000000000000000000, 0.000000000000000000, -1.000000000000000000 ) ) ;
#4152=VERTEX_POINT ( 'NONE', #33658 ) ;
#4154=DIRECTION ( 'NONE',  ( 0.000000000000000000, 0.000000000000000000, 1.000000000000000000 ) ) ;
#4155=ORIENTED_EDGE ( 'NONE', *, *, #5133, .T. ) ;
#4156=CARTESIAN_POINT ( 'NONE',  ( -45.00000337463112743, -60.62177826491080168, -5.000000000000000000 ) ) ;
#4157=DIRECTION ( 'NONE',  ( 0.000000000000000000, 0.000000000000000000, 1.000000000000000000 ) ) ;
#4158=AXIS2_PLACEMENT_3D ( 'NONE', #14422, #31120, #11583 ) ;
#4159=EDGE_CURVE ( 'NONE', #21363, #36216, #7737, .T. ) ;
#4161=EDGE_LOOP ( 'NONE', ( #1708, #24531, #29476, #11004 ) ) ;
#4162=CIRCLE ( 'NONE', #6538, 2.000000000000000000 ) ;
#4163=ADVANCED_FACE ( 'NONE', ( #20134 ), #11504, .F. ) ;
#4165=EDGE_CURVE ( 'NONE', #22817, #32397, #17903, .T. ) ;
#4166=VECTOR ( 'NONE', #36030, 1000.000000000000000 ) ;
#4168=DIRECTION ( 'NONE',  ( 1.000000000000000000, 0.000000000000000000, 0.000000000000000000 ) ) ;
#4169=CIRCLE ( 'NONE', #27530, 2.000000000000001776 ) ;
#4170=DIRECTION ( 'NONE',  ( 0.000000000000000000, 0.000000000000000000, -1.000000000000000000 ) ) ;
#4171=EDGE_CURVE ( 'NONE', #12033, #8275, #5344, .T. ) ;
#4172=CYLINDRICAL_SURFACE ( 'NONE', #31011, 2.000000000000001776 ) ;
#4173=CARTESIAN_POINT ( 'NONE',  ( -35.19434990244938888, 52.39915983220783602, -4.999999999999997335 ) ) ;
#4174=FACE_OUTER_BOUND ( 'NONE', #6718, .T. ) ;
#4176=ORIENTED_EDGE ( 'NONE', *, *, #238, .T. ) ;
#4177=CARTESIAN_POINT ( 'NONE',  ( 69.99999662536838230, -51.96152422706639840, 12.50000000000000000 ) ) ;
#4178=CARTESIAN_POINT ( 'NONE',  ( -43.00000337463111322, 77.94228634059959404, -9.999999999999998224 ) ) ;
#4180=VERTEX_POINT ( 'NONE', #17682 ) ;
#4182=CARTESIAN_POINT ( 'NONE',  ( -35.00000337463116296, -60.62177826491080168, -9.999999999999998224 ) ) ;
#4183=DIRECTION ( 'NONE',  ( -1.000000000000000000, 8.737866397512802015E-15, 0.000000000000000000 ) ) ;
#4184=VECTOR ( 'NONE', #21104, 1000.000000000000000 ) ;
#4186=ORIENTED_EDGE ( 'NONE', *, *, #17058, .T. ) ;
#4187=ADVANCED_FACE ( 'NONE', ( #17499 ), #32105, .F. ) ;
#4190=EDGE_CURVE ( 'NONE', #32632, #3470, #32262, .T. ) ;
#4191=ADVANCED_FACE ( 'NONE', ( #28926 ), #9062, .T. ) ;
#4192=DIRECTION ( 'NONE',  ( 0.000000000000000000, 0.000000000000000000, -1.000000000000000000 ) ) ;
#4193=AXIS2_PLACEMENT_3D ( 'NONE', #26858, #10176, #21213 ) ;
#4194=DIRECTION ( 'NONE',  ( 0.000000000000000000, 0.000000000000000000, 1.000000000000000000 ) ) ;
#4195=CARTESIAN_POINT ( 'NONE',  ( 0.000000000000000000, 0.000000000000000000, -5.000000000000000000 ) ) ;
#4196=VERTEX_POINT ( 'NONE', #8518 ) ;
#4199=ORIENTED_EDGE ( 'NONE', *, *, #31119, .F. ) ;
#4200=DIRECTION ( 'NONE',  ( 0.000000000000000000, 0.000000000000000000, -1.000000000000000000 ) ) ;
#4201=AXIS2_PLACEMENT_3D ( 'NONE', #17519, #26153, #34241 ) ;
#4202=EDGE_LOOP ( 'NONE', ( #25482, #5938, #4975, #24808, #36574 ) ) ;
#4203=ORIENTED_EDGE ( 'NONE', *, *, #11586, .F. ) ;
#4204=CIRCLE ( 'NONE', #35378, 27.00000000000001421 ) ;
#4205=DIRECTION ( 'NONE',  ( -1.000000000000000000, 0.000000000000000000, 0.000000000000000000 ) ) ;
#4206=ORIENTED_EDGE ( 'NONE', *, *, #36000, .T. ) ;
#4207=ORIENTED_EDGE ( 'NONE', *, *, #21309, .F. ) ;
#4208=CARTESIAN_POINT ( 'NONE',  ( 89.99999662536828282, 0.000000000000000000, -5.000000000000000000 ) ) ;
#4209=CARTESIAN_POINT ( 'NONE',  ( -18.00000337463123756, -69.28203230275522628, -9.999999999999998224 ) ) ;
#4211=EDGE_LOOP ( 'NONE', ( #23698, #1469, #4926, #31837, #5298, #11673 ) ) ;
#4212=DIRECTION ( 'NONE',  ( 0.000000000000000000, 0.000000000000000000, 1.000000000000000000 ) ) ;
#4215=DIRECTION ( 'NONE',  ( 1.000000000000000000, 0.000000000000000000, 0.000000000000000000 ) ) ;
#4217=VERTEX_POINT ( 'NONE', #12041 ) ;
#4218=CYLINDRICAL_SURFACE ( 'NONE', #15343, 2.000000000000001776 ) ;
#4219=ORIENTED_EDGE ( 'NONE', *, *, #851, .T. ) ;
#4222=FACE_OUTER_BOUND ( 'NONE', #17842, .T. ) ;
#4224=CARTESIAN_POINT ( 'NONE',  ( 69.99999662536838230, -34.64101615137759183, 12.50000000000000000 ) ) ;
#4225=DIRECTION ( 'NONE',  ( 0.000000000000000000, 0.000000000000000000, -1.000000000000000000 ) ) ;
#4227=DIRECTION ( 'NONE',  ( -0.000000000000000000, 0.000000000000000000, -1.000000000000000000 ) ) ;
#4228=AXIS2_PLACEMENT_3D ( 'NONE', #26769, #1085, #11957 ) ;
#4231=DIRECTION ( 'NONE',  ( 1.000000000000000000, 0.000000000000000000, 0.000000000000000000 ) ) ;
#4232=CYLINDRICAL_SURFACE ( 'NONE', #354, 2.000000000000001776 ) ;
#4235=VERTEX_POINT ( 'NONE', #5702 ) ;
#4236=ORIENTED_EDGE ( 'NONE', *, *, #7965, .T. ) ;
#4239=DIRECTION ( 'NONE',  ( 1.000000000000000000, 0.000000000000000000, 0.000000000000000000 ) ) ;
#4241=AXIS2_PLACEMENT_3D ( 'NONE', #23876, #14871, #18218 ) ;
#4242=ORIENTED_EDGE ( 'NONE', *, *, #4384, .T. ) ;
#4243=CARTESIAN_POINT ( 'NONE',  ( -55.88972745734202618, -33.99999999999965894, -4.999999999999997335 ) ) ;
#4244=CARTESIAN_POINT ( 'NONE',  ( -10.00000337463125000, -86.60254037844400443, 12.50000000000000000 ) ) ;
#4245=VERTEX_POINT ( 'NONE', #20674 ) ;
#4246=CARTESIAN_POINT ( 'NONE',  ( -62.33939050065184517, 13.89091430021398565, 12.49999999999999822 ) ) ;
#4247=ORIENTED_EDGE ( 'NONE', *, *, #1221, .F. ) ;
#4248=DIRECTION ( 'NONE',  ( -1.000000000000000000, 0.000000000000000000, 0.000000000000000000 ) ) ;
#4251=DIRECTION ( 'NONE',  ( -0.000000000000000000, -0.000000000000000000, -1.000000000000000000 ) ) ;
#4252=ORIENTED_EDGE ( 'NONE', *, *, #18480, .T. ) ;
#4254=EDGE_CURVE ( 'NONE', #16375, #21830, #9237, .T. ) ;
#4256=EDGE_CURVE ( 'NONE', #34663, #13150, #4123, .T. ) ;
#4258=DIRECTION ( 'NONE',  ( 1.000000000000000000, 0.000000000000000000, 0.000000000000000000 ) ) ;
#4259=FACE_OUTER_BOUND ( 'NONE', #232, .T. ) ;
#4260=ORIENTED_EDGE ( 'NONE', *, *, #3843, .F. ) ;
#4262=FACE_OUTER_BOUND ( 'NONE', #21189, .T. ) ;
#4263=DIRECTION ( 'NONE',  ( 0.000000000000000000, 0.000000000000000000, 1.000000000000000000 ) ) ;
#4264=EDGE_CURVE ( 'NONE', #30055, #3619, #14335, .T. ) ;
#4265=ORIENTED_EDGE ( 'NONE', *, *, #34788, .F. ) ;
#4267=ORIENTED_EDGE ( 'NONE', *, *, #17535, .T. ) ;
#4268=CARTESIAN_POINT ( 'NONE',  ( -55.00000337463109901, -60.62177826491083010, -9.999999999999998224 ) ) ;
#4269=CARTESIAN_POINT ( 'NONE',  ( 27.99999662536857414, -69.28203230275519786, -9.999999999999998224 ) ) ;
#4271=EDGE_LOOP ( 'NONE', ( #9312, #31055, #8524, #234 ) ) ;
#4273=CYLINDRICAL_SURFACE ( 'NONE', #8610, 33.00000000000001421 ) ;
#4274=DIRECTION ( 'NONE',  ( -0.000000000000000000, 0.000000000000000000, -1.000000000000000000 ) ) ;
#4275=DIRECTION ( 'NONE',  ( 1.000000000000000000, 0.000000000000000000, 0.000000000000000000 ) ) ;
#4278=ORIENTED_EDGE ( 'NONE', *, *, #30046, .T. ) ;
#4279=FACE_OUTER_BOUND ( 'NONE', #26180, .T. ) ;
#4280=CARTESIAN_POINT ( 'NONE',  ( 21.99999662536862033, -69.28203230275519786, 12.50000000000000000 ) ) ;
#4281=EDGE_LOOP ( 'NONE', ( #11633, #25273, #21587, #13740 ) ) ;
#4282=DIRECTION ( 'NONE',  ( 0.000000000000000000, 0.000000000000000000, -1.000000000000000000 ) ) ;
#4283=ORIENTED_EDGE ( 'NONE', *, *, #18796, .F. ) ;
#4284=DIRECTION ( 'NONE',  ( 0.000000000000000000, 0.000000000000000000, 1.000000000000000000 ) ) ;
#4285=FACE_BOUND ( 'NONE', #25163, .T. ) ;
#4286=ORIENTED_EDGE ( 'NONE', *, *, #19810, .T. ) ;
#4287=EDGE_LOOP ( 'NONE', ( #14624, #18513 ) ) ;
#4288=EDGE_CURVE ( 'NONE', #36402, #12408, #16124, .T. ) ;
#4289=CYLINDRICAL_SURFACE ( 'NONE', #28418, 2.000000000000001776 ) ;
#4290=VERTEX_POINT ( 'NONE', #28377 ) ;
#4293=CARTESIAN_POINT ( 'NONE',  ( 74.99999662536835388, -25.98076211353319565, -9.999999999999998224 ) ) ;
#4294=DIRECTION ( 'NONE',  ( 0.000000000000000000, 0.000000000000000000, 1.000000000000000000 ) ) ;
#4295=ORIENTED_EDGE ( 'NONE', *, *, #14257, .F. ) ;
#4296=DIRECTION ( 'NONE',  ( 0.000000000000000000, 0.000000000000000000, 1.000000000000000000 ) ) ;
#4297=EDGE_CURVE ( 'NONE', #17677, #6217, #37030, .T. ) ;
#4298=DIRECTION ( 'NONE',  ( 0.000000000000000000, 0.000000000000000000, 1.000000000000000000 ) ) ;
#4299=ORIENTED_EDGE ( 'NONE', *, *, #24390, .F. ) ;
#4300=ORIENTED_EDGE ( 'NONE', *, *, #4474, .T. ) ;
#4301=ADVANCED_FACE ( 'NONE', ( #11871 ), #23328, .F. ) ;
#4302=ORIENTED_EDGE ( 'NONE', *, *, #21889, .T. ) ;
#4303=CARTESIAN_POINT ( 'NONE',  ( -18.03953374218250971, 86.20686523360116382, -5.000000000000000000 ) ) ;
#4306=ORIENTED_EDGE ( 'NONE', *, *, #19034, .F. ) ;
#4307=AXIS2_PLACEMENT_3D ( 'NONE', #23274, #190, #22901 ) ;
#4308=DIRECTION ( 'NONE',  ( 0.000000000000000000, 0.000000000000000000, -1.000000000000000000 ) ) ;
#4309=CARTESIAN_POINT ( 'NONE',  ( -80.00000337463094979, 17.32050807568878525, -9.999999999999998224 ) ) ;
#4312=CYLINDRICAL_SURFACE ( 'NONE', #1258, 2.000000000000001776 ) ;
#4313=DIRECTION ( 'NONE',  ( 0.000000000000000000, 0.000000000000000000, 1.000000000000000000 ) ) ;
#4314=DIRECTION ( 'NONE',  ( 0.000000000000000000, 0.000000000000000000, -1.000000000000000000 ) ) ;
#4315=DIRECTION ( 'NONE',  ( 0.000000000000000000, 0.000000000000000000, 1.000000000000000000 ) ) ;
#4316=CARTESIAN_POINT ( 'NONE',  ( 62.99999662536839651, 60.62177826491078747, -5.000000000000000000 ) ) ;
#4317=ORIENTED_EDGE ( 'NONE', *, *, #14862, .F. ) ;
#4318=VERTEX_POINT ( 'NONE', #12781 ) ;
#4319=EDGE_CURVE ( 'NONE', #25810, #12047, #34672, .T. ) ;
#4320=CARTESIAN_POINT ( 'NONE',  ( -52.00000337463110611, -69.28203230275519786, -9.999999999999998224 ) ) ;
#4321=DIRECTION ( 'NONE',  ( 0.000000000000000000, 0.000000000000000000, 1.000000000000000000 ) ) ;
#4322=FACE_OUTER_BOUND ( 'NONE', #15200, .T. ) ;
#4323=CARTESIAN_POINT ( 'NONE',  ( 22.99999662536859901, -77.94228634059960825, 12.50000000000000000 ) ) ;
#4324=ORIENTED_EDGE ( 'NONE', *, *, #734, .F. ) ;
#4326=EDGE_CURVE ( 'NONE', #20492, #27413, #25099, .T. ) ;
#4328=CARTESIAN_POINT ( 'NONE',  ( 7.999996625368656744, -86.60254037844400443, 17.49999999999999645 ) ) ;
#4329=ORIENTED_EDGE ( 'NONE', *, *, #11175, .F. ) ;
#4330=CIRCLE ( 'NONE', #21692, 27.00000000000001421 ) ;
#4332=CARTESIAN_POINT ( 'NONE',  ( 0.000000000000000000, 0.000000000000000000, -5.000000000000000000 ) ) ;
#4333=EDGE_LOOP ( 'NONE', ( #24062, #32598 ) ) ;
#4334=LINE ( 'NONE', #18402, #6126 ) ;
#4335=DIRECTION ( 'NONE',  ( 1.000000000000000000, 0.000000000000000000, 0.000000000000000000 ) ) ;
#4336=CARTESIAN_POINT ( 'NONE',  ( -3.000003374631269981, -77.94228634059960825, 17.49999999999999645 ) ) ;
#4337=ORIENTED_EDGE ( 'NONE', *, *, #2751, .T. ) ;
#4338=ORIENTED_EDGE ( 'NONE', *, *, #13797, .T. ) ;
#4340=AXIS2_PLACEMENT_3D ( 'NONE', #14828, #3754, #32041 ) ;
#4341=EDGE_CURVE ( 'NONE', #27983, #10548, #6525, .T. ) ;
#4342=EDGE_LOOP ( 'NONE', ( #28730, #27086, #8884, #32843, #32594 ) ) ;
#4344=FACE_BOUND ( 'NONE', #14014, .T. ) ;
#4345=CARTESIAN_POINT ( 'NONE',  ( -75.00000337463097821, 8.660254037844374864, -5.000000000000000000 ) ) ;
#4347=DIRECTION ( 'NONE',  ( 0.000000000000000000, 0.000000000000000000, 1.000000000000000000 ) ) ;
#4348=ORIENTED_EDGE ( 'NONE', *, *, #16881, .F. ) ;
#4349=DIRECTION ( 'NONE',  ( 0.000000000000000000, 0.000000000000000000, 1.000000000000000000 ) ) ;
#4350=DIRECTION ( 'NONE',  ( 0.000000000000000000, 0.000000000000000000, 1.000000000000000000 ) ) ;
#4351=DIRECTION ( 'NONE',  ( 0.000000000000000000, 0.000000000000000000, -1.000000000000000000 ) ) ;
#4353=CARTESIAN_POINT ( 'NONE',  ( 84.99999662536831124, -8.660254037844397956, -9.999999999999998224 ) ) ;
#4354=CARTESIAN_POINT ( 'NONE',  ( -82.00000337463094979, 34.64101615137757051, -9.999999999999998224 ) ) ;
#4355=VERTEX_POINT ( 'NONE', #32875 ) ;
#4356=ORIENTED_EDGE ( 'NONE', *, *, #14523, .F. ) ;
#4357=EDGE_CURVE ( 'NONE', #29261, #36951, #802, .T. ) ;
#4358=CARTESIAN_POINT ( 'NONE',  ( -23.00000337463120559, 77.94228634059957983, -9.999999999999998224 ) ) ;
#4359=CARTESIAN_POINT ( 'NONE',  ( -57.00000337463111322, -43.30127018922202353, -5.000000000000000000 ) ) ;
#4360=EDGE_CURVE ( 'NONE', #14063, #26676, #8333, .T. ) ;
#4362=ORIENTED_EDGE ( 'NONE', *, *, #34337, .F. ) ;
#4364=ORIENTED_EDGE ( 'NONE', *, *, #23902, .T. ) ;
#4365=EDGE_CURVE ( 'NONE', #5993, #12630, #14318, .T. ) ;
#4366=DIRECTION ( 'NONE',  ( 0.000000000000000000, 0.000000000000000000, 1.000000000000000000 ) ) ;
#4367=AXIS2_PLACEMENT_3D ( 'NONE', #29257, #31860, #20441 ) ;
#4368=ORIENTED_EDGE ( 'NONE', *, *, #10515, .T. ) ;
#4371=FACE_BOUND ( 'NONE', #13107, .T. ) ;
#4372=ORIENTED_EDGE ( 'NONE', *, *, #19297, .T. ) ;
#4373=EDGE_CURVE ( 'NONE', #6775, #29382, #8107, .T. ) ;
#4374=ORIENTED_EDGE ( 'NONE', *, *, #27980, .F. ) ;
#4375=DIRECTION ( 'NONE',  ( -1.000000000000000000, 0.000000000000000000, 0.000000000000000000 ) ) ;
#4376=CIRCLE ( 'NONE', #16953, 2.000000000000001776 ) ;
#4377=DIRECTION ( 'NONE',  ( 1.000000000000000000, 0.000000000000000000, 0.000000000000000000 ) ) ;
#4378=ORIENTED_EDGE ( 'NONE', *, *, #12635, .F. ) ;
#4379=ORIENTED_EDGE ( 'NONE', *, *, #2258, .T. ) ;
#4380=DIRECTION ( 'NONE',  ( 0.000000000000000000, 0.000000000000000000, 1.000000000000000000 ) ) ;
#4381=CARTESIAN_POINT ( 'NONE',  ( -68.00000337463099243, 17.32050807568877460, 12.50000000000000000 ) ) ;
#4382=ADVANCED_FACE ( 'NONE', ( #33051 ), #12213, .F. ) ;
#4384=EDGE_CURVE ( 'NONE', #10733, #13581, #27262, .T. ) ;
#4385=CARTESIAN_POINT ( 'NONE',  ( 69.99999662536839651, 34.64101615137758472, -9.999999999999998224 ) ) ;
#4386=ADVANCED_FACE ( 'NONE', ( #996 ), #21434, .F. ) ;
#4387=EDGE_LOOP ( 'NONE', ( #20606, #16740, #34539, #1841, #12519, #27487, #21851, #31216, #21093, #3175, #33503, #28793, #8810, #16944, #10907, #34125, #10500, #894, #6028, #24981, #2421, #4699, #6332, #30781 ) ) ;
#4389=ADVANCED_FACE ( 'NONE', ( #29310 ), #32669, .F. ) ;
#4391=FACE_OUTER_BOUND ( 'NONE', #2022, .T. ) ;
#4392=ADVANCED_FACE ( 'NONE', ( #18058 ), #9632, .F. ) ;
#4393=CARTESIAN_POINT ( 'NONE',  ( -56.67878100130369035, 27.78182860042797131, -4.999999999999997335 ) ) ;
#4394=CYLINDRICAL_SURFACE ( 'NONE', #6420, 2.000000000000001776 ) ;
#4395=CARTESIAN_POINT ( 'NONE',  ( -70.00000337463099243, 34.64101615137758472, -5.000000000000000000 ) ) ;
#4397=CIRCLE ( 'NONE', #9160, 33.00000000000001421 ) ;
#4399=CARTESIAN_POINT ( 'NONE',  ( -13.00000337463125710, -77.94228634059960825, -9.999999999999998224 ) ) ;
#4403=DIRECTION ( 'NONE',  ( -1.000000000000000000, 0.000000000000000000, 0.000000000000000000 ) ) ;
#4404=CIRCLE ( 'NONE', #33136, 2.000000000000001776 ) ;
#4405=ORIENTED_EDGE ( 'NONE', *, *, #12561, .T. ) ;
#4406=ORIENTED_EDGE ( 'NONE', *, *, #11948, .T. ) ;
#4407=VERTEX_POINT ( 'NONE', #29665 ) ;
#4413=CIRCLE ( 'NONE', #34948, 1.999999999999998224 ) ;
#4414=DIRECTION ( 'NONE',  ( 0.000000000000000000, 0.000000000000000000, 1.000000000000000000 ) ) ;
#4415=DIRECTION ( 'NONE',  ( 0.000000000000000000, 0.000000000000000000, -1.000000000000000000 ) ) ;
#4416=ORIENTED_EDGE ( 'NONE', *, *, #7937, .F. ) ;
#4417=CARTESIAN_POINT ( 'NONE',  ( -32.49191361593891969, -89.27079897466117586, -5.000000000000000000 ) ) ;
#4418=EDGE_LOOP ( 'NONE', ( #36820, #36692 ) ) ;
#4419=DIRECTION ( 'NONE',  ( 1.000000000000000000, 0.000000000000000000, 0.000000000000000000 ) ) ;
#4421=CIRCLE ( 'NONE', #24193, 2.000000000000000000 ) ;
#4424=DIRECTION ( 'NONE',  ( 0.000000000000000000, 0.000000000000000000, 1.000000000000000000 ) ) ;
#4426=FACE_OUTER_BOUND ( 'NONE', #31737, .T. ) ;
#4428=AXIS2_PLACEMENT_3D ( 'NONE', #6090, #36844, #19968 ) ;
#4429=DIRECTION ( 'NONE',  ( -1.000000000000000000, 0.000000000000000000, 0.000000000000000000 ) ) ;
#4431=EDGE_CURVE ( 'NONE', #33934, #8519, #3997, .T. ) ;
#4433=EDGE_CURVE ( 'NONE', #15350, #36079, #30777, .T. ) ;
#4434=DIRECTION ( 'NONE',  ( -1.000000000000000000, 0.000000000000000000, 0.000000000000000000 ) ) ;
#4435=DIRECTION ( 'NONE',  ( 1.000000000000000000, 0.000000000000000000, 0.000000000000000000 ) ) ;
#4436=EDGE_CURVE ( 'NONE', #28556, #16244, #25191, .T. ) ;
#4437=ORIENTED_EDGE ( 'NONE', *, *, #26850, .F. ) ;
#4439=DIRECTION ( 'NONE',  ( 0.000000000000000000, 0.000000000000000000, 1.000000000000000000 ) ) ;
#4442=VERTEX_POINT ( 'NONE', #2302 ) ;
#4443=DIRECTION ( 'NONE',  ( -0.000000000000000000, 0.000000000000000000, -1.000000000000000000 ) ) ;
#4444=CYLINDRICAL_SURFACE ( 'NONE', #3983, 2.000000000000001776 ) ;
#4447=ORIENTED_EDGE ( 'NONE', *, *, #16696, .T. ) ;
#4448=DIRECTION ( 'NONE',  ( -0.000000000000000000, -0.000000000000000000, 1.000000000000000000 ) ) ;
#4452=ADVANCED_FACE ( 'NONE', ( #4755 ), #7745, .F. ) ;
#4453=VERTEX_POINT ( 'NONE', #24806 ) ;
#4454=AXIS2_PLACEMENT_3D ( 'NONE', #8067, #8261, #36398 ) ;
#4456=CARTESIAN_POINT ( 'NONE',  ( -85.00000337463092137, 8.660254037844389075, 17.49999999999999645 ) ) ;
#4459=ORIENTED_EDGE ( 'NONE', *, *, #4431, .T. ) ;
#4460=DIRECTION ( 'NONE',  ( 0.000000000000000000, 0.000000000000000000, 1.000000000000000000 ) ) ;
#4462=CARTESIAN_POINT ( 'NONE',  ( 49.99999662536846756, -69.28203230275519786, 12.50000000000000000 ) ) ;
#4463=EDGE_CURVE ( 'NONE', #6532, #21999, #8101, .T. ) ;
#4464=FACE_OUTER_BOUND ( 'NONE', #34578, .T. ) ;
#4465=EDGE_LOOP ( 'NONE', ( #2968, #15473 ) ) ;
#4466=ORIENTED_EDGE ( 'NONE', *, *, #3237, .T. ) ;
#4467=AXIS2_PLACEMENT_3D ( 'NONE', #11600, #8620, #34701 ) ;
#4468=DIRECTION ( 'NONE',  ( 0.000000000000000000, 0.000000000000000000, 1.000000000000000000 ) ) ;
#4469=ORIENTED_EDGE ( 'NONE', *, *, #22483, .T. ) ;
#4471=DIRECTION ( 'NONE',  ( -1.000000000000000000, 0.000000000000000000, 0.000000000000000000 ) ) ;
#4473=DIRECTION ( 'NONE',  ( 0.000000000000000000, 0.000000000000000000, 1.000000000000000000 ) ) ;
#4474=EDGE_CURVE ( 'NONE', #3626, #30390, #25477, .T. ) ;
#4476=LINE ( 'NONE', #24913, #29222 ) ;
#4477=FACE_OUTER_BOUND ( 'NONE', #5518, .T. ) ;
#4480=CIRCLE ( 'NONE', #6850, 2.000000000000001776 ) ;
#4482=ORIENTED_EDGE ( 'NONE', *, *, #29871, .T. ) ;
#4483=CARTESIAN_POINT ( 'NONE',  ( -70.00000337463099243, 34.64101615137758472, -9.999999999999998224 ) ) ;
#4484=CIRCLE ( 'NONE', #30135, 3.000000000000002665 ) ;
#4485=CYLINDRICAL_SURFACE ( 'NONE', #35395, 33.00000000000001421 ) ;
#4486=EDGE_LOOP ( 'NONE', ( #32721, #6364 ) ) ;
#4487=DIRECTION ( 'NONE',  ( 1.000000000000000000, 0.000000000000000000, 0.000000000000000000 ) ) ;
#4488=FACE_OUTER_BOUND ( 'NONE', #18027, .T. ) ;
#4489=DIRECTION ( 'NONE',  ( -1.000000000000000000, 0.000000000000000000, 0.000000000000000000 ) ) ;
#4490=CARTESIAN_POINT ( 'NONE',  ( 19.99999662536861678, -69.28203230275519786, -9.999999999999998224 ) ) ;
#4491=AXIS2_PLACEMENT_3D ( 'NONE', #29042, #31491, #565 ) ;
#4492=EDGE_CURVE ( 'NONE', #26329, #20328, #36277, .T. ) ;
#4493=CARTESIAN_POINT ( 'NONE',  ( -18.00000337463123756, -69.28203230275522628, 17.49999999999999645 ) ) ;
#4495=CIRCLE ( 'NONE', #2724, 2.000000000000001776 ) ;
#4497=EDGE_CURVE ( 'NONE', #32590, #22230, #20091, .T. ) ;
#4498=LINE ( 'NONE', #13678, #23232 ) ;
#4499=ORIENTED_EDGE ( 'NONE', *, *, #7872, .T. ) ;
#4501=ORIENTED_EDGE ( 'NONE', *, *, #11952, .F. ) ;
#4502=FACE_OUTER_BOUND ( 'NONE', #10821, .T. ) ;
#4503=DIRECTION ( 'NONE',  ( 1.000000000000000000, 0.000000000000000000, 0.000000000000000000 ) ) ;
#4504=DIRECTION ( 'NONE',  ( 1.000000000000000000, 0.000000000000000000, 0.000000000000000000 ) ) ;
#4505=LINE ( 'NONE', #15943, #20910 ) ;
#4506=EDGE_CURVE ( 'NONE', #16313, #10822, #22472, .T. ) ;
#4507=ORIENTED_EDGE ( 'NONE', *, *, #11193, .T. ) ;
#4508=AXIS2_PLACEMENT_3D ( 'NONE', #12488, #18509, #13237 ) ;
#4509=DIRECTION ( 'NONE',  ( -0.5000000000000101030, -0.8660254037844328234, 0.000000000000000000 ) ) ;
#4510=AXIS2_PLACEMENT_3D ( 'NONE', #14346, #16109, #34403 ) ;
#4511=CARTESIAN_POINT ( 'NONE',  ( 14.99999662536859901, 77.94228634059957983, -9.999999999999998224 ) ) ;
#4512=ADVANCED_FACE ( 'NONE', ( #19357, #22348, #7921, #30427, #16550, #15997, #33792, #21988, #27428 ), #16744, .F. ) ;
#4513=LINE ( 'NONE', #16322, #19791 ) ;
#4515=DIRECTION ( 'NONE',  ( 0.000000000000000000, 0.000000000000000000, -1.000000000000000000 ) ) ;
#4517=( LENGTH_UNIT ( ) NAMED_UNIT ( * ) SI_UNIT ( .MILLI., .METRE. ) );
#4518=DIRECTION ( 'NONE',  ( 0.000000000000000000, 0.000000000000000000, -1.000000000000000000 ) ) ;
#4519=DIRECTION ( 'NONE',  ( 0.000000000000000000, 0.000000000000000000, 1.000000000000000000 ) ) ;
#4520=CIRCLE ( 'NONE', #14083, 65.00000000000000000 ) ;
#4521=CARTESIAN_POINT ( 'NONE',  ( -20.00000337463122690, 86.60254037844397601, 17.49999999999999645 ) ) ;
#4522=EDGE_CURVE ( 'NONE', #6764, #23686, #17679, .T. ) ;
#4523=ORIENTED_EDGE ( 'NONE', *, *, #19403, .F. ) ;
#4524=AXIS2_PLACEMENT_3D ( 'NONE', #7221, #24469, #35910 ) ;
#4525=ORIENTED_EDGE ( 'NONE', *, *, #9686, .T. ) ;
#4527=AXIS2_PLACEMENT_3D ( 'NONE', #7093, #20968, #6711 ) ;
#4528=VECTOR ( 'NONE', #24534, 1000.000000000000000 ) ;
#4529=ORIENTED_EDGE ( 'NONE', *, *, #27213, .T. ) ;
#4531=FACE_BOUND ( 'NONE', #26683, .T. ) ;
#4533=DIRECTION ( 'NONE',  ( 0.000000000000000000, 0.000000000000000000, -1.000000000000000000 ) ) ;
#4534=DIRECTION ( 'NONE',  ( 1.000000000000000000, 0.000000000000000000, 0.000000000000000000 ) ) ;
#4535=ORIENTED_EDGE ( 'NONE', *, *, #381, .F. ) ;
#4536=CARTESIAN_POINT ( 'NONE',  ( -2.374207310413330682E-13, -68.00000000000000000, -4.999999999999997335 ) ) ;
#4537=EDGE_CURVE ( 'NONE', #9991, #23102, #15301, .T. ) ;
#4538=AXIS2_PLACEMENT_3D ( 'NONE', #9318, #9879, #15134 ) ;
#4539=CARTESIAN_POINT ( 'NONE',  ( 11.99999662536865763, -86.60254037844400443, 12.50000000000000000 ) ) ;
#4540=EDGE_CURVE ( 'NONE', #29798, #21959, #24900, .T. ) ;
#4541=FILL_AREA_STYLE_COLOUR ( '', #36762 ) ;
#4543=DIRECTION ( 'NONE',  ( 0.000000000000000000, 0.000000000000000000, 1.000000000000000000 ) ) ;
#4544=DIRECTION ( 'NONE',  ( 1.000000000000000000, 0.000000000000000000, 0.000000000000000000 ) ) ;
#4545=EDGE_LOOP ( 'NONE', ( #25726, #15749 ) ) ;
#4546=ORIENTED_EDGE ( 'NONE', *, *, #35788, .T. ) ;
#4547=VECTOR ( 'NONE', #19572, 1000.000000000000000 ) ;
#4548=FACE_OUTER_BOUND ( 'NONE', #26012, .T. ) ;
#4550=AXIS2_PLACEMENT_3D ( 'NONE', #19886, #15, #8284 ) ;
#4551=CARTESIAN_POINT ( 'NONE',  ( 62.99999662536841072, 25.98076211353318854, -5.000000000000000000 ) ) ;
#4552=ADVANCED_FACE ( 'NONE', ( #7363 ), #36436, .F. ) ;
#4553=ORIENTED_EDGE ( 'NONE', *, *, #23539, .F. ) ;
#4554=EDGE_LOOP ( 'NONE', ( #24738, #8548 ) ) ;
#4555=AXIS2_PLACEMENT_3D ( 'NONE', #34122, #25132, #28109 ) ;
#4557=CIRCLE ( 'NONE', #18925, 2.000000000000001776 ) ;
#4558=AXIS2_PLACEMENT_3D ( 'NONE', #4244, #6495, #20929 ) ;
#4559=CIRCLE ( 'NONE', #33296, 3.000000000000002665 ) ;
#4562=ORIENTED_EDGE ( 'NONE', *, *, #32948, .F. ) ;
#4563=DIRECTION ( 'NONE',  ( 0.000000000000000000, 0.000000000000000000, 1.000000000000000000 ) ) ;
#4564=AXIS2_PLACEMENT_3D ( 'NONE', #30674, #7993, #36684 ) ;
#4565=ORIENTED_EDGE ( 'NONE', *, *, #18622, .F. ) ;
#4566=VERTEX_POINT ( 'NONE', #7550 ) ;
#4567=CIRCLE ( 'NONE', #35102, 3.000000000000002665 ) ;
#4568=CARTESIAN_POINT ( 'NONE',  ( -48.00000337463109190, 69.28203230275518365, -5.000000000000000000 ) ) ;
#4569=CARTESIAN_POINT ( 'NONE',  ( -58.00000337463104216, 51.96152422706639129, -5.000000000000000000 ) ) ;
#4572=DIRECTION ( 'NONE',  ( 0.000000000000000000, 0.000000000000000000, 1.000000000000000000 ) ) ;
#4575=DIRECTION ( 'NONE',  ( 0.000000000000000000, 0.000000000000000000, -1.000000000000000000 ) ) ;
#4578=CARTESIAN_POINT ( 'NONE',  ( -85.00000337463092137, -25.98076211353322051, 17.49999999999999645 ) ) ;
#4581=DIRECTION ( 'NONE',  ( 0.000000000000000000, 0.000000000000000000, -1.000000000000000000 ) ) ;
#4582=FACE_BOUND ( 'NONE', #31237, .T. ) ;
#4584=CIRCLE ( 'NONE', #2192, 3.000000000000002665 ) ;
#4587=CARTESIAN_POINT ( 'NONE',  ( -30.00000337463119848, -69.28203230275522628, 12.50000000000000000 ) ) ;
#4588=ADVANCED_FACE ( 'NONE', ( #25540 ), #198, .F. ) ;
#4589=AXIS2_PLACEMENT_3D ( 'NONE', #16178, #7354, #35496 ) ;
#4590=AXIS2_PLACEMENT_3D ( 'NONE', #25840, #17015, #129 ) ;
#4591=CARTESIAN_POINT ( 'NONE',  ( -70.00000337463099243, 51.96152422706637708, -5.000000000000000000 ) ) ;
#4592=EDGE_CURVE ( 'NONE', #11580, #23569, #23280, .T. ) ;
#4594=ORIENTED_EDGE ( 'NONE', *, *, #4165, .T. ) ;
#4595=DIRECTION ( 'NONE',  ( -1.000000000000000000, 0.000000000000000000, 0.000000000000000000 ) ) ;
#4597=DIRECTION ( 'NONE',  ( 0.000000000000000000, 0.000000000000000000, 1.000000000000000000 ) ) ;
#4598=DIRECTION ( 'NONE',  ( 0.000000000000000000, 0.000000000000000000, 1.000000000000000000 ) ) ;
#4600=CIRCLE ( 'NONE', #25546, 27.00000000000001421 ) ;
#4601=EDGE_LOOP ( 'NONE', ( #22253, #28291, #24183, #9520 ) ) ;
#4604=CARTESIAN_POINT ( 'NONE',  ( 59.99999662536843914, -34.64101615137759893, -9.999999999999998224 ) ) ;
#4605=ORIENTED_EDGE ( 'NONE', *, *, #19753, .T. ) ;
#4606=CARTESIAN_POINT ( 'NONE',  ( -52.39915983220772233, -35.19434990244957362, -4.999999999999997335 ) ) ;
#4607=EDGE_CURVE ( 'NONE', #4052, #8893, #15898, .T. ) ;
#4608=CIRCLE ( 'NONE', #4005, 2.000000000000001776 ) ;
#4611=DIRECTION ( 'NONE',  ( 1.000000000000000000, -0.000000000000000000, 0.000000000000000000 ) ) ;
#4612=VERTEX_POINT ( 'NONE', #23081 ) ;
#4614=FACE_BOUND ( 'NONE', #7088, .T. ) ;
#4615=VECTOR ( 'NONE', #12014, 1000.000000000000000 ) ;
#4616=AXIS2_PLACEMENT_3D ( 'NONE', #371, #26262, #34717 ) ;
#4618=DIRECTION ( 'NONE',  ( 1.000000000000000000, 0.000000000000000000, 0.000000000000000000 ) ) ;
#4619=DIRECTION ( 'NONE',  ( 1.000000000000000000, 0.000000000000000000, 0.000000000000000000 ) ) ;
#4620=DIRECTION ( 'NONE',  ( 0.000000000000000000, 0.000000000000000000, 1.000000000000000000 ) ) ;
#4621=VERTEX_POINT ( 'NONE', #31868 ) ;
#4622=DIRECTION ( 'NONE',  ( 0.000000000000000000, 0.000000000000000000, 1.000000000000000000 ) ) ;
#4623=CIRCLE ( 'NONE', #19584, 2.000000000000001776 ) ;
#4625=CYLINDRICAL_SURFACE ( 'NONE', #5598, 2.000000000000000000 ) ;
#4628=CARTESIAN_POINT ( 'NONE',  ( -2.000003374631303732, -86.60254037844400443, -5.000000000000000000 ) ) ;
#4629=ORIENTED_EDGE ( 'NONE', *, *, #32560, .F. ) ;
#4630=EDGE_CURVE ( 'NONE', #7478, #3872, #921, .T. ) ;
#4631=DIRECTION ( 'NONE',  ( 1.000000000000000000, 0.000000000000000000, 0.000000000000000000 ) ) ;
#4632=AXIS2_PLACEMENT_3D ( 'NONE', #23357, #20349, #28949 ) ;
#4634=CARTESIAN_POINT ( 'NONE',  ( -3.000003374631308173, 77.94228634059957983, 12.50000000000000000 ) ) ;
#4638=ORIENTED_EDGE ( 'NONE', *, *, #12629, .F. ) ;
#4639=EDGE_CURVE ( 'NONE', #2266, #126, #35061, .T. ) ;
#4640=DIRECTION ( 'NONE',  ( 0.000000000000000000, 0.000000000000000000, 1.000000000000000000 ) ) ;
#4641=FACE_OUTER_BOUND ( 'NONE', #30345, .T. ) ;
#4642=CARTESIAN_POINT ( 'NONE',  ( -73.00000337463100664, -43.30127018922202353, -5.000000000000000000 ) ) ;
#4643=AXIS2_PLACEMENT_3D ( 'NONE', #25026, #18832, #15822 ) ;
#4644=ORIENTED_EDGE ( 'NONE', *, *, #31404, .T. ) ;
#4645=CARTESIAN_POINT ( 'NONE',  ( 21.99999662536862033, -69.28203230275519786, -5.000000000000000000 ) ) ;
#4646=CARTESIAN_POINT ( 'NONE',  ( 72.28378166042060116, 61.53067111003190348, -4.999999999999997335 ) ) ;
#4647=DIRECTION ( 'NONE',  ( 1.000000000000000000, 0.000000000000000000, 0.000000000000000000 ) ) ;
#4652=EDGE_CURVE ( 'NONE', #12600, #15693, #19484, .T. ) ;
#4653=VERTEX_POINT ( 'NONE', #28881 ) ;
#4654=CARTESIAN_POINT ( 'NONE',  ( -75.00000337463097821, 43.30127018922197379, -9.999999999999998224 ) ) ;
#4656=CIRCLE ( 'NONE', #35197, 2.000000000000001776 ) ;
#4658=ORIENTED_EDGE ( 'NONE', *, *, #55, .T. ) ;
#4661=VERTEX_POINT ( 'NONE', #3204 ) ;
#4663=CIRCLE ( 'NONE', #33997, 2.000000000000001776 ) ;
#4664=CARTESIAN_POINT ( 'NONE',  ( -47.00000337463111322, -77.94228634059960825, -9.999999999999998224 ) ) ;
#4665=CIRCLE ( 'NONE', #12420, 27.00000000000001066 ) ;
#4667=DIRECTION ( 'NONE',  ( 0.000000000000000000, 0.000000000000000000, 1.000000000000000000 ) ) ;
#4668=ORIENTED_EDGE ( 'NONE', *, *, #17737, .F. ) ;
#4669=CARTESIAN_POINT ( 'NONE',  ( 54.99999662536844625, -60.62177826491080168, -9.999999999999998224 ) ) ;
#4670=ORIENTED_EDGE ( 'NONE', *, *, #18379, .T. ) ;
#4672=CIRCLE ( 'NONE', #10631, 2.000000000000001776 ) ;
#4674=CIRCLE ( 'NONE', #32790, 2.000000000000001776 ) ;
#4675=CARTESIAN_POINT ( 'NONE',  ( 84.99999662536832545, 25.98076211353319565, -9.999999999999998224 ) ) ;
#4676=DIRECTION ( 'NONE',  ( 0.000000000000000000, 0.000000000000000000, 1.000000000000000000 ) ) ;
#4677=EDGE_LOOP ( 'NONE', ( #13548, #3195 ) ) ;
#4678=CYLINDRICAL_SURFACE ( 'NONE', #16080, 2.000000000000001776 ) ;
#4679=CARTESIAN_POINT ( 'NONE',  ( -52.39915983220772233, -35.19434990244957362, 12.49999999999999822 ) ) ;
#4680=AXIS2_PLACEMENT_3D ( 'NONE', #6820, #30245, #10213 ) ;
#4685=EDGE_LOOP ( 'NONE', ( #12320, #20407, #6996, #21912, #1930 ) ) ;
#4688=CIRCLE ( 'NONE', #25617, 2.000000000000001776 ) ;
#4689=AXIS2_PLACEMENT_3D ( 'NONE', #7170, #35857, #35658 ) ;
#4691=CARTESIAN_POINT ( 'NONE',  ( 84.99999662536832545, 8.660254037844394404, -9.999999999999998224 ) ) ;
#4692=CIRCLE ( 'NONE', #8271, 2.000000000000001776 ) ;
#4693=DIRECTION ( 'NONE',  ( 0.000000000000000000, -0.000000000000000000, -1.000000000000000000 ) ) ;
#4694=CIRCLE ( 'NONE', #28627, 2.000000000000001776 ) ;
#4695=CARTESIAN_POINT ( 'NONE',  ( -23.00000337463121980, -77.94228634059963667, 17.49999999999999645 ) ) ;
#4696=LINE ( 'NONE', #24377, #14292 ) ;
#4698=DIRECTION ( 'NONE',  ( 0.000000000000000000, 0.000000000000000000, 1.000000000000000000 ) ) ;
#4699=ORIENTED_EDGE ( 'NONE', *, *, #16412, .T. ) ;
#4700=VERTEX_POINT ( 'NONE', #19905 ) ;
#4701=VECTOR ( 'NONE', #5047, 1000.000000000000000 ) ;
#4702=DIRECTION ( 'NONE',  ( -1.000000000000000000, 0.000000000000000000, 0.000000000000000000 ) ) ;
#4703=DIRECTION ( 'NONE',  ( 1.000000000000000000, 0.000000000000000000, 0.000000000000000000 ) ) ;
#4704=EDGE_CURVE ( 'NONE', #22301, #6746, #10512, .T. ) ;
#4705=DIRECTION ( 'NONE',  ( 1.000000000000000000, 0.000000000000000000, 0.000000000000000000 ) ) ;
#4706=DIRECTION ( 'NONE',  ( 1.000000000000000000, 0.000000000000000000, 0.000000000000000000 ) ) ;
#4707=ORIENTED_EDGE ( 'NONE', *, *, #17502, .T. ) ;
#4709=CIRCLE ( 'NONE', #9493, 33.00000000000001421 ) ;
#4710=CARTESIAN_POINT ( 'NONE',  ( -68.00000000000000000, 0.000000000000000000, -49.86348611802629449 ) ) ;
#4711=DIRECTION ( 'NONE',  ( 0.000000000000000000, 0.000000000000000000, -1.000000000000000000 ) ) ;
#4713=AXIS2_PLACEMENT_3D ( 'NONE', #12136, #28844, #32011 ) ;
#4714=EDGE_LOOP ( 'NONE', ( #23125, #19838, #13363, #8521 ) ) ;
#4715=VECTOR ( 'NONE', #26429, 1000.000000000000000 ) ;
#4716=CARTESIAN_POINT ( 'NONE',  ( -55.00000337463107059, 60.62177826491078747, -9.999999999999998224 ) ) ;
#4718=CIRCLE ( 'NONE', #29233, 2.000000000000001776 ) ;
#4719=CARTESIAN_POINT ( 'NONE',  ( -55.00000337463109901, -60.62177826491083010, 12.50000000000000000 ) ) ;
#4720=LINE ( 'NONE', #16331, #36784 ) ;
#4721=CIRCLE ( 'NONE', #22088, 2.000000000000001776 ) ;
#4722=CARTESIAN_POINT ( 'NONE',  ( -87.00000337463093558, 8.660254037844389075, 12.50000000000000000 ) ) ;
#4723=EDGE_LOOP ( 'NONE', ( #4368, #32539 ) ) ;
#4724=VERTEX_POINT ( 'NONE', #8838 ) ;
#4726=ADVANCED_FACE ( 'NONE', ( #20825 ), #32443, .F. ) ;
#4727=FACE_OUTER_BOUND ( 'NONE', #11369, .T. ) ;
#4728=ORIENTED_EDGE ( 'NONE', *, *, #12498, .T. ) ;
#4729=DIRECTION ( 'NONE',  ( -0.5000000000000098810, -0.8660254037844328234, 0.000000000000000000 ) ) ;
#4730=DIRECTION ( 'NONE',  ( 0.000000000000000000, 0.000000000000000000, 1.000000000000000000 ) ) ;
#4731=PLANE ( 'NONE',  #5856 ) ;
#4732=CARTESIAN_POINT ( 'NONE',  ( -58.00000337463104216, 34.64101615137757051, -9.999999999999998224 ) ) ;
#4733=LINE ( 'NONE', #21964, #32719 ) ;
#4735=CARTESIAN_POINT ( 'NONE',  ( -70.00000337463099243, -2.428612866367529932E-14, 17.49999999999999645 ) ) ;
#4739=AXIS2_PLACEMENT_3D ( 'NONE', #9550, #23991, #30148 ) ;
#4741=EDGE_LOOP ( 'NONE', ( #2665, #32761, #3413, #33240 ) ) ;
#4742=DIRECTION ( 'NONE',  ( 0.000000000000000000, 0.000000000000000000, 1.000000000000000000 ) ) ;
#4743=FACE_OUTER_BOUND ( 'NONE', #12767, .T. ) ;
#4745=EDGE_LOOP ( 'NONE', ( #29743, #33940, #13619, #32481, #7404 ) ) ;
#4746=CIRCLE ( 'NONE', #29266, 33.00000000000001421 ) ;
#4748=EDGE_CURVE ( 'NONE', #14472, #33302, #19543, .T. ) ;
#4751=ORIENTED_EDGE ( 'NONE', *, *, #29260, .T. ) ;
#4753=VERTEX_POINT ( 'NONE', #9587 ) ;
#4754=CIRCLE ( 'NONE', #28686, 2.000000000000001776 ) ;
#4755=FACE_OUTER_BOUND ( 'NONE', #26288, .T. ) ;
#4756=AXIS2_PLACEMENT_3D ( 'NONE', #11001, #31078, #22441 ) ;
#4758=AXIS2_PLACEMENT_3D ( 'NONE', #7222, #4227, #35533 ) ;
#4759=CARTESIAN_POINT ( 'NONE',  ( 4.279621169095998212, -62.97617850287780072, -4.999999999999997335 ) ) ;
#4761=ORIENTED_EDGE ( 'NONE', *, *, #25041, .T. ) ;
#4762=DIRECTION ( 'NONE',  ( -1.000000000000000000, 0.000000000000000000, 0.000000000000000000 ) ) ;
#4763=AXIS2_PLACEMENT_3D ( 'NONE', #24125, #18689, #7068 ) ;
#4766=ORIENTED_EDGE ( 'NONE', *, *, #10549, .T. ) ;
#4768=CARTESIAN_POINT ( 'NONE',  ( 54.99999662536846046, -43.30127018922200222, -9.999999999999998224 ) ) ;
#4770=CYLINDRICAL_SURFACE ( 'NONE', #6980, 1.999999999999998224 ) ;
#4771=CARTESIAN_POINT ( 'NONE',  ( -88.00000337463090716, -1.040834085586084257E-14, -5.000000000000000000 ) ) ;
#4772=DIRECTION ( 'NONE',  ( -0.000000000000000000, 0.000000000000000000, -1.000000000000000000 ) ) ;
#4774=CARTESIAN_POINT ( 'NONE',  ( -72.00000337463100664, 34.64101615137758472, 12.50000000000000000 ) ) ;
#4775=FACE_BOUND ( 'NONE', #31293, .T. ) ;
#4776=EDGE_CURVE ( 'NONE', #24912, #12365, #32056, .T. ) ;
#4778=DIRECTION ( 'NONE',  ( 0.5000000000000039968, 0.8660254037844363761, 0.000000000000000000 ) ) ;
#4779=CARTESIAN_POINT ( 'NONE',  ( 66.99999662536839651, -60.62177826491080168, -5.000000000000000000 ) ) ;
#4780=AXIS2_PLACEMENT_3D ( 'NONE', #8394, #31426, #5565 ) ;
#4781=DIRECTION ( 'NONE',  ( 0.000000000000000000, 0.000000000000000000, 1.000000000000000000 ) ) ;
#4782=CYLINDRICAL_SURFACE ( 'NONE', #9536, 2.000000000000001776 ) ;
#4784=LINE ( 'NONE', #27810, #8597 ) ;
#4785=ORIENTED_EDGE ( 'NONE', *, *, #6664, .T. ) ;
#4786=DIRECTION ( 'NONE',  ( 1.000000000000000000, 0.000000000000000000, 0.000000000000000000 ) ) ;
#4787=DIRECTION ( 'NONE',  ( 0.000000000000000000, 0.000000000000000000, 1.000000000000000000 ) ) ;
#4788=AXIS2_PLACEMENT_3D ( 'NONE', #9652, #29688, #35707 ) ;
#4790=ORIENTED_EDGE ( 'NONE', *, *, #17334, .F. ) ;
#4791=EDGE_LOOP ( 'NONE', ( #28617, #35683, #34393, #624 ) ) ;
#4793=AXIS2_PLACEMENT_3D ( 'NONE', #4820, #13609, #33108 ) ;
#4794=CYLINDRICAL_SURFACE ( 'NONE', #26734, 2.000000000000000000 ) ;
#4796=AXIS2_PLACEMENT_3D ( 'NONE', #34273, #28635, #34100 ) ;
#4797=VERTEX_POINT ( 'NONE', #3591 ) ;
#4798=DIRECTION ( 'NONE',  ( 0.000000000000000000, 0.000000000000000000, -1.000000000000000000 ) ) ;
#4799=EDGE_CURVE ( 'NONE', #7714, #25889, #21319, .T. ) ;
#4800=FACE_OUTER_BOUND ( 'NONE', #19182, .T. ) ;
#4801=ORIENTED_EDGE ( 'NONE', *, *, #6912, .F. ) ;
#4802=DIRECTION ( 'NONE',  ( 0.000000000000000000, 0.000000000000000000, 1.000000000000000000 ) ) ;
#4803=EDGE_LOOP ( 'NONE', ( #24203, #34220, #35381, #10075 ) ) ;
#4804=PLANE ( 'NONE',  #336 ) ;
#4805=AXIS2_PLACEMENT_3D ( 'NONE', #22223, #33662, #13788 ) ;
#4806=EDGE_CURVE ( 'NONE', #20017, #2812, #30292, .T. ) ;
#4807=CARTESIAN_POINT ( 'NONE',  ( 19.99999662536857770, 86.60254037844397601, -9.999999999999998224 ) ) ;
#4808=FACE_OUTER_BOUND ( 'NONE', #24142, .T. ) ;
#4809=EDGE_CURVE ( 'NONE', #23895, #34851, #21919, .T. ) ;
#4810=DIRECTION ( 'NONE',  ( 1.000000000000000000, 0.000000000000000000, 0.000000000000000000 ) ) ;
#4811=CIRCLE ( 'NONE', #21554, 2.000000000000001776 ) ;
#4813=CARTESIAN_POINT ( 'NONE',  ( -15.00000337463126066, 77.94228634059957983, 17.49999999999999645 ) ) ;
#4814=AXIS2_PLACEMENT_3D ( 'NONE', #35445, #9362, #9731 ) ;
#4816=CYLINDRICAL_SURFACE ( 'NONE', #6906, 1.999999999999998224 ) ;
#4817=DIRECTION ( 'NONE',  ( 1.000000000000000000, 0.000000000000000000, 0.000000000000000000 ) ) ;
#4818=EDGE_LOOP ( 'NONE', ( #7556, #26983, #27021, #34137 ) ) ;
#4819=LINE ( 'NONE', #21500, #28144 ) ;
#4820=CARTESIAN_POINT ( 'NONE',  ( -65.00000337463104927, -25.98076211353322051, 12.50000000000000000 ) ) ;
#4821=EDGE_LOOP ( 'NONE', ( #21628, #3865, #32039, #35325 ) ) ;
#4822=CARTESIAN_POINT ( 'NONE',  ( -37.00000337463116296, 77.94228634059957983, -9.999999999999998224 ) ) ;
#4823=VECTOR ( 'NONE', #33504, 1000.000000000000000 ) ;
#4824=DIRECTION ( 'NONE',  ( -0.000000000000000000, -0.000000000000000000, 1.000000000000000000 ) ) ;
#4825=CARTESIAN_POINT ( 'NONE',  ( -47.04203867989546950, 43.19957991610416315, 12.49999999999999822 ) ) ;
#4826=ORIENTED_EDGE ( 'NONE', *, *, #31749, .T. ) ;
#4829=VECTOR ( 'NONE', #16479, 1000.000000000000000 ) ;
#4830=FACE_OUTER_BOUND ( 'NONE', #339, .T. ) ;
#4831=DIRECTION ( 'NONE',  ( 1.000000000000000000, 0.000000000000000000, 0.000000000000000000 ) ) ;
#4832=DIRECTION ( 'NONE',  ( 0.000000000000000000, 0.000000000000000000, 1.000000000000000000 ) ) ;
#4833=ORIENTED_EDGE ( 'NONE', *, *, #36204, .F. ) ;
#4834=ORIENTED_EDGE ( 'NONE', *, *, #26069, .T. ) ;
#4835=CIRCLE ( 'NONE', #17987, 2.000000000000000000 ) ;
#4836=DIRECTION ( 'NONE',  ( 0.000000000000000000, 0.000000000000000000, -1.000000000000000000 ) ) ;
#4837=CARTESIAN_POINT ( 'NONE',  ( 0.000000000000000000, 0.000000000000000000, 17.49999999999999645 ) ) ;
#4839=AXIS2_PLACEMENT_3D ( 'NONE', #1220, #12639, #35912 ) ;
#4841=VERTEX_POINT ( 'NONE', #4328 ) ;
#4842=ORIENTED_EDGE ( 'NONE', *, *, #33937, .T. ) ;
#4843=DIRECTION ( 'NONE',  ( 0.000000000000000000, 0.000000000000000000, -1.000000000000000000 ) ) ;
#4844=EDGE_CURVE ( 'NONE', #25741, #19087, #35088, .T. ) ;
#4845=CARTESIAN_POINT ( 'NONE',  ( -75.00000337463097821, 25.98076211353318854, 17.49999999999999645 ) ) ;
#4846=EDGE_LOOP ( 'NONE', ( #3809, #15910, #17879, #17988 ) ) ;
#4847=ADVANCED_FACE ( 'NONE', ( #18592 ), #21191, .T. ) ;
#4849=ORIENTED_EDGE ( 'NONE', *, *, #9612, .F. ) ;
#4850=DIRECTION ( 'NONE',  ( 0.000000000000000000, 0.000000000000000000, 1.000000000000000000 ) ) ;
#4852=CARTESIAN_POINT ( 'NONE',  ( 59.99999662536842493, -51.96152422706639840, 17.49999999999999645 ) ) ;
#4853=ADVANCED_FACE ( 'NONE', ( #1499 ), #6756, .F. ) ;
#4854=FACE_OUTER_BOUND ( 'NONE', #17749, .T. ) ;
#4857=DIRECTION ( 'NONE',  ( 0.000000000000000000, 0.000000000000000000, 1.000000000000000000 ) ) ;
#4858=DIRECTION ( 'NONE',  ( 0.000000000000000000, 0.000000000000000000, -1.000000000000000000 ) ) ;
#4859=CARTESIAN_POINT ( 'NONE',  ( 29.99999662536857770, -69.28203230275519786, 17.49999999999999645 ) ) ;
#4861=ORIENTED_EDGE ( 'NONE', *, *, #31721, .F. ) ;
#4862=CARTESIAN_POINT ( 'NONE',  ( -80.00000337463094979, -17.32050807568882078, 12.50000000000000000 ) ) ;
#4863=DIRECTION ( 'NONE',  ( 0.000000000000000000, 0.000000000000000000, 1.000000000000000000 ) ) ;
#4864=DIRECTION ( 'NONE',  ( 0.000000000000000000, 0.000000000000000000, 1.000000000000000000 ) ) ;
#4865=ADVANCED_FACE ( 'NONE', ( #23461 ), #36191, .F. ) ;
#4866=ORIENTED_EDGE ( 'NONE', *, *, #17737, .T. ) ;
#4867=EDGE_CURVE ( 'NONE', #21984, #22983, #20122, .T. ) ;
#4868=ORIENTED_EDGE ( 'NONE', *, *, #4341, .F. ) ;
#4869=VERTEX_POINT ( 'NONE', #35840 ) ;
#4870=EDGE_CURVE ( 'NONE', #29683, #21341, #8163, .T. ) ;
#4871=EDGE_CURVE ( 'NONE', #36051, #17344, #351, .T. ) ;
#4872=CARTESIAN_POINT ( 'NONE',  ( -50.00000337463110611, -69.28203230275519786, -9.999999999999998224 ) ) ;
#4873=ORIENTED_EDGE ( 'NONE', *, *, #22376, .T. ) ;
#4874=EDGE_CURVE ( 'NONE', #26842, #35523, #9323, .T. ) ;
#4875=CARTESIAN_POINT ( 'NONE',  ( 64.99999662536839651, -43.30127018922199511, -5.000000000000000000 ) ) ;
#4876=DIRECTION ( 'NONE',  ( 1.000000000000000000, 0.000000000000000000, 0.000000000000000000 ) ) ;
#4877=CARTESIAN_POINT ( 'NONE',  ( -20.00000337463124112, 69.28203230275516944, -9.999999999999998224 ) ) ;
#4878=CYLINDRICAL_SURFACE ( 'NONE', #28974, 33.00000000000001421 ) ;
#4879=DIRECTION ( 'NONE',  ( -0.000000000000000000, -0.000000000000000000, 1.000000000000000000 ) ) ;
#4880=DIRECTION ( 'NONE',  ( 0.000000000000000000, 0.000000000000000000, 1.000000000000000000 ) ) ;
#4881=CIRCLE ( 'NONE', #1275, 95.00000000000000000 ) ;
#4882=DIRECTION ( 'NONE',  ( 1.000000000000000000, 0.000000000000000000, 0.000000000000000000 ) ) ;
#4883=DIRECTION ( 'NONE',  ( 0.000000000000000000, 0.000000000000000000, 1.000000000000000000 ) ) ;
#4885=ORIENTED_EDGE ( 'NONE', *, *, #27225, .T. ) ;
#4886=DIRECTION ( 'NONE',  ( 0.000000000000000000, 0.000000000000000000, 1.000000000000000000 ) ) ;
#4887=DIRECTION ( 'NONE',  ( 1.000000000000000000, 0.000000000000000000, 0.000000000000000000 ) ) ;
#4888=DIRECTION ( 'NONE',  ( 0.000000000000000000, 0.000000000000000000, 1.000000000000000000 ) ) ;
#4890=CARTESIAN_POINT ( 'NONE',  ( 69.99999662536839651, 17.32050807568879236, -9.999999999999998224 ) ) ;
#4891=FACE_OUTER_BOUND ( 'NONE', #17722, .T. ) ;
#4892=VERTEX_POINT ( 'NONE', #24950 ) ;
#4894=CARTESIAN_POINT ( 'NONE',  ( -80.00000337463096400, -34.64101615137762025, -9.999999999999998224 ) ) ;
#4895=ORIENTED_EDGE ( 'NONE', *, *, #20162, .T. ) ;
#4897=DIRECTION ( 'NONE',  ( -1.000000000000000000, 0.000000000000000000, 0.000000000000000000 ) ) ;
#4898=DIRECTION ( 'NONE',  ( 0.000000000000000000, 0.000000000000000000, 1.000000000000000000 ) ) ;
#4899=AXIS2_PLACEMENT_3D ( 'NONE', #32498, #12795, #10208 ) ;
#4900=VERTEX_POINT ( 'NONE', #13486 ) ;
#4901=VERTEX_POINT ( 'NONE', #24592 ) ;
#4902=CIRCLE ( 'NONE', #9085, 1.999999999999998224 ) ;
#4903=ORIENTED_EDGE ( 'NONE', *, *, #1074, .T. ) ;
#4904=CARTESIAN_POINT ( 'NONE',  ( 0.000000000000000000, 0.000000000000000000, 12.49999999999999822 ) ) ;
#4905=EDGE_CURVE ( 'NONE', #8144, #31157, #7548, .T. ) ;
#4906=CARTESIAN_POINT ( 'NONE',  ( 45.00000000000000711, 0.000000000000000000, -10.00000000000000000 ) ) ;
#4907=DIRECTION ( 'NONE',  ( 1.000000000000000000, 0.000000000000000000, 0.000000000000000000 ) ) ;
#4908=DIRECTION ( 'NONE',  ( 1.000000000000000000, 0.000000000000000000, 0.000000000000000000 ) ) ;
#4910=VERTEX_POINT ( 'NONE', #27576 ) ;
#4911=CYLINDRICAL_SURFACE ( 'NONE', #23117, 2.000000000000001776 ) ;
#4913=FILL_AREA_STYLE ('',( #4541 ) ) ;
#4914=ORIENTED_EDGE ( 'NONE', *, *, #31721, .T. ) ;
#4917=EDGE_LOOP ( 'NONE', ( #28268, #7454, #871, #1290, #348, #6131 ) ) ;
#4918=ORIENTED_EDGE ( 'NONE', *, *, #27403, .F. ) ;
#4919=DIRECTION ( 'NONE',  ( 0.000000000000000000, 0.000000000000000000, 1.000000000000000000 ) ) ;
#4923=EDGE_LOOP ( 'NONE', ( #26480, #25783 ) ) ;
#4925=CARTESIAN_POINT ( 'NONE',  ( -33.99999999999945288, 58.88972745734214698, -4.999999999999997335 ) ) ;
#4926=ORIENTED_EDGE ( 'NONE', *, *, #26252, .T. ) ;
#4927=FACE_OUTER_BOUND ( 'NONE', #30989, .T. ) ;
#4928=ORIENTED_EDGE ( 'NONE', *, *, #6135, .F. ) ;
#4929=EDGE_LOOP ( 'NONE', ( #15844, #32999 ) ) ;
#4930=DIRECTION ( 'NONE',  ( 0.000000000000000000, 0.000000000000000000, 1.000000000000000000 ) ) ;
#4931=FACE_BOUND ( 'NONE', #5382, .T. ) ;
#4932=ORIENTED_EDGE ( 'NONE', *, *, #34337, .T. ) ;
#4933=ORIENTED_EDGE ( 'NONE', *, *, #18131, .F. ) ;
#4936=CARTESIAN_POINT ( 'NONE',  ( -68.00000337463099243, 17.32050807568877460, -9.999999999999998224 ) ) ;
#4937=DIRECTION ( 'NONE',  ( 0.000000000000000000, 0.000000000000000000, 1.000000000000000000 ) ) ;
#4938=ORIENTED_EDGE ( 'NONE', *, *, #8184, .F. ) ;
#4939=DIRECTION ( 'NONE',  ( 0.000000000000000000, 0.000000000000000000, 1.000000000000000000 ) ) ;
#4940=VECTOR ( 'NONE', #26607, 1000.000000000000000 ) ;
#4941=EDGE_CURVE ( 'NONE', #23803, #22301, #21747, .T. ) ;
#4942=FACE_BOUND ( 'NONE', #7434, .T. ) ;
#4943=CARTESIAN_POINT ( 'NONE',  ( -47.63139720814380951, 27.50000000000055422, -10.00000000000000178 ) ) ;
#4944=DIRECTION ( 'NONE',  ( 0.000000000000000000, 0.000000000000000000, 1.000000000000000000 ) ) ;
#4945=CYLINDRICAL_SURFACE ( 'NONE', #7538, 2.000000000000001776 ) ;
#4947=DIRECTION ( 'NONE',  ( 0.000000000000000000, 0.000000000000000000, 1.000000000000000000 ) ) ;
#4949=ORIENTED_EDGE ( 'NONE', *, *, #9627, .T. ) ;
#4950=DIRECTION ( 'NONE',  ( 0.000000000000000000, 0.000000000000000000, -1.000000000000000000 ) ) ;
#4951=LINE ( 'NONE', #10776, #27909 ) ;
#4952=FACE_OUTER_BOUND ( 'NONE', #15032, .T. ) ;
#4953=VERTEX_POINT ( 'NONE', #10697 ) ;
#4954=VECTOR ( 'NONE', #29654, 1000.000000000000000 ) ;
#4955=ORIENTED_EDGE ( 'NONE', *, *, #27259, .T. ) ;
#4956=ORIENTED_EDGE ( 'NONE', *, *, #10827, .F. ) ;
#4959=FACE_OUTER_BOUND ( 'NONE', #23586, .T. ) ;
#4960=ORIENTED_EDGE ( 'NONE', *, *, #33626, .T. ) ;
#4961=EDGE_CURVE ( 'NONE', #15953, #16595, #4557, .T. ) ;
#4965=ORIENTED_EDGE ( 'NONE', *, *, #28529, .F. ) ;
#4966=AXIS2_PLACEMENT_3D ( 'NONE', #22381, #7401, #10778 ) ;
#4967=CARTESIAN_POINT ( 'NONE',  ( 1.999996625368665182, 69.28203230275516944, -9.999999999999998224 ) ) ;
#4969=EDGE_CURVE ( 'NONE', #15313, #15633, #30180, .T. ) ;
#4970=ORIENTED_EDGE ( 'NONE', *, *, #4905, .F. ) ;
#4971=DIRECTION ( 'NONE',  ( 1.000000000000000000, 0.000000000000000000, 0.000000000000000000 ) ) ;
#4972=EDGE_CURVE ( 'NONE', #4038, #32213, #33891, .T. ) ;
#4973=CARTESIAN_POINT ( 'NONE',  ( -45.00000337463112743, -60.62177826491080168, -9.999999999999998224 ) ) ;
#4975=ORIENTED_EDGE ( 'NONE', *, *, #12138, .T. ) ;
#4976=LINE ( 'NONE', #37044, #34468 ) ;
#4977=CIRCLE ( 'NONE', #27125, 2.000000000000000000 ) ;
#4979=FACE_OUTER_BOUND ( 'NONE', #11173, .T. ) ;
#4980=DIRECTION ( 'NONE',  ( 0.000000000000000000, 0.000000000000000000, -1.000000000000000000 ) ) ;
#4981=CIRCLE ( 'NONE', #6149, 2.000000000000001776 ) ;
#4983=LINE ( 'NONE', #35571, #25167 ) ;
#4984=DIRECTION ( 'NONE',  ( 0.000000000000000000, 0.000000000000000000, 1.000000000000000000 ) ) ;
#4985=ORIENTED_EDGE ( 'NONE', *, *, #5511, .T. ) ;
#4986=LINE ( 'NONE', #2723, #15454 ) ;
#4987=CARTESIAN_POINT ( 'NONE',  ( -93.36492675454779544, -17.14523346298311779, -4.999999999999997335 ) ) ;
#4988=CARTESIAN_POINT ( 'NONE',  ( 0.000000000000000000, 0.000000000000000000, -5.000000000000000000 ) ) ;
#4989=EDGE_CURVE ( 'NONE', #13923, #24391, #22503, .T. ) ;
#4990=ORIENTED_EDGE ( 'NONE', *, *, #16986, .F. ) ;
#4991=AXIS2_PLACEMENT_3D ( 'NONE', #20472, #28555, #8677 ) ;
#4992=ORIENTED_EDGE ( 'NONE', *, *, #4799, .F. ) ;
#4993=CARTESIAN_POINT ( 'NONE',  ( -73.00000337463097821, 25.98076211353318854, -9.999999999999998224 ) ) ;
#4994=DIRECTION ( 'NONE',  ( 1.000000000000000000, 0.000000000000000000, 0.000000000000000000 ) ) ;
#4995=EDGE_CURVE ( 'NONE', #36127, #792, #26704, .T. ) ;
#4996=DIRECTION ( 'NONE',  ( -0.000000000000000000, -0.000000000000000000, -1.000000000000000000 ) ) ;
#4999=EDGE_CURVE ( 'NONE', #18775, #4152, #32754, .T. ) ;
#5003=CIRCLE ( 'NONE', #3201, 27.00000000000001066 ) ;
#5004=CARTESIAN_POINT ( 'NONE',  ( 81.99999662536832545, -34.64101615137759183, 17.49999999999999645 ) ) ;
#5005=EDGE_LOOP ( 'NONE', ( #11292, #20253 ) ) ;
#5006=ORIENTED_EDGE ( 'NONE', *, *, #16403, .T. ) ;
#5007=CIRCLE ( 'NONE', #3790, 2.000000000000001776 ) ;
#5008=DIRECTION ( 'NONE',  ( 3.491481338843135327E-15, 1.000000000000000000, 0.000000000000000000 ) ) ;
#5009=DIRECTION ( 'NONE',  ( 1.000000000000000000, 0.000000000000000000, 0.000000000000000000 ) ) ;
#5010=ORIENTED_EDGE ( 'NONE', *, *, #241, .T. ) ;
#5011=DIRECTION ( 'NONE',  ( 0.000000000000000000, -0.000000000000000000, -1.000000000000000000 ) ) ;
#5012=EDGE_LOOP ( 'NONE', ( #14358, #15048, #21632, #33214 ) ) ;
#5013=CARTESIAN_POINT ( 'NONE',  ( -28.00000337463118427, 69.28203230275516944, 12.50000000000000000 ) ) ;
#5014=CIRCLE ( 'NONE', #22382, 3.499999999999989342 ) ;
#5015=EDGE_CURVE ( 'NONE', #4869, #17775, #27119, .T. ) ;
#5016=DIRECTION ( 'NONE',  ( 0.000000000000000000, 0.000000000000000000, 1.000000000000000000 ) ) ;
#5017=CIRCLE ( 'NONE', #25975, 3.000000000000002665 ) ;
#5018=VERTEX_POINT ( 'NONE', #1434 ) ;
#5019=AXIS2_PLACEMENT_3D ( 'NONE', #11531, #22985, #22815 ) ;
#5021=CARTESIAN_POINT ( 'NONE',  ( 77.99999662536832545, -34.64101615137759183, -9.999999999999998224 ) ) ;
#5023=VERTEX_POINT ( 'NONE', #27306 ) ;
#5024=CARTESIAN_POINT ( 'NONE',  ( 57.99999662536844625, 34.64101615137759893, -9.999999999999998224 ) ) ;
#5025=CARTESIAN_POINT ( 'NONE',  ( -70.00000337463102085, -34.64101615137762025, -9.999999999999998224 ) ) ;
#5027=ORIENTED_EDGE ( 'NONE', *, *, #21083, .T. ) ;
#5028=CIRCLE ( 'NONE', #28360, 2.000000000000001776 ) ;
#5030=ORIENTED_EDGE ( 'NONE', *, *, #28678, .F. ) ;
#5031=FACE_OUTER_BOUND ( 'NONE', #9432, .T. ) ;
#5032=EDGE_CURVE ( 'NONE', #17931, #32624, #1628, .T. ) ;
#5033=ORIENTED_EDGE ( 'NONE', *, *, #12828, .T. ) ;
#5034=DIRECTION ( 'NONE',  ( -0.8660254037844379305, 0.5000000000000012212, 0.000000000000000000 ) ) ;
#5035=CARTESIAN_POINT ( 'NONE',  ( 36.99999662536853862, 77.94228634059959404, -9.999999999999998224 ) ) ;
#5036=CIRCLE ( 'NONE', #8617, 2.000000000000001776 ) ;
#5037=ADVANCED_FACE ( 'NONE', ( #23771 ), #6523, .F. ) ;
#5038=DIRECTION ( 'NONE',  ( 0.5000000000000038858, 0.8660254037844362651, 0.000000000000000000 ) ) ;
#5039=AXIS2_PLACEMENT_3D ( 'NONE', #23447, #1130, #3577 ) ;
#5040=CARTESIAN_POINT ( 'NONE',  ( 7.999996625368656744, -69.28203230275519786, -9.999999999999998224 ) ) ;
#5044=EDGE_CURVE ( 'NONE', #26423, #13225, #29071, .T. ) ;
#5046=EDGE_CURVE ( 'NONE', #13221, #11018, #18325, .T. ) ;
#5047=DIRECTION ( 'NONE',  ( 0.000000000000000000, 0.000000000000000000, 1.000000000000000000 ) ) ;
#5048=ORIENTED_EDGE ( 'NONE', *, *, #31424, .T. ) ;
#5050=CARTESIAN_POINT ( 'NONE',  ( -65.00000337463102085, 43.30127018922198801, -5.000000000000000000 ) ) ;
#5051=CARTESIAN_POINT ( 'NONE',  ( -92.00000337463090716, -1.016341149603137227E-14, -9.999999999999998224 ) ) ;
#5052=CARTESIAN_POINT ( 'NONE',  ( -31.02796211690907668, 59.29837256189569672, -4.999999999999997335 ) ) ;
#5053=FACE_OUTER_BOUND ( 'NONE', #15014, .T. ) ;
#5054=ORIENTED_EDGE ( 'NONE', *, *, #36343, .F. ) ;
#5056=EDGE_CURVE ( 'NONE', #36279, #12950, #6952, .T. ) ;
#5057=EDGE_CURVE ( 'NONE', #29611, #716, #26145, .T. ) ;
#5058=CIRCLE ( 'NONE', #21807, 2.000000000000001776 ) ;
#5060=DIRECTION ( 'NONE',  ( -0.000000000000000000, -0.000000000000000000, 1.000000000000000000 ) ) ;
#5061=ORIENTED_EDGE ( 'NONE', *, *, #9337, .T. ) ;
#5062=ORIENTED_EDGE ( 'NONE', *, *, #11553, .F. ) ;
#5063=CARTESIAN_POINT ( 'NONE',  ( -56.67878100130369035, 27.78182860042797131, -4.999999999999997335 ) ) ;
#5064=ORIENTED_EDGE ( 'NONE', *, *, #12536, .T. ) ;
#5067=AXIS2_PLACEMENT_3D ( 'NONE', #14599, #20417, #344 ) ;
#5068=PLANE ( 'NONE',  #12202 ) ;
#5069=CIRCLE ( 'NONE', #30214, 33.00000000000001421 ) ;
#5072=VERTEX_POINT ( 'NONE', #18524 ) ;
#5073=ADVANCED_FACE ( 'NONE', ( #26564 ), #4444, .F. ) ;
#5074=ORIENTED_EDGE ( 'NONE', *, *, #29724, .F. ) ;
#5075=CIRCLE ( 'NONE', #25446, 2.000000000000001776 ) ;
#5077=DIRECTION ( 'NONE',  ( -1.000000000000000000, 0.000000000000000000, 0.000000000000000000 ) ) ;
#5078=EDGE_CURVE ( 'NONE', #15625, #19893, #26735, .T. ) ;
#5079=AXIS2_PLACEMENT_3D ( 'NONE', #358, #17266, #17434 ) ;
#5080=CARTESIAN_POINT ( 'NONE',  ( -47.63139720814380951, 27.50000000000055422, -5.000000000000000000 ) ) ;
#5081=CARTESIAN_POINT ( 'NONE',  ( 56.99999662536846046, -43.30127018922200222, 12.50000000000000000 ) ) ;
#5082=DIRECTION ( 'NONE',  ( -1.000000000000000000, 0.000000000000000000, 0.000000000000000000 ) ) ;
#5083=ORIENTED_EDGE ( 'NONE', *, *, #29965, .T. ) ;
#5084=CARTESIAN_POINT ( 'NONE',  ( -70.00000337463099243, 34.64101615137758472, -5.000000000000000000 ) ) ;
#5085=VECTOR ( 'NONE', #17620, 1000.000000000000000 ) ;
#5087=CYLINDRICAL_SURFACE ( 'NONE', #3215, 2.000000000000000000 ) ;
#5088=ORIENTED_EDGE ( 'NONE', *, *, #18488, .T. ) ;
#5089=CYLINDRICAL_SURFACE ( 'NONE', #25068, 95.00000000000000000 ) ;
#5090=ADVANCED_FACE ( 'NONE', ( #32190 ), #3875, .F. ) ;
#5092=AXIS2_PLACEMENT_3D ( 'NONE', #688, #12095, #17554 ) ;
#5093=VERTEX_POINT ( 'NONE', #23964 ) ;
#5094=AXIS2_PLACEMENT_3D ( 'NONE', #13648, #7658, #33141 ) ;
#5095=VERTEX_POINT ( 'NONE', #35414 ) ;
#5096=DIRECTION ( 'NONE',  ( -1.000000000000000000, 0.000000000000000000, 0.000000000000000000 ) ) ;
#5097=CARTESIAN_POINT ( 'NONE',  ( 81.99999662536832545, -34.64101615137759183, 12.50000000000000000 ) ) ;
#5101=VERTEX_POINT ( 'NONE', #18316 ) ;
#5102=ORIENTED_EDGE ( 'NONE', *, *, #2186, .F. ) ;
#5104=EDGE_CURVE ( 'NONE', #21168, #14334, #19571, .T. ) ;
#5105=CARTESIAN_POINT ( 'NONE',  ( 1.999996625368665182, 69.28203230275516944, -9.999999999999998224 ) ) ;
#5107=CIRCLE ( 'NONE', #26048, 3.000000000000002665 ) ;
#5108=ORIENTED_EDGE ( 'NONE', *, *, #5986, .F. ) ;
#5109=EDGE_CURVE ( 'NONE', #2284, #902, #29721, .T. ) ;
#5110=CARTESIAN_POINT ( 'NONE',  ( -28.00000337463118427, 69.28203230275516944, -9.999999999999998224 ) ) ;
#5111=ORIENTED_EDGE ( 'NONE', *, *, #31864, .T. ) ;
#5113=VERTEX_POINT ( 'NONE', #9811 ) ;
#5114=AXIS2_PLACEMENT_3D ( 'NONE', #34847, #8975, #12309 ) ;
#5115=DIRECTION ( 'NONE',  ( 0.000000000000000000, 0.000000000000000000, 1.000000000000000000 ) ) ;
#5116=LINE ( 'NONE', #19746, #23839 ) ;
#5117=VERTEX_POINT ( 'NONE', #24456 ) ;
#5118=EDGE_LOOP ( 'NONE', ( #7955, #6356, #14327, #8441, #11510 ) ) ;
#5120=AXIS2_PLACEMENT_3D ( 'NONE', #23375, #4043, #32524 ) ;
#5124=DIRECTION ( 'NONE',  ( 0.000000000000000000, 0.000000000000000000, 1.000000000000000000 ) ) ;
#5125=AXIS2_PLACEMENT_3D ( 'NONE', #20620, #6895, #26966 ) ;
#5126=CARTESIAN_POINT ( 'NONE',  ( -13.00000337463125710, -77.94228634059960825, -9.999999999999998224 ) ) ;
#5127=VERTEX_POINT ( 'NONE', #9645 ) ;
#5128=CARTESIAN_POINT ( 'NONE',  ( -70.00000337463099243, 17.32050807568877460, 17.49999999999999645 ) ) ;
#5129=FACE_BOUND ( 'NONE', #25098, .T. ) ;
#5131=DIRECTION ( 'NONE',  ( 1.000000000000000000, 0.000000000000000000, 0.000000000000000000 ) ) ;
#5132=DIRECTION ( 'NONE',  ( 1.000000000000000000, 0.000000000000000000, 0.000000000000000000 ) ) ;
#5133=EDGE_CURVE ( 'NONE', #30504, #8840, #25537, .T. ) ;
#5134=CARTESIAN_POINT ( 'NONE',  ( -58.88972745734155723, 34.00000000000049027, -49.22241343995295892 ) ) ;
#5136=VECTOR ( 'NONE', #19379, 1000.000000000000000 ) ;
#5137=CARTESIAN_POINT ( 'NONE',  ( 14.99999662536863632, -77.94228634059960825, -9.999999999999998224 ) ) ;
#5138=ORIENTED_EDGE ( 'NONE', *, *, #19930, .T. ) ;
#5139=DIRECTION ( 'NONE',  ( 1.000000000000000000, 0.000000000000000000, 0.000000000000000000 ) ) ;
#5140=AXIS2_PLACEMENT_3D ( 'NONE', #19575, #34207, #19764 ) ;
#5142=CARTESIAN_POINT ( 'NONE',  ( -65.00000337463102085, 25.98076211353317433, -5.000000000000000000 ) ) ;
#5143=VECTOR ( 'NONE', #17765, 1000.000000000000000 ) ;
#5144=VECTOR ( 'NONE', #10909, 1000.000000000000000 ) ;
#5145=AXIS2_PLACEMENT_3D ( 'NONE', #15489, #30092, #35389 ) ;
#5146=ORIENTED_EDGE ( 'NONE', *, *, #18566, .F. ) ;
#5147=CIRCLE ( 'NONE', #30876, 3.000000000000008882 ) ;
#5148=VERTEX_POINT ( 'NONE', #15455 ) ;
#5150=CARTESIAN_POINT ( 'NONE',  ( 12.99999662536859901, 77.94228634059957983, -9.999999999999998224 ) ) ;
#5151=CARTESIAN_POINT ( 'NONE',  ( 4.999996625368645198, 77.94228634059957983, 17.49999999999999645 ) ) ;
#5152=ORIENTED_EDGE ( 'NONE', *, *, #17840, .F. ) ;
#5155=DIRECTION ( 'NONE',  ( 1.000000000000000000, 0.000000000000000000, 0.000000000000000000 ) ) ;
#5157=EDGE_CURVE ( 'NONE', #21984, #10822, #27060, .T. ) ;
#5158=CARTESIAN_POINT ( 'NONE',  ( -56.67878100130369035, 27.78182860042797131, -4.999999999999997335 ) ) ;
#5159=ORIENTED_EDGE ( 'NONE', *, *, #27853, .F. ) ;
#5160=PLANE ( 'NONE',  #24343 ) ;
#5161=VECTOR ( 'NONE', #26343, 1000.000000000000000 ) ;
#5162=DIRECTION ( 'NONE',  ( 0.000000000000000000, 0.000000000000000000, 1.000000000000000000 ) ) ;
#5163=CARTESIAN_POINT ( 'NONE',  ( -29.97040610772328861, 71.28181329121154874, 12.50000000000000000 ) ) ;
#5165=ORIENTED_EDGE ( 'NONE', *, *, #800, .F. ) ;
#5167=CARTESIAN_POINT ( 'NONE',  ( -58.88972745734155723, 34.00000000000049027, -4.999999999999997335 ) ) ;
#5169=CIRCLE ( 'NONE', #3364, 2.000000000000001776 ) ;
#5170=CIRCLE ( 'NONE', #5757, 2.000000000000001776 ) ;
#5171=DIRECTION ( 'NONE',  ( 1.000000000000000000, 0.000000000000000000, 0.000000000000000000 ) ) ;
#5172=FACE_OUTER_BOUND ( 'NONE', #19366, .T. ) ;
#5173=CIRCLE ( 'NONE', #23126, 2.000000000000001776 ) ;
#5175=DIRECTION ( 'NONE',  ( 0.000000000000000000, 0.000000000000000000, -1.000000000000000000 ) ) ;
#5176=CARTESIAN_POINT ( 'NONE',  ( 62.99999662536839651, -60.62177826491080168, 17.49999999999999645 ) ) ;
#5177=ORIENTED_EDGE ( 'NONE', *, *, #26667, .T. ) ;
#5179=CARTESIAN_POINT ( 'NONE',  ( 17.99999662536858125, 86.60254037844397601, -5.000000000000000000 ) ) ;
#5180=DIRECTION ( 'NONE',  ( 1.000000000000000000, 0.000000000000000000, 0.000000000000000000 ) ) ;
#5182=DIRECTION ( 'NONE',  ( -1.000000000000000000, 0.000000000000000000, 0.000000000000000000 ) ) ;
#5183=CIRCLE ( 'NONE', #33340, 2.000000000000001776 ) ;
#5185=VERTEX_POINT ( 'NONE', #6643 ) ;
#5186=EDGE_CURVE ( 'NONE', #32494, #5564, #9976, .T. ) ;
#5187=DIRECTION ( 'NONE',  ( 0.000000000000000000, 0.000000000000000000, 1.000000000000000000 ) ) ;
#5188=CYLINDRICAL_SURFACE ( 'NONE', #14132, 2.000000000000001776 ) ;
#5189=AXIS2_PLACEMENT_3D ( 'NONE', #31720, #23476, #6053 ) ;
#5190=DIRECTION ( 'NONE',  ( 0.000000000000000000, 0.000000000000000000, 1.000000000000000000 ) ) ;
#5191=EDGE_CURVE ( 'NONE', #34395, #35595, #12968, .T. ) ;
#5192=ORIENTED_EDGE ( 'NONE', *, *, #2949, .T. ) ;
#5193=VERTEX_POINT ( 'NONE', #4381 ) ;
#5196=CARTESIAN_POINT ( 'NONE',  ( -73.00000337463097821, 25.98076211353318854, -9.999999999999998224 ) ) ;
#5197=VECTOR ( 'NONE', #24818, 1000.000000000000000 ) ;
#5198=ORIENTED_EDGE ( 'NONE', *, *, #15391, .F. ) ;
#5199=CIRCLE ( 'NONE', #26737, 2.000000000000001776 ) ;
#5201=CARTESIAN_POINT ( 'NONE',  ( -65.00000000000000000, 0.000000000000000000, 12.49999999999999822 ) ) ;
#5202=AXIS2_PLACEMENT_3D ( 'NONE', #870, #12287, #23762 ) ;
#5203=DIRECTION ( 'NONE',  ( 0.000000000000000000, 0.000000000000000000, 1.000000000000000000 ) ) ;
#5204=ORIENTED_EDGE ( 'NONE', *, *, #28086, .F. ) ;
#5207=ORIENTED_EDGE ( 'NONE', *, *, #12798, .T. ) ;
#5208=FACE_BOUND ( 'NONE', #25050, .T. ) ;
#5209=AXIS2_PLACEMENT_3D ( 'NONE', #31707, #6040, #14842 ) ;
#5212=ORIENTED_EDGE ( 'NONE', *, *, #8159, .T. ) ;
#5215=EDGE_CURVE ( 'NONE', #18101, #31393, #7012, .T. ) ;
#5219=DIRECTION ( 'NONE',  ( 1.000000000000000000, 0.000000000000000000, 0.000000000000000000 ) ) ;
#5220=CIRCLE ( 'NONE', #7520, 33.00000000000001421 ) ;
#5221=EDGE_CURVE ( 'NONE', #5127, #18549, #14150, .T. ) ;
#5223=FACE_OUTER_BOUND ( 'NONE', #15709, .T. ) ;
#5224=ADVANCED_FACE ( 'NONE', ( #35147 ), #14344, .F. ) ;
#5226=DIRECTION ( 'NONE',  ( 1.000000000000000000, 0.000000000000000000, 0.000000000000000000 ) ) ;
#5227=VECTOR ( 'NONE', #23511, 1000.000000000000000 ) ;
#5228=VECTOR ( 'NONE', #4138, 1000.000000000000000 ) ;
#5229=ORIENTED_EDGE ( 'NONE', *, *, #22616, .F. ) ;
#5230=VECTOR ( 'NONE', #7010, 1000.000000000000000 ) ;
#5231=AXIS2_PLACEMENT_3D ( 'NONE', #16381, #19378, #10572 ) ;
#5233=DIRECTION ( 'NONE',  ( 0.000000000000000000, 0.000000000000000000, 1.000000000000000000 ) ) ;
#5234=EDGE_LOOP ( 'NONE', ( #20249, #28405, #5656, #36141 ) ) ;
#5235=EDGE_CURVE ( 'NONE', #31695, #203, #29101, .T. ) ;
#5236=DIRECTION ( 'NONE',  ( -1.000000000000000000, 0.000000000000000000, 0.000000000000000000 ) ) ;
#5237=CYLINDRICAL_SURFACE ( 'NONE', #14784, 2.000000000000001776 ) ;
#5238=AXIS2_PLACEMENT_3D ( 'NONE', #21591, #18192, #9591 ) ;
#5239=DIRECTION ( 'NONE',  ( 0.000000000000000000, 0.000000000000000000, 1.000000000000000000 ) ) ;
#5241=DIRECTION ( 'NONE',  ( 0.000000000000000000, 0.000000000000000000, 1.000000000000000000 ) ) ;
#5242=CARTESIAN_POINT ( 'NONE',  ( 17.99999662536858835, 69.28203230275516944, 12.50000000000000000 ) ) ;
#5243=DIRECTION ( 'NONE',  ( -0.5000000000000098810, -0.8660254037844328234, 0.000000000000000000 ) ) ;
#5244=DIRECTION ( 'NONE',  ( 0.000000000000000000, 0.000000000000000000, 1.000000000000000000 ) ) ;
#5246=CYLINDRICAL_SURFACE ( 'NONE', #19077, 2.000000000000001776 ) ;
#5247=VERTEX_POINT ( 'NONE', #21635 ) ;
#5249=ORIENTED_EDGE ( 'NONE', *, *, #34389, .T. ) ;
#5250=DIRECTION ( 'NONE',  ( 0.000000000000000000, 0.000000000000000000, 1.000000000000000000 ) ) ;
#5251=CIRCLE ( 'NONE', #26171, 2.000000000000001776 ) ;
#5252=CYLINDRICAL_SURFACE ( 'NONE', #10967, 2.000000000000001776 ) ;
#5254=CARTESIAN_POINT ( 'NONE',  ( -31.83425564451526668, -89.42901512340343118, -5.000000000000011546 ) ) ;
#5255=ORIENTED_EDGE ( 'NONE', *, *, #18796, .T. ) ;
#5257=AXIS2_PLACEMENT_3D ( 'NONE', #23023, #5982, #17411 ) ;
#5258=VECTOR ( 'NONE', #30231, 1000.000000000000000 ) ;
#5260=CARTESIAN_POINT ( 'NONE',  ( 4.999996625368676284, -77.94228634059960825, 12.50000000000000000 ) ) ;
#5261=VERTEX_POINT ( 'NONE', #23905 ) ;
#5262=EDGE_LOOP ( 'NONE', ( #29125, #22914 ) ) ;
#5264=ORIENTED_EDGE ( 'NONE', *, *, #9126, .F. ) ;
#5267=DIRECTION ( 'NONE',  ( 0.000000000000000000, 0.000000000000000000, 1.000000000000000000 ) ) ;
#5272=LINE ( 'NONE', #16707, #22079 ) ;
#5273=EDGE_CURVE ( 'NONE', #13581, #14423, #4584, .T. ) ;
#5274=ORIENTED_EDGE ( 'NONE', *, *, #22868, .F. ) ;
#5276=AXIS2_PLACEMENT_3D ( 'NONE', #18096, #29354, #15483 ) ;
#5277=VECTOR ( 'NONE', #33202, 1000.000000000000000 ) ;
#5278=ORIENTED_EDGE ( 'NONE', *, *, #5323, .T. ) ;
#5279=VECTOR ( 'NONE', #23564, 1000.000000000000000 ) ;
#5280=ORIENTED_EDGE ( 'NONE', *, *, #31373, .F. ) ;
#5281=CIRCLE ( 'NONE', #11233, 2.000000000000001776 ) ;
#5282=ORIENTED_EDGE ( 'NONE', *, *, #36128, .F. ) ;
#5283=CARTESIAN_POINT ( 'NONE',  ( -55.88972745734155012, 34.00000000000049027, 12.49999999999999822 ) ) ;
#5284=LINE ( 'NONE', #27950, #32752 ) ;
#5285=CARTESIAN_POINT ( 'NONE',  ( -32.00000337463119848, -69.28203230275522628, 12.50000000000000000 ) ) ;
#5287=CARTESIAN_POINT ( 'NONE',  ( -80.00000337463096400, -34.64101615137762025, -5.000000000000000000 ) ) ;
#5290=AXIS2_PLACEMENT_3D ( 'NONE', #13545, #10136, #33169 ) ;
#5292=DIRECTION ( 'NONE',  ( 0.000000000000000000, 0.000000000000000000, -1.000000000000000000 ) ) ;
#5293=VERTEX_POINT ( 'NONE', #25013 ) ;
#5294=DIRECTION ( 'NONE',  ( 0.000000000000000000, 0.000000000000000000, 1.000000000000000000 ) ) ;
#5296=VECTOR ( 'NONE', #4296, 1000.000000000000000 ) ;
#5297=ORIENTED_EDGE ( 'NONE', *, *, #26934, .F. ) ;
#5298=ORIENTED_EDGE ( 'NONE', *, *, #23183, .F. ) ;
#5299=DIRECTION ( 'NONE',  ( 0.000000000000000000, 0.000000000000000000, 1.000000000000000000 ) ) ;
#5303=CARTESIAN_POINT ( 'NONE',  ( -92.00000337463090716, -1.016341149603137227E-14, -5.000000000000000000 ) ) ;
#5304=ORIENTED_EDGE ( 'NONE', *, *, #33888, .T. ) ;
#5306=AXIS2_PLACEMENT_3D ( 'NONE', #31793, #23388, #3304 ) ;
#5307=CIRCLE ( 'NONE', #35174, 2.000000000000001776 ) ;
#5309=ADVANCED_FACE ( 'NONE', ( #16204 ), #4770, .F. ) ;
#5310=AXIS2_PLACEMENT_3D ( 'NONE', #35277, #9374, #20811 ) ;
#5311=ORIENTED_EDGE ( 'NONE', *, *, #28365, .F. ) ;
#5312=ADVANCED_FACE ( 'NONE', ( #19561 ), #33243, .F. ) ;
#5313=DIRECTION ( 'NONE',  ( -1.000000000000000000, 0.000000000000000000, 0.000000000000000000 ) ) ;
#5315=AXIS2_PLACEMENT_3D ( 'NONE', #3199, #380, #31324 ) ;
#5316=DIRECTION ( 'NONE',  ( 1.000000000000000000, 0.000000000000000000, 0.000000000000000000 ) ) ;
#5317=ADVANCED_FACE ( 'NONE', ( #27795 ), #36448, .F. ) ;
#5318=AXIS2_PLACEMENT_3D ( 'NONE', #9465, #26340, #6464 ) ;
#5319=CARTESIAN_POINT ( 'NONE',  ( -48.00000337463110611, -69.28203230275519786, 17.49999999999999645 ) ) ;
#5320=DIRECTION ( 'NONE',  ( 0.000000000000000000, 0.000000000000000000, 1.000000000000000000 ) ) ;
#5321=ORIENTED_EDGE ( 'NONE', *, *, #15546, .T. ) ;
#5322=ORIENTED_EDGE ( 'NONE', *, *, #32012, .F. ) ;
#5323=EDGE_CURVE ( 'NONE', #9159, #12004, #30991, .T. ) ;
#5325=FACE_OUTER_BOUND ( 'NONE', #26325, .T. ) ;
#5326=ADVANCED_FACE ( 'NONE', ( #5325 ), #16922, .F. ) ;
#5327=CYLINDRICAL_SURFACE ( 'NONE', #24678, 2.000000000000001776 ) ;
#5328=CARTESIAN_POINT ( 'NONE',  ( -70.00000337463099243, 34.64101615137758472, -9.999999999999998224 ) ) ;
#5332=FACE_BOUND ( 'NONE', #18711, .T. ) ;
#5333=EDGE_CURVE ( 'NONE', #20237, #26555, #25366, .T. ) ;
#5335=DIRECTION ( 'NONE',  ( 0.000000000000000000, 0.000000000000000000, 1.000000000000000000 ) ) ;
#5336=FACE_OUTER_BOUND ( 'NONE', #34082, .T. ) ;
#5337=LINE ( 'NONE', #8127, #320 ) ;
#5339=CARTESIAN_POINT ( 'NONE',  ( 19.99999662536861678, -86.60254037844400443, -9.999999999999998224 ) ) ;
#5341=FACE_OUTER_BOUND ( 'NONE', #18621, .T. ) ;
#5342=EDGE_CURVE ( 'NONE', #27334, #28791, #10922, .T. ) ;
#5343=ADVANCED_FACE ( 'NONE', ( #27992 ), #36252, .F. ) ;
#5344=CIRCLE ( 'NONE', #20306, 3.000000000000002665 ) ;
#5345=CARTESIAN_POINT ( 'NONE',  ( 69.99999662536839651, 34.64101615137758472, -9.999999999999998224 ) ) ;
#5347=DIRECTION ( 'NONE',  ( -1.000000000000000000, 0.000000000000000000, 0.000000000000000000 ) ) ;
#5348=DIRECTION ( 'NONE',  ( -1.000000000000000000, 0.000000000000000000, 0.000000000000000000 ) ) ;
#5349=PLANE ( 'NONE',  #17981 ) ;
#5350=ORIENTED_EDGE ( 'NONE', *, *, #949, .F. ) ;
#5351=EDGE_LOOP ( 'NONE', ( #20713, #34438, #30276, #15553 ) ) ;
#5352=AXIS2_PLACEMENT_3D ( 'NONE', #33543, #28082, #19280 ) ;
#5353=VERTEX_POINT ( 'NONE', #2318 ) ;
#5354=CARTESIAN_POINT ( 'NONE',  ( 24.99999662536859546, -77.94228634059960825, -5.000000000000000000 ) ) ;
#5355=FACE_OUTER_BOUND ( 'NONE', #29675, .T. ) ;
#5358=AXIS2_PLACEMENT_3D ( 'NONE', #29580, #3908, #26792 ) ;
#5359=ORIENTED_EDGE ( 'NONE', *, *, #14597, .F. ) ;
#5360=CARTESIAN_POINT ( 'NONE',  ( -66.98486643701050980, 43.54686869003479899, 12.50000000000000000 ) ) ;
#5361=ORIENTED_EDGE ( 'NONE', *, *, #31654, .F. ) ;
#5362=DIRECTION ( 'NONE',  ( 0.000000000000000000, 0.000000000000000000, 1.000000000000000000 ) ) ;
#5363=ORIENTED_EDGE ( 'NONE', *, *, #23431, .F. ) ;
#5364=CARTESIAN_POINT ( 'NONE',  ( -43.00000337463111322, -77.94228634059960825, 17.49999999999999645 ) ) ;
#5365=CYLINDRICAL_SURFACE ( 'NONE', #22147, 2.000000000000001776 ) ;
#5366=VECTOR ( 'NONE', #7047, 1000.000000000000000 ) ;
#5368=CARTESIAN_POINT ( 'NONE',  ( 72.99999662536836809, -8.660254037844401509, -9.999999999999998224 ) ) ;
#5370=CARTESIAN_POINT ( 'NONE',  ( 11.99999662536865763, -69.28203230275519786, -9.999999999999998224 ) ) ;
#5371=DIRECTION ( 'NONE',  ( 1.000000000000000000, 0.000000000000000000, 0.000000000000000000 ) ) ;
#5372=VECTOR ( 'NONE', #12269, 1000.000000000000000 ) ;
#5374=DIRECTION ( 'NONE',  ( 1.000000000000000000, 0.000000000000000000, 0.000000000000000000 ) ) ;
#5376=EDGE_LOOP ( 'NONE', ( #29401, #5304 ) ) ;
#5377=CIRCLE ( 'NONE', #1158, 33.00000000000001421 ) ;
#5378=CARTESIAN_POINT ( 'NONE',  ( -80.00000337463094979, 34.64101615137757051, -9.999999999999998224 ) ) ;
#5380=FACE_OUTER_BOUND ( 'NONE', #11142, .T. ) ;
#5382=EDGE_LOOP ( 'NONE', ( #12370, #2552 ) ) ;
#5383=CIRCLE ( 'NONE', #15540, 2.000000000000001776 ) ;
#5385=ORIENTED_EDGE ( 'NONE', *, *, #29396, .T. ) ;
#5386=CARTESIAN_POINT ( 'NONE',  ( 9.999996625368655856, -86.60254037844400443, 17.49999999999999645 ) ) ;
#5387=DIRECTION ( 'NONE',  ( 0.000000000000000000, 0.000000000000000000, 1.000000000000000000 ) ) ;
#5388=VERTEX_POINT ( 'NONE', #30441 ) ;
#5391=DIRECTION ( 'NONE',  ( 0.000000000000000000, 0.000000000000000000, -1.000000000000000000 ) ) ;
#5394=ORIENTED_EDGE ( 'NONE', *, *, #30263, .F. ) ;
#5395=EDGE_LOOP ( 'NONE', ( #19397, #34925 ) ) ;
#5396=DIRECTION ( 'NONE',  ( -1.000000000000000000, 0.000000000000000000, 0.000000000000000000 ) ) ;
#5397=AXIS2_PLACEMENT_3D ( 'NONE', #19317, #30176, #16317 ) ;
#5399=ORIENTED_EDGE ( 'NONE', *, *, #4497, .T. ) ;
#5400=DIRECTION ( 'NONE',  ( -0.000000000000000000, 0.000000000000000000, -1.000000000000000000 ) ) ;
#5401=ORIENTED_EDGE ( 'NONE', *, *, #729, .F. ) ;
#5402=FACE_BOUND ( 'NONE', #21764, .T. ) ;
#5403=CIRCLE ( 'NONE', #13772, 2.000000000000001776 ) ;
#5404=ADVANCED_FACE ( 'NONE', ( #33631 ), #7934, .F. ) ;
#5405=EDGE_CURVE ( 'NONE', #3127, #22150, #31510, .T. ) ;
#5406=DIRECTION ( 'NONE',  ( 1.000000000000000000, 0.000000000000000000, 0.000000000000000000 ) ) ;
#5407=AXIS2_PLACEMENT_3D ( 'NONE', #27495, #19419, #30838 ) ;
#5408=CIRCLE ( 'NONE', #16193, 2.000000000000001776 ) ;
#5409=ORIENTED_EDGE ( 'NONE', *, *, #461, .T. ) ;
#5411=CYLINDRICAL_SURFACE ( 'NONE', #14661, 2.000000000000001776 ) ;
#5412=ADVANCED_FACE ( 'NONE', ( #8118 ), #31181, .F. ) ;
#5414=DIRECTION ( 'NONE',  ( 0.000000000000000000, 0.000000000000000000, 1.000000000000000000 ) ) ;
#5415=VERTEX_POINT ( 'NONE', #25553 ) ;
#5417=DIRECTION ( 'NONE',  ( 1.000000000000000000, 0.000000000000000000, 0.000000000000000000 ) ) ;
#5418=CARTESIAN_POINT ( 'NONE',  ( -72.00000337463102085, -51.96152422706641971, -9.999999999999998224 ) ) ;
#5419=DIRECTION ( 'NONE',  ( -1.000000000000000000, 0.000000000000000000, 0.000000000000000000 ) ) ;
#5420=AXIS2_PLACEMENT_3D ( 'NONE', #28121, #21749, #33183 ) ;
#5421=EDGE_LOOP ( 'NONE', ( #14886, #17296, #2109, #5255 ) ) ;
#5422=ORIENTED_EDGE ( 'NONE', *, *, #5986, .T. ) ;
#5423=EDGE_CURVE ( 'NONE', #12033, #29187, #15352, .T. ) ;
#5425=DIRECTION ( 'NONE',  ( 0.000000000000000000, 0.000000000000000000, 1.000000000000000000 ) ) ;
#5426=CIRCLE ( 'NONE', #26373, 2.000000000000000000 ) ;
#5427=DIRECTION ( 'NONE',  ( 1.000000000000000000, 0.000000000000000000, 0.000000000000000000 ) ) ;
#5429=DIRECTION ( 'NONE',  ( 0.8660254037844415942, 0.4999999999999949485, 0.000000000000000000 ) ) ;
#5432=CARTESIAN_POINT ( 'NONE',  ( -65.00000337463102085, 25.98076211353317433, -5.000000000000000000 ) ) ;
#5434=ORIENTED_EDGE ( 'NONE', *, *, #19072, .F. ) ;
#5436=ORIENTED_EDGE ( 'NONE', *, *, #14831, .T. ) ;
#5437=DIRECTION ( 'NONE',  ( -1.000000000000000000, 0.000000000000000000, 0.000000000000000000 ) ) ;
#5438=EDGE_CURVE ( 'NONE', #16509, #21044, #29079, .T. ) ;
#5439=CARTESIAN_POINT ( 'NONE',  ( 61.99999662536843914, -34.64101615137759893, 17.49999999999999645 ) ) ;
#5440=DIRECTION ( 'NONE',  ( -1.000000000000000000, 0.000000000000000000, 0.000000000000000000 ) ) ;
#5442=ORIENTED_EDGE ( 'NONE', *, *, #30402, .T. ) ;
#5443=UNCERTAINTY_MEASURE_WITH_UNIT (LENGTH_MEASURE( 1.000000000000000082E-05 ), #4517, 'distance_accuracy_value', 'NONE');
#5444=EDGE_CURVE ( 'NONE', #16686, #11450, #31343, .T. ) ;
#5445=FACE_BOUND ( 'NONE', #26045, .T. ) ;
#5446=ORIENTED_EDGE ( 'NONE', *, *, #24969, .T. ) ;
#5447=VERTEX_POINT ( 'NONE', #11305 ) ;
#5450=ORIENTED_EDGE ( 'NONE', *, *, #26667, .F. ) ;
#5451=CARTESIAN_POINT ( 'NONE',  ( -3.374631334790434423E-06, 69.28203230275516944, -9.999999999999998224 ) ) ;
#5452=CARTESIAN_POINT ( 'NONE',  ( 31.99999662536856704, 69.28203230275518365, -5.000000000000000000 ) ) ;
#5453=EDGE_CURVE ( 'NONE', #21264, #21182, #19918, .T. ) ;
#5454=DIRECTION ( 'NONE',  ( 1.000000000000000000, 0.000000000000000000, 0.000000000000000000 ) ) ;
#5455=ORIENTED_EDGE ( 'NONE', *, *, #33103, .F. ) ;
#5456=ORIENTED_EDGE ( 'NONE', *, *, #34431, .T. ) ;
#5458=ORIENTED_EDGE ( 'NONE', *, *, #7849, .F. ) ;
#5459=ORIENTED_EDGE ( 'NONE', *, *, #31836, .T. ) ;
#5460=CARTESIAN_POINT ( 'NONE',  ( 54.99999662536844625, -60.62177826491080168, 12.50000000000000000 ) ) ;
#5461=DIRECTION ( 'NONE',  ( 1.000000000000000000, 0.000000000000000000, 0.000000000000000000 ) ) ;
#5462=DIRECTION ( 'NONE',  ( 0.000000000000000000, 0.000000000000000000, 1.000000000000000000 ) ) ;
#5463=DIRECTION ( 'NONE',  ( 1.000000000000000000, 0.000000000000000000, 0.000000000000000000 ) ) ;
#5465=VERTEX_POINT ( 'NONE', #23294 ) ;
#5467=EDGE_CURVE ( 'NONE', #406, #20086, #32121, .T. ) ;
#5468=CARTESIAN_POINT ( 'NONE',  ( -65.00000337463104927, -43.30127018922202353, -5.000000000000000000 ) ) ;
#5469=DIRECTION ( 'NONE',  ( 0.4999999999999919509, -0.8660254037844433705, 0.000000000000000000 ) ) ;
#5470=VERTEX_POINT ( 'NONE', #9035 ) ;
#5471=CYLINDRICAL_SURFACE ( 'NONE', #11259, 2.000000000000001776 ) ;
#5472=CARTESIAN_POINT ( 'NONE',  ( -51.13139720814379530, 27.50000000000055422, -10.00000000000000178 ) ) ;
#5473=VERTEX_POINT ( 'NONE', #26096 ) ;
#5475=VERTEX_POINT ( 'NONE', #17107 ) ;
#5476=CYLINDRICAL_SURFACE ( 'NONE', #18240, 2.000000000000001776 ) ;
#5477=EDGE_CURVE ( 'NONE', #8103, #28577, #36937, .T. ) ;
#5478=DIRECTION ( 'NONE',  ( 0.000000000000000000, 0.000000000000000000, -1.000000000000000000 ) ) ;
#5481=ORIENTED_EDGE ( 'NONE', *, *, #1794, .F. ) ;
#5482=ORIENTED_EDGE ( 'NONE', *, *, #6964, .F. ) ;
#5483=DIRECTION ( 'NONE',  ( -1.000000000000000000, -8.994862468027885935E-16, 0.000000000000000000 ) ) ;
#5484=ORIENTED_EDGE ( 'NONE', *, *, #36172, .F. ) ;
#5485=AXIS2_PLACEMENT_3D ( 'NONE', #19860, #14033, #25485 ) ;
#5486=DIRECTION ( 'NONE',  ( -1.000000000000000000, 0.000000000000000000, 0.000000000000000000 ) ) ;
#5487=ORIENTED_EDGE ( 'NONE', *, *, #33894, .F. ) ;
#5488=VERTEX_POINT ( 'NONE', #6214 ) ;
#5491=EDGE_CURVE ( 'NONE', #281, #3592, #10696, .T. ) ;
#5492=DIRECTION ( 'NONE',  ( -1.000000000000000000, 0.000000000000000000, 0.000000000000000000 ) ) ;
#5493=VERTEX_POINT ( 'NONE', #34359 ) ;
#5494=ORIENTED_EDGE ( 'NONE', *, *, #21590, .F. ) ;
#5496=DIRECTION ( 'NONE',  ( 1.000000000000000000, 0.000000000000000000, 0.000000000000000000 ) ) ;
#5497=CARTESIAN_POINT ( 'NONE',  ( 13.89091430021463935, 62.33939050065170306, 12.49999999999999822 ) ) ;
#5499=ORIENTED_EDGE ( 'NONE', *, *, #11864, .F. ) ;
#5500=CARTESIAN_POINT ( 'NONE',  ( -36.97203788308986105, 58.48108235278859013, -4.999999999999997335 ) ) ;
#5501=FACE_BOUND ( 'NONE', #35424, .T. ) ;
#5503=CARTESIAN_POINT ( 'NONE',  ( -90.60231327712325822, -15.97563234535699017, -49.86561046011506448 ) ) ;
#5505=FACE_OUTER_BOUND ( 'NONE', #5873, .T. ) ;
#5511=EDGE_CURVE ( 'NONE', #29140, #34620, #8490, .T. ) ;
#5513=FACE_OUTER_BOUND ( 'NONE', #20011, .T. ) ;
#5516=ADVANCED_FACE ( 'NONE', ( #211 ), #28346, .F. ) ;
#5518=EDGE_LOOP ( 'NONE', ( #36607, #1065, #18068, #14849 ) ) ;
#5519=CYLINDRICAL_SURFACE ( 'NONE', #12331, 1.999999999999998224 ) ;
#5521=EDGE_CURVE ( 'NONE', #15624, #8981, #11642, .T. ) ;
#5524=LINE ( 'NONE', #33837, #21516 ) ;
#5525=ORIENTED_EDGE ( 'NONE', *, *, #6407, .T. ) ;
#5527=ORIENTED_EDGE ( 'NONE', *, *, #10048, .F. ) ;
#5528=DIRECTION ( 'NONE',  ( 0.000000000000000000, 0.000000000000000000, 1.000000000000000000 ) ) ;
#5529=EDGE_CURVE ( 'NONE', #28630, #19593, #28733, .T. ) ;
#5530=VERTEX_POINT ( 'NONE', #34546 ) ;
#5531=EDGE_CURVE ( 'NONE', #17059, #7036, #14859, .T. ) ;
#5532=DIRECTION ( 'NONE',  ( 0.000000000000000000, 0.000000000000000000, 1.000000000000000000 ) ) ;
#5533=CARTESIAN_POINT ( 'NONE',  ( 33.99999999999986500, -58.88972745734191250, 12.49999999999999822 ) ) ;
#5534=EDGE_CURVE ( 'NONE', #19701, #31662, #11276, .T. ) ;
#5535=ADVANCED_FACE ( 'NONE', ( #29277 ), #4678, .F. ) ;
#5536=ORIENTED_EDGE ( 'NONE', *, *, #8297, .T. ) ;
#5537=DIRECTION ( 'NONE',  ( 0.000000000000000000, 0.000000000000000000, 1.000000000000000000 ) ) ;
#5539=DIRECTION ( 'NONE',  ( 1.000000000000000000, 0.000000000000000000, 0.000000000000000000 ) ) ;
#5540=CARTESIAN_POINT ( 'NONE',  ( -85.00000337463092137, 8.660254037844389075, -9.999999999999998224 ) ) ;
#5541=ORIENTED_EDGE ( 'NONE', *, *, #23082, .T. ) ;
#5542=FACE_OUTER_BOUND ( 'NONE', #13616, .T. ) ;
#5544=ORIENTED_EDGE ( 'NONE', *, *, #34515, .F. ) ;
#5545=CYLINDRICAL_SURFACE ( 'NONE', #425, 2.000000000000001776 ) ;
#5546=FACE_OUTER_BOUND ( 'NONE', #27278, .T. ) ;
#5547=CARTESIAN_POINT ( 'NONE',  ( 15.97563234535730814, -90.60231327712320137, 12.49999999999999822 ) ) ;
#5548=DIRECTION ( 'NONE',  ( 0.000000000000000000, 0.000000000000000000, -1.000000000000000000 ) ) ;
#5549=ORIENTED_EDGE ( 'NONE', *, *, #22393, .F. ) ;
#5550=ORIENTED_EDGE ( 'NONE', *, *, #2321, .T. ) ;
#5551=DIRECTION ( 'NONE',  ( -1.000000000000000000, 0.000000000000000000, -0.000000000000000000 ) ) ;
#5552=CARTESIAN_POINT ( 'NONE',  ( 51.99999662536847467, 51.96152422706637708, -9.999999999999998224 ) ) ;
#5553=VERTEX_POINT ( 'NONE', #24729 ) ;
#5557=CYLINDRICAL_SURFACE ( 'NONE', #20799, 2.000000000000001776 ) ;
#5558=FACE_OUTER_BOUND ( 'NONE', #3030, .T. ) ;
#5559=VERTEX_POINT ( 'NONE', #36162 ) ;
#5560=VERTEX_POINT ( 'NONE', #12183 ) ;
#5562=DIRECTION ( 'NONE',  ( 0.000000000000000000, 0.000000000000000000, -1.000000000000000000 ) ) ;
#5563=CYLINDRICAL_SURFACE ( 'NONE', #26057, 1.999999999999998224 ) ;
#5564=VERTEX_POINT ( 'NONE', #7666 ) ;
#5565=DIRECTION ( 'NONE',  ( 1.000000000000000000, 0.000000000000000000, 0.000000000000000000 ) ) ;
#5566=ORIENTED_EDGE ( 'NONE', *, *, #23638, .F. ) ;
#5567=FACE_BOUND ( 'NONE', #28915, .T. ) ;
#5568=EDGE_CURVE ( 'NONE', #24605, #30139, #767, .T. ) ;
#5571=EDGE_CURVE ( 'NONE', #34006, #9332, #23861, .T. ) ;
#5572=EDGE_CURVE ( 'NONE', #21745, #6695, #28640, .T. ) ;
#5573=ORIENTED_EDGE ( 'NONE', *, *, #32457, .T. ) ;
#5575=FACE_OUTER_BOUND ( 'NONE', #2183, .T. ) ;
#5576=CIRCLE ( 'NONE', #12730, 2.000000000000001776 ) ;
#5581=DIRECTION ( 'NONE',  ( 0.000000000000000000, 0.000000000000000000, 1.000000000000000000 ) ) ;
#5582=CARTESIAN_POINT ( 'NONE',  ( -85.00000337463092137, -25.98076211353322051, -5.000000000000000000 ) ) ;
#5583=VERTEX_POINT ( 'NONE', #15033 ) ;
#5584=VERTEX_POINT ( 'NONE', #26460 ) ;
#5585=ORIENTED_EDGE ( 'NONE', *, *, #8745, .T. ) ;
#5586=FACE_OUTER_BOUND ( 'NONE', #16492, .T. ) ;
#5587=AXIS2_PLACEMENT_3D ( 'NONE', #18436, #6624, #32659 ) ;
#5589=EDGE_CURVE ( 'NONE', #26322, #36878, #21719, .T. ) ;
#5590=AXIS2_PLACEMENT_3D ( 'NONE', #8786, #333, #35598 ) ;
#5596=DIRECTION ( 'NONE',  ( 1.000000000000000000, 0.000000000000000000, 0.000000000000000000 ) ) ;
#5597=ORIENTED_EDGE ( 'NONE', *, *, #8868, .F. ) ;
#5598=AXIS2_PLACEMENT_3D ( 'NONE', #36501, #10801, #28041 ) ;
#5599=EDGE_LOOP ( 'NONE', ( #12777, #35180, #19986, #24095 ) ) ;
#5602=DIRECTION ( 'NONE',  ( 1.000000000000000000, 0.000000000000000000, 0.000000000000000000 ) ) ;
#5603=DIRECTION ( 'NONE',  ( 0.000000000000000000, 0.000000000000000000, 1.000000000000000000 ) ) ;
#5605=ORIENTED_EDGE ( 'NONE', *, *, #12567, .F. ) ;
#5606=AXIS2_PLACEMENT_3D ( 'NONE', #20357, #5936, #11170 ) ;
#5607=FACE_BOUND ( 'NONE', #429, .T. ) ;
#5608=ORIENTED_EDGE ( 'NONE', *, *, #34183, .F. ) ;
#5609=ORIENTED_EDGE ( 'NONE', *, *, #5438, .T. ) ;
#5610=EDGE_CURVE ( 'NONE', #902, #3385, #37036, .T. ) ;
#5612=ORIENTED_EDGE ( 'NONE', *, *, #16330, .F. ) ;
#5614=CARTESIAN_POINT ( 'NONE',  ( 74.99999662536836809, -8.660254037844401509, -9.999999999999998224 ) ) ;
#5616=CARTESIAN_POINT ( 'NONE',  ( 54.99999662536844625, 60.62177826491077326, -9.999999999999998224 ) ) ;
#5617=CARTESIAN_POINT ( 'NONE',  ( 69.99999662536838230, -51.96152422706639840, 12.50000000000000000 ) ) ;
#5618=ORIENTED_EDGE ( 'NONE', *, *, #17941, .T. ) ;
#5620=ORIENTED_EDGE ( 'NONE', *, *, #7055, .T. ) ;
#5621=VECTOR ( 'NONE', #32537, 1000.000000000000000 ) ;
#5622=ORIENTED_EDGE ( 'NONE', *, *, #5323, .F. ) ;
#5623=EDGE_LOOP ( 'NONE', ( #5926, #32484, #2209, #27208 ) ) ;
#5625=CIRCLE ( 'NONE', #14585, 2.000000000000001776 ) ;
#5626=CARTESIAN_POINT ( 'NONE',  ( -57.00000337463111322, -43.30127018922202353, 17.49999999999999645 ) ) ;
#5628=DIRECTION ( 'NONE',  ( 1.000000000000000000, 0.000000000000000000, 0.000000000000000000 ) ) ;
#5629=DIRECTION ( 'NONE',  ( 1.000000000000000000, 0.000000000000000000, 0.000000000000000000 ) ) ;
#5630=ADVANCED_FACE ( 'NONE', ( #12899 ), #24355, .T. ) ;
#5631=ORIENTED_EDGE ( 'NONE', *, *, #4870, .T. ) ;
#5632=DIRECTION ( 'NONE',  ( 0.000000000000000000, 0.000000000000000000, 1.000000000000000000 ) ) ;
#5633=LINE ( 'NONE', #17275, #8992 ) ;
#5634=DIRECTION ( 'NONE',  ( 0.000000000000000000, 0.000000000000000000, 1.000000000000000000 ) ) ;
#5635=ORIENTED_EDGE ( 'NONE', *, *, #14250, .T. ) ;
#5636=DIRECTION ( 'NONE',  ( -1.000000000000000000, 0.000000000000000000, 0.000000000000000000 ) ) ;
#5637=EDGE_CURVE ( 'NONE', #35831, #32910, #4476, .T. ) ;
#5638=DIRECTION ( 'NONE',  ( -0.8660254037844455910, -0.4999999999999878431, 0.000000000000000000 ) ) ;
#5639=EDGE_LOOP ( 'NONE', ( #15835, #8141, #21391, #25745 ) ) ;
#5640=CIRCLE ( 'NONE', #25403, 2.000000000000001776 ) ;
#5643=DIRECTION ( 'NONE',  ( 0.000000000000000000, 0.000000000000000000, 1.000000000000000000 ) ) ;
#5645=LINE ( 'NONE', #8301, #2515 ) ;
#5646=DIRECTION ( 'NONE',  ( 0.000000000000000000, 0.000000000000000000, 1.000000000000000000 ) ) ;
#5647=VERTEX_POINT ( 'NONE', #18559 ) ;
#5648=ORIENTED_EDGE ( 'NONE', *, *, #31414, .T. ) ;
#5650=CYLINDRICAL_SURFACE ( 'NONE', #3322, 2.000000000000001776 ) ;
#5651=DIRECTION ( 'NONE',  ( -1.000000000000000000, 0.000000000000000000, 0.000000000000000000 ) ) ;
#5653=ORIENTED_EDGE ( 'NONE', *, *, #11287, .T. ) ;
#5654=EDGE_CURVE ( 'NONE', #7645, #17074, #16663, .T. ) ;
#5655=CARTESIAN_POINT ( 'NONE',  ( 83.49774710563264080, -24.66044155380014402, -5.000000000000000000 ) ) ;
#5656=ORIENTED_EDGE ( 'NONE', *, *, #3410, .F. ) ;
#5657=ORIENTED_EDGE ( 'NONE', *, *, #11577, .T. ) ;
#5659=CARTESIAN_POINT ( 'NONE',  ( -48.00000337463109190, 51.96152422706637708, -5.000000000000000000 ) ) ;
#5660=CIRCLE ( 'NONE', #13528, 2.000000000000000000 ) ;
#5661=FACE_BOUND ( 'NONE', #5737, .T. ) ;
#5662=EDGE_LOOP ( 'NONE', ( #14126, #34485, #29872, #15244 ) ) ;
#5667=EDGE_CURVE ( 'NONE', #5415, #16153, #19082, .T. ) ;
#5669=CARTESIAN_POINT ( 'NONE',  ( -62.97617850287781494, -4.279621169095772615, -4.999999999999997335 ) ) ;
#5671=DIRECTION ( 'NONE',  ( 0.000000000000000000, 0.000000000000000000, 1.000000000000000000 ) ) ;
#5672=ADVANCED_FACE ( 'NONE', ( #27344 ), #18730, .F. ) ;
#5673=FACE_BOUND ( 'NONE', #3440, .T. ) ;
#5674=CYLINDRICAL_SURFACE ( 'NONE', #16616, 2.000000000000001776 ) ;
#5675=CARTESIAN_POINT ( 'NONE',  ( 19.13981058454793072, -60.93295298010985306, 12.49999999999999822 ) ) ;
#5676=FACE_OUTER_BOUND ( 'NONE', #24590, .T. ) ;
#5677=DIRECTION ( 'NONE',  ( 0.000000000000000000, 0.000000000000000000, 1.000000000000000000 ) ) ;
#5678=CIRCLE ( 'NONE', #14046, 2.000000000000001776 ) ;
#5679=EDGE_CURVE ( 'NONE', #23785, #29460, #28032, .T. ) ;
#5680=CIRCLE ( 'NONE', #12233, 27.00000000000001421 ) ;
#5681=DIRECTION ( 'NONE',  ( -1.000000000000000000, 0.000000000000000000, 0.000000000000000000 ) ) ;
#5684=CARTESIAN_POINT ( 'NONE',  ( -75.00000337463097821, 43.30127018922197379, -5.000000000000000000 ) ) ;
#5685=ORIENTED_EDGE ( 'NONE', *, *, #1310, .T. ) ;
#5686=DIRECTION ( 'NONE',  ( 1.000000000000000000, 0.000000000000000000, 0.000000000000000000 ) ) ;
#5687=EDGE_CURVE ( 'NONE', #12630, #5993, #12467, .T. ) ;
#5688=CARTESIAN_POINT ( 'NONE',  ( 74.99999662536836809, -8.660254037844401509, 12.50000000000000000 ) ) ;
#5689=CARTESIAN_POINT ( 'NONE',  ( -25.00000337463120914, 77.94228634059957983, -9.999999999999998224 ) ) ;
#5690=ORIENTED_EDGE ( 'NONE', *, *, #10819, .F. ) ;
#5691=EDGE_LOOP ( 'NONE', ( #1645, #19043 ) ) ;
#5692=ORIENTED_EDGE ( 'NONE', *, *, #35597, .T. ) ;
#5693=ADVANCED_FACE ( 'NONE', ( #18913 ), #16116, .F. ) ;
#5696=DIRECTION ( 'NONE',  ( 0.000000000000000000, 0.000000000000000000, 1.000000000000000000 ) ) ;
#5697=CIRCLE ( 'NONE', #10483, 2.000000000000001776 ) ;
#5698=CARTESIAN_POINT ( 'NONE',  ( 14.80603122773119118, -87.83969979969866415, -4.999999999999997335 ) ) ;
#5699=VERTEX_POINT ( 'NONE', #19290 ) ;
#5700=CIRCLE ( 'NONE', #5732, 2.000000000000000000 ) ;
#5702=CARTESIAN_POINT ( 'NONE',  ( 2.999996625368645198, 77.94228634059957983, -5.000000000000000000 ) ) ;
#5703=EDGE_LOOP ( 'NONE', ( #28947, #13400, #26881, #34096 ) ) ;
#5704=DIRECTION ( 'NONE',  ( -1.000000000000000000, 1.798972493605577187E-15, 0.000000000000000000 ) ) ;
#5705=VERTEX_POINT ( 'NONE', #11558 ) ;
#5706=DIRECTION ( 'NONE',  ( 0.000000000000000000, 0.000000000000000000, -1.000000000000000000 ) ) ;
#5707=EDGE_LOOP ( 'NONE', ( #27266, #7839, #4199, #649 ) ) ;
#5708=CIRCLE ( 'NONE', #24880, 33.00000000000002132 ) ;
#5709=EDGE_LOOP ( 'NONE', ( #22541, #7241, #33591, #26599 ) ) ;
#5711=EDGE_CURVE ( 'NONE', #12879, #25301, #17280, .T. ) ;
#5713=DIRECTION ( 'NONE',  ( 0.000000000000000000, 0.000000000000000000, 1.000000000000000000 ) ) ;
#5714=ORIENTED_EDGE ( 'NONE', *, *, #28098, .T. ) ;
#5715=CARTESIAN_POINT ( 'NONE',  ( 69.99999662536838230, -51.96152422706639840, -9.999999999999998224 ) ) ;
#5717=EDGE_CURVE ( 'NONE', #35764, #28135, #18490, .T. ) ;
#5721=ORIENTED_EDGE ( 'NONE', *, *, #36200, .T. ) ;
#5722=DIRECTION ( 'NONE',  ( 0.000000000000000000, 0.000000000000000000, 1.000000000000000000 ) ) ;
#5723=FACE_OUTER_BOUND ( 'NONE', #4846, .T. ) ;
#5724=EDGE_CURVE ( 'NONE', #30650, #1757, #2317, .T. ) ;
#5725=VERTEX_POINT ( 'NONE', #28638 ) ;
#5726=CARTESIAN_POINT ( 'NONE',  ( 7.122621931239992550E-13, 68.00000000000000000, 12.49999999999999822 ) ) ;
#5727=AXIS2_PLACEMENT_3D ( 'NONE', #18039, #14490, #14660 ) ;
#5728=EDGE_CURVE ( 'NONE', #15109, #9425, #11847, .T. ) ;
#5729=CARTESIAN_POINT ( 'NONE',  ( -67.00000337463102085, 60.62177826491077326, -9.999999999999998224 ) ) ;
#5731=AXIS2_PLACEMENT_3D ( 'NONE', #29063, #14291, #14836 ) ;
#5732=AXIS2_PLACEMENT_3D ( 'NONE', #32964, #18143, #1648 ) ;
#5735=VERTEX_POINT ( 'NONE', #28265 ) ;
#5736=VECTOR ( 'NONE', #3764, 1000.000000000000000 ) ;
#5737=EDGE_LOOP ( 'NONE', ( #24273, #27245 ) ) ;
#5738=CARTESIAN_POINT ( 'NONE',  ( -43.00000337463111322, -77.94228634059960825, -9.999999999999998224 ) ) ;
#5739=LINE ( 'NONE', #34254, #9803 ) ;
#5740=CIRCLE ( 'NONE', #23694, 2.000000000000001776 ) ;
#5741=VERTEX_POINT ( 'NONE', #36713 ) ;
#5742=ORIENTED_EDGE ( 'NONE', *, *, #21967, .T. ) ;
#5743=EDGE_CURVE ( 'NONE', #26422, #21946, #1700, .T. ) ;
#5744=DIRECTION ( 'NONE',  ( -0.000000000000000000, 0.000000000000000000, -1.000000000000000000 ) ) ;
#5745=DIRECTION ( 'NONE',  ( 0.000000000000000000, 0.000000000000000000, -1.000000000000000000 ) ) ;
#5746=DIRECTION ( 'NONE',  ( -0.000000000000000000, -0.000000000000000000, 1.000000000000000000 ) ) ;
#5747=EDGE_LOOP ( 'NONE', ( #10837, #962, #32016, #22866, #12723, #14069, #22623, #4523, #6373, #19311, #17991, #35602, #21785, #11422, #16988, #22383, #26959, #6556, #9313, #7228, #14880, #20971, #18334, #1230 ) ) ;
#5748=AXIS2_PLACEMENT_3D ( 'NONE', #21644, #1942, #33642 ) ;
#5749=DIRECTION ( 'NONE',  ( 1.000000000000000000, 0.000000000000000000, 0.000000000000000000 ) ) ;
#5750=VERTEX_POINT ( 'NONE', #37095 ) ;
#5751=CARTESIAN_POINT ( 'NONE',  ( 39.99999662536853151, 69.28203230275518365, -9.999999999999998224 ) ) ;
#5752=EDGE_LOOP ( 'NONE', ( #32441, #3564 ) ) ;
#5753=FACE_BOUND ( 'NONE', #1815, .T. ) ;
#5754=VECTOR ( 'NONE', #16148, 1000.000000000000000 ) ;
#5757=AXIS2_PLACEMENT_3D ( 'NONE', #34028, #36467, #2893 ) ;
#5758=AXIS2_PLACEMENT_3D ( 'NONE', #3966, #14010, #13453 ) ;
#5759=EDGE_CURVE ( 'NONE', #19312, #15209, #485, .T. ) ;
#5763=ORIENTED_EDGE ( 'NONE', *, *, #23290, .T. ) ;
#5765=AXIS2_PLACEMENT_3D ( 'NONE', #3398, #14834, #11458 ) ;
#5766=EDGE_CURVE ( 'NONE', #15986, #17720, #21448, .T. ) ;
#5767=CARTESIAN_POINT ( 'NONE',  ( -75.00000337463099243, -25.98076211353322051, 17.49999999999999645 ) ) ;
#5769=DIRECTION ( 'NONE',  ( 0.000000000000000000, 0.000000000000000000, -1.000000000000000000 ) ) ;
#5770=VERTEX_POINT ( 'NONE', #10848 ) ;
#5771=DIRECTION ( 'NONE',  ( 0.000000000000000000, 0.000000000000000000, 1.000000000000000000 ) ) ;
#5772=EDGE_CURVE ( 'NONE', #36626, #19079, #31030, .T. ) ;
#5773=DIRECTION ( 'NONE',  ( 0.000000000000000000, 0.000000000000000000, 1.000000000000000000 ) ) ;
#5774=CARTESIAN_POINT ( 'NONE',  ( -68.00000337463099243, 17.32050807568877460, -5.000000000000000000 ) ) ;
#5775=ADVANCED_FACE ( 'NONE', ( #5223 ), #25662, .F. ) ;
#5776=AXIS2_PLACEMENT_3D ( 'NONE', #3471, #3271, #14706 ) ;
#5777=VERTEX_POINT ( 'NONE', #28440 ) ;
#5778=ORIENTED_EDGE ( 'NONE', *, *, #21162, .F. ) ;
#5780=ORIENTED_EDGE ( 'NONE', *, *, #24013, .F. ) ;
#5783=AXIS2_PLACEMENT_3D ( 'NONE', #29387, #15133, #6700 ) ;
#5784=EDGE_CURVE ( 'NONE', #16909, #8594, #2772, .T. ) ;
#5785=AXIS2_PLACEMENT_3D ( 'NONE', #26478, #12199, #23668 ) ;
#5786=EDGE_CURVE ( 'NONE', #22308, #30710, #4709, .T. ) ;
#5787=CARTESIAN_POINT ( 'NONE',  ( 52.99999662536846046, -43.30127018922200222, -9.999999999999998224 ) ) ;
#5788=CIRCLE ( 'NONE', #15357, 2.000000000000000000 ) ;
#5790=EDGE_CURVE ( 'NONE', #13632, #5750, #31057, .T. ) ;
#5793=CYLINDRICAL_SURFACE ( 'NONE', #20702, 2.000000000000001776 ) ;
#5794=DIRECTION ( 'NONE',  ( -1.000000000000000000, 0.000000000000000000, 0.000000000000000000 ) ) ;
#5797=AXIS2_PLACEMENT_3D ( 'NONE', #2152, #13594, #28031 ) ;
#5798=ORIENTED_EDGE ( 'NONE', *, *, #1259, .T. ) ;
#5800=DIRECTION ( 'NONE',  ( 1.000000000000000000, 0.000000000000000000, 0.000000000000000000 ) ) ;
#5801=DIRECTION ( 'NONE',  ( 1.000000000000000000, 0.000000000000000000, 0.000000000000000000 ) ) ;
#5802=CARTESIAN_POINT ( 'NONE',  ( -65.00000337463102085, 43.30127018922198801, 12.50000000000000000 ) ) ;
#5805=AXIS2_PLACEMENT_3D ( 'NONE', #24004, #7305, #15738 ) ;
#5806=CARTESIAN_POINT ( 'NONE',  ( 31.27962116909601420, -62.97617850287780072, -4.999999999999997335 ) ) ;
#5807=ORIENTED_EDGE ( 'NONE', *, *, #13744, .T. ) ;
#5809=CARTESIAN_POINT ( 'NONE',  ( -38.00000337463113453, -69.28203230275519786, -9.999999999999998224 ) ) ;
#5810=EDGE_LOOP ( 'NONE', ( #15299, #27496 ) ) ;
#5814=DIRECTION ( 'NONE',  ( 1.000000000000000000, 0.000000000000000000, 0.000000000000000000 ) ) ;
#5815=VECTOR ( 'NONE', #13562, 1000.000000000000000 ) ;
#5816=DIRECTION ( 'NONE',  ( 0.000000000000000000, 0.000000000000000000, 1.000000000000000000 ) ) ;
#5817=VERTEX_POINT ( 'NONE', #33721 ) ;
#5818=EDGE_LOOP ( 'NONE', ( #27589, #29699, #25715, #12969 ) ) ;
#5821=VECTOR ( 'NONE', #15632, 1000.000000000000000 ) ;
#5822=VERTEX_POINT ( 'NONE', #8023 ) ;
#5823=ORIENTED_EDGE ( 'NONE', *, *, #27328, .T. ) ;
#5824=FACE_OUTER_BOUND ( 'NONE', #9459, .T. ) ;
#5825=DIRECTION ( 'NONE',  ( 0.000000000000000000, 0.000000000000000000, -1.000000000000000000 ) ) ;
#5826=AXIS2_PLACEMENT_3D ( 'NONE', #24466, #4581, #35906 ) ;
#5828=CARTESIAN_POINT ( 'NONE',  ( -62.00000337463107769, -34.64101615137762025, -9.999999999999998224 ) ) ;
#5830=FACE_OUTER_BOUND ( 'NONE', #24686, .T. ) ;
#5834=ADVANCED_FACE ( 'NONE', ( #16660 ), #2416, .F. ) ;
#5835=CARTESIAN_POINT ( 'NONE',  ( 17.99999662536861678, -69.28203230275519786, -9.999999999999998224 ) ) ;
#5836=ORIENTED_EDGE ( 'NONE', *, *, #6002, .T. ) ;
#5837=FACE_OUTER_BOUND ( 'NONE', #11541, .T. ) ;
#5838=CYLINDRICAL_SURFACE ( 'NONE', #29167, 2.000000000000000000 ) ;
#5839=AXIS2_PLACEMENT_3D ( 'NONE', #32318, #34779, #6082 ) ;
#5840=VERTEX_POINT ( 'NONE', #33903 ) ;
#5841=AXIS2_PLACEMENT_3D ( 'NONE', #6145, #26403, #3333 ) ;
#5842=ORIENTED_EDGE ( 'NONE', *, *, #22571, .F. ) ;
#5843=AXIS2_PLACEMENT_3D ( 'NONE', #35349, #34951, #23341 ) ;
#5844=CARTESIAN_POINT ( 'NONE',  ( 52.39915983220795681, 35.19434990244919703, 12.49999999999999822 ) ) ;
#5845=DIRECTION ( 'NONE',  ( 1.000000000000000000, 0.000000000000000000, 0.000000000000000000 ) ) ;
#5847=CARTESIAN_POINT ( 'NONE',  ( -79.83584802575171580, -32.64776428033012934, -5.000000000000000000 ) ) ;
#5848=ORIENTED_EDGE ( 'NONE', *, *, #19549, .T. ) ;
#5850=AXIS2_PLACEMENT_3D ( 'NONE', #26201, #6692, #17397 ) ;
#5851=DIRECTION ( 'NONE',  ( 0.000000000000000000, 0.000000000000000000, 1.000000000000000000 ) ) ;
#5856=AXIS2_PLACEMENT_3D ( 'NONE', #27758, #7719, #13711 ) ;
#5857=DIRECTION ( 'NONE',  ( 1.000000000000000000, 0.000000000000000000, 0.000000000000000000 ) ) ;
#5858=ORIENTED_EDGE ( 'NONE', *, *, #4540, .T. ) ;
#5859=EDGE_CURVE ( 'NONE', #1125, #22827, #28057, .T. ) ;
#5860=EDGE_CURVE ( 'NONE', #17303, #6640, #23267, .T. ) ;
#5861=VECTOR ( 'NONE', #22453, 1000.000000000000000 ) ;
#5862=EDGE_LOOP ( 'NONE', ( #6667, #36625, #36718, #34464 ) ) ;
#5864=CIRCLE ( 'NONE', #10655, 2.000000000000001776 ) ;
#5865=DIRECTION ( 'NONE',  ( -1.000000000000000000, 0.000000000000000000, 0.000000000000000000 ) ) ;
#5866=ORIENTED_EDGE ( 'NONE', *, *, #9576, .T. ) ;
#5867=ORIENTED_EDGE ( 'NONE', *, *, #2139, .F. ) ;
#5868=DIRECTION ( 'NONE',  ( 0.000000000000000000, 0.000000000000000000, 1.000000000000000000 ) ) ;
#5869=DIRECTION ( 'NONE',  ( 0.000000000000000000, 0.000000000000000000, 1.000000000000000000 ) ) ;
#5870=DIRECTION ( 'NONE',  ( 0.000000000000000000, 0.000000000000000000, 1.000000000000000000 ) ) ;
#5871=AXIS2_PLACEMENT_3D ( 'NONE', #23703, #12057, #3652 ) ;
#5872=ADVANCED_FACE ( 'NONE', ( #6311 ), #9306, .T. ) ;
#5873=EDGE_LOOP ( 'NONE', ( #32178, #9799, #26930 ) ) ;
#5874=DIRECTION ( 'NONE',  ( 0.000000000000000000, 0.000000000000000000, 1.000000000000000000 ) ) ;
#5875=FACE_BOUND ( 'NONE', #36860, .T. ) ;
#5877=DIRECTION ( 'NONE',  ( 0.000000000000000000, 0.000000000000000000, -1.000000000000000000 ) ) ;
#5878=CIRCLE ( 'NONE', #20241, 2.000000000000001776 ) ;
#5879=CARTESIAN_POINT ( 'NONE',  ( -12.00000337463128197, 86.60254037844397601, -5.000000000000000000 ) ) ;
#5880=DIRECTION ( 'NONE',  ( 1.000000000000000000, 0.000000000000000000, 0.000000000000000000 ) ) ;
#5882=CARTESIAN_POINT ( 'NONE',  ( 9.999996625368625658, 86.60254037844397601, 12.50000000000000000 ) ) ;
#5883=AXIS2_PLACEMENT_3D ( 'NONE', #16158, #12748, #29835 ) ;
#5884=EDGE_CURVE ( 'NONE', #9210, #36782, #16695, .T. ) ;
#5885=DIRECTION ( 'NONE',  ( 0.000000000000000000, 0.000000000000000000, 1.000000000000000000 ) ) ;
#5886=ORIENTED_EDGE ( 'NONE', *, *, #26187, .T. ) ;
#5887=DIRECTION ( 'NONE',  ( -0.5000000000000112133, -0.8660254037844322683, 0.000000000000000000 ) ) ;
#5888=AXIS2_PLACEMENT_3D ( 'NONE', #26721, #24102, #18487 ) ;
#5889=CIRCLE ( 'NONE', #37045, 95.00000000000001421 ) ;
#5890=FACE_BOUND ( 'NONE', #29207, .T. ) ;
#5893=VERTEX_POINT ( 'NONE', #32179 ) ;
#5894=ORIENTED_EDGE ( 'NONE', *, *, #20040, .T. ) ;
#5895=VERTEX_POINT ( 'NONE', #35005 ) ;
#5898=CARTESIAN_POINT ( 'NONE',  ( -72.00000337463102085, -34.64101615137762025, 12.50000000000000000 ) ) ;
#5903=EDGE_LOOP ( 'NONE', ( #6803, #33611 ) ) ;
#5905=FACE_OUTER_BOUND ( 'NONE', #33697, .T. ) ;
#5906=ORIENTED_EDGE ( 'NONE', *, *, #6463, .F. ) ;
#5908=ORIENTED_EDGE ( 'NONE', *, *, #11943, .T. ) ;
#5909=EDGE_LOOP ( 'NONE', ( #31566, #32402, #28800, #21060, #7469, #33330, #34789, #158 ) ) ;
#5911=DIRECTION ( 'NONE',  ( -1.000000000000000000, 0.000000000000000000, 0.000000000000000000 ) ) ;
#5912=VECTOR ( 'NONE', #2264, 1000.000000000000000 ) ;
#5913=DIRECTION ( 'NONE',  ( 1.000000000000000000, 0.000000000000000000, 0.000000000000000000 ) ) ;
#5914=EDGE_CURVE ( 'NONE', #12313, #8445, #8233, .T. ) ;
#5915=VERTEX_POINT ( 'NONE', #20741 ) ;
#5916=FACE_OUTER_BOUND ( 'NONE', #7589, .T. ) ;
#5917=VECTOR ( 'NONE', #20005, 1000.000000000000000 ) ;
#5918=AXIS2_PLACEMENT_3D ( 'NONE', #11703, #25805, #465 ) ;
#5919=DIRECTION ( 'NONE',  ( -0.000000000000000000, -0.000000000000000000, 1.000000000000000000 ) ) ;
#5920=CARTESIAN_POINT ( 'NONE',  ( -58.00000337463104216, 51.96152422706639129, -9.999999999999998224 ) ) ;
#5922=AXIS2_PLACEMENT_3D ( 'NONE', #24578, #30358, #24934 ) ;
#5923=ORIENTED_EDGE ( 'NONE', *, *, #24914, .F. ) ;
#5924=CARTESIAN_POINT ( 'NONE',  ( -80.00000337463096400, -34.64101615137762025, -5.000000000000000000 ) ) ;
#5925=CARTESIAN_POINT ( 'NONE',  ( -40.00000337463113453, 69.28203230275516944, -9.999999999999998224 ) ) ;
#5926=ORIENTED_EDGE ( 'NONE', *, *, #20422, .F. ) ;
#5928=CARTESIAN_POINT ( 'NONE',  ( 0.000000000000000000, 0.000000000000000000, 12.49999999999999822 ) ) ;
#5930=VECTOR ( 'NONE', #13134, 1000.000000000000000 ) ;
#5931=LINE ( 'NONE', #101, #31403 ) ;
#5932=VECTOR ( 'NONE', #17846, 1000.000000000000000 ) ;
#5933=CYLINDRICAL_SURFACE ( 'NONE', #29275, 2.000000000000001776 ) ;
#5936=DIRECTION ( 'NONE',  ( 0.000000000000000000, 0.000000000000000000, 1.000000000000000000 ) ) ;
#5938=ORIENTED_EDGE ( 'NONE', *, *, #29573, .F. ) ;
#5939=EDGE_CURVE ( 'NONE', #25343, #10270, #33392, .T. ) ;
#5942=AXIS2_PLACEMENT_3D ( 'NONE', #26003, #690, #125 ) ;
#5943=CARTESIAN_POINT ( 'NONE',  ( -35.00000337463117717, -77.94228634059963667, -9.999999999999998224 ) ) ;
#5944=CARTESIAN_POINT ( 'NONE',  ( -85.00000337463092137, -8.660254037844422825, -5.000000000000000000 ) ) ;
#5945=CYLINDRICAL_SURFACE ( 'NONE', #27832, 2.000000000000001776 ) ;
#5946=EDGE_CURVE ( 'NONE', #15938, #5488, #20948, .T. ) ;
#5947=DIRECTION ( 'NONE',  ( 1.000000000000000000, 0.000000000000000000, 0.000000000000000000 ) ) ;
#5948=ORIENTED_EDGE ( 'NONE', *, *, #15165, .T. ) ;
#5949=AXIS2_PLACEMENT_3D ( 'NONE', #23133, #34586, #77 ) ;
#5950=EDGE_CURVE ( 'NONE', #10634, #26137, #3695, .T. ) ;
#5951=DIRECTION ( 'NONE',  ( 1.000000000000000000, 0.000000000000000000, 0.000000000000000000 ) ) ;
#5952=VERTEX_POINT ( 'NONE', #867 ) ;
#5953=FACE_BOUND ( 'NONE', #15367, .T. ) ;
#5954=CIRCLE ( 'NONE', #8914, 2.000000000000001776 ) ;
#5955=AXIS2_PLACEMENT_3D ( 'NONE', #10275, #21707, #33137 ) ;
#5957=CARTESIAN_POINT ( 'NONE',  ( -72.00000337463100664, 51.96152422706637708, -9.999999999999998224 ) ) ;
#5958=CIRCLE ( 'NONE', #4839, 2.000000000000001776 ) ;
#5959=CARTESIAN_POINT ( 'NONE',  ( 62.99999662536839651, 60.62177826491078747, 17.49999999999999645 ) ) ;
#5962=CIRCLE ( 'NONE', #1162, 27.00000000000001421 ) ;
#5963=ADVANCED_FACE ( 'NONE', ( #29378 ), #15123, .F. ) ;
#5964=CIRCLE ( 'NONE', #4763, 3.000000000000004885 ) ;
#5965=DIRECTION ( 'NONE',  ( 1.000000000000000000, 0.000000000000000000, 0.000000000000000000 ) ) ;
#5966=CARTESIAN_POINT ( 'NONE',  ( -2.000003374631327713, 86.60254037844397601, 17.49999999999999645 ) ) ;
#5967=ORIENTED_EDGE ( 'NONE', *, *, #10642, .T. ) ;
#5968=DIRECTION ( 'NONE',  ( 1.000000000000000000, 0.000000000000000000, 0.000000000000000000 ) ) ;
#5972=EDGE_LOOP ( 'NONE', ( #25885, #29686 ) ) ;
#5975=AXIS2_PLACEMENT_3D ( 'NONE', #18896, #15710, #30327 ) ;
#5976=FACE_BOUND ( 'NONE', #1359, .T. ) ;
#5978=EDGE_CURVE ( 'NONE', #33338, #9891, #1051, .T. ) ;
#5980=CARTESIAN_POINT ( 'NONE',  ( 56.67878100130369035, -27.78182860042797131, -4.999999999999997335 ) ) ;
#5981=EDGE_CURVE ( 'NONE', #9506, #7462, #14215, .T. ) ;
#5982=DIRECTION ( 'NONE',  ( 0.000000000000000000, -0.000000000000000000, -1.000000000000000000 ) ) ;
#5983=VECTOR ( 'NONE', #35656, 1000.000000000000000 ) ;
#5984=DIRECTION ( 'NONE',  ( 0.000000000000000000, 0.000000000000000000, 1.000000000000000000 ) ) ;
#5986=EDGE_CURVE ( 'NONE', #32159, #24412, #26005, .T. ) ;
#5987=EDGE_LOOP ( 'NONE', ( #21795, #6589, #2242, #5249 ) ) ;
#5988=CARTESIAN_POINT ( 'NONE',  ( 36.99999662536855283, -60.62177826491080168, 12.50000000000000000 ) ) ;
#5989=CIRCLE ( 'NONE', #21383, 2.000000000000001776 ) ;
#5991=DIRECTION ( 'NONE',  ( 0.000000000000000000, 0.000000000000000000, -1.000000000000000000 ) ) ;
#5992=EDGE_CURVE ( 'NONE', #2172, #1857, #23206, .T. ) ;
#5993=VERTEX_POINT ( 'NONE', #23397 ) ;
#5995=ADVANCED_FACE ( 'NONE', ( #34828 ), #9122, .F. ) ;
#5996=FACE_BOUND ( 'NONE', #31581, .T. ) ;
#5997=EDGE_LOOP ( 'NONE', ( #29635, #26327, #33515, #1906 ) ) ;
#5998=ORIENTED_EDGE ( 'NONE', *, *, #9096, .T. ) ;
#5999=CYLINDRICAL_SURFACE ( 'NONE', #880, 1.999999999999998224 ) ;
#6000=ORIENTED_EDGE ( 'NONE', *, *, #8976, .T. ) ;
#6001=AXIS2_PLACEMENT_3D ( 'NONE', #9448, #12424, #6248 ) ;
#6002=EDGE_CURVE ( 'NONE', #22484, #18228, #19024, .T. ) ;
#6003=EDGE_CURVE ( 'NONE', #17282, #22792, #24400, .T. ) ;
#6004=CARTESIAN_POINT ( 'NONE',  ( 69.99999662536838230, -34.64101615137759183, -9.999999999999998224 ) ) ;
#6005=EDGE_CURVE ( 'NONE', #24584, #28819, #10250, .T. ) ;
#6006=CARTESIAN_POINT ( 'NONE',  ( 72.99999662536836809, 25.98076211353319565, 17.49999999999999645 ) ) ;
#6007=EDGE_CURVE ( 'NONE', #21544, #5447, #31578, .T. ) ;
#6008=ORIENTED_EDGE ( 'NONE', *, *, #15783, .F. ) ;
#6009=ADVANCED_FACE ( 'NONE', ( #10070 ), #19073, .F. ) ;
#6010=ORIENTED_EDGE ( 'NONE', *, *, #24301, .F. ) ;
#6011=ORIENTED_EDGE ( 'NONE', *, *, #7220, .F. ) ;
#6014=CYLINDRICAL_SURFACE ( 'NONE', #33201, 27.00000000000001066 ) ;
#6015=CIRCLE ( 'NONE', #20796, 2.000000000000001776 ) ;
#6016=CARTESIAN_POINT ( 'NONE',  ( -4.279621169095561228, 62.97617850287782915, 12.49999999999999822 ) ) ;
#6017=DIRECTION ( 'NONE',  ( -1.000000000000000000, 0.000000000000000000, 0.000000000000000000 ) ) ;
#6020=ORIENTED_EDGE ( 'NONE', *, *, #23180, .F. ) ;
#6021=CARTESIAN_POINT ( 'NONE',  ( -72.00000337463100664, 51.96152422706637708, -9.999999999999998224 ) ) ;
#6023=DIRECTION ( 'NONE',  ( 1.000000000000000000, 0.000000000000000000, 0.000000000000000000 ) ) ;
#6026=LINE ( 'NONE', #12158, #33436 ) ;
#6027=CYLINDRICAL_SURFACE ( 'NONE', #11781, 2.000000000000001776 ) ;
#6028=ORIENTED_EDGE ( 'NONE', *, *, #36005, .T. ) ;
#6029=EDGE_LOOP ( 'NONE', ( #28725, #3437 ) ) ;
#6030=DIRECTION ( 'NONE',  ( 1.000000000000000000, 0.000000000000000000, 0.000000000000000000 ) ) ;
#6031=CARTESIAN_POINT ( 'NONE',  ( 41.99999662536853151, 69.28203230275518365, -9.999999999999998224 ) ) ;
#6032=AXIS2_PLACEMENT_3D ( 'NONE', #30764, #22717, #16346 ) ;
#6033=DIRECTION ( 'NONE',  ( -1.000000000000000000, 0.000000000000000000, 0.000000000000000000 ) ) ;
#6034=FACE_OUTER_BOUND ( 'NONE', #17888, .T. ) ;
#6035=ORIENTED_EDGE ( 'NONE', *, *, #27011, .F. ) ;
#6036=DIRECTION ( 'NONE',  ( 1.000000000000000000, 0.000000000000000000, 0.000000000000000000 ) ) ;
#6037=DIRECTION ( 'NONE',  ( 0.000000000000000000, 0.000000000000000000, 1.000000000000000000 ) ) ;
#6039=ORIENTED_EDGE ( 'NONE', *, *, #22238, .F. ) ;
#6040=DIRECTION ( 'NONE',  ( 0.000000000000000000, 0.000000000000000000, -1.000000000000000000 ) ) ;
#6041=EDGE_LOOP ( 'NONE', ( #33797, #13649 ) ) ;
#6045=CARTESIAN_POINT ( 'NONE',  ( -5.000003374631269537, -77.94228634059960825, 17.49999999999999645 ) ) ;
#6046=EDGE_CURVE ( 'NONE', #6156, #14042, #18872, .T. ) ;
#6048=ORIENTED_EDGE ( 'NONE', *, *, #13867, .T. ) ;
#6049=CARTESIAN_POINT ( 'NONE',  ( 52.39915983220795681, 35.19434990244919703, -4.999999999999997335 ) ) ;
#6050=DIRECTION ( 'NONE',  ( 0.000000000000000000, 0.000000000000000000, 1.000000000000000000 ) ) ;
#6051=CYLINDRICAL_SURFACE ( 'NONE', #9509, 2.000000000000001776 ) ;
#6053=DIRECTION ( 'NONE',  ( 1.000000000000000000, 0.000000000000000000, 0.000000000000000000 ) ) ;
#6054=FACE_BOUND ( 'NONE', #14891, .T. ) ;
#6055=CARTESIAN_POINT ( 'NONE',  ( 19.99999662536858835, 69.28203230275516944, 12.50000000000000000 ) ) ;
#6058=CARTESIAN_POINT ( 'NONE',  ( 45.00000000000000711, 0.000000000000000000, -5.000000000000000000 ) ) ;
#6059=CARTESIAN_POINT ( 'NONE',  ( 69.99999662536839651, 17.32050807568879236, -9.999999999999998224 ) ) ;
#6061=VERTEX_POINT ( 'NONE', #4822 ) ;
#6064=DIRECTION ( 'NONE',  ( 1.000000000000000000, 0.000000000000000000, 0.000000000000000000 ) ) ;
#6066=ORIENTED_EDGE ( 'NONE', *, *, #3708, .T. ) ;
#6067=ORIENTED_EDGE ( 'NONE', *, *, #34041, .F. ) ;
#6068=ORIENTED_EDGE ( 'NONE', *, *, #12726, .F. ) ;
#6069=CARTESIAN_POINT ( 'NONE',  ( 19.99999662536861678, -69.28203230275519786, -9.999999999999998224 ) ) ;
#6071=DIRECTION ( 'NONE',  ( 0.000000000000000000, 0.000000000000000000, 1.000000000000000000 ) ) ;
#6072=ORIENTED_EDGE ( 'NONE', *, *, #22021, .F. ) ;
#6074=EDGE_CURVE ( 'NONE', #20247, #33988, #23805, .T. ) ;
#6076=EDGE_LOOP ( 'NONE', ( #14437, #8293, #14825, #8058 ) ) ;
#6077=DIRECTION ( 'NONE',  ( -1.000000000000000000, 0.000000000000000000, 0.000000000000000000 ) ) ;
#6078=ORIENTED_EDGE ( 'NONE', *, *, #30736, .F. ) ;
#6079=CARTESIAN_POINT ( 'NONE',  ( -3.000003374631308173, 77.94228634059957983, -5.000000000000000000 ) ) ;
#6080=ORIENTED_EDGE ( 'NONE', *, *, #23134, .F. ) ;
#6081=ORIENTED_EDGE ( 'NONE', *, *, #16288, .F. ) ;
#6082=DIRECTION ( 'NONE',  ( 1.000000000000000000, 0.000000000000000000, 0.000000000000000000 ) ) ;
#6084=FACE_OUTER_BOUND ( 'NONE', #19992, .T. ) ;
#6085=EDGE_CURVE ( 'NONE', #34784, #9159, #2857, .T. ) ;
#6087=ORIENTED_EDGE ( 'NONE', *, *, #18561, .T. ) ;
#6088=CARTESIAN_POINT ( 'NONE',  ( 56.99999662536846046, -43.30127018922200222, -9.999999999999998224 ) ) ;
#6089=CARTESIAN_POINT ( 'NONE',  ( 3.499999999999991562, -55.00000000000000000, -10.00000000000000000 ) ) ;
#6090=CARTESIAN_POINT ( 'NONE',  ( -65.00000337463106348, -60.62177826491083010, 12.50000000000000000 ) ) ;
#6093=PLANE ( 'NONE',  #594 ) ;
#6095=ORIENTED_EDGE ( 'NONE', *, *, #35889, .F. ) ;
#6096=CARTESIAN_POINT ( 'NONE',  ( -60.00000337463107059, -34.64101615137762025, -9.999999999999998224 ) ) ;
#6097=CIRCLE ( 'NONE', #30042, 2.000000000000001776 ) ;
#6098=CARTESIAN_POINT ( 'NONE',  ( 69.99999662536839651, -3.469446951953614189E-15, -5.000000000000000000 ) ) ;
#6099=CARTESIAN_POINT ( 'NONE',  ( 34.99999662536855283, 60.62177826491078747, -9.999999999999998224 ) ) ;
#6100=DIRECTION ( 'NONE',  ( 1.000000000000000000, 0.000000000000000000, 0.000000000000000000 ) ) ;
#6101=DIRECTION ( 'NONE',  ( -0.4999999999999980016, 0.8660254037844398178, 0.000000000000000000 ) ) ;
#6102=EDGE_CURVE ( 'NONE', #3063, #34990, #16025, .T. ) ;
#6105=LINE ( 'NONE', #34802, #8017 ) ;
#6106=EDGE_CURVE ( 'NONE', #859, #30760, #27975, .T. ) ;
#6108=ORIENTED_EDGE ( 'NONE', *, *, #12609, .T. ) ;
#6109=ORIENTED_EDGE ( 'NONE', *, *, #30397, .T. ) ;
#6110=CYLINDRICAL_SURFACE ( 'NONE', #27798, 2.000000000000001776 ) ;
#6111=DIRECTION ( 'NONE',  ( 1.000000000000000000, 0.000000000000000000, 0.000000000000000000 ) ) ;
#6113=CARTESIAN_POINT ( 'NONE',  ( -7.000003374631307729, 77.94228634059957983, 17.49999999999999645 ) ) ;
#6114=ADVANCED_FACE ( 'NONE', ( #18691 ), #6866, .F. ) ;
#6115=DIRECTION ( 'NONE',  ( 1.000000000000000000, 0.000000000000000000, 0.000000000000000000 ) ) ;
#6116=EDGE_LOOP ( 'NONE', ( #25095, #2446, #23430, #26963 ) ) ;
#6117=CARTESIAN_POINT ( 'NONE',  ( 61.99999662536842493, 51.96152422706639129, -9.999999999999998224 ) ) ;
#6118=EDGE_LOOP ( 'NONE', ( #12284, #226, #36419, #19895 ) ) ;
#6119=FACE_BOUND ( 'NONE', #35341, .T. ) ;
#6120=CYLINDRICAL_SURFACE ( 'NONE', #3542, 2.000000000000000000 ) ;
#6121=DIRECTION ( 'NONE',  ( 1.000000000000000000, 0.000000000000000000, 0.000000000000000000 ) ) ;
#6123=DIRECTION ( 'NONE',  ( 0.000000000000000000, 0.000000000000000000, 1.000000000000000000 ) ) ;
#6125=CARTESIAN_POINT ( 'NONE',  ( -3.374631303565411855E-06, -86.60254037844400443, -5.000000000000000000 ) ) ;
#6126=VECTOR ( 'NONE', #21950, 1000.000000000000000 ) ;
#6127=EDGE_CURVE ( 'NONE', #23686, #6764, #8835, .T. ) ;
#6128=AXIS2_PLACEMENT_3D ( 'NONE', #11081, #13729, #22731 ) ;
#6129=FACE_OUTER_BOUND ( 'NONE', #36974, .T. ) ;
#6130=DIRECTION ( 'NONE',  ( 0.000000000000000000, 0.000000000000000000, -1.000000000000000000 ) ) ;
#6131=ORIENTED_EDGE ( 'NONE', *, *, #16412, .F. ) ;
#6134=DIRECTION ( 'NONE',  ( 0.000000000000000000, 0.000000000000000000, -1.000000000000000000 ) ) ;
#6135=EDGE_CURVE ( 'NONE', #1757, #30650, #11787, .T. ) ;
#6136=ORIENTED_EDGE ( 'NONE', *, *, #32051, .T. ) ;
#6137=EDGE_LOOP ( 'NONE', ( #20883, #11085, #4785 ) ) ;
#6140=EDGE_LOOP ( 'NONE', ( #29870, #32473, #22904, #36445 ) ) ;
#6141=LINE ( 'NONE', #28993, #13533 ) ;
#6142=FACE_BOUND ( 'NONE', #10988, .T. ) ;
#6144=DIRECTION ( 'NONE',  ( -1.000000000000000000, 0.000000000000000000, -0.000000000000000000 ) ) ;
#6145=CARTESIAN_POINT ( 'NONE',  ( -50.00000337463112032, -51.96152422706641971, -9.999999999999998224 ) ) ;
#6146=DIRECTION ( 'NONE',  ( 1.000000000000000000, 0.000000000000000000, 0.000000000000000000 ) ) ;
#6147=ORIENTED_EDGE ( 'NONE', *, *, #23889, .F. ) ;
#6149=AXIS2_PLACEMENT_3D ( 'NONE', #28710, #11997, #32253 ) ;
#6150=DIRECTION ( 'NONE',  ( -0.000000000000000000, -0.000000000000000000, 1.000000000000000000 ) ) ;
#6152=CARTESIAN_POINT ( 'NONE',  ( 93.36492675454790913, 17.14523346298246409, -4.999999999999997335 ) ) ;
#6153=CARTESIAN_POINT ( 'NONE',  ( 44.99999662536849598, 60.62177826491077326, -9.999999999999998224 ) ) ;
#6154=ORIENTED_EDGE ( 'NONE', *, *, #23477, .T. ) ;
#6155=FACE_BOUND ( 'NONE', #33250, .T. ) ;
#6156=VERTEX_POINT ( 'NONE', #19974 ) ;
#6158=ORIENTED_EDGE ( 'NONE', *, *, #15111, .F. ) ;
#6159=CIRCLE ( 'NONE', #31291, 2.000000000000001776 ) ;
#6160=DIRECTION ( 'NONE',  ( 1.000000000000000000, 0.000000000000000000, 0.000000000000000000 ) ) ;
#6161=VERTEX_POINT ( 'NONE', #10972 ) ;
#6162=CYLINDRICAL_SURFACE ( 'NONE', #13428, 2.000000000000001776 ) ;
#6163=ADVANCED_FACE ( 'NONE', ( #36851 ), #7817, .F. ) ;
#6166=ORIENTED_EDGE ( 'NONE', *, *, #13322, .T. ) ;
#6169=ADVANCED_FACE ( 'NONE', ( #10809 ), #5545, .F. ) ;
#6170=ORIENTED_EDGE ( 'NONE', *, *, #4522, .F. ) ;
#6171=AXIS2_PLACEMENT_3D ( 'NONE', #9711, #32574, #24536 ) ;
#6172=ORIENTED_EDGE ( 'NONE', *, *, #13744, .F. ) ;
#6173=DIRECTION ( 'NONE',  ( 1.000000000000000000, 0.000000000000000000, 0.000000000000000000 ) ) ;
#6174=EDGE_CURVE ( 'NONE', #34827, #8340, #29755, .T. ) ;
#6175=CYLINDRICAL_SURFACE ( 'NONE', #621, 2.000000000000000000 ) ;
#6177=CARTESIAN_POINT ( 'NONE',  ( 44.99999662536851019, -60.62177826491080168, -5.000000000000000000 ) ) ;
#6180=ORIENTED_EDGE ( 'NONE', *, *, #9579, .T. ) ;
#6181=CYLINDRICAL_SURFACE ( 'NONE', #4491, 2.000000000000001776 ) ;
#6182=CARTESIAN_POINT ( 'NONE',  ( 12.99999662536859901, 77.94228634059957983, -9.999999999999998224 ) ) ;
#6183=CIRCLE ( 'NONE', #18777, 1.999999999999998224 ) ;
#6184=LINE ( 'NONE', #3747, #11028 ) ;
#6186=CARTESIAN_POINT ( 'NONE',  ( -63.00000337463102085, 25.98076211353317433, -9.999999999999998224 ) ) ;
#6187=FACE_OUTER_BOUND ( 'NONE', #26077, .T. ) ;
#6188=EDGE_CURVE ( 'NONE', #22417, #16140, #26184, .T. ) ;
#6189=ORIENTED_EDGE ( 'NONE', *, *, #20369, .F. ) ;
#6190=EDGE_LOOP ( 'NONE', ( #3055, #17204, #19916, #17862 ) ) ;
#6191=DIRECTION ( 'NONE',  ( 0.000000000000000000, 0.000000000000000000, 1.000000000000000000 ) ) ;
#6192=EDGE_CURVE ( 'NONE', #35130, #28991, #10019, .T. ) ;
#6193=CARTESIAN_POINT ( 'NONE',  ( -73.00000337463097821, -8.660254037844422825, -9.999999999999998224 ) ) ;
#6194=CARTESIAN_POINT ( 'NONE',  ( -50.00000337463110611, -69.28203230275519786, -5.000000000000000000 ) ) ;
#6197=CIRCLE ( 'NONE', #33755, 2.000000000000000000 ) ;
#6199=CARTESIAN_POINT ( 'NONE',  ( 19.99999662536861678, -86.60254037844400443, -9.999999999999998224 ) ) ;
#6201=DIRECTION ( 'NONE',  ( -0.000000000000000000, -0.000000000000000000, 1.000000000000000000 ) ) ;
#6202=AXIS2_PLACEMENT_3D ( 'NONE', #9883, #1438, #26954 ) ;
#6203=ORIENTED_EDGE ( 'NONE', *, *, #13322, .F. ) ;
#6204=DIRECTION ( 'NONE',  ( 1.000000000000000000, 0.000000000000000000, 0.000000000000000000 ) ) ;
#6206=DIRECTION ( 'NONE',  ( 0.000000000000000000, 0.000000000000000000, -1.000000000000000000 ) ) ;
#6207=CIRCLE ( 'NONE', #23581, 2.000000000000001776 ) ;
#6208=DIRECTION ( 'NONE',  ( 0.000000000000000000, 0.000000000000000000, 1.000000000000000000 ) ) ;
#6209=EDGE_CURVE ( 'NONE', #14593, #22384, #11819, .T. ) ;
#6210=CARTESIAN_POINT ( 'NONE',  ( -33.00000337463117006, -77.94228634059963667, -9.999999999999998224 ) ) ;
#6211=ORIENTED_EDGE ( 'NONE', *, *, #826, .T. ) ;
#6212=EDGE_CURVE ( 'NONE', #19957, #18483, #10052, .T. ) ;
#6213=ORIENTED_EDGE ( 'NONE', *, *, #24053, .F. ) ;
#6214=CARTESIAN_POINT ( 'NONE',  ( 61.25926521283102488, -32.16008401677932227, 12.49999999999999645 ) ) ;
#6217=VERTEX_POINT ( 'NONE', #25416 ) ;
#6218=CARTESIAN_POINT ( 'NONE',  ( 74.99999662536836809, 25.98076211353319565, -9.999999999999998224 ) ) ;
#6219=FACE_BOUND ( 'NONE', #9271, .T. ) ;
#6221=CARTESIAN_POINT ( 'NONE',  ( -57.00000337463111322, -43.30127018922202353, -9.999999999999998224 ) ) ;
#6223=CARTESIAN_POINT ( 'NONE',  ( -55.00000337463107059, 43.30127018922197379, -9.999999999999998224 ) ) ;
#6224=DIRECTION ( 'NONE',  ( 0.000000000000000000, 0.000000000000000000, 1.000000000000000000 ) ) ;
#6226=CARTESIAN_POINT ( 'NONE',  ( -63.00000337463104927, -25.98076211353322051, 12.50000000000000000 ) ) ;
#6227=FACE_OUTER_BOUND ( 'NONE', #25491, .T. ) ;
#6229=FACE_OUTER_BOUND ( 'NONE', #10448, .T. ) ;
#6230=FACE_BOUND ( 'NONE', #34854, .T. ) ;
#6231=FACE_OUTER_BOUND ( 'NONE', #16994, .T. ) ;
#6232=EDGE_CURVE ( 'NONE', #36096, #13826, #31003, .T. ) ;
#6233=AXIS2_PLACEMENT_3D ( 'NONE', #11250, #3006, #5814 ) ;
#6234=VERTEX_POINT ( 'NONE', #22067 ) ;
#6235=ADVANCED_FACE ( 'NONE', ( #19252 ), #30667, .F. ) ;
#6238=EDGE_CURVE ( 'NONE', #36749, #4152, #5878, .T. ) ;
#6239=AXIS2_PLACEMENT_3D ( 'NONE', #26062, #11804, #32429 ) ;
#6240=EDGE_CURVE ( 'NONE', #32504, #36248, #4986, .T. ) ;
#6241=CARTESIAN_POINT ( 'NONE',  ( -65.00000337463102085, 43.30127018922198801, -5.000000000000000000 ) ) ;
#6242=CARTESIAN_POINT ( 'NONE',  ( -45.00000337463112743, -60.62177826491080168, -5.000000000000000000 ) ) ;
#6243=DIRECTION ( 'NONE',  ( 0.000000000000000000, 0.000000000000000000, 1.000000000000000000 ) ) ;
#6244=VERTEX_POINT ( 'NONE', #27844 ) ;
#6245=ORIENTED_EDGE ( 'NONE', *, *, #8716, .F. ) ;
#6246=CARTESIAN_POINT ( 'NONE',  ( 59.13646009116148150, -70.47608876694609137, -4.999999999999997335 ) ) ;
#6247=VERTEX_POINT ( 'NONE', #25616 ) ;
#6248=DIRECTION ( 'NONE',  ( 1.000000000000000000, 0.000000000000000000, 0.000000000000000000 ) ) ;
#6249=CIRCLE ( 'NONE', #24209, 2.000000000000001776 ) ;
#6250=ORIENTED_EDGE ( 'NONE', *, *, #15320, .T. ) ;
#6251=CYLINDRICAL_SURFACE ( 'NONE', #21334, 3.000000000000005773 ) ;
#6255=DIRECTION ( 'NONE',  ( 1.000000000000000000, 0.000000000000000000, 0.000000000000000000 ) ) ;
#6257=DIRECTION ( 'NONE',  ( 0.000000000000000000, 0.000000000000000000, -1.000000000000000000 ) ) ;
#6261=AXIS2_PLACEMENT_3D ( 'NONE', #30337, #30145, #13273 ) ;
#6262=CARTESIAN_POINT ( 'NONE',  ( -68.00000337463100664, -17.32050807568882078, 12.50000000000000000 ) ) ;
#6264=DIRECTION ( 'NONE',  ( 0.000000000000000000, 0.000000000000000000, 1.000000000000000000 ) ) ;
#6265=ORIENTED_EDGE ( 'NONE', *, *, #12344, .T. ) ;
#6266=CIRCLE ( 'NONE', #27216, 2.000000000000001776 ) ;
#6267=CYLINDRICAL_SURFACE ( 'NONE', #2153, 1.999999999999998224 ) ;
#6269=VERTEX_POINT ( 'NONE', #16615 ) ;
#6270=CARTESIAN_POINT ( 'NONE',  ( -58.88972745734203329, -33.99999999999965894, -49.86561046011506448 ) ) ;
#6271=DIRECTION ( 'NONE',  ( 1.000000000000000000, 0.000000000000000000, 0.000000000000000000 ) ) ;
#6272=FACE_OUTER_BOUND ( 'NONE', #31179, .T. ) ;
#6274=DIRECTION ( 'NONE',  ( 0.000000000000000000, 0.000000000000000000, 1.000000000000000000 ) ) ;
#6275=AXIS2_PLACEMENT_3D ( 'NONE', #31794, #25998, #17390 ) ;
#6276=CARTESIAN_POINT ( 'NONE',  ( -63.00000337463102085, 25.98076211353317433, -9.999999999999998224 ) ) ;
#6278=CARTESIAN_POINT ( 'NONE',  ( 95.00000000000001421, 0.000000000000000000, -5.000000000000000000 ) ) ;
#6279=AXIS2_PLACEMENT_3D ( 'NONE', #29148, #14912, #26350 ) ;
#6280=DIRECTION ( 'NONE',  ( 0.000000000000000000, 0.000000000000000000, 1.000000000000000000 ) ) ;
#6281=CARTESIAN_POINT ( 'NONE',  ( -80.00000337463094979, -2.428612866367529932E-14, -9.999999999999998224 ) ) ;
#6282=VERTEX_POINT ( 'NONE', #28047 ) ;
#6284=ORIENTED_EDGE ( 'NONE', *, *, #31945, .F. ) ;
#6285=ORIENTED_EDGE ( 'NONE', *, *, #11000, .T. ) ;
#6286=ADVANCED_FACE ( 'NONE', ( #25968 ), #2931, .F. ) ;
#6287=CYLINDRICAL_SURFACE ( 'NONE', #36192, 2.000000000000001776 ) ;
#6289=DIRECTION ( 'NONE',  ( 0.000000000000000000, 0.000000000000000000, 1.000000000000000000 ) ) ;
#6290=AXIS2_PLACEMENT_3D ( 'NONE', #6125, #15118, #2963 ) ;
#6291=CIRCLE ( 'NONE', #25461, 2.000000000000001776 ) ;
#6292=CYLINDRICAL_SURFACE ( 'NONE', #11675, 3.499999999999989342 ) ;
#6293=ORIENTED_EDGE ( 'NONE', *, *, #18999, .T. ) ;
#6294=DIRECTION ( 'NONE',  ( -1.000000000000000000, 0.000000000000000000, 0.000000000000000000 ) ) ;
#6295=ORIENTED_EDGE ( 'NONE', *, *, #31394, .F. ) ;
#6296=FACE_BOUND ( 'NONE', #30432, .T. ) ;
#6297=CARTESIAN_POINT ( 'NONE',  ( 32.99999662536855283, -77.94228634059960825, -9.999999999999998224 ) ) ;
#6298=VECTOR ( 'NONE', #28389, 1000.000000000000000 ) ;
#6300=AXIS2_PLACEMENT_3D ( 'NONE', #5339, #11113, #22932 ) ;
#6301=ORIENTED_EDGE ( 'NONE', *, *, #17558, .T. ) ;
#6302=CARTESIAN_POINT ( 'NONE',  ( -67.00000337463102085, 25.98076211353317433, -9.999999999999998224 ) ) ;
#6305=AXIS2_PLACEMENT_3D ( 'NONE', #19824, #8931, #28423 ) ;
#6306=CIRCLE ( 'NONE', #14681, 33.00000000000002132 ) ;
#6307=CARTESIAN_POINT ( 'NONE',  ( 29.99999662536857770, -69.28203230275519786, -5.000000000000000000 ) ) ;
#6308=DIRECTION ( 'NONE',  ( 0.000000000000000000, 0.000000000000000000, 1.000000000000000000 ) ) ;
#6309=LINE ( 'NONE', #29185, #17337 ) ;
#6311=FACE_OUTER_BOUND ( 'NONE', #34335, .T. ) ;
#6313=CARTESIAN_POINT ( 'NONE',  ( -35.00000337463116296, -60.62177826491080168, -5.000000000000000000 ) ) ;
#6314=AXIS2_PLACEMENT_3D ( 'NONE', #31923, #453, #8903 ) ;
#6316=EDGE_CURVE ( 'NONE', #12117, #7645, #35807, .T. ) ;
#6317=ORIENTED_EDGE ( 'NONE', *, *, #22779, .T. ) ;
#6318=ORIENTED_EDGE ( 'NONE', *, *, #16318, .T. ) ;
#6319=DIRECTION ( 'NONE',  ( 0.000000000000000000, 0.000000000000000000, -1.000000000000000000 ) ) ;
#6320=CARTESIAN_POINT ( 'NONE',  ( -90.60231327712325822, -15.97563234535699017, -4.999999999999997335 ) ) ;
#6321=CIRCLE ( 'NONE', #8741, 2.000000000000001776 ) ;
#6322=EDGE_CURVE ( 'NONE', #16351, #29605, #26829, .T. ) ;
#6323=DIRECTION ( 'NONE',  ( 0.000000000000000000, 0.000000000000000000, -1.000000000000000000 ) ) ;
#6324=DIRECTION ( 'NONE',  ( 1.000000000000000000, 0.000000000000000000, 0.000000000000000000 ) ) ;
#6325=AXIS2_PLACEMENT_3D ( 'NONE', #4536, #3974, #24214 ) ;
#6327=AXIS2_PLACEMENT_3D ( 'NONE', #29390, #23022, #6324 ) ;
#6329=CYLINDRICAL_SURFACE ( 'NONE', #23363, 2.000000000000001776 ) ;
#6330=CIRCLE ( 'NONE', #5145, 2.000000000000001776 ) ;
#6332=ORIENTED_EDGE ( 'NONE', *, *, #8672, .F. ) ;
#6333=CARTESIAN_POINT ( 'NONE',  ( -73.00000337463099243, -25.98076211353322051, -5.000000000000000000 ) ) ;
#6334=DIRECTION ( 'NONE',  ( 0.000000000000000000, 0.000000000000000000, 1.000000000000000000 ) ) ;
#6335=CARTESIAN_POINT ( 'NONE',  ( 68.66839587347284635, 56.74224907228958870, 12.49999999999999645 ) ) ;
#6336=ORIENTED_EDGE ( 'NONE', *, *, #5772, .F. ) ;
#6337=CIRCLE ( 'NONE', #32066, 2.000000000000001776 ) ;
#6339=FACE_BOUND ( 'NONE', #12691, .T. ) ;
#6340=ORIENTED_EDGE ( 'NONE', *, *, #31569, .T. ) ;
#6341=ORIENTED_EDGE ( 'NONE', *, *, #9315, .F. ) ;
#6342=EDGE_CURVE ( 'NONE', #20659, #12315, #10667, .T. ) ;
#6344=ORIENTED_EDGE ( 'NONE', *, *, #31869, .T. ) ;
#6345=CIRCLE ( 'NONE', #9942, 2.000000000000000000 ) ;
#6346=CYLINDRICAL_SURFACE ( 'NONE', #17625, 1.999999999999998224 ) ;
#6347=AXIS2_PLACEMENT_3D ( 'NONE', #14659, #9414, #29459 ) ;
#6349=CARTESIAN_POINT ( 'NONE',  ( 69.13212189986965939, 2.778182860042805125, 12.49999999999999645 ) ) ;
#6350=VERTEX_POINT ( 'NONE', #14359 ) ;
#6351=VERTEX_POINT ( 'NONE', #462 ) ;
#6352=EDGE_CURVE ( 'NONE', #26240, #24381, #25055, .T. ) ;
#6353=COLOUR_RGB ( '', 0.72549020, 0.75294118, 0.79215686) ;
#6354=AXIS2_PLACEMENT_3D ( 'NONE', #29109, #32302, #9230 ) ;
#6355=VECTOR ( 'NONE', #10006, 1000.000000000000000 ) ;
#6356=ORIENTED_EDGE ( 'NONE', *, *, #26715, .T. ) ;
#6357=VECTOR ( 'NONE', #20558, 1000.000000000000000 ) ;
#6358=AXIS2_PLACEMENT_3D ( 'NONE', #16942, #6425, #12031 ) ;
#6360=AXIS2_PLACEMENT_3D ( 'NONE', #6601, #32454, #24559 ) ;
#6362=EDGE_LOOP ( 'NONE', ( #15130, #31334 ) ) ;
#6363=LINE ( 'NONE', #9361, #6867 ) ;
#6364=ORIENTED_EDGE ( 'NONE', *, *, #5078, .T. ) ;
#6365=DIRECTION ( 'NONE',  ( 0.000000000000000000, 0.000000000000000000, 1.000000000000000000 ) ) ;
#6366=DIRECTION ( 'NONE',  ( 0.000000000000000000, 0.000000000000000000, 1.000000000000000000 ) ) ;
#6368=ORIENTED_EDGE ( 'NONE', *, *, #26539, .T. ) ;
#6369=FACE_OUTER_BOUND ( 'NONE', #23523, .T. ) ;
#6370=AXIS2_PLACEMENT_3D ( 'NONE', #20138, #26684, #34394 ) ;
#6371=CARTESIAN_POINT ( 'NONE',  ( -31.09745072740852123, -83.47442710120344600, -49.86348611802629449 ) ) ;
#6372=DIRECTION ( 'NONE',  ( 0.000000000000000000, 0.000000000000000000, 1.000000000000000000 ) ) ;
#6373=ORIENTED_EDGE ( 'NONE', *, *, #1387, .T. ) ;
#6374=CARTESIAN_POINT ( 'NONE',  ( 79.99999662536832545, -17.32050807568879591, 17.49999999999999645 ) ) ;
#6375=CYLINDRICAL_SURFACE ( 'NONE', #25599, 2.000000000000001776 ) ;
#6376=EDGE_LOOP ( 'NONE', ( #1541, #8143 ) ) ;
#6377=AXIS2_PLACEMENT_3D ( 'NONE', #2325, #5671, #30793 ) ;
#6378=ORIENTED_EDGE ( 'NONE', *, *, #15982, .T. ) ;
#6379=ADVANCED_FACE ( 'NONE', ( #17359 ), #3274, .F. ) ;
#6381=AXIS2_PLACEMENT_3D ( 'NONE', #12716, #6926, #27159 ) ;
#6382=CYLINDRICAL_SURFACE ( 'NONE', #4340, 2.000000000000001776 ) ;
#6383=DIRECTION ( 'NONE',  ( 0.5000000000000039968, 0.8660254037844363761, 0.000000000000000000 ) ) ;
#6386=ORIENTED_EDGE ( 'NONE', *, *, #11837, .F. ) ;
#6388=ADVANCED_FACE ( 'NONE', ( #9471 ), #3104, .F. ) ;
#6391=ORIENTED_EDGE ( 'NONE', *, *, #4969, .T. ) ;
#6392=EDGE_CURVE ( 'NONE', #35809, #14334, #23160, .T. ) ;
#6394=VERTEX_POINT ( 'NONE', #11701 ) ;
#6395=CARTESIAN_POINT ( 'NONE',  ( -57.00000337463107059, 43.30127018922197379, -9.999999999999998224 ) ) ;
#6397=VECTOR ( 'NONE', #31518, 1000.000000000000000 ) ;
#6398=DIRECTION ( 'NONE',  ( 1.000000000000000000, 0.000000000000000000, 0.000000000000000000 ) ) ;
#6399=CARTESIAN_POINT ( 'NONE',  ( 14.99999662536863632, -77.94228634059960825, -9.999999999999998224 ) ) ;
#6400=ORIENTED_EDGE ( 'NONE', *, *, #5529, .F. ) ;
#6402=CARTESIAN_POINT ( 'NONE',  ( 72.99999662536836809, 43.30127018922198801, -9.999999999999998224 ) ) ;
#6403=AXIS2_PLACEMENT_3D ( 'NONE', #15703, #1640, #13425 ) ;
#6404=CIRCLE ( 'NONE', #25587, 27.00000000000001421 ) ;
#6405=CARTESIAN_POINT ( 'NONE',  ( 79.99999662536832545, -34.64101615137759183, 17.49999999999999645 ) ) ;
#6406=CARTESIAN_POINT ( 'NONE',  ( 69.99999662536839651, 34.64101615137758472, -5.000000000000000000 ) ) ;
#6407=EDGE_CURVE ( 'NONE', #22954, #12040, #14530, .T. ) ;
#6408=AXIS2_PLACEMENT_3D ( 'NONE', #33263, #7582, #13018 ) ;
#6409=ORIENTED_EDGE ( 'NONE', *, *, #22546, .F. ) ;
#6410=DIRECTION ( 'NONE',  ( 1.000000000000000000, 0.000000000000000000, 0.000000000000000000 ) ) ;
#6411=FACE_BOUND ( 'NONE', #2528, .T. ) ;
#6415=DIRECTION ( 'NONE',  ( -0.000000000000000000, -0.000000000000000000, 1.000000000000000000 ) ) ;
#6417=ORIENTED_EDGE ( 'NONE', *, *, #14088, .F. ) ;
#6419=AXIS2_PLACEMENT_3D ( 'NONE', #10484, #16859, #8240 ) ;
#6420=AXIS2_PLACEMENT_3D ( 'NONE', #7572, #33071, #13206 ) ;
#6421=CARTESIAN_POINT ( 'NONE',  ( -83.10591231744739105, 8.018055418181152305, 12.50000000000000000 ) ) ;
#6424=DIRECTION ( 'NONE',  ( -0.000000000000000000, -0.000000000000000000, 1.000000000000000000 ) ) ;
#6425=DIRECTION ( 'NONE',  ( 0.000000000000000000, 0.000000000000000000, 1.000000000000000000 ) ) ;
#6428=EDGE_LOOP ( 'NONE', ( #32363, #25815, #6011, #31074, #29642 ) ) ;
#6433=DIRECTION ( 'NONE',  ( 0.000000000000000000, 0.000000000000000000, -1.000000000000000000 ) ) ;
#6434=DIRECTION ( 'NONE',  ( 0.000000000000000000, 0.000000000000000000, 1.000000000000000000 ) ) ;
#6436=DIRECTION ( 'NONE',  ( 0.000000000000000000, 0.000000000000000000, 1.000000000000000000 ) ) ;
#6437=ORIENTED_EDGE ( 'NONE', *, *, #13618, .T. ) ;
#6438=ORIENTED_EDGE ( 'NONE', *, *, #19640, .T. ) ;
#6440=ORIENTED_EDGE ( 'NONE', *, *, #32078, .T. ) ;
#6441=EDGE_CURVE ( 'NONE', #33332, #29281, #20506, .T. ) ;
#6443=AXIS2_PLACEMENT_3D ( 'NONE', #18983, #21418, #30209 ) ;
#6444=ORIENTED_EDGE ( 'NONE', *, *, #33031, .F. ) ;
#6446=ORIENTED_EDGE ( 'NONE', *, *, #7277, .T. ) ;
#6447=ADVANCED_FACE ( 'NONE', ( #28948 ), #9084, .T. ) ;
#6448=CARTESIAN_POINT ( 'NONE',  ( 1.999996625368672287, 86.60254037844397601, 12.50000000000000000 ) ) ;
#6449=ORIENTED_EDGE ( 'NONE', *, *, #31999, .T. ) ;
#6451=VERTEX_POINT ( 'NONE', #26347 ) ;
#6452=VECTOR ( 'NONE', #30086, 1000.000000000000000 ) ;
#6453=CIRCLE ( 'NONE', #1043, 2.000000000000001776 ) ;
#6455=LINE ( 'NONE', #4004, #22007 ) ;
#6456=DIRECTION ( 'NONE',  ( 0.000000000000000000, 0.000000000000000000, 1.000000000000000000 ) ) ;
#6457=EDGE_LOOP ( 'NONE', ( #22170, #34256 ) ) ;
#6458=VERTEX_POINT ( 'NONE', #23525 ) ;
#6459=DIRECTION ( 'NONE',  ( 0.000000000000000000, 0.000000000000000000, 1.000000000000000000 ) ) ;
#6462=CARTESIAN_POINT ( 'NONE',  ( 52.39915983220795681, 35.19434990244919703, -49.22241343995293761 ) ) ;
#6463=EDGE_CURVE ( 'NONE', #12329, #26842, #13039, .T. ) ;
#6464=DIRECTION ( 'NONE',  ( 1.000000000000000000, 0.000000000000000000, 0.000000000000000000 ) ) ;
#6465=EDGE_CURVE ( 'NONE', #33068, #3582, #28003, .T. ) ;
#6466=EDGE_LOOP ( 'NONE', ( #16468, #16631, #1260, #30822 ) ) ;
#6467=DIRECTION ( 'NONE',  ( 1.000000000000000000, 0.000000000000000000, 0.000000000000000000 ) ) ;
#6470=ADVANCED_FACE ( 'NONE', ( #15820 ), #26700, .F. ) ;
#6471=ORIENTED_EDGE ( 'NONE', *, *, #30727, .T. ) ;
#6473=AXIS2_PLACEMENT_3D ( 'NONE', #4837, #33877, #30517 ) ;
#6474=CIRCLE ( 'NONE', #7677, 3.000000000000007105 ) ;
#6475=FACE_OUTER_BOUND ( 'NONE', #27330, .T. ) ;
#6477=CARTESIAN_POINT ( 'NONE',  ( -4.279621169095561228, 62.97617850287782915, -4.999999999999997335 ) ) ;
#6478=CIRCLE ( 'NONE', #2270, 2.000000000000001776 ) ;
#6479=DIRECTION ( 'NONE',  ( 1.000000000000000000, 0.000000000000000000, 0.000000000000000000 ) ) ;
#6482=ORIENTED_EDGE ( 'NONE', *, *, #20485, .F. ) ;
#6483=DIRECTION ( 'NONE',  ( 0.000000000000000000, 0.000000000000000000, 1.000000000000000000 ) ) ;
#6484=CARTESIAN_POINT ( 'NONE',  ( 59.13646009116148150, -70.47608876694609137, 12.49999999999999822 ) ) ;
#6485=CARTESIAN_POINT ( 'NONE',  ( -90.00000337463090716, -1.040834085586084257E-14, -9.999999999999998224 ) ) ;
#6486=ORIENTED_EDGE ( 'NONE', *, *, #4264, .T. ) ;
#6487=VECTOR ( 'NONE', #16683, 1000.000000000000000 ) ;
#6492=CARTESIAN_POINT ( 'NONE',  ( 44.99999662536851019, -60.62177826491080168, -9.999999999999998224 ) ) ;
#6493=CARTESIAN_POINT ( 'NONE',  ( -80.00000337463094979, -2.428612866367529932E-14, -9.999999999999998224 ) ) ;
#6494=AXIS2_PLACEMENT_3D ( 'NONE', #17427, #17986, #34693 ) ;
#6495=DIRECTION ( 'NONE',  ( 0.000000000000000000, 0.000000000000000000, 1.000000000000000000 ) ) ;
#6496=EDGE_LOOP ( 'NONE', ( #28432, #29880 ) ) ;
#6497=DIRECTION ( 'NONE',  ( 0.000000000000000000, 0.000000000000000000, 1.000000000000000000 ) ) ;
#6498=EDGE_LOOP ( 'NONE', ( #10311, #30224 ) ) ;
#6499=VECTOR ( 'NONE', #26053, 1000.000000000000000 ) ;
#6500=FACE_BOUND ( 'NONE', #12889, .T. ) ;
#6502=AXIS2_PLACEMENT_3D ( 'NONE', #21925, #18378, #15571 ) ;
#6503=DIRECTION ( 'NONE',  ( 1.000000000000000000, 0.000000000000000000, 0.000000000000000000 ) ) ;
#6504=CARTESIAN_POINT ( 'NONE',  ( -87.00000337463093558, -8.660254037844422825, 17.49999999999999645 ) ) ;
#6505=ORIENTED_EDGE ( 'NONE', *, *, #10425, .T. ) ;
#6506=DIRECTION ( 'NONE',  ( 0.000000000000000000, 0.000000000000000000, 1.000000000000000000 ) ) ;
#6508=DIRECTION ( 'NONE',  ( 0.000000000000000000, 0.000000000000000000, 1.000000000000000000 ) ) ;
#6509=VECTOR ( 'NONE', #6264, 1000.000000000000000 ) ;
#6512=EDGE_CURVE ( 'NONE', #28925, #35441, #1668, .T. ) ;
#6516=CARTESIAN_POINT ( 'NONE',  ( -5.000003374631307729, 77.94228634059957983, 17.49999999999999645 ) ) ;
#6517=ORIENTED_EDGE ( 'NONE', *, *, #36910, .F. ) ;
#6518=ORIENTED_EDGE ( 'NONE', *, *, #27943, .F. ) ;
#6519=AXIS2_PLACEMENT_3D ( 'NONE', #14796, #31473, #23428 ) ;
#6520=VERTEX_POINT ( 'NONE', #21811 ) ;
#6521=AXIS2_PLACEMENT_3D ( 'NONE', #17201, #20537, #9294 ) ;
#6522=DIRECTION ( 'NONE',  ( 0.000000000000000000, 0.000000000000000000, 1.000000000000000000 ) ) ;
#6523=PLANE ( 'NONE',  #27287 ) ;
#6525=CIRCLE ( 'NONE', #2335, 2.000000000000001776 ) ;
#6526=CARTESIAN_POINT ( 'NONE',  ( -92.00000337463090716, -1.016341149603137227E-14, 12.50000000000000000 ) ) ;
#6529=VECTOR ( 'NONE', #24588, 1000.000000000000000 ) ;
#6530=DIRECTION ( 'NONE',  ( 0.000000000000000000, 0.000000000000000000, 1.000000000000000000 ) ) ;
#6531=EDGE_CURVE ( 'NONE', #12570, #13186, #32189, .T. ) ;
#6532=VERTEX_POINT ( 'NONE', #1569 ) ;
#6534=FACE_OUTER_BOUND ( 'NONE', #749, .T. ) ;
#6535=CIRCLE ( 'NONE', #5955, 2.000000000000001776 ) ;
#6536=DIRECTION ( 'NONE',  ( 1.000000000000000000, 0.000000000000000000, 0.000000000000000000 ) ) ;
#6537=ORIENTED_EDGE ( 'NONE', *, *, #27528, .F. ) ;
#6538=AXIS2_PLACEMENT_3D ( 'NONE', #23361, #20512, #3482 ) ;
#6539=FACE_OUTER_BOUND ( 'NONE', #20336, .T. ) ;
#6540=ORIENTED_EDGE ( 'NONE', *, *, #11667, .F. ) ;
#6541=ADVANCED_FACE ( 'NONE', ( #29504 ), #18829, .F. ) ;
#6543=FACE_BOUND ( 'NONE', #15314, .T. ) ;
#6544=CIRCLE ( 'NONE', #8350, 27.00000000000001421 ) ;
#6546=VERTEX_POINT ( 'NONE', #35905 ) ;
#6547=CIRCLE ( 'NONE', #8354, 27.00000000000001421 ) ;
#6548=FACE_OUTER_BOUND ( 'NONE', #7493, .T. ) ;
#6549=ORIENTED_EDGE ( 'NONE', *, *, #8641, .T. ) ;
#6551=DIRECTION ( 'NONE',  ( 0.000000000000000000, 0.000000000000000000, 1.000000000000000000 ) ) ;
#6553=AXIS2_PLACEMENT_3D ( 'NONE', #35733, #32526, #7411 ) ;
#6554=EDGE_CURVE ( 'NONE', #20492, #15386, #7668, .T. ) ;
#6555=ORIENTED_EDGE ( 'NONE', *, *, #17358, .T. ) ;
#6556=ORIENTED_EDGE ( 'NONE', *, *, #27, .F. ) ;
#6557=CIRCLE ( 'NONE', #14351, 3.499999999999991562 ) ;
#6559=ORIENTED_EDGE ( 'NONE', *, *, #23183, .T. ) ;
#6560=AXIS2_PLACEMENT_3D ( 'NONE', #26739, #23749, #11925 ) ;
#6561=VERTEX_POINT ( 'NONE', #27448 ) ;
#6562=CARTESIAN_POINT ( 'NONE',  ( 59.99999662536842493, -51.96152422706639840, 12.50000000000000000 ) ) ;
#6565=CARTESIAN_POINT ( 'NONE',  ( 64.99999662536842493, 43.30127018922200222, -9.999999999999998224 ) ) ;
#6566=DIRECTION ( 'NONE',  ( 1.000000000000000000, 0.000000000000000000, 0.000000000000000000 ) ) ;
#6567=CARTESIAN_POINT ( 'NONE',  ( 17.99999662536858835, 69.28203230275516944, -9.999999999999998224 ) ) ;
#6568=VERTEX_POINT ( 'NONE', #7215 ) ;
#6569=DIRECTION ( 'NONE',  ( 0.000000000000000000, 0.000000000000000000, 1.000000000000000000 ) ) ;
#6570=CARTESIAN_POINT ( 'NONE',  ( -78.00000337463094979, -17.32050807568882078, -5.000000000000000000 ) ) ;
#6571=CIRCLE ( 'NONE', #14336, 2.000000000000001776 ) ;
#6572=ADVANCED_FACE ( 'NONE', ( #4391 ), #18466, .F. ) ;
#6573=ORIENTED_EDGE ( 'NONE', *, *, #27053, .T. ) ;
#6574=DIRECTION ( 'NONE',  ( -1.047444401652940007E-14, -1.000000000000000000, 0.000000000000000000 ) ) ;
#6575=FACE_OUTER_BOUND ( 'NONE', #11995, .T. ) ;
#6577=ORIENTED_EDGE ( 'NONE', *, *, #24598, .T. ) ;
#6578=ORIENTED_EDGE ( 'NONE', *, *, #30808, .T. ) ;
#6579=DIRECTION ( 'NONE',  ( 1.000000000000000000, 0.000000000000000000, 0.000000000000000000 ) ) ;
#6580=DIRECTION ( 'NONE',  ( 1.000000000000000000, 0.000000000000000000, 0.000000000000000000 ) ) ;
#6581=CARTESIAN_POINT ( 'NONE',  ( 49.99999662536846756, 51.96152422706637708, 12.50000000000000000 ) ) ;
#6582=CARTESIAN_POINT ( 'NONE',  ( -52.39915983220772233, -35.19434990244957362, 12.49999999999999822 ) ) ;
#6584=EDGE_LOOP ( 'NONE', ( #17012, #4356 ) ) ;
#6589=ORIENTED_EDGE ( 'NONE', *, *, #36000, .F. ) ;
#6590=CIRCLE ( 'NONE', #23967, 2.000000000000001776 ) ;
#6591=CYLINDRICAL_SURFACE ( 'NONE', #15402, 2.000000000000001776 ) ;
#6593=ORIENTED_EDGE ( 'NONE', *, *, #1479, .T. ) ;
#6594=DIRECTION ( 'NONE',  ( 0.000000000000000000, 0.000000000000000000, 1.000000000000000000 ) ) ;
#6595=CARTESIAN_POINT ( 'NONE',  ( -61.25926521283079751, 32.16008401677975570, -49.22241343995295892 ) ) ;
#6596=CARTESIAN_POINT ( 'NONE',  ( -53.00000337463106348, 60.62177826491078747, -9.999999999999998224 ) ) ;
#6597=VERTEX_POINT ( 'NONE', #15264 ) ;
#6598=ORIENTED_EDGE ( 'NONE', *, *, #578, .T. ) ;
#6599=AXIS2_PLACEMENT_3D ( 'NONE', #18511, #32740, #15868 ) ;
#6600=DIRECTION ( 'NONE',  ( 0.000000000000000000, 0.000000000000000000, -1.000000000000000000 ) ) ;
#6601=CARTESIAN_POINT ( 'NONE',  ( -55.00000337463109901, -60.62177826491083010, 17.49999999999999645 ) ) ;
#6602=EDGE_CURVE ( 'NONE', #15126, #18489, #23358, .T. ) ;
#6603=VERTEX_POINT ( 'NONE', #15463 ) ;
#6604=DIRECTION ( 'NONE',  ( 1.000000000000000000, 0.000000000000000000, 0.000000000000000000 ) ) ;
#6605=DIRECTION ( 'NONE',  ( -1.000000000000000000, 0.000000000000000000, -0.000000000000000000 ) ) ;
#6610=EDGE_LOOP ( 'NONE', ( #5967, #31234 ) ) ;
#6611=CARTESIAN_POINT ( 'NONE',  ( -15.00000337463126066, 77.94228634059957983, -9.999999999999998224 ) ) ;
#6613=EDGE_CURVE ( 'NONE', #22407, #9038, #28723, .T. ) ;
#6614=CIRCLE ( 'NONE', #16210, 2.000000000000001776 ) ;
#6615=CARTESIAN_POINT ( 'NONE',  ( -65.00000337463104927, -43.30127018922202353, -9.999999999999998224 ) ) ;
#6616=ORIENTED_EDGE ( 'NONE', *, *, #8297, .F. ) ;
#6617=CARTESIAN_POINT ( 'NONE',  ( -57.00000337463107059, 60.62177826491078747, -5.000000000000000000 ) ) ;
#6619=CIRCLE ( 'NONE', #10799, 2.000000000000000000 ) ;
#6620=CARTESIAN_POINT ( 'NONE',  ( 4.279621169095998212, -62.97617850287780072, -4.999999999999997335 ) ) ;
#6621=ORIENTED_EDGE ( 'NONE', *, *, #11776, .T. ) ;
#6622=ORIENTED_EDGE ( 'NONE', *, *, #4961, .T. ) ;
#6623=DIRECTION ( 'NONE',  ( 0.000000000000000000, 0.000000000000000000, 1.000000000000000000 ) ) ;
#6624=DIRECTION ( 'NONE',  ( 0.000000000000000000, 0.000000000000000000, 1.000000000000000000 ) ) ;
#6625=CARTESIAN_POINT ( 'NONE',  ( -40.00000337463113453, -69.28203230275519786, 12.50000000000000000 ) ) ;
#6626=VERTEX_POINT ( 'NONE', #13559 ) ;
#6627=EDGE_LOOP ( 'NONE', ( #29741, #4091 ) ) ;
#6628=ORIENTED_EDGE ( 'NONE', *, *, #13188, .T. ) ;
#6630=ADVANCED_FACE ( 'NONE', ( #14108, #22557, #25561, #2120, #22010, #28354, #2503, #22368, #37004, #11311, #4942, #31188, #7769, #8326, #16211, #10929, #27628, #34014, #5129, #30794, #31000, #5332, #10764, #33812, #19758, #5501, #16929, #16568, #28000, #1939, #13365, #2327, #33638, #16378, #16765, #22760, #13757, #36454, #34202, #25373, #19212, #19021, #22201, #8124, #7941, #19567, #28185, #13927, #24824, #36260, #30449, #4775, #27801, #19375, #10570, #36805, #33455, #25208, #36635, #11109, #20300, #3066, #6054, #29283, #6411, #25760, #26102, #9212, #34918, #17479, #31722, #28546, #23478, #12188, #8859, #14311, #8496, #28899, #23301, #15039, #3227, #6219, #20643, #20107, #28738, #3611, #23658, #19924, #5673, #605, #32074, #17850, #26466, #8667, #11844, #775, #20465, #218, #31534, #12021, #14656, #31349, #17115, #2881, #54, #5875, #34750, #11480, #31886, #11648, #17312, #22927, #409, #9042, #14485, #34365, #25920, #23104, #14856, #34556, #17652, #29086, #3422, #26297, #6965, #12585, #21030, #21406, #1722, #32640, #18205, #24414, #4344, #23858, #15776, #32458, #27196, #32280, #4531, #32849, #13156, #35856, #6770, #10169, #27023, #21601 ), #29455, .T. ) ;
#6631=ORIENTED_EDGE ( 'NONE', *, *, #22729, .T. ) ;
#6633=ORIENTED_EDGE ( 'NONE', *, *, #1259, .F. ) ;
#6635=VERTEX_POINT ( 'NONE', #21205 ) ;
#6637=FACE_BOUND ( 'NONE', #17400, .T. ) ;
#6638=CARTESIAN_POINT ( 'NONE',  ( 47.63139720814400846, -27.50000000000022737, -10.00000000000000000 ) ) ;
#6639=CIRCLE ( 'NONE', #34201, 2.000000000000001776 ) ;
#6640=VERTEX_POINT ( 'NONE', #26849 ) ;
#6641=ORIENTED_EDGE ( 'NONE', *, *, #2245, .T. ) ;
#6642=DIRECTION ( 'NONE',  ( 1.000000000000000000, 0.000000000000000000, 0.000000000000000000 ) ) ;
#6643=CARTESIAN_POINT ( 'NONE',  ( -87.00000337463093558, 25.98076211353317433, -5.000000000000000000 ) ) ;
#6644=DIRECTION ( 'NONE',  ( 0.000000000000000000, 0.000000000000000000, -1.000000000000000000 ) ) ;
#6646=ADVANCED_FACE ( 'NONE', ( #18416 ), #15601, .F. ) ;
#6648=DIRECTION ( 'NONE',  ( 1.000000000000000000, 0.000000000000000000, 0.000000000000000000 ) ) ;
#6649=DIRECTION ( 'NONE',  ( 1.000000000000000000, 0.000000000000000000, 0.000000000000000000 ) ) ;
#6650=ORIENTED_EDGE ( 'NONE', *, *, #29801, .T. ) ;
#6654=DIRECTION ( 'NONE',  ( 1.000000000000000000, 0.000000000000000000, 0.000000000000000000 ) ) ;
#6656=EDGE_CURVE ( 'NONE', #17608, #29309, #25744, .T. ) ;
#6657=CARTESIAN_POINT ( 'NONE',  ( 24.99999662536857059, 77.94228634059957983, -5.000000000000000000 ) ) ;
#6658=CARTESIAN_POINT ( 'NONE',  ( -44.13139720814439215, -27.49999999999955591, -10.00000000000000178 ) ) ;
#6659=ORIENTED_EDGE ( 'NONE', *, *, #29871, .F. ) ;
#6663=DIRECTION ( 'NONE',  ( 1.000000000000000000, 0.000000000000000000, 0.000000000000000000 ) ) ;
#6664=EDGE_CURVE ( 'NONE', #23562, #22366, #19161, .T. ) ;
#6666=VERTEX_POINT ( 'NONE', #7342 ) ;
#6667=ORIENTED_EDGE ( 'NONE', *, *, #13683, .F. ) ;
#6668=CARTESIAN_POINT ( 'NONE',  ( -70.47608876694631874, -59.13646009116124702, -4.999999999999997335 ) ) ;
#6669=DIRECTION ( 'NONE',  ( 1.000000000000000000, 0.000000000000000000, 0.000000000000000000 ) ) ;
#6670=DIRECTION ( 'NONE',  ( -1.000000000000000000, 0.000000000000000000, 0.000000000000000000 ) ) ;
#6671=EDGE_CURVE ( 'NONE', #25751, #5018, #15412, .T. ) ;
#6673=CARTESIAN_POINT ( 'NONE',  ( 66.99999662536842493, 43.30127018922200222, -5.000000000000000000 ) ) ;
#6674=EDGE_CURVE ( 'NONE', #27152, #16822, #8397, .T. ) ;
#6677=EDGE_CURVE ( 'NONE', #29194, #17753, #33542, .T. ) ;
#6679=ORIENTED_EDGE ( 'NONE', *, *, #3650, .T. ) ;
#6680=FACE_BOUND ( 'NONE', #31484, .T. ) ;
#6682=VECTOR ( 'NONE', #34237, 1000.000000000000000 ) ;
#6683=LINE ( 'NONE', #21670, #5621 ) ;
#6684=ORIENTED_EDGE ( 'NONE', *, *, #21793, .T. ) ;
#6685=DIRECTION ( 'NONE',  ( 0.8660254037844415942, 0.4999999999999949485, 0.000000000000000000 ) ) ;
#6686=AXIS2_PLACEMENT_3D ( 'NONE', #33932, #20720, #34296 ) ;
#6687=DIRECTION ( 'NONE',  ( 3.491481338843133355E-15, 1.000000000000000000, 0.000000000000000000 ) ) ;
#6688=EDGE_CURVE ( 'NONE', #17057, #24286, #32935, .T. ) ;
#6689=CARTESIAN_POINT ( 'NONE',  ( -2.374207310413330682E-13, -68.00000000000000000, 12.49999999999999822 ) ) ;
#6690=CARTESIAN_POINT ( 'NONE',  ( -37.00000337463116296, 60.62177826491077326, 12.50000000000000000 ) ) ;
#6692=DIRECTION ( 'NONE',  ( 0.000000000000000000, 0.000000000000000000, 1.000000000000000000 ) ) ;
#6693=CARTESIAN_POINT ( 'NONE',  ( 64.99999662536839651, 60.62177826491078747, 17.49999999999999645 ) ) ;
#6694=CARTESIAN_POINT ( 'NONE',  ( -70.00000337463102085, -34.64101615137762025, -9.999999999999998224 ) ) ;
#6695=VERTEX_POINT ( 'NONE', #27402 ) ;
#6696=ORIENTED_EDGE ( 'NONE', *, *, #22776, .F. ) ;
#6697=ORIENTED_EDGE ( 'NONE', *, *, #28221, .T. ) ;
#6698=EDGE_CURVE ( 'NONE', #21989, #12964, #24570, .T. ) ;
#6699=CYLINDRICAL_SURFACE ( 'NONE', #17736, 2.000000000000001776 ) ;
#6700=DIRECTION ( 'NONE',  ( 1.000000000000000000, 0.000000000000000000, 0.000000000000000000 ) ) ;
#6701=LINE ( 'NONE', #29554, #9311 ) ;
#6702=CIRCLE ( 'NONE', #24701, 2.000000000000001776 ) ;
#6703=DIRECTION ( 'NONE',  ( 0.000000000000000000, 0.000000000000000000, 1.000000000000000000 ) ) ;
#6704=DIRECTION ( 'NONE',  ( -0.000000000000000000, -0.000000000000000000, 1.000000000000000000 ) ) ;
#6706=ORIENTED_EDGE ( 'NONE', *, *, #35454, .T. ) ;
#6707=EDGE_CURVE ( 'NONE', #15541, #30886, #8277, .T. ) ;
#6708=ORIENTED_EDGE ( 'NONE', *, *, #5491, .F. ) ;
#6711=DIRECTION ( 'NONE',  ( -0.8660254037844379305, 0.5000000000000011102, 0.000000000000000000 ) ) ;
#6713=EDGE_CURVE ( 'NONE', #3771, #31778, #590, .T. ) ;
#6714=DIRECTION ( 'NONE',  ( 1.000000000000000000, 0.000000000000000000, 0.000000000000000000 ) ) ;
#6716=FACE_BOUND ( 'NONE', #23174, .T. ) ;
#6717=ORIENTED_EDGE ( 'NONE', *, *, #30503, .F. ) ;
#6718=EDGE_LOOP ( 'NONE', ( #5484, #35460, #16708, #16605 ) ) ;
#6719=CARTESIAN_POINT ( 'NONE',  ( -68.00000337463102085, -34.64101615137762025, -9.999999999999998224 ) ) ;
#6720=ORIENTED_EDGE ( 'NONE', *, *, #16086, .T. ) ;
#6721=DIRECTION ( 'NONE',  ( 0.000000000000000000, 0.000000000000000000, 1.000000000000000000 ) ) ;
#6722=AXIS2_PLACEMENT_3D ( 'NONE', #34159, #28857, #8455 ) ;
#6723=CARTESIAN_POINT ( 'NONE',  ( 52.39915983220795681, 35.19434990244919703, -4.999999999999997335 ) ) ;
#6724=DIRECTION ( 'NONE',  ( 0.000000000000000000, 0.000000000000000000, -1.000000000000000000 ) ) ;
#6725=EDGE_LOOP ( 'NONE', ( #17371, #2574, #6916, #34177 ) ) ;
#6726=ORIENTED_EDGE ( 'NONE', *, *, #12081, .F. ) ;
#6727=EDGE_LOOP ( 'NONE', ( #33995, #36190 ) ) ;
#6730=ORIENTED_EDGE ( 'NONE', *, *, #18137, .T. ) ;
#6731=CARTESIAN_POINT ( 'NONE',  ( -25.30168483247182820, 79.91940249752995840, 12.50000000000000000 ) ) ;
#6733=VERTEX_POINT ( 'NONE', #30588 ) ;
#6734=CARTESIAN_POINT ( 'NONE',  ( -62.97617850287781494, -4.279621169095772615, 12.49999999999999822 ) ) ;
#6737=ORIENTED_EDGE ( 'NONE', *, *, #13435, .T. ) ;
#6738=CYLINDRICAL_SURFACE ( 'NONE', #7486, 3.000000000000002665 ) ;
#6741=CARTESIAN_POINT ( 'NONE',  ( -30.00000337463118427, 69.28203230275516944, 12.50000000000000000 ) ) ;
#6742=ORIENTED_EDGE ( 'NONE', *, *, #19830, .T. ) ;
#6743=DIRECTION ( 'NONE',  ( 1.000000000000000000, 0.000000000000000000, 0.000000000000000000 ) ) ;
#6744=CARTESIAN_POINT ( 'NONE',  ( -78.00000337463094979, 17.32050807568878525, 12.50000000000000000 ) ) ;
#6745=EDGE_LOOP ( 'NONE', ( #1671, #26277, #16426, #9957 ) ) ;
#6746=VERTEX_POINT ( 'NONE', #33200 ) ;
#6748=AXIS2_PLACEMENT_3D ( 'NONE', #19303, #4308, #7304 ) ;
#6749=DIRECTION ( 'NONE',  ( 0.000000000000000000, 0.000000000000000000, 1.000000000000000000 ) ) ;
#6750=EDGE_CURVE ( 'NONE', #29589, #12416, #8971, .T. ) ;
#6751=DIRECTION ( 'NONE',  ( 0.000000000000000000, 0.000000000000000000, 1.000000000000000000 ) ) ;
#6754=EDGE_LOOP ( 'NONE', ( #12308, #24533, #20269, #8106 ) ) ;
#6756=CYLINDRICAL_SURFACE ( 'NONE', #17131, 2.000000000000001776 ) ;
#6757=ORIENTED_EDGE ( 'NONE', *, *, #20735, .F. ) ;
#6758=PLANE ( 'NONE',  #35777 ) ;
#6759=EDGE_LOOP ( 'NONE', ( #6245, #28296 ) ) ;
#6760=CARTESIAN_POINT ( 'NONE',  ( 17.99999662536861678, -86.60254037844400443, -5.000000000000000000 ) ) ;
#6761=AXIS2_PLACEMENT_3D ( 'NONE', #28875, #17453, #3197 ) ;
#6763=CARTESIAN_POINT ( 'NONE',  ( 7.999996625368656744, -69.28203230275519786, -5.000000000000000000 ) ) ;
#6764=VERTEX_POINT ( 'NONE', #16166 ) ;
#6765=ORIENTED_EDGE ( 'NONE', *, *, #2045, .F. ) ;
#6766=ADVANCED_FACE ( 'NONE', ( #31142 ), #8079, .F. ) ;
#6767=CARTESIAN_POINT ( 'NONE',  ( -62.00000337463107769, -34.64101615137762025, 17.49999999999999645 ) ) ;
#6768=ORIENTED_EDGE ( 'NONE', *, *, #6392, .F. ) ;
#6769=DIRECTION ( 'NONE',  ( -0.8660254037844381525, 0.5000000000000009992, 0.000000000000000000 ) ) ;
#6770=FACE_BOUND ( 'NONE', #16614, .T. ) ;
#6771=ADVANCED_FACE ( 'NONE', ( #10518 ), #16888, .F. ) ;
#6772=CARTESIAN_POINT ( 'NONE',  ( 44.99999662536849598, 60.62177826491077326, -9.999999999999998224 ) ) ;
#6775=VERTEX_POINT ( 'NONE', #33597 ) ;
#6776=CARTESIAN_POINT ( 'NONE',  ( -78.00000337463094979, -17.32050807568882078, -9.999999999999998224 ) ) ;
#6777=CARTESIAN_POINT ( 'NONE',  ( -40.00000337463113453, -69.28203230275519786, -9.999999999999998224 ) ) ;
#6778=EDGE_CURVE ( 'NONE', #36669, #16909, #5403, .T. ) ;
#6779=EDGE_LOOP ( 'NONE', ( #5499, #23508 ) ) ;
#6781=CARTESIAN_POINT ( 'NONE',  ( -4.279621169095561228, 62.97617850287782915, -4.999999999999997335 ) ) ;
#6782=CARTESIAN_POINT ( 'NONE',  ( -44.13139720814381661, 27.50000000000055422, -10.00000000000000178 ) ) ;
#6783=AXIS2_PLACEMENT_3D ( 'NONE', #20130, #5696, #14674 ) ;
#6784=DIRECTION ( 'NONE',  ( 0.000000000000000000, 0.000000000000000000, 1.000000000000000000 ) ) ;
#6785=ORIENTED_EDGE ( 'NONE', *, *, #29637, .F. ) ;
#6786=CIRCLE ( 'NONE', #16384, 2.000000000000001776 ) ;
#6787=ORIENTED_EDGE ( 'NONE', *, *, #15522, .T. ) ;
#6789=EDGE_CURVE ( 'NONE', #34315, #25502, #5284, .T. ) ;
#6790=CARTESIAN_POINT ( 'NONE',  ( 79.99999662536832545, -17.32050807568879591, -9.999999999999998224 ) ) ;
#6791=DIRECTION ( 'NONE',  ( 0.000000000000000000, 0.000000000000000000, 1.000000000000000000 ) ) ;
#6792=ORIENTED_EDGE ( 'NONE', *, *, #16782, .F. ) ;
#6793=VERTEX_POINT ( 'NONE', #24610 ) ;
#6796=CARTESIAN_POINT ( 'NONE',  ( -27.78182860042817026, -56.67878100130359087, -4.999999999999997335 ) ) ;
#6797=AXIS2_PLACEMENT_3D ( 'NONE', #5137, #19031, #16219 ) ;
#6798=ORIENTED_EDGE ( 'NONE', *, *, #22160, .F. ) ;
#6799=VERTEX_POINT ( 'NONE', #4906 ) ;
#6800=CYLINDRICAL_SURFACE ( 'NONE', #2234, 2.000000000000000000 ) ;
#6801=VERTEX_POINT ( 'NONE', #2462 ) ;
#6802=AXIS2_PLACEMENT_3D ( 'NONE', #6485, #24269, #664 ) ;
#6803=ORIENTED_EDGE ( 'NONE', *, *, #33121, .F. ) ;
#6804=ADVANCED_FACE ( 'NONE', ( #36040 ), #10332, .F. ) ;
#6805=DIRECTION ( 'NONE',  ( -0.000000000000000000, -0.000000000000000000, 1.000000000000000000 ) ) ;
#6806=ADVANCED_FACE ( 'NONE', ( #30398 ), #1902, .T. ) ;
#6807=FACE_OUTER_BOUND ( 'NONE', #29528, .T. ) ;
#6808=ORIENTED_EDGE ( 'NONE', *, *, #27193, .F. ) ;
#6810=CARTESIAN_POINT ( 'NONE',  ( 66.99999662536839651, -60.62177826491080168, -9.999999999999998224 ) ) ;
#6811=DIRECTION ( 'NONE',  ( 1.000000000000000000, 0.000000000000000000, 0.000000000000000000 ) ) ;
#6814=CARTESIAN_POINT ( 'NONE',  ( 12.99999662536863632, -77.94228634059960825, 12.50000000000000000 ) ) ;
#6816=ORIENTED_EDGE ( 'NONE', *, *, #35793, .T. ) ;
#6817=DIRECTION ( 'NONE',  ( 0.000000000000000000, 0.000000000000000000, 1.000000000000000000 ) ) ;
#6818=DIRECTION ( 'NONE',  ( 0.000000000000000000, 0.000000000000000000, 1.000000000000000000 ) ) ;
#6820=CARTESIAN_POINT ( 'NONE',  ( -60.00000337463107059, -34.64101615137762025, -9.999999999999998224 ) ) ;
#6821=EDGE_CURVE ( 'NONE', #12416, #22484, #25166, .T. ) ;
#6822=DIRECTION ( 'NONE',  ( 0.000000000000000000, 0.000000000000000000, 1.000000000000000000 ) ) ;
#6824=CARTESIAN_POINT ( 'NONE',  ( 39.99999662536853151, 69.28203230275518365, 17.49999999999999645 ) ) ;
#6825=CIRCLE ( 'NONE', #21817, 2.000000000000001776 ) ;
#6826=DIRECTION ( 'NONE',  ( 0.000000000000000000, 0.000000000000000000, 1.000000000000000000 ) ) ;
#6827=EDGE_CURVE ( 'NONE', #5822, #1919, #2989, .T. ) ;
#6829=CARTESIAN_POINT ( 'NONE',  ( 74.99999662536836809, 43.30127018922198801, 17.49999999999999645 ) ) ;
#6830=ORIENTED_EDGE ( 'NONE', *, *, #34904, .T. ) ;
#6831=CARTESIAN_POINT ( 'NONE',  ( -95.00000000000000000, 0.000000000000000000, 17.49999999999999645 ) ) ;
#6832=DIRECTION ( 'NONE',  ( 1.000000000000000000, 0.000000000000000000, 0.000000000000000000 ) ) ;
#6833=CARTESIAN_POINT ( 'NONE',  ( 77.99999662536833966, 17.32050807568879236, -9.999999999999998224 ) ) ;
#6834=ORIENTED_EDGE ( 'NONE', *, *, #28434, .T. ) ;
#6836=VERTEX_POINT ( 'NONE', #2275 ) ;
#6838=DIRECTION ( 'NONE',  ( 0.000000000000000000, 0.000000000000000000, 1.000000000000000000 ) ) ;
#6840=CARTESIAN_POINT ( 'NONE',  ( -33.00000337463116296, 60.62177826491077326, -9.999999999999998224 ) ) ;
#6843=EDGE_CURVE ( 'NONE', #4052, #27516, #33770, .T. ) ;
#6844=DIRECTION ( 'NONE',  ( 1.000000000000000000, 0.000000000000000000, 0.000000000000000000 ) ) ;
#6845=ORIENTED_EDGE ( 'NONE', *, *, #6854, .F. ) ;
#6847=ORIENTED_EDGE ( 'NONE', *, *, #33150, .F. ) ;
#6848=FACE_BOUND ( 'NONE', #997, .T. ) ;
#6849=EDGE_CURVE ( 'NONE', #691, #25535, #19775, .T. ) ;
#6850=AXIS2_PLACEMENT_3D ( 'NONE', #21539, #30140, #32972 ) ;
#6852=CYLINDRICAL_SURFACE ( 'NONE', #1774, 2.000000000000001776 ) ;
#6853=AXIS2_PLACEMENT_3D ( 'NONE', #1866, #24743, #30559 ) ;
#6854=EDGE_CURVE ( 'NONE', #6733, #2698, #32335, .T. ) ;
#6855=CARTESIAN_POINT ( 'NONE',  ( 41.99999662536853151, -69.28203230275519786, -9.999999999999998224 ) ) ;
#6856=EDGE_CURVE ( 'NONE', #31054, #29609, #32308, .T. ) ;
#6857=EDGE_LOOP ( 'NONE', ( #21201, #21810 ) ) ;
#6858=DIRECTION ( 'NONE',  ( 0.000000000000000000, 0.000000000000000000, 1.000000000000000000 ) ) ;
#6862=CIRCLE ( 'NONE', #24866, 2.000000000000001776 ) ;
#6863=DIRECTION ( 'NONE',  ( 3.491481338843135327E-15, 1.000000000000000000, 0.000000000000000000 ) ) ;
#6865=ORIENTED_EDGE ( 'NONE', *, *, #29588, .T. ) ;
#6866=CYLINDRICAL_SURFACE ( 'NONE', #25027, 2.000000000000001776 ) ;
#6867=VECTOR ( 'NONE', #28691, 1000.000000000000000 ) ;
#6868=DIRECTION ( 'NONE',  ( 1.000000000000000000, 0.000000000000000000, 0.000000000000000000 ) ) ;
#6869=CARTESIAN_POINT ( 'NONE',  ( -70.00000337463102085, -51.96152422706641971, 12.50000000000000000 ) ) ;
#6870=ORIENTED_EDGE ( 'NONE', *, *, #21361, .F. ) ;
#6871=AXIS2_PLACEMENT_3D ( 'NONE', #26072, #8829, #6030 ) ;
#6875=CARTESIAN_POINT ( 'NONE',  ( 42.99999662536850309, 77.94228634059959404, -5.000000000000000000 ) ) ;
#6876=CARTESIAN_POINT ( 'NONE',  ( 34.99999662536855283, -77.94228634059960825, -9.999999999999998224 ) ) ;
#6877=CIRCLE ( 'NONE', #12260, 2.000000000000001776 ) ;
#6878=AXIS2_PLACEMENT_3D ( 'NONE', #16199, #19201, #30436 ) ;
#6879=AXIS2_PLACEMENT_3D ( 'NONE', #34630, #16827, #19634 ) ;
#6880=DIRECTION ( 'NONE',  ( -0.000000000000000000, -0.000000000000000000, 1.000000000000000000 ) ) ;
#6881=DIRECTION ( 'NONE',  ( 0.000000000000000000, 0.000000000000000000, -1.000000000000000000 ) ) ;
#6882=DIRECTION ( 'NONE',  ( 1.000000000000000000, 0.000000000000000000, 0.000000000000000000 ) ) ;
#6883=DIRECTION ( 'NONE',  ( 0.000000000000000000, 0.000000000000000000, -1.000000000000000000 ) ) ;
#6884=ORIENTED_EDGE ( 'NONE', *, *, #9666, .F. ) ;
#6886=CARTESIAN_POINT ( 'NONE',  ( 26.99999662536859546, -77.94228634059960825, -9.999999999999998224 ) ) ;
#6887=EDGE_CURVE ( 'NONE', #19642, #30141, #24596, .T. ) ;
#6888=AXIS2_PLACEMENT_3D ( 'NONE', #8531, #22798, #22402 ) ;
#6889=CARTESIAN_POINT ( 'NONE',  ( 0.000000000000000000, 0.000000000000000000, -5.000000000000000000 ) ) ;
#6890=VERTEX_POINT ( 'NONE', #7 ) ;
#6892=AXIS2_PLACEMENT_3D ( 'NONE', #20911, #12450, #18084 ) ;
#6893=FACE_OUTER_BOUND ( 'NONE', #14873, .T. ) ;
#6894=VERTEX_POINT ( 'NONE', #32020 ) ;
#6895=DIRECTION ( 'NONE',  ( 0.000000000000000000, 0.000000000000000000, 1.000000000000000000 ) ) ;
#6896=VECTOR ( 'NONE', #28799, 1000.000000000000000 ) ;
#6897=ADVANCED_FACE ( 'NONE', ( #22884 ), #6175, .F. ) ;
#6898=CARTESIAN_POINT ( 'NONE',  ( -35.00000337463116296, 77.94228634059957983, 17.49999999999999645 ) ) ;
#6899=ORIENTED_EDGE ( 'NONE', *, *, #31314, .F. ) ;
#6900=ORIENTED_EDGE ( 'NONE', *, *, #9596, .F. ) ;
#6901=EDGE_CURVE ( 'NONE', #15350, #35412, #8995, .T. ) ;
#6904=CIRCLE ( 'NONE', #29048, 3.000000000000001332 ) ;
#6905=ADVANCED_FACE ( 'NONE', ( #11262 ), #3018, .T. ) ;
#6906=AXIS2_PLACEMENT_3D ( 'NONE', #13403, #25065, #5171 ) ;
#6908=CARTESIAN_POINT ( 'NONE',  ( -80.00000337463094979, -17.32050807568882078, -9.999999999999998224 ) ) ;
#6909=DIRECTION ( 'NONE',  ( 0.000000000000000000, 0.000000000000000000, 1.000000000000000000 ) ) ;
#6910=ORIENTED_EDGE ( 'NONE', *, *, #30612, .F. ) ;
#6911=VERTEX_POINT ( 'NONE', #5626 ) ;
#6912=EDGE_CURVE ( 'NONE', #33445, #18148, #26956, .T. ) ;
#6913=ORIENTED_EDGE ( 'NONE', *, *, #18323, .F. ) ;
#6914=EDGE_CURVE ( 'NONE', #9484, #32397, #16213, .T. ) ;
#6915=ORIENTED_EDGE ( 'NONE', *, *, #28174, .T. ) ;
#6916=ORIENTED_EDGE ( 'NONE', *, *, #28616, .T. ) ;
#6917=EDGE_CURVE ( 'NONE', #12472, #14042, #6619, .T. ) ;
#6918=DIRECTION ( 'NONE',  ( 0.000000000000000000, 0.000000000000000000, -1.000000000000000000 ) ) ;
#6919=ADVANCED_FACE ( 'NONE', ( #9004 ), #29985, .F. ) ;
#6921=ORIENTED_EDGE ( 'NONE', *, *, #9396, .F. ) ;
#6922=CIRCLE ( 'NONE', #6300, 2.000000000000001776 ) ;
#6926=DIRECTION ( 'NONE',  ( 0.000000000000000000, 0.000000000000000000, 1.000000000000000000 ) ) ;
#6927=AXIS2_PLACEMENT_3D ( 'NONE', #1360, #3635, #35139 ) ;
#6930=DIRECTION ( 'NONE',  ( 1.000000000000000000, 0.000000000000000000, 0.000000000000000000 ) ) ;
#6931=CIRCLE ( 'NONE', #36858, 33.00000000000001421 ) ;
#6932=FACE_OUTER_BOUND ( 'NONE', #34477, .T. ) ;
#6934=ORIENTED_EDGE ( 'NONE', *, *, #683, .T. ) ;
#6936=DIRECTION ( 'NONE',  ( 0.000000000000000000, 0.000000000000000000, 1.000000000000000000 ) ) ;
#6937=ORIENTED_EDGE ( 'NONE', *, *, #5724, .T. ) ;
#6939=DIRECTION ( 'NONE',  ( -1.000000000000000000, 0.000000000000000000, 0.000000000000000000 ) ) ;
#6940=LINE ( 'NONE', #18387, #7954 ) ;
#6942=DIRECTION ( 'NONE',  ( 0.000000000000000000, 0.000000000000000000, 1.000000000000000000 ) ) ;
#6943=ORIENTED_EDGE ( 'NONE', *, *, #33031, .T. ) ;
#6944=AXIS2_PLACEMENT_3D ( 'NONE', #23706, #14527, #26152 ) ;
#6945=CARTESIAN_POINT ( 'NONE',  ( -56.67878100130369035, 27.78182860042797131, -4.999999999999997335 ) ) ;
#6947=AXIS2_PLACEMENT_3D ( 'NONE', #29893, #27453, #30248 ) ;
#6948=VERTEX_POINT ( 'NONE', #23810 ) ;
#6949=AXIS2_PLACEMENT_3D ( 'NONE', #18784, #36045, #13330 ) ;
#6951=VERTEX_POINT ( 'NONE', #35817 ) ;
#6952=CIRCLE ( 'NONE', #5783, 2.000000000000001776 ) ;
#6954=DIRECTION ( 'NONE',  ( 0.000000000000000000, 0.000000000000000000, 1.000000000000000000 ) ) ;
#6955=VECTOR ( 'NONE', #8506, 1000.000000000000000 ) ;
#6958=DIRECTION ( 'NONE',  ( 0.000000000000000000, 0.000000000000000000, 1.000000000000000000 ) ) ;
#6962=EDGE_LOOP ( 'NONE', ( #15021, #18285 ) ) ;
#6963=DIRECTION ( 'NONE',  ( 0.000000000000000000, 0.000000000000000000, 1.000000000000000000 ) ) ;
#6964=EDGE_CURVE ( 'NONE', #36953, #8381, #1296, .T. ) ;
#6965=FACE_BOUND ( 'NONE', #4545, .T. ) ;
#6966=DIRECTION ( 'NONE',  ( 0.000000000000000000, 0.000000000000000000, 1.000000000000000000 ) ) ;
#6968=DIRECTION ( 'NONE',  ( 0.000000000000000000, 0.000000000000000000, 1.000000000000000000 ) ) ;
#6969=ORIENTED_EDGE ( 'NONE', *, *, #24907, .F. ) ;
#6970=DIRECTION ( 'NONE',  ( 0.000000000000000000, 0.000000000000000000, 1.000000000000000000 ) ) ;
#6971=VECTOR ( 'NONE', #3226, 1000.000000000000000 ) ;
#6972=DIRECTION ( 'NONE',  ( 0.000000000000000000, 0.000000000000000000, 1.000000000000000000 ) ) ;
#6973=VECTOR ( 'NONE', #176, 1000.000000000000000 ) ;
#6975=EDGE_LOOP ( 'NONE', ( #7279, #35921, #29209, #11623 ) ) ;
#6976=CARTESIAN_POINT ( 'NONE',  ( 84.99999662536831124, -25.98076211353319565, -5.000000000000000000 ) ) ;
#6977=PRODUCT_DEFINITION_FORMATION_WITH_SPECIFIED_SOURCE ( 'ANY', '', #8866, .NOT_KNOWN. ) ;
#6979=CYLINDRICAL_SURFACE ( 'NONE', #1821, 2.000000000000001776 ) ;
#6980=AXIS2_PLACEMENT_3D ( 'NONE', #36073, #36628, #13919 ) ;
#6981=CIRCLE ( 'NONE', #10602, 2.000000000000001776 ) ;
#6984=ORIENTED_EDGE ( 'NONE', *, *, #6856, .T. ) ;
#6985=CIRCLE ( 'NONE', #32730, 2.000000000000001776 ) ;
#6987=DIRECTION ( 'NONE',  ( 0.000000000000000000, 0.000000000000000000, 1.000000000000000000 ) ) ;
#6989=VERTEX_POINT ( 'NONE', #29790 ) ;
#6990=ORIENTED_EDGE ( 'NONE', *, *, #15723, .T. ) ;
#6991=ORIENTED_EDGE ( 'NONE', *, *, #14088, .T. ) ;
#6994=CIRCLE ( 'NONE', #18373, 33.00000000000001421 ) ;
#6996=ORIENTED_EDGE ( 'NONE', *, *, #14817, .T. ) ;
#6998=ORIENTED_EDGE ( 'NONE', *, *, #29801, .F. ) ;
#6999=CARTESIAN_POINT ( 'NONE',  ( 9.999996625368655856, -86.60254037844400443, -9.999999999999998224 ) ) ;
#7002=ORIENTED_EDGE ( 'NONE', *, *, #4082, .T. ) ;
#7004=FACE_OUTER_BOUND ( 'NONE', #27680, .T. ) ;
#7005=AXIS2_PLACEMENT_3D ( 'NONE', #25879, #23256, #9007 ) ;
#7006=CIRCLE ( 'NONE', #23177, 2.000000000000001776 ) ;
#7007=DIRECTION ( 'NONE',  ( 1.000000000000000000, 0.000000000000000000, 0.000000000000000000 ) ) ;
#7009=EDGE_LOOP ( 'NONE', ( #30750, #33999, #22185, #6072 ) ) ;
#7010=DIRECTION ( 'NONE',  ( -0.000000000000000000, -0.000000000000000000, 1.000000000000000000 ) ) ;
#7011=FACE_OUTER_BOUND ( 'NONE', #8488, .T. ) ;
#7012=LINE ( 'NONE', #18459, #35741 ) ;
#7013=VECTOR ( 'NONE', #6936, 1000.000000000000000 ) ;
#7017=AXIS2_PLACEMENT_3D ( 'NONE', #4224, #24259, #35371 ) ;
#7018=ORIENTED_EDGE ( 'NONE', *, *, #6613, .T. ) ;
#7019=DIRECTION ( 'NONE',  ( 1.000000000000000000, 0.000000000000000000, 0.000000000000000000 ) ) ;
#7020=ORIENTED_EDGE ( 'NONE', *, *, #3387, .T. ) ;
#7021=ADVANCED_FACE ( 'NONE', ( #7300 ), #4125, .F. ) ;
#7023=CARTESIAN_POINT ( 'NONE',  ( -20.00000337463123756, -69.28203230275522628, 17.49999999999999645 ) ) ;
#7024=CARTESIAN_POINT ( 'NONE',  ( -77.00000337463100664, -43.30127018922202353, -5.000000000000000000 ) ) ;
#7025=VECTOR ( 'NONE', #20386, 1000.000000000000000 ) ;
#7026=CARTESIAN_POINT ( 'NONE',  ( 74.99999662536835388, -43.30127018922199511, -9.999999999999998224 ) ) ;
#7027=DIRECTION ( 'NONE',  ( 0.000000000000000000, 0.000000000000000000, 1.000000000000000000 ) ) ;
#7028=CYLINDRICAL_SURFACE ( 'NONE', #26531, 2.000000000000000000 ) ;
#7029=VERTEX_POINT ( 'NONE', #35265 ) ;
#7030=CARTESIAN_POINT ( 'NONE',  ( -37.00000337463116296, 77.94228634059957983, -5.000000000000000000 ) ) ;
#7031=CIRCLE ( 'NONE', #27981, 1.999999999999998224 ) ;
#7032=DIRECTION ( 'NONE',  ( -1.000000000000000000, 0.000000000000000000, 0.000000000000000000 ) ) ;
#7033=DIRECTION ( 'NONE',  ( 0.000000000000000000, 0.000000000000000000, 1.000000000000000000 ) ) ;
#7034=CIRCLE ( 'NONE', #15439, 2.000000000000001776 ) ;
#7036=VERTEX_POINT ( 'NONE', #12146 ) ;
#7037=VERTEX_POINT ( 'NONE', #32597 ) ;
#7038=AXIS2_PLACEMENT_3D ( 'NONE', #9829, #24092, #4231 ) ;
#7039=EDGE_CURVE ( 'NONE', #29631, #3733, #3011, .T. ) ;
#7040=DIRECTION ( 'NONE',  ( 1.000000000000000000, 0.000000000000000000, 0.000000000000000000 ) ) ;
#7041=PLANE ( 'NONE',  #15816 ) ;
#7043=ORIENTED_EDGE ( 'NONE', *, *, #23640, .F. ) ;
#7045=AXIS2_PLACEMENT_3D ( 'NONE', #8425, #19853, #8590 ) ;
#7046=CIRCLE ( 'NONE', #19628, 2.000000000000001776 ) ;
#7047=DIRECTION ( 'NONE',  ( -0.000000000000000000, -0.000000000000000000, 1.000000000000000000 ) ) ;
#7048=DIRECTION ( 'NONE',  ( 1.000000000000000000, 0.000000000000000000, 0.000000000000000000 ) ) ;
#7049=ORIENTED_EDGE ( 'NONE', *, *, #21889, .F. ) ;
#7050=LINE ( 'NONE', #18496, #22765 ) ;
#7051=ADVANCED_FACE ( 'NONE', ( #18738 ), #12342, .T. ) ;
#7052=ORIENTED_EDGE ( 'NONE', *, *, #1553, .F. ) ;
#7053=FACE_BOUND ( 'NONE', #19723, .T. ) ;
#7055=EDGE_CURVE ( 'NONE', #6532, #24891, #5426, .T. ) ;
#7056=CARTESIAN_POINT ( 'NONE',  ( 79.99999662536833966, 34.64101615137759183, -9.999999999999998224 ) ) ;
#7057=DIRECTION ( 'NONE',  ( 1.000000000000000000, 0.000000000000000000, 0.000000000000000000 ) ) ;
#7058=AXIS2_PLACEMENT_3D ( 'NONE', #1537, #18437, #26485 ) ;
#7060=ORIENTED_EDGE ( 'NONE', *, *, #34814, .T. ) ;
#7062=AXIS2_PLACEMENT_3D ( 'NONE', #23969, #4274, #35417 ) ;
#7063=CIRCLE ( 'NONE', #28015, 2.000000000000001776 ) ;
#7064=AXIS2_PLACEMENT_3D ( 'NONE', #20387, #9123, #17751 ) ;
#7065=DIRECTION ( 'NONE',  ( 1.000000000000000000, 0.000000000000000000, 0.000000000000000000 ) ) ;
#7066=CIRCLE ( 'NONE', #8247, 2.000000000000001776 ) ;
#7068=DIRECTION ( 'NONE',  ( 0.8660254037844413721, 0.4999999999999950595, 0.000000000000000000 ) ) ;
#7069=VERTEX_POINT ( 'NONE', #32800 ) ;
#7070=DIRECTION ( 'NONE',  ( 0.000000000000000000, 0.000000000000000000, 1.000000000000000000 ) ) ;
#7072=DIRECTION ( 'NONE',  ( -1.000000000000000000, 0.000000000000000000, 0.000000000000000000 ) ) ;
#7073=AXIS2_PLACEMENT_3D ( 'NONE', #7929, #16557, #8111 ) ;
#7074=EDGE_CURVE ( 'NONE', #14854, #18637, #16188, .T. ) ;
#7075=EDGE_LOOP ( 'NONE', ( #11140, #9843, #14511, #36433 ) ) ;
#7076=ORIENTED_EDGE ( 'NONE', *, *, #11586, .T. ) ;
#7077=DIRECTION ( 'NONE',  ( 1.000000000000000000, 0.000000000000000000, 0.000000000000000000 ) ) ;
#7078=DIRECTION ( 'NONE',  ( -0.8660254037844449249, -0.4999999999999888423, 0.000000000000000000 ) ) ;
#7079=ADVANCED_FACE ( 'NONE', ( #20797 ), #32233, .F. ) ;
#7080=CARTESIAN_POINT ( 'NONE',  ( -75.00000337463097821, 43.30127018922197379, -5.000000000000000000 ) ) ;
#7081=EDGE_LOOP ( 'NONE', ( #36238, #3760 ) ) ;
#7082=AXIS2_PLACEMENT_3D ( 'NONE', #13915, #45, #22357 ) ;
#7083=EDGE_CURVE ( 'NONE', #12432, #21828, #31166, .T. ) ;
#7084=DIRECTION ( 'NONE',  ( 0.5000000000000039968, 0.8660254037844363761, 0.000000000000000000 ) ) ;
#7085=CARTESIAN_POINT ( 'NONE',  ( 44.99999662536849598, 60.62177826491077326, -9.999999999999998224 ) ) ;
#7086=AXIS2_PLACEMENT_3D ( 'NONE', #29709, #21479, #35730 ) ;
#7087=DIRECTION ( 'NONE',  ( 0.000000000000000000, 0.000000000000000000, 1.000000000000000000 ) ) ;
#7088=EDGE_LOOP ( 'NONE', ( #2847, #15188 ) ) ;
#7090=ORIENTED_EDGE ( 'NONE', *, *, #26571, .F. ) ;
#7091=DIRECTION ( 'NONE',  ( 1.000000000000000000, 0.000000000000000000, 0.000000000000000000 ) ) ;
#7092=CIRCLE ( 'NONE', #25652, 2.000000000000001776 ) ;
#7093=CARTESIAN_POINT ( 'NONE',  ( 35.19434990244975126, -52.39915983220758022, 12.49999999999999822 ) ) ;
#7094=ORIENTED_EDGE ( 'NONE', *, *, #36493, .F. ) ;
#7096=ORIENTED_EDGE ( 'NONE', *, *, #4607, .F. ) ;
#7097=CARTESIAN_POINT ( 'NONE',  ( 66.99999662536841072, -25.98076211353320275, -9.999999999999998224 ) ) ;
#7098=AXIS2_PLACEMENT_3D ( 'NONE', #8303, #25895, #34340 ) ;
#7101=FACE_BOUND ( 'NONE', #31418, .T. ) ;
#7102=EDGE_LOOP ( 'NONE', ( #4126, #19256, #33852, #25643 ) ) ;
#7103=ORIENTED_EDGE ( 'NONE', *, *, #5186, .F. ) ;
#7104=CARTESIAN_POINT ( 'NONE',  ( 12.99999662536863632, -77.94228634059960825, -9.999999999999998224 ) ) ;
#7105=ORIENTED_EDGE ( 'NONE', *, *, #20342, .F. ) ;
#7106=AXIS2_PLACEMENT_3D ( 'NONE', #2217, #22279, #13657 ) ;
#7108=CIRCLE ( 'NONE', #2326, 2.000000000000000000 ) ;
#7109=DIRECTION ( 'NONE',  ( 0.000000000000000000, 0.000000000000000000, -1.000000000000000000 ) ) ;
#7111=VERTEX_POINT ( 'NONE', #26604 ) ;
#7113=AXIS2_PLACEMENT_3D ( 'NONE', #10205, #26889, #9644 ) ;
#7114=ORIENTED_EDGE ( 'NONE', *, *, #22154, .T. ) ;
#7115=ORIENTED_EDGE ( 'NONE', *, *, #3985, .F. ) ;
#7118=ORIENTED_EDGE ( 'NONE', *, *, #29345, .T. ) ;
#7119=CARTESIAN_POINT ( 'NONE',  ( -77.00000337463097821, -8.660254037844422825, -5.000000000000000000 ) ) ;
#7120=AXIS2_PLACEMENT_3D ( 'NONE', #13389, #22582, #25227 ) ;
#7121=DIRECTION ( 'NONE',  ( 0.000000000000000000, 0.000000000000000000, 1.000000000000000000 ) ) ;
#7122=EDGE_CURVE ( 'NONE', #26515, #25741, #29419, .T. ) ;
#7123=EDGE_LOOP ( 'NONE', ( #7096, #27423, #10961, #2693, #24769 ) ) ;
#7124=CARTESIAN_POINT ( 'NONE',  ( -37.00000337463116296, 60.62177826491077326, -9.999999999999998224 ) ) ;
#7125=DIRECTION ( 'NONE',  ( 0.000000000000000000, 0.000000000000000000, -1.000000000000000000 ) ) ;
#7127=ORIENTED_EDGE ( 'NONE', *, *, #17358, .F. ) ;
#7129=EDGE_CURVE ( 'NONE', #6217, #27465, #28750, .T. ) ;
#7131=FACE_OUTER_BOUND ( 'NONE', #34149, .T. ) ;
#7132=FACE_OUTER_BOUND ( 'NONE', #22221, .T. ) ;
#7134=ADVANCED_FACE ( 'NONE', ( #5031 ), #33560, .T. ) ;
#7135=DIRECTION ( 'NONE',  ( 1.000000000000000000, 0.000000000000000000, 0.000000000000000000 ) ) ;
#7136=ADVANCED_FACE ( 'NONE', ( #27357 ), #13285, .F. ) ;
#7139=ORIENTED_EDGE ( 'NONE', *, *, #14019, .T. ) ;
#7140=CARTESIAN_POINT ( 'NONE',  ( -58.00000337463107059, -34.64101615137762025, -9.999999999999998224 ) ) ;
#7141=CARTESIAN_POINT ( 'NONE',  ( -53.00000337463109190, -60.62177826491083010, -5.000000000000000000 ) ) ;
#7142=DIRECTION ( 'NONE',  ( -1.000000000000000000, 0.000000000000000000, 0.000000000000000000 ) ) ;
#7144=EDGE_LOOP ( 'NONE', ( #8181, #6696 ) ) ;
#7145=EDGE_CURVE ( 'NONE', #4037, #25006, #33563, .T. ) ;
#7146=DIRECTION ( 'NONE',  ( 1.000000000000000000, 0.000000000000000000, 0.000000000000000000 ) ) ;
#7147=EDGE_CURVE ( 'NONE', #34111, #35831, #2426, .T. ) ;
#7148=DIRECTION ( 'NONE',  ( 1.000000000000000000, 0.000000000000000000, 0.000000000000000000 ) ) ;
#7150=ORIENTED_EDGE ( 'NONE', *, *, #31656, .F. ) ;
#7151=ADVANCED_FACE ( 'NONE', ( #19469 ), #27901, .F. ) ;
#7152=CIRCLE ( 'NONE', #16151, 95.00000000000000000 ) ;
#7153=ADVANCED_FACE ( 'NONE', ( #13665 ), #30896, .F. ) ;
#7154=FACE_OUTER_BOUND ( 'NONE', #906, .T. ) ;
#7155=ORIENTED_EDGE ( 'NONE', *, *, #28916, .T. ) ;
#7156=CIRCLE ( 'NONE', #10154, 2.000000000000001776 ) ;
#7157=DIRECTION ( 'NONE',  ( 1.000000000000000000, 0.000000000000000000, 0.000000000000000000 ) ) ;
#7158=DIRECTION ( 'NONE',  ( 0.000000000000000000, 0.000000000000000000, 1.000000000000000000 ) ) ;
#7161=VERTEX_POINT ( 'NONE', #2423 ) ;
#7162=CIRCLE ( 'NONE', #8944, 27.00000000000001421 ) ;
#7165=ORIENTED_EDGE ( 'NONE', *, *, #31999, .F. ) ;
#7166=LINE ( 'NONE', #18415, #27956 ) ;
#7167=VECTOR ( 'NONE', #305, 1000.000000000000000 ) ;
#7169=VECTOR ( 'NONE', #6308, 1000.000000000000000 ) ;
#7170=CARTESIAN_POINT ( 'NONE',  ( -55.00000337463110611, -43.30127018922202353, -9.999999999999998224 ) ) ;
#7171=CARTESIAN_POINT ( 'NONE',  ( -83.00000337463092137, -8.660254037844422825, -5.000000000000000000 ) ) ;
#7176=CARTESIAN_POINT ( 'NONE',  ( -20.00000337463124112, 69.28203230275516944, 17.49999999999999645 ) ) ;
#7177=ORIENTED_EDGE ( 'NONE', *, *, #31039, .F. ) ;
#7178=DIRECTION ( 'NONE',  ( 0.000000000000000000, 0.000000000000000000, 1.000000000000000000 ) ) ;
#7179=FACE_OUTER_BOUND ( 'NONE', #2484, .T. ) ;
#7180=AXIS2_PLACEMENT_3D ( 'NONE', #244, #9064, #6077 ) ;
#7181=ORIENTED_EDGE ( 'NONE', *, *, #16279, .T. ) ;
#7182=VERTEX_POINT ( 'NONE', #22286 ) ;
#7184=DIRECTION ( 'NONE',  ( 0.000000000000000000, 0.000000000000000000, 1.000000000000000000 ) ) ;
#7185=VECTOR ( 'NONE', #21607, 1000.000000000000000 ) ;
#7186=DIRECTION ( 'NONE',  ( 1.000000000000000000, 0.000000000000000000, 0.000000000000000000 ) ) ;
#7187=DIRECTION ( 'NONE',  ( 0.000000000000000000, 0.000000000000000000, -1.000000000000000000 ) ) ;
#7189=ORIENTED_EDGE ( 'NONE', *, *, #34064, .T. ) ;
#7190=AXIS2_PLACEMENT_3D ( 'NONE', #30625, #2675, #25024 ) ;
#7191=ORIENTED_EDGE ( 'NONE', *, *, #22663, .T. ) ;
#7192=EDGE_CURVE ( 'NONE', #2273, #15837, #34702, .T. ) ;
#7193=CARTESIAN_POINT ( 'NONE',  ( 39.99999662536853151, -69.28203230275519786, -9.999999999999998224 ) ) ;
#7194=CIRCLE ( 'NONE', #4201, 2.000000000000001776 ) ;
#7195=ORIENTED_EDGE ( 'NONE', *, *, #31020, .F. ) ;
#7197=ORIENTED_EDGE ( 'NONE', *, *, #23872, .F. ) ;
#7198=VECTOR ( 'NONE', #33107, 1000.000000000000000 ) ;
#7199=CARTESIAN_POINT ( 'NONE',  ( 39.99999662536853151, -69.28203230275519786, 12.50000000000000000 ) ) ;
#7202=CARTESIAN_POINT ( 'NONE',  ( -40.00000337463113453, -69.28203230275519786, -9.999999999999998224 ) ) ;
#7203=DIRECTION ( 'NONE',  ( 0.000000000000000000, 0.000000000000000000, 1.000000000000000000 ) ) ;
#7204=ORIENTED_EDGE ( 'NONE', *, *, #26011, .T. ) ;
#7205=ORIENTED_EDGE ( 'NONE', *, *, #14865, .F. ) ;
#7208=CIRCLE ( 'NONE', #2419, 2.000000000000000000 ) ;
#7209=CARTESIAN_POINT ( 'NONE',  ( -80.00000337463094979, -17.32050807568882078, 12.50000000000000000 ) ) ;
#7210=DIRECTION ( 'NONE',  ( 1.000000000000000000, 0.000000000000000000, 0.000000000000000000 ) ) ;
#7211=ORIENTED_EDGE ( 'NONE', *, *, #18731, .F. ) ;
#7213=EDGE_LOOP ( 'NONE', ( #31507, #20051, #23766, #26085 ) ) ;
#7214=CIRCLE ( 'NONE', #34174, 2.000000000000001776 ) ;
#7215=CARTESIAN_POINT ( 'NONE',  ( -83.00000337463092137, 25.98076211353317433, 17.49999999999999645 ) ) ;
#7217=AXIS2_PLACEMENT_3D ( 'NONE', #27713, #10853, #19128 ) ;
#7219=DIRECTION ( 'NONE',  ( 1.000000000000000000, 0.000000000000000000, 0.000000000000000000 ) ) ;
#7220=EDGE_CURVE ( 'NONE', #1919, #30886, #12517, .T. ) ;
#7221=CARTESIAN_POINT ( 'NONE',  ( -59.13646009116099833, 70.47608876694653190, -4.999999999999997335 ) ) ;
#7222=CARTESIAN_POINT ( 'NONE',  ( -33.99999999999945288, 58.88972745734214698, 12.49999999999999822 ) ) ;
#7224=EDGE_LOOP ( 'NONE', ( #21446, #20791 ) ) ;
#7225=CARTESIAN_POINT ( 'NONE',  ( 14.99999662536863632, -77.94228634059960825, 17.49999999999999645 ) ) ;
#7226=FACE_OUTER_BOUND ( 'NONE', #2706, .T. ) ;
#7227=CARTESIAN_POINT ( 'NONE',  ( 74.99999662536836809, 25.98076211353319565, 17.49999999999999645 ) ) ;
#7228=ORIENTED_EDGE ( 'NONE', *, *, #7798, .T. ) ;
#7229=EDGE_LOOP ( 'NONE', ( #14601, #27687 ) ) ;
#7231=DIRECTION ( 'NONE',  ( 1.000000000000000000, 0.000000000000000000, 0.000000000000000000 ) ) ;
#7232=LINE ( 'NONE', #35547, #12194 ) ;
#7233=CARTESIAN_POINT ( 'NONE',  ( 71.99999662536839651, 34.64101615137758472, 17.49999999999999645 ) ) ;
#7235=CYLINDRICAL_SURFACE ( 'NONE', #22730, 2.000000000000001776 ) ;
#7236=DIRECTION ( 'NONE',  ( 0.000000000000000000, 0.000000000000000000, 1.000000000000000000 ) ) ;
#7238=AXIS2_PLACEMENT_3D ( 'NONE', #34284, #31809, #17227 ) ;
#7239=EDGE_CURVE ( 'NONE', #18905, #11624, #7674, .T. ) ;
#7240=CARTESIAN_POINT ( 'NONE',  ( -63.00000337463106348, -60.62177826491083010, -9.999999999999998224 ) ) ;
#7241=ORIENTED_EDGE ( 'NONE', *, *, #27783, .T. ) ;
#7242=FACE_BOUND ( 'NONE', #19263, .T. ) ;
#7243=LINE ( 'NONE', #18859, #12366 ) ;
#7244=CYLINDRICAL_SURFACE ( 'NONE', #9556, 2.000000000000001776 ) ;
#7245=CARTESIAN_POINT ( 'NONE',  ( -62.33939050065184517, 13.89091430021398565, 12.49999999999999822 ) ) ;
#7247=CARTESIAN_POINT ( 'NONE',  ( 61.99999662536843914, -34.64101615137759893, -5.000000000000000000 ) ) ;
#7250=DIRECTION ( 'NONE',  ( -0.4999999999999980016, 0.8660254037844398178, 0.000000000000000000 ) ) ;
#7251=CYLINDRICAL_SURFACE ( 'NONE', #9601, 2.000000000000001776 ) ;
#7252=CARTESIAN_POINT ( 'NONE',  ( -23.00000337463120559, 77.94228634059957983, -9.999999999999998224 ) ) ;
#7253=ADVANCED_FACE ( 'NONE', ( #24922 ), #22459, .F. ) ;
#7254=ORIENTED_EDGE ( 'NONE', *, *, #14136, .F. ) ;
#7256=CARTESIAN_POINT ( 'NONE',  ( -70.00000337463099243, 51.96152422706637708, 12.50000000000000000 ) ) ;
#7257=LINE ( 'NONE', #32381, #14768 ) ;
#7258=ADVANCED_FACE ( 'NONE', ( #30158 ), #4485, .T. ) ;
#7259=EDGE_LOOP ( 'NONE', ( #9279, #4278 ) ) ;
#7260=CIRCLE ( 'NONE', #28210, 2.000000000000001776 ) ;
#7261=EDGE_LOOP ( 'NONE', ( #6517, #18722, #33634, #17983, #12343 ) ) ;
#7262=EDGE_CURVE ( 'NONE', #1362, #4953, #15533, .T. ) ;
#7263=CARTESIAN_POINT ( 'NONE',  ( 83.10590767357030018, -8.018049208621972568, -5.000000000000000000 ) ) ;
#7264=DIRECTION ( 'NONE',  ( 0.000000000000000000, 0.000000000000000000, -1.000000000000000000 ) ) ;
#7266=EDGE_CURVE ( 'NONE', #35823, #5530, #19215, .T. ) ;
#7267=ORIENTED_EDGE ( 'NONE', *, *, #8986, .F. ) ;
#7270=CARTESIAN_POINT ( 'NONE',  ( 64.99999662536839651, -43.30127018922199511, 17.49999999999999645 ) ) ;
#7273=VERTEX_POINT ( 'NONE', #34618 ) ;
#7274=DIRECTION ( 'NONE',  ( 0.000000000000000000, 0.000000000000000000, 1.000000000000000000 ) ) ;
#7277=EDGE_CURVE ( 'NONE', #3917, #4661, #9089, .T. ) ;
#7279=ORIENTED_EDGE ( 'NONE', *, *, #18335, .F. ) ;
#7282=ORIENTED_EDGE ( 'NONE', *, *, #30075, .F. ) ;
#7283=ORIENTED_EDGE ( 'NONE', *, *, #35507, .T. ) ;
#7284=DIRECTION ( 'NONE',  ( 0.000000000000000000, 0.000000000000000000, 1.000000000000000000 ) ) ;
#7286=ADVANCED_FACE ( 'NONE', ( #9479 ), #5933, .F. ) ;
#7287=CARTESIAN_POINT ( 'NONE',  ( 34.00000000000068923, 58.88972745734143643, -4.999999999999997335 ) ) ;
#7288=DIRECTION ( 'NONE',  ( 1.000000000000000000, 0.000000000000000000, 0.000000000000000000 ) ) ;
#7289=CYLINDRICAL_SURFACE ( 'NONE', #17310, 2.000000000000001776 ) ;
#7290=EDGE_CURVE ( 'NONE', #6890, #2002, #28692, .T. ) ;
#7291=ORIENTED_EDGE ( 'NONE', *, *, #27781, .T. ) ;
#7293=DIRECTION ( 'NONE',  ( 0.000000000000000000, -0.000000000000000000, -1.000000000000000000 ) ) ;
#7294=CYLINDRICAL_SURFACE ( 'NONE', #34617, 3.000000000000002665 ) ;
#7297=EDGE_LOOP ( 'NONE', ( #27641, #25542, #7422, #28201 ) ) ;
#7298=DIRECTION ( 'NONE',  ( -1.000000000000000000, 0.000000000000000000, 0.000000000000000000 ) ) ;
#7300=FACE_OUTER_BOUND ( 'NONE', #26228, .T. ) ;
#7301=EDGE_LOOP ( 'NONE', ( #31263, #3836 ) ) ;
#7302=EDGE_CURVE ( 'NONE', #203, #16962, #30578, .T. ) ;
#7303=CIRCLE ( 'NONE', #17466, 27.00000000000001421 ) ;
#7304=DIRECTION ( 'NONE',  ( -1.000000000000000000, 0.000000000000000000, 0.000000000000000000 ) ) ;
#7305=DIRECTION ( 'NONE',  ( 0.000000000000000000, 0.000000000000000000, -1.000000000000000000 ) ) ;
#7306=VERTEX_POINT ( 'NONE', #17528 ) ;
#7308=LINE ( 'NONE', #9568, #24018 ) ;
#7310=DIRECTION ( 'NONE',  ( 0.000000000000000000, 0.000000000000000000, 1.000000000000000000 ) ) ;
#7313=DIRECTION ( 'NONE',  ( 0.000000000000000000, 0.000000000000000000, 1.000000000000000000 ) ) ;
#7314=VERTEX_POINT ( 'NONE', #11902 ) ;
#7315=ORIENTED_EDGE ( 'NONE', *, *, #34978, .F. ) ;
#7317=CARTESIAN_POINT ( 'NONE',  ( 61.99999662536842493, 51.96152422706639129, -9.999999999999998224 ) ) ;
#7318=DIRECTION ( 'NONE',  ( 1.000000000000000000, 0.000000000000000000, 0.000000000000000000 ) ) ;
#7320=ORIENTED_EDGE ( 'NONE', *, *, #5046, .F. ) ;
#7322=FACE_OUTER_BOUND ( 'NONE', #27235, .T. ) ;
#7323=DIRECTION ( 'NONE',  ( 1.000000000000000000, 0.000000000000000000, 0.000000000000000000 ) ) ;
#7327=AXIS2_PLACEMENT_3D ( 'NONE', #4173, #29843, #12190 ) ;
#7328=CARTESIAN_POINT ( 'NONE',  ( 70.47608876694671665, 59.13646009116074964, -49.22241343995293761 ) ) ;
#7329=ORIENTED_EDGE ( 'NONE', *, *, #34064, .F. ) ;
#7331=DIRECTION ( 'NONE',  ( 0.000000000000000000, 0.000000000000000000, 1.000000000000000000 ) ) ;
#7332=ADVANCED_FACE ( 'NONE', ( #15091 ), #35373, .F. ) ;
#7333=DIRECTION ( 'NONE',  ( 0.000000000000000000, 0.000000000000000000, 1.000000000000000000 ) ) ;
#7335=EDGE_CURVE ( 'NONE', #24169, #1857, #21529, .T. ) ;
#7336=ORIENTED_EDGE ( 'NONE', *, *, #16458, .F. ) ;
#7338=EDGE_CURVE ( 'NONE', #32985, #12040, #35303, .T. ) ;
#7339=AXIS2_PLACEMENT_3D ( 'NONE', #4156, #15957, #4897 ) ;
#7342=CARTESIAN_POINT ( 'NONE',  ( 31.09745072740910388, 83.47442710120324705, 12.49999999999999645 ) ) ;
#7343=CARTESIAN_POINT ( 'NONE',  ( 71.99999662536839651, 17.32050807568879236, -5.000000000000000000 ) ) ;
#7345=DIRECTION ( 'NONE',  ( -1.000000000000000000, 0.000000000000000000, 0.000000000000000000 ) ) ;
#7346=ORIENTED_EDGE ( 'NONE', *, *, #2019, .T. ) ;
#7347=DIRECTION ( 'NONE',  ( 1.000000000000000000, 0.000000000000000000, 0.000000000000000000 ) ) ;
#7348=DIRECTION ( 'NONE',  ( -1.000000000000000000, 0.000000000000000000, 0.000000000000000000 ) ) ;
#7349=EDGE_CURVE ( 'NONE', #19893, #14036, #3111, .T. ) ;
#7351=CARTESIAN_POINT ( 'NONE',  ( 64.99999662536839651, 60.62177826491078747, -5.000000000000000000 ) ) ;
#7353=DIRECTION ( 'NONE',  ( -1.000000000000000000, 0.000000000000000000, 0.000000000000000000 ) ) ;
#7354=DIRECTION ( 'NONE',  ( 0.000000000000000000, 0.000000000000000000, 1.000000000000000000 ) ) ;
#7355=ORIENTED_EDGE ( 'NONE', *, *, #11843, .F. ) ;
#7356=VERTEX_POINT ( 'NONE', #26161 ) ;
#7358=CARTESIAN_POINT ( 'NONE',  ( 64.99999662536841072, -25.98076211353320275, 12.50000000000000000 ) ) ;
#7360=VERTEX_POINT ( 'NONE', #23166 ) ;
#7361=ORIENTED_EDGE ( 'NONE', *, *, #30865, .T. ) ;
#7363=FACE_OUTER_BOUND ( 'NONE', #17797, .T. ) ;
#7364=CIRCLE ( 'NONE', #35532, 2.000000000000001776 ) ;
#7365=EDGE_CURVE ( 'NONE', #23506, #12265, #470, .T. ) ;
#7366=VERTEX_POINT ( 'NONE', #28953 ) ;
#7367=EDGE_CURVE ( 'NONE', #1054, #32590, #29899, .T. ) ;
#7368=VERTEX_POINT ( 'NONE', #8917 ) ;
#7369=FACE_OUTER_BOUND ( 'NONE', #35217, .T. ) ;
#7371=ORIENTED_EDGE ( 'NONE', *, *, #12245, .T. ) ;
#7372=LINE ( 'NONE', #18814, #5258 ) ;
#7373=AXIS2_PLACEMENT_3D ( 'NONE', #21917, #33364, #4487 ) ;
#7374=DIRECTION ( 'NONE',  ( 0.000000000000000000, 0.000000000000000000, 1.000000000000000000 ) ) ;
#7376=ORIENTED_EDGE ( 'NONE', *, *, #18611, .T. ) ;
#7377=EDGE_CURVE ( 'NONE', #12408, #12313, #7162, .T. ) ;
#7378=DIRECTION ( 'NONE',  ( 1.000000000000000000, 0.000000000000000000, 0.000000000000000000 ) ) ;
#7380=DIRECTION ( 'NONE',  ( 0.000000000000000000, 0.000000000000000000, 1.000000000000000000 ) ) ;
#7381=CARTESIAN_POINT ( 'NONE',  ( -15.00000337463126066, 77.94228634059957983, -9.999999999999998224 ) ) ;
#7383=DIRECTION ( 'NONE',  ( 1.000000000000000000, 0.000000000000000000, 0.000000000000000000 ) ) ;
#7384=ORIENTED_EDGE ( 'NONE', *, *, #31079, .T. ) ;
#7386=DIRECTION ( 'NONE',  ( 0.000000000000000000, 0.000000000000000000, 1.000000000000000000 ) ) ;
#7387=CIRCLE ( 'NONE', #2000, 2.000000000000001776 ) ;
#7388=CARTESIAN_POINT ( 'NONE',  ( 35.83991598322139538, 56.52018970185221747, -49.22241343995293761 ) ) ;
#7389=CARTESIAN_POINT ( 'NONE',  ( 69.99999662536841072, 51.96152422706640550, -5.000000000000000000 ) ) ;
#7390=EDGE_CURVE ( 'NONE', #2540, #28847, #4162, .T. ) ;
#7391=CARTESIAN_POINT ( 'NONE',  ( -55.00000337463107059, 60.62177826491078747, 17.49999999999999645 ) ) ;
#7392=EDGE_CURVE ( 'NONE', #32947, #21445, #14915, .T. ) ;
#7393=AXIS2_PLACEMENT_3D ( 'NONE', #14779, #34682, #34480 ) ;
#7394=DIRECTION ( 'NONE',  ( 0.000000000000000000, 0.000000000000000000, 1.000000000000000000 ) ) ;
#7395=EDGE_CURVE ( 'NONE', #13632, #33336, #16136, .T. ) ;
#7398=ORIENTED_EDGE ( 'NONE', *, *, #26805, .T. ) ;
#7399=CARTESIAN_POINT ( 'NONE',  ( 73.47608876694671665, 59.13646009116074964, -49.22241343995293761 ) ) ;
#7400=DIRECTION ( 'NONE',  ( 0.000000000000000000, 0.000000000000000000, -1.000000000000000000 ) ) ;
#7401=DIRECTION ( 'NONE',  ( 0.000000000000000000, 0.000000000000000000, 1.000000000000000000 ) ) ;
#7402=CIRCLE ( 'NONE', #35019, 3.000000000000007105 ) ;
#7403=VERTEX_POINT ( 'NONE', #4027 ) ;
#7404=ORIENTED_EDGE ( 'NONE', *, *, #18758, .F. ) ;
#7406=CIRCLE ( 'NONE', #28341, 2.000000000000001776 ) ;
#7408=DIRECTION ( 'NONE',  ( 1.000000000000000000, 0.000000000000000000, 0.000000000000000000 ) ) ;
#7410=AXIS2_PLACEMENT_3D ( 'NONE', #35380, #23927, #30080 ) ;
#7411=DIRECTION ( 'NONE',  ( 1.000000000000000000, 0.000000000000000000, 0.000000000000000000 ) ) ;
#7413=EDGE_LOOP ( 'NONE', ( #2008, #4074, #20125, #24446 ) ) ;
#7415=VERTEX_POINT ( 'NONE', #30456 ) ;
#7416=FACE_BOUND ( 'NONE', #19550, .T. ) ;
#7417=AXIS2_PLACEMENT_3D ( 'NONE', #35677, #35329, #18627 ) ;
#7419=DIRECTION ( 'NONE',  ( 1.000000000000000000, 0.000000000000000000, 0.000000000000000000 ) ) ;
#7420=CARTESIAN_POINT ( 'NONE',  ( 54.99999662536846046, -43.30127018922200222, -9.999999999999998224 ) ) ;
#7422=ORIENTED_EDGE ( 'NONE', *, *, #3706, .T. ) ;
#7424=AXIS2_PLACEMENT_3D ( 'NONE', #858, #15499, #18107 ) ;
#7425=CYLINDRICAL_SURFACE ( 'NONE', #35070, 3.000000000000002665 ) ;
#7426=CYLINDRICAL_SURFACE ( 'NONE', #10473, 2.000000000000001776 ) ;
#7428=CARTESIAN_POINT ( 'NONE',  ( -78.00000337463096400, -34.64101615137762025, -9.999999999999998224 ) ) ;
#7429=DIRECTION ( 'NONE',  ( 1.000000000000000000, 0.000000000000000000, 0.000000000000000000 ) ) ;
#7433=FACE_OUTER_BOUND ( 'NONE', #18307, .T. ) ;
#7434=EDGE_LOOP ( 'NONE', ( #15665, #3103 ) ) ;
#7435=EDGE_CURVE ( 'NONE', #13911, #22954, #17331, .T. ) ;
#7436=VERTEX_POINT ( 'NONE', #36086 ) ;
#7437=CARTESIAN_POINT ( 'NONE',  ( -68.00000337463099243, 34.64101615137758472, -9.999999999999998224 ) ) ;
#7438=CARTESIAN_POINT ( 'NONE',  ( 46.99999662536849598, 60.62177826491077326, -9.999999999999998224 ) ) ;
#7439=VECTOR ( 'NONE', #33524, 1000.000000000000000 ) ;
#7440=DIRECTION ( 'NONE',  ( -0.000000000000000000, -0.000000000000000000, 1.000000000000000000 ) ) ;
#7441=EDGE_LOOP ( 'NONE', ( #33974, #17537, #6154, #2943, #31652 ) ) ;
#7442=DIRECTION ( 'NONE',  ( 1.000000000000000000, 0.000000000000000000, 0.000000000000000000 ) ) ;
#7445=FACE_OUTER_BOUND ( 'NONE', #17533, .T. ) ;
#7446=ORIENTED_EDGE ( 'NONE', *, *, #19753, .F. ) ;
#7447=CIRCLE ( 'NONE', #23000, 2.000000000000001776 ) ;
#7448=VERTEX_POINT ( 'NONE', #32701 ) ;
#7449=DIRECTION ( 'NONE',  ( 1.000000000000000000, 0.000000000000000000, 0.000000000000000000 ) ) ;
#7451=CARTESIAN_POINT ( 'NONE',  ( -70.00000337463102085, -51.96152422706641971, 17.49999999999999645 ) ) ;
#7452=ORIENTED_EDGE ( 'NONE', *, *, #2319, .T. ) ;
#7454=ORIENTED_EDGE ( 'NONE', *, *, #15395, .T. ) ;
#7455=CARTESIAN_POINT ( 'NONE',  ( -70.00000337463099243, 51.96152422706637708, -9.999999999999998224 ) ) ;
#7456=EDGE_CURVE ( 'NONE', #7637, #9530, #25130, .T. ) ;
#7457=EDGE_CURVE ( 'NONE', #8932, #30738, #5377, .T. ) ;
#7458=DIRECTION ( 'NONE',  ( 1.000000000000000000, 0.000000000000000000, 0.000000000000000000 ) ) ;
#7460=CIRCLE ( 'NONE', #8659, 2.000000000000001776 ) ;
#7462=VERTEX_POINT ( 'NONE', #1775 ) ;
#7464=CIRCLE ( 'NONE', #20036, 2.000000000000000000 ) ;
#7465=DIRECTION ( 'NONE',  ( 0.000000000000000000, 0.000000000000000000, -1.000000000000000000 ) ) ;
#7466=EDGE_CURVE ( 'NONE', #21403, #27674, #5958, .T. ) ;
#7467=DIRECTION ( 'NONE',  ( 0.000000000000000000, 0.000000000000000000, 1.000000000000000000 ) ) ;
#7468=DIRECTION ( 'NONE',  ( 1.000000000000000000, 0.000000000000000000, 0.000000000000000000 ) ) ;
#7469=ORIENTED_EDGE ( 'NONE', *, *, #8184, .T. ) ;
#7470=DIRECTION ( 'NONE',  ( 0.000000000000000000, 0.000000000000000000, 1.000000000000000000 ) ) ;
#7471=DIRECTION ( 'NONE',  ( 0.5000000000000039968, 0.8660254037844363761, 0.000000000000000000 ) ) ;
#7473=ORIENTED_EDGE ( 'NONE', *, *, #32564, .T. ) ;
#7474=VECTOR ( 'NONE', #1105, 1000.000000000000000 ) ;
#7475=CIRCLE ( 'NONE', #31416, 2.000000000000001776 ) ;
#7477=CIRCLE ( 'NONE', #33216, 33.00000000000001421 ) ;
#7478=VERTEX_POINT ( 'NONE', #24653 ) ;
#7479=AXIS2_PLACEMENT_3D ( 'NONE', #19800, #31387, #8168 ) ;
#7480=EDGE_CURVE ( 'NONE', #11344, #16972, #20915, .T. ) ;
#7481=DIRECTION ( 'NONE',  ( 1.000000000000000000, 0.000000000000000000, 0.000000000000000000 ) ) ;
#7482=VERTEX_POINT ( 'NONE', #27456 ) ;
#7483=DIRECTION ( 'NONE',  ( 0.000000000000000000, 0.000000000000000000, -1.000000000000000000 ) ) ;
#7484=DIRECTION ( 'NONE',  ( 0.000000000000000000, 0.000000000000000000, 1.000000000000000000 ) ) ;
#7485=CARTESIAN_POINT ( 'NONE',  ( 59.99999662536842493, -51.96152422706639840, -9.999999999999998224 ) ) ;
#7486=AXIS2_PLACEMENT_3D ( 'NONE', #26812, #18743, #24174 ) ;
#7487=DIRECTION ( 'NONE',  ( -0.000000000000000000, -0.000000000000000000, 1.000000000000000000 ) ) ;
#7488=DIRECTION ( 'NONE',  ( 1.000000000000000000, 0.000000000000000000, 0.000000000000000000 ) ) ;
#7489=FACE_OUTER_BOUND ( 'NONE', #32444, .T. ) ;
#7490=CARTESIAN_POINT ( 'NONE',  ( 62.99999662536841072, -25.98076211353320275, 17.49999999999999645 ) ) ;
#7491=ORIENTED_EDGE ( 'NONE', *, *, #3146, .T. ) ;
#7492=CIRCLE ( 'NONE', #22446, 2.000000000000001776 ) ;
#7493=EDGE_LOOP ( 'NONE', ( #25181, #18986, #12274, #17819 ) ) ;
#7494=CARTESIAN_POINT ( 'NONE',  ( -85.00000337463092137, 8.660254037844389075, 17.49999999999999645 ) ) ;
#7495=ADVANCED_FACE ( 'NONE', ( #27252 ), #4782, .F. ) ;
#7496=FACE_OUTER_BOUND ( 'NONE', #25199, .T. ) ;
#7497=DIRECTION ( 'NONE',  ( 0.000000000000000000, 0.000000000000000000, 1.000000000000000000 ) ) ;
#7498=CARTESIAN_POINT ( 'NONE',  ( 49.99999662536846756, 69.28203230275516944, -9.999999999999998224 ) ) ;
#7499=ORIENTED_EDGE ( 'NONE', *, *, #17102, .F. ) ;
#7500=VECTOR ( 'NONE', #20543, 1000.000000000000000 ) ;
#7501=CARTESIAN_POINT ( 'NONE',  ( 41.99999662536853151, -69.28203230275519786, -5.000000000000000000 ) ) ;
#7502=VECTOR ( 'NONE', #16008, 1000.000000000000000 ) ;
#7503=DIRECTION ( 'NONE',  ( 1.000000000000000000, 0.000000000000000000, 0.000000000000000000 ) ) ;
#7504=CYLINDRICAL_SURFACE ( 'NONE', #31155, 2.000000000000001776 ) ;
#7505=VERTEX_POINT ( 'NONE', #29897 ) ;
#7506=EDGE_CURVE ( 'NONE', #31238, #26391, #30498, .T. ) ;
#7507=LINE ( 'NONE', #35644, #22600 ) ;
#7508=ORIENTED_EDGE ( 'NONE', *, *, #27435, .F. ) ;
#7511=EDGE_CURVE ( 'NONE', #550, #29302, #14332, .T. ) ;
#7512=AXIS2_PLACEMENT_3D ( 'NONE', #33293, #1247, #13401 ) ;
#7514=ORIENTED_EDGE ( 'NONE', *, *, #20903, .T. ) ;
#7515=VECTOR ( 'NONE', #36085, 1000.000000000000000 ) ;
#7516=ORIENTED_EDGE ( 'NONE', *, *, #11134, .T. ) ;
#7518=PLANE ( 'NONE',  #36538 ) ;
#7519=CIRCLE ( 'NONE', #18900, 27.00000000000001066 ) ;
#7520=AXIS2_PLACEMENT_3D ( 'NONE', #21020, #34737, #11830 ) ;
#7522=FACE_OUTER_BOUND ( 'NONE', #30640, .T. ) ;
#7523=DIRECTION ( 'NONE',  ( 1.000000000000000000, 0.000000000000000000, 0.000000000000000000 ) ) ;
#7524=DIRECTION ( 'NONE',  ( 0.000000000000000000, 0.000000000000000000, 1.000000000000000000 ) ) ;
#7525=CARTESIAN_POINT ( 'NONE',  ( -60.00000337463107059, -34.64101615137762025, -9.999999999999998224 ) ) ;
#7527=VERTEX_POINT ( 'NONE', #27077 ) ;
#7529=AXIS2_PLACEMENT_3D ( 'NONE', #32562, #21314, #18699 ) ;
#7533=CARTESIAN_POINT ( 'NONE',  ( 79.83584911142594365, 32.64776363509508883, -5.000000000000000000 ) ) ;
#7534=DIRECTION ( 'NONE',  ( 0.000000000000000000, 0.000000000000000000, 1.000000000000000000 ) ) ;
#7535=ORIENTED_EDGE ( 'NONE', *, *, #36084, .F. ) ;
#7536=ADVANCED_FACE ( 'NONE', ( #21819 ), #12810, .F. ) ;
#7537=ORIENTED_EDGE ( 'NONE', *, *, #33856, .F. ) ;
#7538=AXIS2_PLACEMENT_3D ( 'NONE', #1385, #18653, #25028 ) ;
#7540=CARTESIAN_POINT ( 'NONE',  ( 72.99999662536836809, 43.30127018922198801, -5.000000000000000000 ) ) ;
#7541=DIRECTION ( 'NONE',  ( 0.000000000000000000, -0.000000000000000000, -1.000000000000000000 ) ) ;
#7542=AXIS2_PLACEMENT_3D ( 'NONE', #1342, #21412, #7724 ) ;
#7543=DIRECTION ( 'NONE',  ( 1.000000000000000000, 0.000000000000000000, 0.000000000000000000 ) ) ;
#7544=ORIENTED_EDGE ( 'NONE', *, *, #18131, .T. ) ;
#7545=ORIENTED_EDGE ( 'NONE', *, *, #22194, .T. ) ;
#7546=CIRCLE ( 'NONE', #17707, 27.00000000000001421 ) ;
#7547=EDGE_LOOP ( 'NONE', ( #14302, #10711 ) ) ;
#7548=CIRCLE ( 'NONE', #955, 2.000000000000001776 ) ;
#7549=AXIS2_PLACEMENT_3D ( 'NONE', #19936, #2339, #25219 ) ;
#7550=CARTESIAN_POINT ( 'NONE',  ( -58.00000337463104216, 34.64101615137757051, -5.000000000000000000 ) ) ;
#7551=AXIS2_PLACEMENT_3D ( 'NONE', #11560, #34460, #14208 ) ;
#7552=ORIENTED_EDGE ( 'NONE', *, *, #1319, .T. ) ;
#7553=CARTESIAN_POINT ( 'NONE',  ( -95.00000000000001421, 1.163414459189985801E-14, -10.00000000000000000 ) ) ;
#7554=AXIS2_PLACEMENT_3D ( 'NONE', #22249, #33688, #16821 ) ;
#7555=VERTEX_POINT ( 'NONE', #15827 ) ;
#7556=ORIENTED_EDGE ( 'NONE', *, *, #20296, .F. ) ;
#7557=AXIS2_PLACEMENT_3D ( 'NONE', #22588, #34044, #22791 ) ;
#7558=CARTESIAN_POINT ( 'NONE',  ( -77.00000337463099243, -25.98076211353322051, 17.49999999999999645 ) ) ;
#7559=EDGE_CURVE ( 'NONE', #34954, #34992, #34120, .T. ) ;
#7560=DIRECTION ( 'NONE',  ( -1.000000000000000000, 0.000000000000000000, 0.000000000000000000 ) ) ;
#7561=VERTEX_POINT ( 'NONE', #22565 ) ;
#7562=ORIENTED_EDGE ( 'NONE', *, *, #25041, .F. ) ;
#7563=CARTESIAN_POINT ( 'NONE',  ( -40.00000337463113453, 69.28203230275516944, -9.999999999999998224 ) ) ;
#7565=AXIS2_PLACEMENT_3D ( 'NONE', #34058, #28228, #5374 ) ;
#7566=CARTESIAN_POINT ( 'NONE',  ( 62.99999662536839651, -60.62177826491080168, -9.999999999999998224 ) ) ;
#7567=LINE ( 'NONE', #16374, #4102 ) ;
#7569=CARTESIAN_POINT ( 'NONE',  ( 4.999996625368645198, 77.94228634059957983, -9.999999999999998224 ) ) ;
#7570=DIRECTION ( 'NONE',  ( 1.000000000000000000, 0.000000000000000000, 0.000000000000000000 ) ) ;
#7571=DIRECTION ( 'NONE',  ( 0.000000000000000000, 0.000000000000000000, -1.000000000000000000 ) ) ;
#7572=CARTESIAN_POINT ( 'NONE',  ( 84.99999662536831124, -8.660254037844397956, -9.999999999999998224 ) ) ;
#7573=DIRECTION ( 'NONE',  ( 1.000000000000000000, 0.000000000000000000, 0.000000000000000000 ) ) ;
#7574=DIRECTION ( 'NONE',  ( 0.000000000000000000, 0.000000000000000000, 1.000000000000000000 ) ) ;
#7577=EDGE_CURVE ( 'NONE', #6948, #10265, #26319, .T. ) ;
#7578=DIRECTION ( 'NONE',  ( 0.000000000000000000, 0.000000000000000000, -1.000000000000000000 ) ) ;
#7580=ORIENTED_EDGE ( 'NONE', *, *, #19939, .F. ) ;
#7581=EDGE_CURVE ( 'NONE', #36464, #36567, #14946, .T. ) ;
#7582=DIRECTION ( 'NONE',  ( 0.000000000000000000, 0.000000000000000000, 1.000000000000000000 ) ) ;
#7585=ORIENTED_EDGE ( 'NONE', *, *, #945, .F. ) ;
#7586=CIRCLE ( 'NONE', #24968, 2.000000000000001776 ) ;
#7588=ORIENTED_EDGE ( 'NONE', *, *, #10732, .F. ) ;
#7589=EDGE_LOOP ( 'NONE', ( #6847, #17308, #19190, #29526 ) ) ;
#7590=CARTESIAN_POINT ( 'NONE',  ( 24.99999662536859546, -77.94228634059960825, -9.999999999999998224 ) ) ;
#7591=DIRECTION ( 'NONE',  ( 0.000000000000000000, 0.000000000000000000, 1.000000000000000000 ) ) ;
#7592=EDGE_CURVE ( 'NONE', #4869, #34330, #24539, .T. ) ;
#7593=ORIENTED_EDGE ( 'NONE', *, *, #910, .T. ) ;
#7594=EDGE_CURVE ( 'NONE', #8273, #10919, #3566, .T. ) ;
#7595=AXIS2_PLACEMENT_3D ( 'NONE', #35901, #10211, #7383 ) ;
#7596=DIRECTION ( 'NONE',  ( 0.000000000000000000, 0.000000000000000000, 1.000000000000000000 ) ) ;
#7597=FACE_OUTER_BOUND ( 'NONE', #22745, .T. ) ;
#7598=ORIENTED_EDGE ( 'NONE', *, *, #24319, .T. ) ;
#7599=CARTESIAN_POINT ( 'NONE',  ( -72.00000337463100664, -2.404119930384582903E-14, -9.999999999999998224 ) ) ;
#7600=ORIENTED_EDGE ( 'NONE', *, *, #12389, .T. ) ;
#7601=FACE_BOUND ( 'NONE', #21800, .T. ) ;
#7602=EDGE_CURVE ( 'NONE', #7637, #12047, #28553, .T. ) ;
#7603=AXIS2_PLACEMENT_3D ( 'NONE', #36516, #14369, #5551 ) ;
#7604=AXIS2_PLACEMENT_3D ( 'NONE', #15573, #13126, #933 ) ;
#7605=ADVANCED_FACE ( 'NONE', ( #16385 ), #2887, .F. ) ;
#7606=AXIS2_PLACEMENT_3D ( 'NONE', #15467, #18652, #24085 ) ;
#7608=DIRECTION ( 'NONE',  ( 1.000000000000000000, 0.000000000000000000, 0.000000000000000000 ) ) ;
#7609=EDGE_CURVE ( 'NONE', #942, #14720, #4811, .T. ) ;
#7611=FACE_OUTER_BOUND ( 'NONE', #25967, .T. ) ;
#7612=ADVANCED_FACE ( 'NONE', ( #2509 ), #36267, .F. ) ;
#7613=VERTEX_POINT ( 'NONE', #28191 ) ;
#7616=AXIS2_PLACEMENT_3D ( 'NONE', #27051, #1364, #35689 ) ;
#7617=CARTESIAN_POINT ( 'NONE',  ( 19.99999662536858835, 69.28203230275516944, -9.999999999999998224 ) ) ;
#7618=CARTESIAN_POINT ( 'NONE',  ( -60.00000337463104216, 51.96152422706639129, -9.999999999999998224 ) ) ;
#7619=ORIENTED_EDGE ( 'NONE', *, *, #26377, .F. ) ;
#7621=CYLINDRICAL_SURFACE ( 'NONE', #34711, 2.000000000000001776 ) ;
#7622=ORIENTED_EDGE ( 'NONE', *, *, #20422, .T. ) ;
#7623=DIRECTION ( 'NONE',  ( 0.000000000000000000, 0.000000000000000000, 1.000000000000000000 ) ) ;
#7626=FACE_OUTER_BOUND ( 'NONE', #11340, .T. ) ;
#7627=CIRCLE ( 'NONE', #23787, 2.000000000000001776 ) ;
#7628=AXIS2_PLACEMENT_3D ( 'NONE', #5460, #172, #34319 ) ;
#7629=ORIENTED_EDGE ( 'NONE', *, *, #32567, .F. ) ;
#7630=AXIS2_PLACEMENT_3D ( 'NONE', #18477, #12248, #15273 ) ;
#7631=EDGE_LOOP ( 'NONE', ( #22935, #11297 ) ) ;
#7632=FACE_OUTER_BOUND ( 'NONE', #15542, .T. ) ;
#7634=CIRCLE ( 'NONE', #28578, 2.000000000000001776 ) ;
#7635=CARTESIAN_POINT ( 'NONE',  ( -37.00000337463116296, -60.62177826491080168, 17.49999999999999645 ) ) ;
#7636=CIRCLE ( 'NONE', #28580, 33.00000000000002132 ) ;
#7637=VERTEX_POINT ( 'NONE', #13571 ) ;
#7638=VERTEX_POINT ( 'NONE', #7775 ) ;
#7639=PLANE ( 'NONE',  #12772 ) ;
#7643=DIRECTION ( 'NONE',  ( 1.000000000000000000, 0.000000000000000000, 0.000000000000000000 ) ) ;
#7644=ORIENTED_EDGE ( 'NONE', *, *, #4871, .F. ) ;
#7645=VERTEX_POINT ( 'NONE', #25214 ) ;
#7648=ORIENTED_EDGE ( 'NONE', *, *, #9673, .F. ) ;
#7649=CARTESIAN_POINT ( 'NONE',  ( 71.99999662536838230, -34.64101615137759183, 17.49999999999999645 ) ) ;
#7651=VECTOR ( 'NONE', #34983, 1000.000000000000000 ) ;
#7652=CIRCLE ( 'NONE', #28599, 2.000000000000001776 ) ;
#7654=VECTOR ( 'NONE', #11306, 1000.000000000000000 ) ;
#7655=VECTOR ( 'NONE', #27032, 1000.000000000000000 ) ;
#7656=CARTESIAN_POINT ( 'NONE',  ( -52.00000337463112032, -51.96152422706641971, 17.49999999999999645 ) ) ;
#7657=EDGE_CURVE ( 'NONE', #32118, #24986, #36461, .T. ) ;
#7658=DIRECTION ( 'NONE',  ( 0.000000000000000000, 0.000000000000000000, -1.000000000000000000 ) ) ;
#7659=ORIENTED_EDGE ( 'NONE', *, *, #15113, .T. ) ;
#7662=CIRCLE ( 'NONE', #28609, 95.00000000000001421 ) ;
#7663=CARTESIAN_POINT ( 'NONE',  ( 56.67878100130369035, -27.78182860042797131, 12.49999999999999822 ) ) ;
#7664=CARTESIAN_POINT ( 'NONE',  ( 0.000000000000000000, 0.000000000000000000, -5.000000000000000000 ) ) ;
#7665=ORIENTED_EDGE ( 'NONE', *, *, #639, .T. ) ;
#7666=CARTESIAN_POINT ( 'NONE',  ( -66.98486643701050980, 43.54686869003479899, -5.000000000000000000 ) ) ;
#7667=DIRECTION ( 'NONE',  ( 1.000000000000000000, 0.000000000000000000, 0.000000000000000000 ) ) ;
#7668=CIRCLE ( 'NONE', #33419, 3.000000000000002220 ) ;
#7669=CARTESIAN_POINT ( 'NONE',  ( 49.99999662536846756, 51.96152422706637708, 17.49999999999999645 ) ) ;
#7670=EDGE_LOOP ( 'NONE', ( #35271, #3200 ) ) ;
#7672=ORIENTED_EDGE ( 'NONE', *, *, #8278, .T. ) ;
#7673=AXIS2_PLACEMENT_3D ( 'NONE', #19914, #34356, #16558 ) ;
#7674=LINE ( 'NONE', #13461, #18541 ) ;
#7675=VERTEX_POINT ( 'NONE', #13765 ) ;
#7677=AXIS2_PLACEMENT_3D ( 'NONE', #29639, #9412, #21207 ) ;
#7678=CARTESIAN_POINT ( 'NONE',  ( 59.99999662536845335, 34.64101615137759893, 12.50000000000000000 ) ) ;
#7679=DIRECTION ( 'NONE',  ( 1.000000000000000000, 0.000000000000000000, 0.000000000000000000 ) ) ;
#7680=EDGE_CURVE ( 'NONE', #2655, #33332, #34731, .T. ) ;
#7681=AXIS2_PLACEMENT_3D ( 'NONE', #15510, #4439, #21305 ) ;
#7682=FACE_OUTER_BOUND ( 'NONE', #26598, .T. ) ;
#7683=AXIS2_PLACEMENT_3D ( 'NONE', #31852, #1132, #6743 ) ;
#7684=CARTESIAN_POINT ( 'NONE',  ( 34.99999662536855283, -60.62177826491080168, -9.999999999999998224 ) ) ;
#7685=CARTESIAN_POINT ( 'NONE',  ( 83.67710222720860713, -27.48074558388129773, -5.000000000000000000 ) ) ;
#7686=CARTESIAN_POINT ( 'NONE',  ( -72.00000337463100664, 17.32050807568877460, -9.999999999999998224 ) ) ;
#7687=CYLINDRICAL_SURFACE ( 'NONE', #17218, 2.000000000000001776 ) ;
#7690=EDGE_LOOP ( 'NONE', ( #31467, #28838, #4670, #14373 ) ) ;
#7691=CIRCLE ( 'NONE', #28633, 33.00000000000001421 ) ;
#7692=DIRECTION ( 'NONE',  ( 0.000000000000000000, 0.000000000000000000, 1.000000000000000000 ) ) ;
#7693=CARTESIAN_POINT ( 'NONE',  ( 35.19434990244975126, -52.39915983220758022, -4.999999999999997335 ) ) ;
#7694=DIRECTION ( 'NONE',  ( 0.000000000000000000, 0.000000000000000000, 1.000000000000000000 ) ) ;
#7695=CARTESIAN_POINT ( 'NONE',  ( -20.00000337463124112, 69.28203230275516944, -5.000000000000000000 ) ) ;
#7696=ORIENTED_EDGE ( 'NONE', *, *, #11404, .F. ) ;
#7698=AXIS2_PLACEMENT_3D ( 'NONE', #1464, #2023, #15728 ) ;
#7699=CARTESIAN_POINT ( 'NONE',  ( 74.99999662536836809, 8.660254037844394404, 12.50000000000000000 ) ) ;
#7701=VECTOR ( 'NONE', #24032, 1000.000000000000000 ) ;
#7702=ORIENTED_EDGE ( 'NONE', *, *, #8383, .F. ) ;
#7703=ADVANCED_FACE ( 'NONE', ( #5341 ), #36812, .F. ) ;
#7706=CIRCLE ( 'NONE', #28647, 2.000000000000001776 ) ;
#7707=DIRECTION ( 'NONE',  ( 0.000000000000000000, 0.000000000000000000, 1.000000000000000000 ) ) ;
#7708=CARTESIAN_POINT ( 'NONE',  ( 57.99999662536843914, -34.64101615137759893, 12.50000000000000000 ) ) ;
#7710=VERTEX_POINT ( 'NONE', #418 ) ;
#7711=ORIENTED_EDGE ( 'NONE', *, *, #28011, .T. ) ;
#7712=CIRCLE ( 'NONE', #24479, 2.000000000000001776 ) ;
#7713=AXIS2_PLACEMENT_3D ( 'NONE', #7381, #10009, #7210 ) ;
#7714=VERTEX_POINT ( 'NONE', #26304 ) ;
#7715=CARTESIAN_POINT ( 'NONE',  ( 84.99999662536832545, 25.98076211353319565, -9.999999999999998224 ) ) ;
#7716=ADVANCED_FACE ( 'NONE', ( #29092 ), #11850, .F. ) ;
#7717=DIRECTION ( 'NONE',  ( 0.000000000000000000, 0.000000000000000000, 1.000000000000000000 ) ) ;
#7719=DIRECTION ( 'NONE',  ( 0.000000000000000000, 0.000000000000000000, -1.000000000000000000 ) ) ;
#7720=CARTESIAN_POINT ( 'NONE',  ( 9.999996625368625658, 86.60254037844397601, -5.000000000000000000 ) ) ;
#7721=DIRECTION ( 'NONE',  ( -0.000000000000000000, -0.000000000000000000, -1.000000000000000000 ) ) ;
#7722=ADVANCED_FACE ( 'NONE', ( #17660 ), #26472, .F. ) ;
#7723=EDGE_LOOP ( 'NONE', ( #7155, #8906 ) ) ;
#7724=DIRECTION ( 'NONE',  ( -1.000000000000000000, 0.000000000000000000, 0.000000000000000000 ) ) ;
#7726=FACE_OUTER_BOUND ( 'NONE', #5599, .T. ) ;
#7727=CIRCLE ( 'NONE', #5942, 2.000000000000001776 ) ;
#7728=( NAMED_UNIT ( * ) SI_UNIT ( $, .STERADIAN. ) SOLID_ANGLE_UNIT ( ) );
#7729=VERTEX_POINT ( 'NONE', #20652 ) ;
#7730=FACE_OUTER_BOUND ( 'NONE', #3162, .T. ) ;
#7732=AXIS2_PLACEMENT_3D ( 'NONE', #34785, #20499, #6642 ) ;
#7733=CARTESIAN_POINT ( 'NONE',  ( 21.99999662536859191, 69.28203230275516944, -5.000000000000000000 ) ) ;
#7734=EDGE_LOOP ( 'NONE', ( #7189, #32021 ) ) ;
#7735=ORIENTED_EDGE ( 'NONE', *, *, #28390, .F. ) ;
#7736=EDGE_CURVE ( 'NONE', #6161, #12760, #10796, .T. ) ;
#7737=CIRCLE ( 'NONE', #23283, 3.000000000000003553 ) ;
#7738=PLANE ( 'NONE',  #36680 ) ;
#7741=ORIENTED_EDGE ( 'NONE', *, *, #34102, .T. ) ;
#7742=VERTEX_POINT ( 'NONE', #9422 ) ;
#7744=AXIS2_PLACEMENT_3D ( 'NONE', #31996, #12518, #6714 ) ;
#7745=CYLINDRICAL_SURFACE ( 'NONE', #3308, 1.999999999999998224 ) ;
#7746=AXIS2_PLACEMENT_3D ( 'NONE', #37084, #11385, #34268 ) ;
#7747=EDGE_LOOP ( 'NONE', ( #28344, #23095 ) ) ;
#7749=DIRECTION ( 'NONE',  ( 0.000000000000000000, 0.000000000000000000, 1.000000000000000000 ) ) ;
#7750=VERTEX_POINT ( 'NONE', #6421 ) ;
#7752=EDGE_LOOP ( 'NONE', ( #20234, #36014 ) ) ;
#7753=ADVANCED_FACE ( 'NONE', ( #15046 ), #20854, .F. ) ;
#7754=AXIS2_PLACEMENT_3D ( 'NONE', #21395, #4518, #29832 ) ;
#7755=CARTESIAN_POINT ( 'NONE',  ( -13.00000337463125710, -77.94228634059960825, -5.000000000000000000 ) ) ;
#7756=AXIS2_PLACEMENT_3D ( 'NONE', #8172, #1981, #28229 ) ;
#7757=CARTESIAN_POINT ( 'NONE',  ( 72.99999662536836809, 8.660254037844394404, 17.49999999999999645 ) ) ;
#7758=ORIENTED_EDGE ( 'NONE', *, *, #2980, .F. ) ;
#7759=ORIENTED_EDGE ( 'NONE', *, *, #17447, .T. ) ;
#7761=CIRCLE ( 'NONE', #29882, 2.000000000000000000 ) ;
#7762=CARTESIAN_POINT ( 'NONE',  ( -82.00000337463094979, -2.404119930384582903E-14, -9.999999999999998224 ) ) ;
#7763=EDGE_CURVE ( 'NONE', #13023, #24009, #10185, .T. ) ;
#7766=ORIENTED_EDGE ( 'NONE', *, *, #14817, .F. ) ;
#7767=DIRECTION ( 'NONE',  ( -0.000000000000000000, -0.000000000000000000, 1.000000000000000000 ) ) ;
#7768=EDGE_CURVE ( 'NONE', #7356, #9425, #23111, .T. ) ;
#7769=FACE_BOUND ( 'NONE', #5752, .T. ) ;
#7770=CYLINDRICAL_SURFACE ( 'NONE', #30980, 2.000000000000001776 ) ;
#7771=DIRECTION ( 'NONE',  ( -1.000000000000000000, 0.000000000000000000, 0.000000000000000000 ) ) ;
#7772=CARTESIAN_POINT ( 'NONE',  ( -82.00000337463094979, 34.64101615137757051, -5.000000000000000000 ) ) ;
#7774=CARTESIAN_POINT ( 'NONE',  ( -62.00000337463104927, 51.96152422706639129, 17.49999999999999645 ) ) ;
#7775=CARTESIAN_POINT ( 'NONE',  ( 77.99999662536833966, -3.224517592124143893E-15, 17.49999999999999645 ) ) ;
#7776=CYLINDRICAL_SURFACE ( 'NONE', #3189, 2.000000000000001776 ) ;
#7777=ORIENTED_EDGE ( 'NONE', *, *, #32205, .F. ) ;
#7778=CARTESIAN_POINT ( 'NONE',  ( 49.99999662536846756, 69.28203230275516944, -9.999999999999998224 ) ) ;
#7779=DIRECTION ( 'NONE',  ( 0.000000000000000000, 0.000000000000000000, 1.000000000000000000 ) ) ;
#7782=ORIENTED_EDGE ( 'NONE', *, *, #14774, .T. ) ;
#7783=ORIENTED_EDGE ( 'NONE', *, *, #17926, .F. ) ;
#7786=AXIS2_PLACEMENT_3D ( 'NONE', #23707, #12442, #6649 ) ;
#7788=LINE ( 'NONE', #24844, #8873 ) ;
#7789=AXIS2_PLACEMENT_3D ( 'NONE', #36352, #16459, #15908 ) ;
#7790=ORIENTED_EDGE ( 'NONE', *, *, #32607, .T. ) ;
#7791=DIRECTION ( 'NONE',  ( -1.000000000000000000, 0.000000000000000000, 0.000000000000000000 ) ) ;
#7792=DIRECTION ( 'NONE',  ( -0.000000000000000000, -0.000000000000000000, 1.000000000000000000 ) ) ;
#7795=EDGE_LOOP ( 'NONE', ( #28378, #32682 ) ) ;
#7796=FACE_OUTER_BOUND ( 'NONE', #31359, .T. ) ;
#7797=CIRCLE ( 'NONE', #28742, 2.000000000000001776 ) ;
#7798=EDGE_CURVE ( 'NONE', #3339, #406, #31729, .T. ) ;
#7800=CYLINDRICAL_SURFACE ( 'NONE', #28719, 2.000000000000001776 ) ;
#7801=CARTESIAN_POINT ( 'NONE',  ( -45.00000337463111322, -77.94228634059960825, 17.49999999999999645 ) ) ;
#7802=VECTOR ( 'NONE', #11487, 1000.000000000000000 ) ;
#7803=ADVANCED_FACE ( 'NONE', ( #3235 ), #26108, .F. ) ;
#7804=VERTEX_POINT ( 'NONE', #6226 ) ;
#7805=DIRECTION ( 'NONE',  ( 1.000000000000000000, 0.000000000000000000, 0.000000000000000000 ) ) ;
#7806=VECTOR ( 'NONE', #15172, 1000.000000000000000 ) ;
#7807=SHAPE_DEFINITION_REPRESENTATION ( #28906, #26771 ) ;
#7808=EDGE_CURVE ( 'NONE', #33601, #10938, #15557, .T. ) ;
#7809=DIRECTION ( 'NONE',  ( 1.000000000000000000, 0.000000000000000000, 0.000000000000000000 ) ) ;
#7811=AXIS2_PLACEMENT_3D ( 'NONE', #3714, #21135, #20565 ) ;
#7812=VERTEX_POINT ( 'NONE', #4178 ) ;
#7813=FACE_BOUND ( 'NONE', #15099, .T. ) ;
#7815=EDGE_CURVE ( 'NONE', #35811, #32676, #3008, .T. ) ;
#7816=ORIENTED_EDGE ( 'NONE', *, *, #35245, .F. ) ;
#7817=CYLINDRICAL_SURFACE ( 'NONE', #21394, 2.000000000000001776 ) ;
#7820=FACE_OUTER_BOUND ( 'NONE', #13607, .T. ) ;
#7821=DIRECTION ( 'NONE',  ( -1.000000000000000000, 0.000000000000000000, 0.000000000000000000 ) ) ;
#7822=EDGE_CURVE ( 'NONE', #14745, #28198, #27205, .T. ) ;
#7824=ORIENTED_EDGE ( 'NONE', *, *, #35676, .F. ) ;
#7825=VECTOR ( 'NONE', #6784, 1000.000000000000000 ) ;
#7826=DIRECTION ( 'NONE',  ( 0.000000000000000000, 0.000000000000000000, 1.000000000000000000 ) ) ;
#7827=DIRECTION ( 'NONE',  ( 1.000000000000000000, 0.000000000000000000, 0.000000000000000000 ) ) ;
#7828=EDGE_CURVE ( 'NONE', #18936, #11967, #6590, .T. ) ;
#7829=EDGE_CURVE ( 'NONE', #32102, #12218, #31131, .T. ) ;
#7831=VERTEX_POINT ( 'NONE', #18212 ) ;
#7832=ORIENTED_EDGE ( 'NONE', *, *, #14523, .T. ) ;
#7833=EDGE_CURVE ( 'NONE', #25354, #20763, #34147, .T. ) ;
#7834=CIRCLE ( 'NONE', #34756, 2.000000000000001776 ) ;
#7835=DIRECTION ( 'NONE',  ( 0.000000000000000000, 0.000000000000000000, 1.000000000000000000 ) ) ;
#7836=CARTESIAN_POINT ( 'NONE',  ( 32.99999662536853862, 77.94228634059959404, 12.50000000000000000 ) ) ;
#7839=ORIENTED_EDGE ( 'NONE', *, *, #25113, .T. ) ;
#7840=ORIENTED_EDGE ( 'NONE', *, *, #2780, .T. ) ;
#7842=FACE_OUTER_BOUND ( 'NONE', #30536, .T. ) ;
#7843=ORIENTED_EDGE ( 'NONE', *, *, #33232, .F. ) ;
#7845=ORIENTED_EDGE ( 'NONE', *, *, #35526, .T. ) ;
#7846=DIRECTION ( 'NONE',  ( 1.000000000000000000, 0.000000000000000000, 0.000000000000000000 ) ) ;
#7847=EDGE_CURVE ( 'NONE', #23924, #36749, #18614, .T. ) ;
#7848=DIRECTION ( 'NONE',  ( 1.000000000000000000, 0.000000000000000000, 0.000000000000000000 ) ) ;
#7849=EDGE_CURVE ( 'NONE', #5113, #30348, #28134, .T. ) ;
#7850=CARTESIAN_POINT ( 'NONE',  ( 41.99999662536853151, -69.28203230275519786, 17.49999999999999645 ) ) ;
#7854=CARTESIAN_POINT ( 'NONE',  ( -83.00000337463092137, 8.660254037844389075, -9.999999999999998224 ) ) ;
#7855=CARTESIAN_POINT ( 'NONE',  ( 0.000000000000000000, 0.000000000000000000, -5.000000000000000000 ) ) ;
#7857=ORIENTED_EDGE ( 'NONE', *, *, #26589, .F. ) ;
#7858=DIRECTION ( 'NONE',  ( 1.000000000000000000, 0.000000000000000000, 0.000000000000000000 ) ) ;
#7860=DIRECTION ( 'NONE',  ( 1.000000000000000000, 0.000000000000000000, 0.000000000000000000 ) ) ;
#7861=CARTESIAN_POINT ( 'NONE',  ( -65.00000000000000000, 0.000000000000000000, -49.86348611802629449 ) ) ;
#7863=ORIENTED_EDGE ( 'NONE', *, *, #23640, .T. ) ;
#7864=CARTESIAN_POINT ( 'NONE',  ( -85.00000337463092137, 25.98076211353317433, -9.999999999999998224 ) ) ;
#7865=ORIENTED_EDGE ( 'NONE', *, *, #27254, .F. ) ;
#7867=DIRECTION ( 'NONE',  ( 0.000000000000000000, 0.000000000000000000, 1.000000000000000000 ) ) ;
#7868=EDGE_CURVE ( 'NONE', #21906, #26245, #30407, .T. ) ;
#7870=CARTESIAN_POINT ( 'NONE',  ( -47.04203867989546950, 43.19957991610416315, 12.49999999999999822 ) ) ;
#7872=EDGE_CURVE ( 'NONE', #36949, #2973, #35942, .T. ) ;
#7873=DIRECTION ( 'NONE',  ( 0.000000000000000000, 0.000000000000000000, 1.000000000000000000 ) ) ;
#7875=FACE_OUTER_BOUND ( 'NONE', #32435, .T. ) ;
#7876=AXIS2_PLACEMENT_3D ( 'NONE', #21010, #6751, #18388 ) ;
#7878=DIRECTION ( 'NONE',  ( 0.000000000000000000, 0.000000000000000000, 1.000000000000000000 ) ) ;
#7879=ORIENTED_EDGE ( 'NONE', *, *, #1173, .T. ) ;
#7882=DIRECTION ( 'NONE',  ( -0.000000000000000000, 0.000000000000000000, -1.000000000000000000 ) ) ;
#7883=FACE_OUTER_BOUND ( 'NONE', #8028, .T. ) ;
#7884=DIRECTION ( 'NONE',  ( 0.000000000000000000, 0.000000000000000000, -1.000000000000000000 ) ) ;
#7885=ORIENTED_EDGE ( 'NONE', *, *, #22160, .T. ) ;
#7887=ORIENTED_EDGE ( 'NONE', *, *, #10930, .T. ) ;
#7889=VERTEX_POINT ( 'NONE', #4539 ) ;
#7890=EDGE_CURVE ( 'NONE', #2354, #19731, #2844, .T. ) ;
#7891=DIRECTION ( 'NONE',  ( -1.000000000000000000, 0.000000000000000000, 0.000000000000000000 ) ) ;
#7892=DIRECTION ( 'NONE',  ( -1.000000000000000000, 0.000000000000000000, -0.000000000000000000 ) ) ;
#7893=CIRCLE ( 'NONE', #36641, 2.000000000000001776 ) ;
#7894=LINE ( 'NONE', #11053, #5912 ) ;
#7895=ORIENTED_EDGE ( 'NONE', *, *, #11684, .F. ) ;
#7896=ORIENTED_EDGE ( 'NONE', *, *, #15056, .T. ) ;
#7897=AXIS2_PLACEMENT_3D ( 'NONE', #18015, #12362, #3392 ) ;
#7898=ORIENTED_EDGE ( 'NONE', *, *, #7480, .T. ) ;
#7901=CARTESIAN_POINT ( 'NONE',  ( 79.99999662536833966, 17.32050807568879236, -5.000000000000000000 ) ) ;
#7902=LINE ( 'NONE', #4732, #11489 ) ;
#7908=DIRECTION ( 'NONE',  ( 0.000000000000000000, 0.000000000000000000, 1.000000000000000000 ) ) ;
#7909=VERTEX_POINT ( 'NONE', #35666 ) ;
#7910=CARTESIAN_POINT ( 'NONE',  ( 47.04203867989577503, -43.19957991610382919, 12.49999999999999822 ) ) ;
#7911=DIRECTION ( 'NONE',  ( 0.4999999999999924505, -0.8660254037844429265, 0.000000000000000000 ) ) ;
#7912=ORIENTED_EDGE ( 'NONE', *, *, #7239, .F. ) ;
#7914=FACE_OUTER_BOUND ( 'NONE', #66, .T. ) ;
#7915=CIRCLE ( 'NONE', #23485, 2.000000000000001776 ) ;
#7917=DIRECTION ( 'NONE',  ( 1.000000000000000000, 0.000000000000000000, 0.000000000000000000 ) ) ;
#7918=CARTESIAN_POINT ( 'NONE',  ( -35.00000337463116296, 77.94228634059957983, -5.000000000000000000 ) ) ;
#7921=FACE_BOUND ( 'NONE', #29967, .T. ) ;
#7922=ORIENTED_EDGE ( 'NONE', *, *, #24091, .F. ) ;
#7923=DIRECTION ( 'NONE',  ( 1.000000000000000000, 0.000000000000000000, 0.000000000000000000 ) ) ;
#7924=ORIENTED_EDGE ( 'NONE', *, *, #16308, .F. ) ;
#7925=EDGE_CURVE ( 'NONE', #18009, #24444, #22200, .T. ) ;
#7927=CIRCLE ( 'NONE', #9117, 33.00000000000001421 ) ;
#7928=CIRCLE ( 'NONE', #742, 2.000000000000001776 ) ;
#7929=CARTESIAN_POINT ( 'NONE',  ( 29.99999662536857770, -69.28203230275519786, 12.50000000000000000 ) ) ;
#7930=CARTESIAN_POINT ( 'NONE',  ( 21.99999662536862033, -86.60254037844400443, 17.49999999999999645 ) ) ;
#7931=ORIENTED_EDGE ( 'NONE', *, *, #21492, .T. ) ;
#7932=VERTEX_POINT ( 'NONE', #9969 ) ;
#7933=DIRECTION ( 'NONE',  ( 1.000000000000000000, 0.000000000000000000, 0.000000000000000000 ) ) ;
#7934=CYLINDRICAL_SURFACE ( 'NONE', #33326, 2.000000000000001776 ) ;
#7935=DIRECTION ( 'NONE',  ( 0.000000000000000000, 0.000000000000000000, 1.000000000000000000 ) ) ;
#7936=DIRECTION ( 'NONE',  ( 0.000000000000000000, 0.000000000000000000, 1.000000000000000000 ) ) ;
#7937=EDGE_CURVE ( 'NONE', #23931, #21264, #10823, .T. ) ;
#7939=CARTESIAN_POINT ( 'NONE',  ( -85.00000337463092137, 8.660254037844389075, -9.999999999999998224 ) ) ;
#7941=FACE_BOUND ( 'NONE', #11764, .T. ) ;
#7943=PLANE ( 'NONE',  #27968 ) ;
#7944=DIRECTION ( 'NONE',  ( -1.000000000000000000, 0.000000000000000000, 0.000000000000000000 ) ) ;
#7945=DIRECTION ( 'NONE',  ( 0.000000000000000000, 0.000000000000000000, 1.000000000000000000 ) ) ;
#7946=CARTESIAN_POINT ( 'NONE',  ( 49.99999662536846756, 51.96152422706637708, -9.999999999999998224 ) ) ;
#7948=CARTESIAN_POINT ( 'NONE',  ( -50.00000337463110611, -69.28203230275519786, 12.50000000000000000 ) ) ;
#7949=ORIENTED_EDGE ( 'NONE', *, *, #19097, .F. ) ;
#7950=DIRECTION ( 'NONE',  ( 0.000000000000000000, 0.000000000000000000, 1.000000000000000000 ) ) ;
#7951=DIRECTION ( 'NONE',  ( 0.000000000000000000, 0.000000000000000000, -1.000000000000000000 ) ) ;
#7952=CYLINDRICAL_SURFACE ( 'NONE', #22928, 2.000000000000001776 ) ;
#7954=VECTOR ( 'NONE', #29814, 1000.000000000000000 ) ;
#7955=ORIENTED_EDGE ( 'NONE', *, *, #10489, .F. ) ;
#7956=ORIENTED_EDGE ( 'NONE', *, *, #17502, .F. ) ;
#7957=DIRECTION ( 'NONE',  ( 1.000000000000000000, 0.000000000000000000, 0.000000000000000000 ) ) ;
#7958=DIRECTION ( 'NONE',  ( 0.000000000000000000, 0.000000000000000000, 1.000000000000000000 ) ) ;
#7959=ORIENTED_EDGE ( 'NONE', *, *, #11473, .F. ) ;
#7960=EDGE_CURVE ( 'NONE', #32676, #35811, #7834, .T. ) ;
#7961=CARTESIAN_POINT ( 'NONE',  ( -90.60231327712325822, -15.97563234535699017, 12.49999999999999822 ) ) ;
#7962=CIRCLE ( 'NONE', #22951, 95.00000000000001421 ) ;
#7963=LINE ( 'NONE', #34345, #10543 ) ;
#7965=EDGE_CURVE ( 'NONE', #1092, #2403, #34163, .T. ) ;
#7966=DIRECTION ( 'NONE',  ( 0.000000000000000000, 0.000000000000000000, -1.000000000000000000 ) ) ;
#7967=VERTEX_POINT ( 'NONE', #33413 ) ;
#7968=DIRECTION ( 'NONE',  ( 1.000000000000000000, 0.000000000000000000, 0.000000000000000000 ) ) ;
#7969=ADVANCED_FACE ( 'NONE', ( #2080 ), #10723, .F. ) ;
#7970=CYLINDRICAL_SURFACE ( 'NONE', #4044, 2.000000000000001776 ) ;
#7972=EDGE_CURVE ( 'NONE', #31059, #4753, #3040, .T. ) ;
#7973=ORIENTED_EDGE ( 'NONE', *, *, #29463, .T. ) ;
#7974=CARTESIAN_POINT ( 'NONE',  ( 90.60231327712337190, 15.97563234535636134, -4.999999999999997335 ) ) ;
#7975=AXIS2_PLACEMENT_3D ( 'NONE', #15622, #20667, #9791 ) ;
#7978=LINE ( 'NONE', #19247, #26016 ) ;
#7979=VECTOR ( 'NONE', #22682, 1000.000000000000000 ) ;
#7980=EDGE_CURVE ( 'NONE', #25343, #11611, #29951, .T. ) ;
#7981=ORIENTED_EDGE ( 'NONE', *, *, #367, .F. ) ;
#7982=DIRECTION ( 'NONE',  ( 1.000000000000000000, 0.000000000000000000, 0.000000000000000000 ) ) ;
#7984=ORIENTED_EDGE ( 'NONE', *, *, #16808, .T. ) ;
#7985=CARTESIAN_POINT ( 'NONE',  ( 34.99999662536855283, -77.94228634059960825, -9.999999999999998224 ) ) ;
#7986=CYLINDRICAL_SURFACE ( 'NONE', #37046, 2.000000000000001776 ) ;
#7987=CARTESIAN_POINT ( 'NONE',  ( 34.99999662536855283, 60.62177826491078747, -9.999999999999998224 ) ) ;
#7988=DIRECTION ( 'NONE',  ( 1.000000000000000000, 0.000000000000000000, 0.000000000000000000 ) ) ;
#7989=ORIENTED_EDGE ( 'NONE', *, *, #28221, .F. ) ;
#7990=CIRCLE ( 'NONE', #25948, 2.000000000000001776 ) ;
#7991=EDGE_LOOP ( 'NONE', ( #27337, #23884, #15327, #25123 ) ) ;
#7992=CARTESIAN_POINT ( 'NONE',  ( 61.99999662536845335, 34.64101615137759893, 12.50000000000000000 ) ) ;
#7993=DIRECTION ( 'NONE',  ( 0.000000000000000000, 0.000000000000000000, 1.000000000000000000 ) ) ;
#7995=ADVANCED_FACE ( 'NONE', ( #24978 ), #13516, .F. ) ;
#7997=ORIENTED_EDGE ( 'NONE', *, *, #16983, .F. ) ;
#7998=LINE ( 'NONE', #22425, #2619 ) ;
#8001=ORIENTED_EDGE ( 'NONE', *, *, #20759, .F. ) ;
#8004=AXIS2_PLACEMENT_3D ( 'NONE', #28242, #27683, #16266 ) ;
#8006=DIRECTION ( 'NONE',  ( 1.000000000000000000, 0.000000000000000000, 0.000000000000000000 ) ) ;
#8007=ORIENTED_EDGE ( 'NONE', *, *, #13573, .T. ) ;
#8008=ADVANCED_FACE ( 'NONE', ( #16173 ), #13331, .F. ) ;
#8009=LINE ( 'NONE', #34264, #13734 ) ;
#8010=ORIENTED_EDGE ( 'NONE', *, *, #21098, .F. ) ;
#8011=FACE_BOUND ( 'NONE', #29377, .T. ) ;
#8013=CARTESIAN_POINT ( 'NONE',  ( 47.99999662536846756, 51.96152422706637708, -9.999999999999998224 ) ) ;
#8014=CARTESIAN_POINT ( 'NONE',  ( 32.99999662536853862, 77.94228634059959404, 17.49999999999999645 ) ) ;
#8015=VERTEX_POINT ( 'NONE', #22163 ) ;
#8017=VECTOR ( 'NONE', #31943, 1000.000000000000000 ) ;
#8018=DIRECTION ( 'NONE',  ( 1.000000000000000000, 0.000000000000000000, 0.000000000000000000 ) ) ;
#8019=EDGE_CURVE ( 'NONE', #22077, #538, #7214, .T. ) ;
#8021=DIRECTION ( 'NONE',  ( 0.000000000000000000, 0.000000000000000000, 1.000000000000000000 ) ) ;
#8022=ORIENTED_EDGE ( 'NONE', *, *, #8299, .F. ) ;
#8023=CARTESIAN_POINT ( 'NONE',  ( 81.99999662536832545, -17.32050807568879591, -5.000000000000000000 ) ) ;
#8025=CARTESIAN_POINT ( 'NONE',  ( 57.99999662536844625, 34.64101615137759893, 12.50000000000000000 ) ) ;
#8026=ORIENTED_EDGE ( 'NONE', *, *, #11674, .F. ) ;
#8028=EDGE_LOOP ( 'NONE', ( #35266, #1350, #20276, #7267, #35018 ) ) ;
#8029=CARTESIAN_POINT ( 'NONE',  ( 33.99999999999986500, -58.88972745734191250, -49.86561046011506448 ) ) ;
#8030=ORIENTED_EDGE ( 'NONE', *, *, #18531, .F. ) ;
#8031=CYLINDRICAL_SURFACE ( 'NONE', #30113, 3.000000000000006217 ) ;
#8032=FACE_OUTER_BOUND ( 'NONE', #13422, .T. ) ;
#8034=DIRECTION ( 'NONE',  ( 0.000000000000000000, 0.000000000000000000, 1.000000000000000000 ) ) ;
#8037=CARTESIAN_POINT ( 'NONE',  ( 66.99999662536839651, 60.62177826491078747, 17.49999999999999645 ) ) ;
#8038=DIRECTION ( 'NONE',  ( 0.000000000000000000, 0.000000000000000000, 1.000000000000000000 ) ) ;
#8040=EDGE_CURVE ( 'NONE', #18995, #10128, #16800, .T. ) ;
#8041=DIRECTION ( 'NONE',  ( 0.000000000000000000, 0.000000000000000000, 1.000000000000000000 ) ) ;
#8042=DIRECTION ( 'NONE',  ( 0.000000000000000000, -0.000000000000000000, -1.000000000000000000 ) ) ;
#8043=ORIENTED_EDGE ( 'NONE', *, *, #14919, .T. ) ;
#8045=ORIENTED_EDGE ( 'NONE', *, *, #11989, .F. ) ;
#8046=FACE_OUTER_BOUND ( 'NONE', #23768, .T. ) ;
#8050=DIRECTION ( 'NONE',  ( 0.000000000000000000, 0.000000000000000000, 1.000000000000000000 ) ) ;
#8051=ADVANCED_FACE ( 'NONE', ( #7726 ), #10525, .F. ) ;
#8052=ORIENTED_EDGE ( 'NONE', *, *, #34402, .T. ) ;
#8054=EDGE_CURVE ( 'NONE', #34770, #10069, #6614, .T. ) ;
#8055=AXIS2_PLACEMENT_3D ( 'NONE', #35184, #20362, #11719 ) ;
#8058=ORIENTED_EDGE ( 'NONE', *, *, #22695, .F. ) ;
#8061=ADVANCED_FACE ( 'NONE', ( #10893 ), #2637, .F. ) ;
#8063=DIRECTION ( 'NONE',  ( 0.000000000000000000, 0.000000000000000000, 1.000000000000000000 ) ) ;
#8064=AXIS2_PLACEMENT_3D ( 'NONE', #12895, #1460, #15547 ) ;
#8065=AXIS2_PLACEMENT_3D ( 'NONE', #4716, #2054, #13490 ) ;
#8067=CARTESIAN_POINT ( 'NONE',  ( -50.00000337463112032, -51.96152422706641971, -5.000000000000000000 ) ) ;
#8069=VECTOR ( 'NONE', #10614, 1000.000000000000000 ) ;
#8072=ORIENTED_EDGE ( 'NONE', *, *, #8192, .F. ) ;
#8073=ORIENTED_EDGE ( 'NONE', *, *, #27203, .F. ) ;
#8076=ORIENTED_EDGE ( 'NONE', *, *, #709, .F. ) ;
#8078=DIRECTION ( 'NONE',  ( 0.000000000000000000, 0.000000000000000000, 1.000000000000000000 ) ) ;
#8079=CYLINDRICAL_SURFACE ( 'NONE', #11384, 2.000000000000000000 ) ;
#8080=CIRCLE ( 'NONE', #9892, 2.000000000000001776 ) ;
#8082=DIRECTION ( 'NONE',  ( 0.000000000000000000, 0.000000000000000000, 1.000000000000000000 ) ) ;
#8083=CARTESIAN_POINT ( 'NONE',  ( 32.99999662536855283, 60.62177826491078747, -5.000000000000000000 ) ) ;
#8084=ORIENTED_EDGE ( 'NONE', *, *, #19887, .F. ) ;
#8085=CARTESIAN_POINT ( 'NONE',  ( -65.00000337463102085, 60.62177826491077326, -9.999999999999998224 ) ) ;
#8086=CIRCLE ( 'NONE', #36218, 2.000000000000001776 ) ;
#8088=CARTESIAN_POINT ( 'NONE',  ( 37.99999662536853151, 69.28203230275518365, -9.999999999999998224 ) ) ;
#8090=DIRECTION ( 'NONE',  ( 0.4999999999999919509, -0.8660254037844432595, 0.000000000000000000 ) ) ;
#8092=VECTOR ( 'NONE', #22649, 1000.000000000000000 ) ;
#8093=EDGE_LOOP ( 'NONE', ( #31856, #10527, #34513, #31870 ) ) ;
#8094=VECTOR ( 'NONE', #26334, 1000.000000000000000 ) ;
#8095=VERTEX_POINT ( 'NONE', #26257 ) ;
#8097=FACE_OUTER_BOUND ( 'NONE', #31714, .T. ) ;
#8100=ORIENTED_EDGE ( 'NONE', *, *, #32186, .F. ) ;
#8101=LINE ( 'NONE', #5105, #11706 ) ;
#8102=CIRCLE ( 'NONE', #35051, 2.000000000000001776 ) ;
#8103=VERTEX_POINT ( 'NONE', #17071 ) ;
#8105=CARTESIAN_POINT ( 'NONE',  ( -50.00000337463110611, -69.28203230275519786, -5.000000000000000000 ) ) ;
#8106=ORIENTED_EDGE ( 'NONE', *, *, #24579, .F. ) ;
#8107=CIRCLE ( 'NONE', #30260, 2.000000000000001776 ) ;
#8108=AXIS2_PLACEMENT_3D ( 'NONE', #30527, #10833, #19102 ) ;
#8109=EDGE_LOOP ( 'NONE', ( #154, #18243, #8834, #24639 ) ) ;
#8110=AXIS2_PLACEMENT_3D ( 'NONE', #21881, #32962, #7449 ) ;
#8111=DIRECTION ( 'NONE',  ( 1.000000000000000000, 0.000000000000000000, 0.000000000000000000 ) ) ;
#8112=DIRECTION ( 'NONE',  ( 0.000000000000000000, 0.000000000000000000, 1.000000000000000000 ) ) ;
#8116=CARTESIAN_POINT ( 'NONE',  ( -68.00000337463099243, 34.64101615137758472, -5.000000000000000000 ) ) ;
#8117=AXIS2_PLACEMENT_3D ( 'NONE', #8929, #34810, #12466 ) ;
#8118=FACE_OUTER_BOUND ( 'NONE', #23135, .T. ) ;
#8119=CARTESIAN_POINT ( 'NONE',  ( -70.00000337463099243, 17.32050807568877460, -9.999999999999998224 ) ) ;
#8120=CIRCLE ( 'NONE', #25489, 2.000000000000001776 ) ;
#8121=DIRECTION ( 'NONE',  ( 1.000000000000000000, 0.000000000000000000, 0.000000000000000000 ) ) ;
#8122=ORIENTED_EDGE ( 'NONE', *, *, #25808, .F. ) ;
#8123=CYLINDRICAL_SURFACE ( 'NONE', #24948, 3.000000000000005773 ) ;
#8124=FACE_BOUND ( 'NONE', #29413, .T. ) ;
#8125=LINE ( 'NONE', #19569, #12381 ) ;
#8127=CARTESIAN_POINT ( 'NONE',  ( -48.00000337463110611, -69.28203230275519786, -9.999999999999998224 ) ) ;
#8129=DIRECTION ( 'NONE',  ( 0.000000000000000000, 0.000000000000000000, 1.000000000000000000 ) ) ;
#8130=VECTOR ( 'NONE', #6415, 1000.000000000000000 ) ;
#8131=DIRECTION ( 'NONE',  ( -1.000000000000000000, 0.000000000000000000, 0.000000000000000000 ) ) ;
#8132=VERTEX_POINT ( 'NONE', #29246 ) ;
#8133=DIRECTION ( 'NONE',  ( -0.000000000000000000, -0.000000000000000000, 1.000000000000000000 ) ) ;
#8134=DIRECTION ( 'NONE',  ( 0.000000000000000000, 0.000000000000000000, -1.000000000000000000 ) ) ;
#8135=CARTESIAN_POINT ( 'NONE',  ( 54.99999662536844625, 43.30127018922198801, -9.999999999999998224 ) ) ;
#8136=VECTOR ( 'NONE', #14770, 1000.000000000000000 ) ;
#8137=EDGE_CURVE ( 'NONE', #575, #14128, #14992, .T. ) ;
#8138=AXIS2_PLACEMENT_3D ( 'NONE', #32829, #26631, #7148 ) ;
#8140=EDGE_CURVE ( 'NONE', #35823, #27946, #5633, .T. ) ;
#8141=ORIENTED_EDGE ( 'NONE', *, *, #34442, .F. ) ;
#8142=CIRCLE ( 'NONE', #926, 27.00000000000001421 ) ;
#8143=ORIENTED_EDGE ( 'NONE', *, *, #21711, .F. ) ;
#8144=VERTEX_POINT ( 'NONE', #6182 ) ;
#8145=CARTESIAN_POINT ( 'NONE',  ( -78.00000337463096400, -34.64101615137762025, -5.000000000000000000 ) ) ;
#8147=ORIENTED_EDGE ( 'NONE', *, *, #19080, .F. ) ;
#8148=CIRCLE ( 'NONE', #17721, 1.999999999999998224 ) ;
#8150=EDGE_CURVE ( 'NONE', #26529, #30363, #29362, .T. ) ;
#8151=EDGE_LOOP ( 'NONE', ( #16181, #24279, #16352, #31710, #35573, #33440, #7562, #31023 ) ) ;
#8152=CARTESIAN_POINT ( 'NONE',  ( -35.00000337463117717, -77.94228634059963667, 17.49999999999999645 ) ) ;
#8154=CARTESIAN_POINT ( 'NONE',  ( 47.63139720814418610, 27.49999999999988987, -5.000000000000000000 ) ) ;
#8155=VERTEX_POINT ( 'NONE', #32030 ) ;
#8156=FACE_OUTER_BOUND ( 'NONE', #26241, .T. ) ;
#8157=CARTESIAN_POINT ( 'NONE',  ( 51.99999662536848888, -51.96152422706640550, 17.49999999999999645 ) ) ;
#8158=AXIS2_PLACEMENT_3D ( 'NONE', #34323, #11266, #33965 ) ;
#8159=EDGE_CURVE ( 'NONE', #10243, #6282, #19795, .T. ) ;
#8161=DIRECTION ( 'NONE',  ( 0.000000000000000000, 0.000000000000000000, 1.000000000000000000 ) ) ;
#8162=AXIS2_PLACEMENT_3D ( 'NONE', #32712, #2521, #31203 ) ;
#8163=CIRCLE ( 'NONE', #24298, 2.000000000000001776 ) ;
#8165=CIRCLE ( 'NONE', #31479, 2.000000000000001776 ) ;
#8166=AXIS2_PLACEMENT_3D ( 'NONE', #21652, #27081, #27260 ) ;
#8168=DIRECTION ( 'NONE',  ( -1.000000000000000000, 0.000000000000000000, 0.000000000000000000 ) ) ;
#8169=CIRCLE ( 'NONE', #32097, 2.000000000000001776 ) ;
#8170=VERTEX_POINT ( 'NONE', #179 ) ;
#8171=FACE_OUTER_BOUND ( 'NONE', #706, .T. ) ;
#8172=CARTESIAN_POINT ( 'NONE',  ( 34.99999662536853862, 77.94228634059959404, 17.49999999999999645 ) ) ;
#8174=DIRECTION ( 'NONE',  ( -1.000000000000000000, 0.000000000000000000, 0.000000000000000000 ) ) ;
#8175=CARTESIAN_POINT ( 'NONE',  ( -51.13139720814380240, 27.50000000000055422, -5.000000000000000000 ) ) ;
#8177=DIRECTION ( 'NONE',  ( 1.000000000000000000, 0.000000000000000000, 0.000000000000000000 ) ) ;
#8178=CIRCLE ( 'NONE', #13580, 2.000000000000001776 ) ;
#8180=EDGE_CURVE ( 'NONE', #10442, #31670, #20982, .T. ) ;
#8181=ORIENTED_EDGE ( 'NONE', *, *, #15653, .F. ) ;
#8183=DIRECTION ( 'NONE',  ( 1.000000000000000000, 0.000000000000000000, 0.000000000000000000 ) ) ;
#8184=EDGE_CURVE ( 'NONE', #36367, #11611, #23446, .T. ) ;
#8185=CIRCLE ( 'NONE', #12959, 2.000000000000001776 ) ;
#8187=ORIENTED_EDGE ( 'NONE', *, *, #17535, .F. ) ;
#8188=AXIS2_PLACEMENT_3D ( 'NONE', #28102, #474, #36723 ) ;
#8191=CARTESIAN_POINT ( 'NONE',  ( 1.999996625368696490, -86.60254037844400443, -9.999999999999998224 ) ) ;
#8192=EDGE_CURVE ( 'NONE', #17871, #23793, #15008, .T. ) ;
#8194=CARTESIAN_POINT ( 'NONE',  ( -85.00000337463092137, -25.98076211353322051, -9.999999999999998224 ) ) ;
#8197=ORIENTED_EDGE ( 'NONE', *, *, #27873, .T. ) ;
#8198=CIRCLE ( 'NONE', #2789, 2.000000000000001776 ) ;
#8199=EDGE_LOOP ( 'NONE', ( #27898, #36787, #12123, #35997 ) ) ;
#8200=DIRECTION ( 'NONE',  ( -0.000000000000000000, -0.000000000000000000, 1.000000000000000000 ) ) ;
#8201=CIRCLE ( 'NONE', #5202, 2.000000000000001776 ) ;
#8202=EDGE_CURVE ( 'NONE', #7356, #203, #23380, .T. ) ;
#8203=CARTESIAN_POINT ( 'NONE',  ( 64.99999662536841072, 25.98076211353318854, -9.999999999999998224 ) ) ;
#8205=CARTESIAN_POINT ( 'NONE',  ( 71.99999662536839651, 34.64101615137758472, -5.000000000000000000 ) ) ;
#8207=CARTESIAN_POINT ( 'NONE',  ( 69.99999662536841072, 51.96152422706640550, -9.999999999999998224 ) ) ;
#8208=AXIS2_PLACEMENT_3D ( 'NONE', #16913, #22743, #13909 ) ;
#8209=DIRECTION ( 'NONE',  ( 1.000000000000000000, 0.000000000000000000, 0.000000000000000000 ) ) ;
#8210=ORIENTED_EDGE ( 'NONE', *, *, #14171, .F. ) ;
#8213=AXIS2_PLACEMENT_3D ( 'NONE', #1721, #21600, #18970 ) ;
#8214=FACE_OUTER_BOUND ( 'NONE', #6745, .T. ) ;
#8215=EDGE_CURVE ( 'NONE', #35442, #12315, #12154, .T. ) ;
#8216=CIRCLE ( 'NONE', #17209, 2.000000000000001776 ) ;
#8217=DIRECTION ( 'NONE',  ( -0.000000000000000000, -0.000000000000000000, 1.000000000000000000 ) ) ;
#8218=DIRECTION ( 'NONE',  ( -0.000000000000000000, -0.000000000000000000, 1.000000000000000000 ) ) ;
#8220=ORIENTED_EDGE ( 'NONE', *, *, #32957, .F. ) ;
#8221=DIRECTION ( 'NONE',  ( 1.000000000000000000, 0.000000000000000000, 0.000000000000000000 ) ) ;
#8222=CARTESIAN_POINT ( 'NONE',  ( -45.00000337463111322, 77.94228634059959404, -9.999999999999998224 ) ) ;
#8223=CARTESIAN_POINT ( 'NONE',  ( -80.00000337463094979, 34.64101615137757051, 17.49999999999999645 ) ) ;
#8224=CIRCLE ( 'NONE', #11207, 33.00000000000001421 ) ;
#8225=EDGE_CURVE ( 'NONE', #37038, #33197, #31493, .T. ) ;
#8226=CIRCLE ( 'NONE', #6419, 2.000000000000000000 ) ;
#8227=ORIENTED_EDGE ( 'NONE', *, *, #7609, .F. ) ;
#8228=ORIENTED_EDGE ( 'NONE', *, *, #3713, .F. ) ;
#8230=DIRECTION ( 'NONE',  ( -0.8660254037844380415, 0.5000000000000009992, 0.000000000000000000 ) ) ;
#8231=VERTEX_POINT ( 'NONE', #26061 ) ;
#8232=CARTESIAN_POINT ( 'NONE',  ( -17.00000337463125533, -77.94228634059960825, -9.999999999999998224 ) ) ;
#8233=CIRCLE ( 'NONE', #22013, 2.000000000000001776 ) ;
#8234=DIRECTION ( 'NONE',  ( 0.000000000000000000, 0.000000000000000000, 1.000000000000000000 ) ) ;
#8236=DIRECTION ( 'NONE',  ( 0.000000000000000000, 0.000000000000000000, -1.000000000000000000 ) ) ;
#8237=CARTESIAN_POINT ( 'NONE',  ( 56.52018970185258695, -35.83991598322081273, -49.22241343995298024 ) ) ;
#8240=DIRECTION ( 'NONE',  ( 1.000000000000000000, 0.000000000000000000, 0.000000000000000000 ) ) ;
#8241=CIRCLE ( 'NONE', #10028, 2.000000000000000000 ) ;
#8242=LINE ( 'NONE', #17028, #6487 ) ;
#8243=EDGE_LOOP ( 'NONE', ( #16364, #9105, #17016 ) ) ;
#8244=ORIENTED_EDGE ( 'NONE', *, *, #31663, .F. ) ;
#8245=CARTESIAN_POINT ( 'NONE',  ( 69.99999662536839651, 34.64101615137758472, -5.000000000000000000 ) ) ;
#8246=EDGE_CURVE ( 'NONE', #2447, #21044, #4835, .T. ) ;
#8247=AXIS2_PLACEMENT_3D ( 'NONE', #14665, #11118, #31732 ) ;
#8248=DIRECTION ( 'NONE',  ( 1.000000000000000000, 0.000000000000000000, 0.000000000000000000 ) ) ;
#8249=CARTESIAN_POINT ( 'NONE',  ( 4.999996625368645198, 77.94228634059957983, -9.999999999999998224 ) ) ;
#8251=EDGE_LOOP ( 'NONE', ( #30137, #23167, #993, #1088 ) ) ;
#8252=AXIS2_PLACEMENT_3D ( 'NONE', #14579, #22674, #28827 ) ;
#8253=AXIS2_PLACEMENT_3D ( 'NONE', #30783, #36441, #8316 ) ;
#8254=FACE_BOUND ( 'NONE', #5395, .T. ) ;
#8255=VERTEX_POINT ( 'NONE', #15931 ) ;
#8256=ORIENTED_EDGE ( 'NONE', *, *, #32963, .T. ) ;
#8258=ORIENTED_EDGE ( 'NONE', *, *, #15040, .F. ) ;
#8260=DIRECTION ( 'NONE',  ( 0.000000000000000000, 0.000000000000000000, 1.000000000000000000 ) ) ;
#8261=DIRECTION ( 'NONE',  ( 0.000000000000000000, 0.000000000000000000, -1.000000000000000000 ) ) ;
#8262=EDGE_CURVE ( 'NONE', #23780, #22507, #25793, .T. ) ;
#8263=CIRCLE ( 'NONE', #24430, 2.000000000000001776 ) ;
#8264=CARTESIAN_POINT ( 'NONE',  ( -4.279621169095561228, 62.97617850287782915, -4.999999999999997335 ) ) ;
#8265=EDGE_LOOP ( 'NONE', ( #33661, #11069, #20677, #35870 ) ) ;
#8266=ADVANCED_FACE ( 'NONE', ( #36006 ), #3745, .F. ) ;
#8269=CIRCLE ( 'NONE', #1678, 2.000000000000001776 ) ;
#8270=ORIENTED_EDGE ( 'NONE', *, *, #4537, .T. ) ;
#8271=AXIS2_PLACEMENT_3D ( 'NONE', #23011, #17561, #28986 ) ;
#8272=ADVANCED_FACE ( 'NONE', ( #7131 ), #9740, .F. ) ;
#8273=VERTEX_POINT ( 'NONE', #1480 ) ;
#8274=AXIS2_PLACEMENT_3D ( 'NONE', #12354, #3579, #28866 ) ;
#8275=VERTEX_POINT ( 'NONE', #18173 ) ;
#8276=CARTESIAN_POINT ( 'NONE',  ( -12.00000337463128908, 69.28203230275516944, -9.999999999999998224 ) ) ;
#8277=LINE ( 'NONE', #24972, #25161 ) ;
#8278=EDGE_CURVE ( 'NONE', #31054, #29052, #7308, .T. ) ;
#8283=ORIENTED_EDGE ( 'NONE', *, *, #897, .F. ) ;
#8284=DIRECTION ( 'NONE',  ( 1.000000000000000000, 0.000000000000000000, 0.000000000000000000 ) ) ;
#8285=AXIS2_PLACEMENT_3D ( 'NONE', #25852, #33926, #22856 ) ;
#8286=CARTESIAN_POINT ( 'NONE',  ( 4.279621169095998212, -62.97617850287780072, 12.49999999999999822 ) ) ;
#8287=LINE ( 'NONE', #181, #36178 ) ;
#8289=DIRECTION ( 'NONE',  ( 1.000000000000000000, 0.000000000000000000, 0.000000000000000000 ) ) ;
#8291=AXIS2_PLACEMENT_3D ( 'NONE', #4862, #21907, #10285 ) ;
#8292=ADVANCED_FACE ( 'NONE', ( #1684 ), #4312, .F. ) ;
#8293=ORIENTED_EDGE ( 'NONE', *, *, #33614, .F. ) ;
#8294=ADVANCED_FACE ( 'NONE', ( #6932 ), #13121, .F. ) ;
#8296=CARTESIAN_POINT ( 'NONE',  ( 68.19171716056558807, -52.81599796988855644, 12.50000000000000000 ) ) ;
#8297=EDGE_CURVE ( 'NONE', #520, #25333, #18014, .T. ) ;
#8298=AXIS2_PLACEMENT_3D ( 'NONE', #19365, #30784, #9204 ) ;
#8299=EDGE_CURVE ( 'NONE', #25770, #2284, #27003, .T. ) ;
#8300=DIRECTION ( 'NONE',  ( -0.8660254037844379305, 0.5000000000000011102, 0.000000000000000000 ) ) ;
#8301=CARTESIAN_POINT ( 'NONE',  ( -69.13212189986965939, -2.778182860042805125, -49.86348611802629449 ) ) ;
#8302=EDGE_CURVE ( 'NONE', #26696, #17068, #24374, .T. ) ;
#8303=CARTESIAN_POINT ( 'NONE',  ( 44.99999662536849598, -77.94228634059960825, -9.999999999999998224 ) ) ;
#8304=ORIENTED_EDGE ( 'NONE', *, *, #12992, .F. ) ;
#8305=ORIENTED_EDGE ( 'NONE', *, *, #21098, .T. ) ;
#8306=AXIS2_PLACEMENT_3D ( 'NONE', #9562, #32421, #1121 ) ;
#8309=VECTOR ( 'NONE', #29995, 1000.000000000000000 ) ;
#8311=CARTESIAN_POINT ( 'NONE',  ( 36.99999662536855283, 60.62177826491078747, 17.49999999999999645 ) ) ;
#8312=EDGE_LOOP ( 'NONE', ( #23689, #20270 ) ) ;
#8313=CIRCLE ( 'NONE', #7098, 2.000000000000001776 ) ;
#8314=ORIENTED_EDGE ( 'NONE', *, *, #14441, .F. ) ;
#8315=AXIS2_PLACEMENT_3D ( 'NONE', #4385, #25019, #12796 ) ;
#8316=DIRECTION ( 'NONE',  ( 1.000000000000000000, 0.000000000000000000, 0.000000000000000000 ) ) ;
#8317=CARTESIAN_POINT ( 'NONE',  ( -73.00000337463100664, -43.30127018922202353, -9.999999999999998224 ) ) ;
#8318=ORIENTED_EDGE ( 'NONE', *, *, #24301, .T. ) ;
#8319=VERTEX_POINT ( 'NONE', #32242 ) ;
#8320=DIRECTION ( 'NONE',  ( 0.000000000000000000, 0.000000000000000000, -1.000000000000000000 ) ) ;
#8321=DIRECTION ( 'NONE',  ( 0.000000000000000000, 0.000000000000000000, 1.000000000000000000 ) ) ;
#8322=FACE_OUTER_BOUND ( 'NONE', #24689, .T. ) ;
#8323=DIRECTION ( 'NONE',  ( 0.000000000000000000, 0.000000000000000000, 1.000000000000000000 ) ) ;
#8324=ORIENTED_EDGE ( 'NONE', *, *, #6821, .F. ) ;
#8325=DIRECTION ( 'NONE',  ( 1.000000000000000000, 0.000000000000000000, 0.000000000000000000 ) ) ;
#8326=FACE_BOUND ( 'NONE', #17428, .T. ) ;
#8327=AXIS2_PLACEMENT_3D ( 'NONE', #3649, #17350, #256 ) ;
#8330=CARTESIAN_POINT ( 'NONE',  ( -4.279621169095561228, 62.97617850287782915, -4.999999999999997335 ) ) ;
#8331=DIRECTION ( 'NONE',  ( 0.000000000000000000, 0.000000000000000000, -1.000000000000000000 ) ) ;
#8332=CARTESIAN_POINT ( 'NONE',  ( -52.39915983220772233, -35.19434990244957362, -4.999999999999997335 ) ) ;
#8333=CIRCLE ( 'NONE', #11319, 27.00000000000001066 ) ;
#8334=DIRECTION ( 'NONE',  ( 1.000000000000000000, 0.000000000000000000, 0.000000000000000000 ) ) ;
#8335=ORIENTED_EDGE ( 'NONE', *, *, #34866, .T. ) ;
#8336=DIRECTION ( 'NONE',  ( 0.000000000000000000, 0.000000000000000000, 1.000000000000000000 ) ) ;
#8338=DIRECTION ( 'NONE',  ( 0.000000000000000000, 0.000000000000000000, 1.000000000000000000 ) ) ;
#8339=CIRCLE ( 'NONE', #22701, 2.000000000000001776 ) ;
#8340=VERTEX_POINT ( 'NONE', #6570 ) ;
#8341=ADVANCED_FACE ( 'NONE', ( #20998 ), #29802, .F. ) ;
#8342=ORIENTED_EDGE ( 'NONE', *, *, #7192, .F. ) ;
#8345=EDGE_CURVE ( 'NONE', #11561, #5584, #18615, .T. ) ;
#8346=CYLINDRICAL_SURFACE ( 'NONE', #15954, 2.000000000000001776 ) ;
#8349=CARTESIAN_POINT ( 'NONE',  ( 66.99999662536839651, -43.30127018922199511, 17.49999999999999645 ) ) ;
#8350=AXIS2_PLACEMENT_3D ( 'NONE', #12532, #1462, #35988 ) ;
#8351=VERTEX_POINT ( 'NONE', #1128 ) ;
#8353=VERTEX_POINT ( 'NONE', #1304 ) ;
#8354=AXIS2_PLACEMENT_3D ( 'NONE', #6723, #15548, #20980 ) ;
#8355=CARTESIAN_POINT ( 'NONE',  ( 0.000000000000000000, 0.000000000000000000, -10.00000000000000000 ) ) ;
#8356=ORIENTED_EDGE ( 'NONE', *, *, #22485, .F. ) ;
#8357=CYLINDRICAL_SURFACE ( 'NONE', #19014, 2.000000000000000000 ) ;
#8358=DIRECTION ( 'NONE',  ( 0.000000000000000000, 0.000000000000000000, -1.000000000000000000 ) ) ;
#8359=AXIS2_PLACEMENT_3D ( 'NONE', #16592, #16789, #13785 ) ;
#8361=DIRECTION ( 'NONE',  ( 0.000000000000000000, 0.000000000000000000, -1.000000000000000000 ) ) ;
#8362=AXIS2_PLACEMENT_3D ( 'NONE', #10649, #33539, #1449 ) ;
#8364=DIRECTION ( 'NONE',  ( 0.000000000000000000, 0.000000000000000000, -1.000000000000000000 ) ) ;
#8365=CARTESIAN_POINT ( 'NONE',  ( 15.97563234535730814, -90.60231327712320137, -4.999999999999997335 ) ) ;
#8367=ORIENTED_EDGE ( 'NONE', *, *, #2544, .F. ) ;
#8368=CARTESIAN_POINT ( 'NONE',  ( 82.99999662536831124, -25.98076211353319565, 12.50000000000000000 ) ) ;
#8369=CARTESIAN_POINT ( 'NONE',  ( -5.000003374631307729, 77.94228634059957983, -5.000000000000000000 ) ) ;
#8370=VERTEX_POINT ( 'NONE', #2595 ) ;
#8372=DIRECTION ( 'NONE',  ( 1.000000000000000000, 0.000000000000000000, 0.000000000000000000 ) ) ;
#8373=CARTESIAN_POINT ( 'NONE',  ( 76.99999662536836809, 8.660254037844394404, 12.50000000000000000 ) ) ;
#8374=FACE_OUTER_BOUND ( 'NONE', #8643, .T. ) ;
#8376=ORIENTED_EDGE ( 'NONE', *, *, #21797, .F. ) ;
#8377=EDGE_LOOP ( 'NONE', ( #33138, #23680 ) ) ;
#8378=CIRCLE ( 'NONE', #19169, 3.499999999999989342 ) ;
#8380=CARTESIAN_POINT ( 'NONE',  ( 56.67878100130369035, -27.78182860042797131, -4.999999999999997335 ) ) ;
#8381=VERTEX_POINT ( 'NONE', #25127 ) ;
#8382=VERTEX_POINT ( 'NONE', #16854 ) ;
#8383=EDGE_CURVE ( 'NONE', #12339, #36437, #22222, .T. ) ;
#8385=CARTESIAN_POINT ( 'NONE',  ( -55.00000337463109901, -60.62177826491083010, -5.000000000000000000 ) ) ;
#8386=CARTESIAN_POINT ( 'NONE',  ( 11.99999662536865763, -86.60254037844400443, -9.999999999999998224 ) ) ;
#8387=CIRCLE ( 'NONE', #35936, 2.000000000000001776 ) ;
#8389=ORIENTED_EDGE ( 'NONE', *, *, #15831, .T. ) ;
#8390=CARTESIAN_POINT ( 'NONE',  ( -2.374207310413330682E-13, -68.00000000000000000, 12.49999999999999822 ) ) ;
#8391=CIRCLE ( 'NONE', #23257, 2.000000000000001776 ) ;
#8392=FACE_OUTER_BOUND ( 'NONE', #28447, .T. ) ;
#8393=ORIENTED_EDGE ( 'NONE', *, *, #8262, .F. ) ;
#8394=CARTESIAN_POINT ( 'NONE',  ( 44.99999662536851019, 77.94228634059959404, -9.999999999999998224 ) ) ;
#8395=ORIENTED_EDGE ( 'NONE', *, *, #22037, .F. ) ;
#8396=FACE_BOUND ( 'NONE', #19664, .T. ) ;
#8397=CIRCLE ( 'NONE', #13178, 2.000000000000001776 ) ;
#8398=CARTESIAN_POINT ( 'NONE',  ( -47.00000337463111322, 60.62177826491077326, -9.999999999999998224 ) ) ;
#8399=EDGE_CURVE ( 'NONE', #33068, #12455, #644, .T. ) ;
#8400=AXIS2_PLACEMENT_3D ( 'NONE', #30106, #24868, #24304 ) ;
#8401=ORIENTED_EDGE ( 'NONE', *, *, #27109, .T. ) ;
#8404=CARTESIAN_POINT ( 'NONE',  ( -85.00000337463092137, -8.660254037844422825, 12.50000000000000000 ) ) ;
#8405=CARTESIAN_POINT ( 'NONE',  ( 44.99999662536851019, -60.62177826491080168, -9.999999999999998224 ) ) ;
#8406=DIRECTION ( 'NONE',  ( 0.000000000000000000, 0.000000000000000000, 1.000000000000000000 ) ) ;
#8408=CIRCLE ( 'NONE', #12586, 2.000000000000000000 ) ;
#8410=ADVANCED_FACE ( 'NONE', ( #18927 ), #13291, .F. ) ;
#8411=DIRECTION ( 'NONE',  ( 1.000000000000000000, 0.000000000000000000, 0.000000000000000000 ) ) ;
#8412=DIRECTION ( 'NONE',  ( 1.000000000000000000, 0.000000000000000000, 0.000000000000000000 ) ) ;
#8413=VERTEX_POINT ( 'NONE', #30356 ) ;
#8414=EDGE_CURVE ( 'NONE', #4196, #8015, #27599, .T. ) ;
#8415=ORIENTED_EDGE ( 'NONE', *, *, #1152, .T. ) ;
#8417=ORIENTED_EDGE ( 'NONE', *, *, #8868, .T. ) ;
#8418=DIRECTION ( 'NONE',  ( 1.000000000000000000, 0.000000000000000000, 0.000000000000000000 ) ) ;
#8419=DIRECTION ( 'NONE',  ( 1.000000000000000000, 0.000000000000000000, 0.000000000000000000 ) ) ;
#8420=CARTESIAN_POINT ( 'NONE',  ( -13.89091430021420237, -62.33939050065180254, 12.49999999999999822 ) ) ;
#8421=LINE ( 'NONE', #14219, #26550 ) ;
#8422=EDGE_CURVE ( 'NONE', #14720, #942, #33605, .T. ) ;
#8423=CARTESIAN_POINT ( 'NONE',  ( -85.00000337463092137, -25.98076211353322051, -5.000000000000000000 ) ) ;
#8425=CARTESIAN_POINT ( 'NONE',  ( 64.99999662536841072, 25.98076211353318854, 17.49999999999999645 ) ) ;
#8428=ORIENTED_EDGE ( 'NONE', *, *, #3506, .T. ) ;
#8430=CARTESIAN_POINT ( 'NONE',  ( 74.99999662536836809, -8.660254037844401509, -9.999999999999998224 ) ) ;
#8432=CARTESIAN_POINT ( 'NONE',  ( -82.00000337463094979, 17.32050807568878525, 17.49999999999999645 ) ) ;
#8435=ADVANCED_FACE ( 'NONE', ( #33565 ), #31101, .F. ) ;
#8436=FACE_BOUND ( 'NONE', #26342, .T. ) ;
#8438=VERTEX_POINT ( 'NONE', #14020 ) ;
#8439=EDGE_CURVE ( 'NONE', #31907, #28198, #12620, .T. ) ;
#8440=DIRECTION ( 'NONE',  ( -1.000000000000000000, 0.000000000000000000, 0.000000000000000000 ) ) ;
#8441=ORIENTED_EDGE ( 'NONE', *, *, #27036, .F. ) ;
#8442=CYLINDRICAL_SURFACE ( 'NONE', #2964, 2.000000000000001776 ) ;
#8443=DIRECTION ( 'NONE',  ( 1.000000000000000000, 0.000000000000000000, 0.000000000000000000 ) ) ;
#8445=VERTEX_POINT ( 'NONE', #21732 ) ;
#8446=ORIENTED_EDGE ( 'NONE', *, *, #18065, .T. ) ;
#8447=EDGE_CURVE ( 'NONE', #3051, #3447, #10846, .T. ) ;
#8448=EDGE_LOOP ( 'NONE', ( #16159, #37080, #15150, #23412 ) ) ;
#8449=VERTEX_POINT ( 'NONE', #24742 ) ;
#8450=ADVANCED_FACE ( 'NONE', ( #7682 ), #19133, .F. ) ;
#8451=EDGE_LOOP ( 'NONE', ( #1326, #18200, #15528, #11717 ) ) ;
#8452=CARTESIAN_POINT ( 'NONE',  ( -47.00000337463111322, 60.62177826491077326, -9.999999999999998224 ) ) ;
#8453=CARTESIAN_POINT ( 'NONE',  ( -75.00000337463097821, 25.98076211353318854, -9.999999999999998224 ) ) ;
#8454=DIRECTION ( 'NONE',  ( 0.000000000000000000, 0.000000000000000000, -1.000000000000000000 ) ) ;
#8455=DIRECTION ( 'NONE',  ( -1.000000000000000000, 0.000000000000000000, 0.000000000000000000 ) ) ;
#8457=ORIENTED_EDGE ( 'NONE', *, *, #9866, .F. ) ;
#8458=LINE ( 'NONE', #2467, #10537 ) ;
#8459=DIRECTION ( 'NONE',  ( 0.000000000000000000, 0.000000000000000000, 1.000000000000000000 ) ) ;
#8460=LINE ( 'NONE', #5835, #16445 ) ;
#8463=DIRECTION ( 'NONE',  ( -0.000000000000000000, 0.000000000000000000, -1.000000000000000000 ) ) ;
#8465=EDGE_LOOP ( 'NONE', ( #32277, #11285 ) ) ;
#8466=ADVANCED_FACE ( 'NONE', ( #25294 ), #2036, .F. ) ;
#8467=DIRECTION ( 'NONE',  ( 0.000000000000000000, 0.000000000000000000, 1.000000000000000000 ) ) ;
#8471=ORIENTED_EDGE ( 'NONE', *, *, #24185, .T. ) ;
#8472=ORIENTED_EDGE ( 'NONE', *, *, #19145, .F. ) ;
#8474=ADVANCED_FACE ( 'NONE', ( #10678 ), #22120, .F. ) ;
#8476=EDGE_LOOP ( 'NONE', ( #18313, #5350, #24397, #33592 ) ) ;
#8477=VECTOR ( 'NONE', #16564, 1000.000000000000000 ) ;
#8479=ADVANCED_FACE ( 'NONE', ( #11406 ), #25673, .F. ) ;
#8480=VECTOR ( 'NONE', #25307, 1000.000000000000000 ) ;
#8481=DIRECTION ( 'NONE',  ( 0.000000000000000000, 0.000000000000000000, 1.000000000000000000 ) ) ;
#8482=VERTEX_POINT ( 'NONE', #11219 ) ;
#8485=CARTESIAN_POINT ( 'NONE',  ( -45.00000337463111322, 60.62177826491077326, -9.999999999999998224 ) ) ;
#8486=DIRECTION ( 'NONE',  ( 1.000000000000000000, 0.000000000000000000, 0.000000000000000000 ) ) ;
#8487=ORIENTED_EDGE ( 'NONE', *, *, #3511, .T. ) ;
#8488=EDGE_LOOP ( 'NONE', ( #10278, #5573, #15998, #17044 ) ) ;
#8489=LINE ( 'NONE', #22753, #25116 ) ;
#8490=LINE ( 'NONE', #6402, #2912 ) ;
#8491=CARTESIAN_POINT ( 'NONE',  ( 84.88770958243756581, -10.65709945499362554, 12.50000000000000000 ) ) ;
#8492=DIRECTION ( 'NONE',  ( 0.000000000000000000, 0.000000000000000000, 1.000000000000000000 ) ) ;
#8493=EDGE_CURVE ( 'NONE', #22989, #3582, #16824, .T. ) ;
#8494=ORIENTED_EDGE ( 'NONE', *, *, #18044, .T. ) ;
#8495=FACE_OUTER_BOUND ( 'NONE', #19416, .T. ) ;
#8496=FACE_BOUND ( 'NONE', #29784, .T. ) ;
#8497=CARTESIAN_POINT ( 'NONE',  ( 64.99999662536841072, -25.98076211353320275, 12.50000000000000000 ) ) ;
#8498=DIRECTION ( 'NONE',  ( 0.000000000000000000, 0.000000000000000000, 1.000000000000000000 ) ) ;
#8500=CARTESIAN_POINT ( 'NONE',  ( 34.99999662536855283, -60.62177826491080168, 17.49999999999999645 ) ) ;
#8502=AXIS2_PLACEMENT_3D ( 'NONE', #8119, #19563, #36799 ) ;
#8503=DIRECTION ( 'NONE',  ( 0.000000000000000000, 0.000000000000000000, 1.000000000000000000 ) ) ;
#8504=ORIENTED_EDGE ( 'NONE', *, *, #18049, .T. ) ;
#8505=CARTESIAN_POINT ( 'NONE',  ( 56.99999662536844625, 43.30127018922198801, -5.000000000000000000 ) ) ;
#8506=DIRECTION ( 'NONE',  ( 0.000000000000000000, 0.000000000000000000, 1.000000000000000000 ) ) ;
#8507=LINE ( 'NONE', #25386, #29493 ) ;
#8508=ORIENTED_EDGE ( 'NONE', *, *, #31425, .T. ) ;
#8509=EDGE_LOOP ( 'NONE', ( #36451, #28937, #2269, #17596, #31311, #24321, #33282, #29857, #26100, #24984, #13129, #28209 ) ) ;
#8510=EDGE_CURVE ( 'NONE', #36669, #3287, #8776, .T. ) ;
#8511=VERTEX_POINT ( 'NONE', #2790 ) ;
#8513=CARTESIAN_POINT ( 'NONE',  ( -85.00000337463092137, -25.98076211353322051, 12.50000000000000000 ) ) ;
#8515=LINE ( 'NONE', #19946, #12410 ) ;
#8516=VERTEX_POINT ( 'NONE', #5787 ) ;
#8517=EDGE_CURVE ( 'NONE', #1626, #2314, #13819, .T. ) ;
#8518=CARTESIAN_POINT ( 'NONE',  ( -61.25926521283079751, 32.16008401677975570, 12.49999999999999645 ) ) ;
#8519=VERTEX_POINT ( 'NONE', #31983 ) ;
#8520=DIRECTION ( 'NONE',  ( 1.000000000000000000, 0.000000000000000000, 0.000000000000000000 ) ) ;
#8521=ORIENTED_EDGE ( 'NONE', *, *, #4463, .F. ) ;
#8522=ADVANCED_FACE ( 'NONE', ( #14216 ), #17762, .F. ) ;
#8523=CYLINDRICAL_SURFACE ( 'NONE', #15369, 2.000000000000001776 ) ;
#8524=ORIENTED_EDGE ( 'NONE', *, *, #32549, .T. ) ;
#8525=ADVANCED_FACE ( 'NONE', ( #37106 ), #14575, .F. ) ;
#8526=ORIENTED_EDGE ( 'NONE', *, *, #4360, .T. ) ;
#8527=CARTESIAN_POINT ( 'NONE',  ( 79.99999662536832545, -17.32050807568879591, -9.999999999999998224 ) ) ;
#8528=DIRECTION ( 'NONE',  ( 0.000000000000000000, 0.000000000000000000, -1.000000000000000000 ) ) ;
#8530=ORIENTED_EDGE ( 'NONE', *, *, #11671, .T. ) ;
#8531=CARTESIAN_POINT ( 'NONE',  ( 74.99999662536836809, -8.660254037844401509, -5.000000000000000000 ) ) ;
#8533=EDGE_CURVE ( 'NONE', #33319, #23244, #31187, .T. ) ;
#8535=EDGE_CURVE ( 'NONE', #13708, #36567, #6639, .T. ) ;
#8536=CARTESIAN_POINT ( 'NONE',  ( -72.00000337463100664, 17.32050807568877460, 12.50000000000000000 ) ) ;
#8538=ORIENTED_EDGE ( 'NONE', *, *, #18238, .T. ) ;
#8539=DIRECTION ( 'NONE',  ( 0.000000000000000000, 0.000000000000000000, 1.000000000000000000 ) ) ;
#8540=DIRECTION ( 'NONE',  ( 0.000000000000000000, 0.000000000000000000, 1.000000000000000000 ) ) ;
#8542=ORIENTED_EDGE ( 'NONE', *, *, #21202, .T. ) ;
#8544=DIRECTION ( 'NONE',  ( 1.000000000000000000, 0.000000000000000000, 0.000000000000000000 ) ) ;
#8545=CYLINDRICAL_SURFACE ( 'NONE', #10011, 2.000000000000001776 ) ;
#8546=CARTESIAN_POINT ( 'NONE',  ( -67.00000337463104927, -25.98076211353322051, -9.999999999999998224 ) ) ;
#8547=AXIS2_PLACEMENT_3D ( 'NONE', #28, #28162, #22174 ) ;
#8548=ORIENTED_EDGE ( 'NONE', *, *, #5759, .T. ) ;
#8549=ORIENTED_EDGE ( 'NONE', *, *, #25717, .F. ) ;
#8550=DIRECTION ( 'NONE',  ( 0.000000000000000000, 0.000000000000000000, 1.000000000000000000 ) ) ;
#8551=CARTESIAN_POINT ( 'NONE',  ( 64.99999662536839651, 60.62177826491078747, -9.999999999999998224 ) ) ;
#8552=ORIENTED_EDGE ( 'NONE', *, *, #7592, .F. ) ;
#8553=EDGE_LOOP ( 'NONE', ( #14654, #28193 ) ) ;
#8555=CARTESIAN_POINT ( 'NONE',  ( -20.00000337463122690, 86.60254037844397601, 12.50000000000000000 ) ) ;
#8556=AXIS2_PLACEMENT_3D ( 'NONE', #5142, #30462, #33825 ) ;
#8557=LINE ( 'NONE', #19991, #29621 ) ;
#8558=EDGE_CURVE ( 'NONE', #25301, #12879, #668, .T. ) ;
#8559=ORIENTED_EDGE ( 'NONE', *, *, #35027, .F. ) ;
#8560=ORIENTED_EDGE ( 'NONE', *, *, #18598, .F. ) ;
#8561=FACE_OUTER_BOUND ( 'NONE', #34382, .T. ) ;
#8562=DIRECTION ( 'NONE',  ( -1.000000000000000000, 0.000000000000000000, 0.000000000000000000 ) ) ;
#8563=ORIENTED_EDGE ( 'NONE', *, *, #13251, .T. ) ;
#8564=DIRECTION ( 'NONE',  ( -0.5000000000000101030, -0.8660254037844328234, 0.000000000000000000 ) ) ;
#8565=ORIENTED_EDGE ( 'NONE', *, *, #32059, .T. ) ;
#8566=FACE_BOUND ( 'NONE', #20135, .T. ) ;
#8567=CIRCLE ( 'NONE', #18141, 2.000000000000001776 ) ;
#8570=ORIENTED_EDGE ( 'NONE', *, *, #36220, .T. ) ;
#8573=VECTOR ( 'NONE', #5425, 1000.000000000000000 ) ;
#8574=DIRECTION ( 'NONE',  ( 0.000000000000000000, 0.000000000000000000, 1.000000000000000000 ) ) ;
#8575=DIRECTION ( 'NONE',  ( 0.000000000000000000, 0.000000000000000000, -1.000000000000000000 ) ) ;
#8576=ADVANCED_FACE ( 'NONE', ( #23215, #20217, #14767, #6142, #34116, #5976, #523 ), #17407, .F. ) ;
#8577=ORIENTED_EDGE ( 'NONE', *, *, #29139, .F. ) ;
#8578=CARTESIAN_POINT ( 'NONE',  ( -58.88972745734155723, 34.00000000000049027, 12.49999999999999822 ) ) ;
#8579=CARTESIAN_POINT ( 'NONE',  ( -43.19957991610399972, -47.04203867989563292, 12.49999999999999822 ) ) ;
#8581=ORIENTED_EDGE ( 'NONE', *, *, #23047, .F. ) ;
#8582=ORIENTED_EDGE ( 'NONE', *, *, #36845, .T. ) ;
#8583=VERTEX_POINT ( 'NONE', #11950 ) ;
#8584=AXIS2_PLACEMENT_3D ( 'NONE', #26124, #11330, #22782 ) ;
#8585=AXIS2_PLACEMENT_3D ( 'NONE', #31820, #20572, #20232 ) ;
#8587=DIRECTION ( 'NONE',  ( -0.8660254037844453689, -0.4999999999999882871, 0.000000000000000000 ) ) ;
#8590=DIRECTION ( 'NONE',  ( 1.000000000000000000, 0.000000000000000000, 0.000000000000000000 ) ) ;
#8592=CARTESIAN_POINT ( 'NONE',  ( 69.61830985333858735, 36.60425714729669977, -5.000000000000000000 ) ) ;
#8593=ADVANCED_FACE ( 'NONE', ( #15521 ), #32757, .F. ) ;
#8594=VERTEX_POINT ( 'NONE', #15698 ) ;
#8597=VECTOR ( 'NONE', #25216, 1000.000000000000000 ) ;
#8598=FACE_OUTER_BOUND ( 'NONE', #18952, .T. ) ;
#8599=DIRECTION ( 'NONE',  ( 0.000000000000000000, 0.000000000000000000, -1.000000000000000000 ) ) ;
#8600=CARTESIAN_POINT ( 'NONE',  ( 51.13139720814399425, -27.50000000000022737, -10.00000000000000000 ) ) ;
#8601=ORIENTED_EDGE ( 'NONE', *, *, #31624, .T. ) ;
#8602=AXIS2_PLACEMENT_3D ( 'NONE', #8380, #28408, #34424 ) ;
#8603=EDGE_CURVE ( 'NONE', #5113, #9816, #12020, .T. ) ;
#8604=FACE_BOUND ( 'NONE', #15764, .T. ) ;
#8606=VERTEX_POINT ( 'NONE', #10079 ) ;
#8610=AXIS2_PLACEMENT_3D ( 'NONE', #29753, #18528, #26766 ) ;
#8611=CARTESIAN_POINT ( 'NONE',  ( 19.99999662536858835, 69.28203230275516944, -9.999999999999998224 ) ) ;
#8612=CARTESIAN_POINT ( 'NONE',  ( -72.28378166042018904, -61.53067111003240797, -4.999999999999997335 ) ) ;
#8614=VERTEX_POINT ( 'NONE', #35768 ) ;
#8615=ORIENTED_EDGE ( 'NONE', *, *, #22699, .F. ) ;
#8616=ORIENTED_EDGE ( 'NONE', *, *, #9854, .F. ) ;
#8617=AXIS2_PLACEMENT_3D ( 'NONE', #31711, #396, #26639 ) ;
#8618=ORIENTED_EDGE ( 'NONE', *, *, #29451, .F. ) ;
#8619=ORIENTED_EDGE ( 'NONE', *, *, #25633, .F. ) ;
#8620=DIRECTION ( 'NONE',  ( 0.000000000000000000, 0.000000000000000000, 1.000000000000000000 ) ) ;
#8622=CARTESIAN_POINT ( 'NONE',  ( -33.99999999999945288, 58.88972745734214698, -49.86561046011506448 ) ) ;
#8623=LINE ( 'NONE', #23441, #6499 ) ;
#8624=DIRECTION ( 'NONE',  ( -1.000000000000000000, 0.000000000000000000, 0.000000000000000000 ) ) ;
#8626=VERTEX_POINT ( 'NONE', #15318 ) ;
#8627=CYLINDRICAL_SURFACE ( 'NONE', #4550, 2.000000000000001776 ) ;
#8628=DIRECTION ( 'NONE',  ( 1.000000000000000000, 0.000000000000000000, 0.000000000000000000 ) ) ;
#8629=EDGE_CURVE ( 'NONE', #9668, #26406, #7260, .T. ) ;
#8631=ORIENTED_EDGE ( 'NONE', *, *, #20204, .F. ) ;
#8632=LINE ( 'NONE', #2843, #19672 ) ;
#8634=VERTEX_POINT ( 'NONE', #24320 ) ;
#8635=CIRCLE ( 'NONE', #846, 3.000000000000003997 ) ;
#8636=ORIENTED_EDGE ( 'NONE', *, *, #683, .F. ) ;
#8637=CARTESIAN_POINT ( 'NONE',  ( -55.00000337463110611, -43.30127018922202353, -9.999999999999998224 ) ) ;
#8638=DIRECTION ( 'NONE',  ( 0.000000000000000000, 0.000000000000000000, 1.000000000000000000 ) ) ;
#8641=EDGE_CURVE ( 'NONE', #23192, #20237, #21279, .T. ) ;
#8643=EDGE_LOOP ( 'NONE', ( #12348, #18447, #22807, #26446 ) ) ;
#8644=AXIS2_PLACEMENT_3D ( 'NONE', #34861, #8990, #3905 ) ;
#8646=CYLINDRICAL_SURFACE ( 'NONE', #16513, 1.999999999999998224 ) ;
#8649=EDGE_CURVE ( 'NONE', #32403, #35238, #27858, .T. ) ;
#8650=AXIS2_PLACEMENT_3D ( 'NONE', #6741, #9570, #9372 ) ;
#8651=EDGE_LOOP ( 'NONE', ( #23370, #35292, #35083, #9376 ) ) ;
#8653=EDGE_LOOP ( 'NONE', ( #35010, #19933 ) ) ;
#8655=DIRECTION ( 'NONE',  ( 0.000000000000000000, 0.000000000000000000, 1.000000000000000000 ) ) ;
#8656=CIRCLE ( 'NONE', #6949, 3.000000000000002665 ) ;
#8657=DIRECTION ( 'NONE',  ( 0.000000000000000000, 0.000000000000000000, 1.000000000000000000 ) ) ;
#8659=AXIS2_PLACEMENT_3D ( 'NONE', #29417, #16619, #25419 ) ;
#8660=ORIENTED_EDGE ( 'NONE', *, *, #17205, .F. ) ;
#8661=DIRECTION ( 'NONE',  ( 0.000000000000000000, 0.000000000000000000, 1.000000000000000000 ) ) ;
#8662=DIRECTION ( 'NONE',  ( 1.000000000000000000, 0.000000000000000000, 0.000000000000000000 ) ) ;
#8666=FACE_OUTER_BOUND ( 'NONE', #1444, .T. ) ;
#8667=FACE_BOUND ( 'NONE', #17430, .T. ) ;
#8668=LINE ( 'NONE', #6221, #3449 ) ;
#8670=CARTESIAN_POINT ( 'NONE',  ( -7.000003374631269537, -77.94228634059960825, 12.50000000000000000 ) ) ;
#8672=EDGE_CURVE ( 'NONE', #21445, #15730, #19496, .T. ) ;
#8673=VECTOR ( 'NONE', #1200, 1000.000000000000000 ) ;
#8677=DIRECTION ( 'NONE',  ( 1.000000000000000000, 0.000000000000000000, 0.000000000000000000 ) ) ;
#8679=LINE ( 'NONE', #31196, #30368 ) ;
#8680=DIRECTION ( 'NONE',  ( 1.000000000000000000, 0.000000000000000000, 0.000000000000000000 ) ) ;
#8681=CARTESIAN_POINT ( 'NONE',  ( 84.99999662536831124, -25.98076211353319565, -5.000000000000000000 ) ) ;
#8682=ORIENTED_EDGE ( 'NONE', *, *, #3052, .T. ) ;
#8683=VERTEX_POINT ( 'NONE', #35224 ) ;
#8684=ORIENTED_EDGE ( 'NONE', *, *, #2824, .T. ) ;
#8685=CIRCLE ( 'NONE', #30812, 2.000000000000001776 ) ;
#8686=CARTESIAN_POINT ( 'NONE',  ( -58.00000337463104216, 51.96152422706639129, 12.50000000000000000 ) ) ;
#8687=DIRECTION ( 'NONE',  ( 1.000000000000000000, 0.000000000000000000, 0.000000000000000000 ) ) ;
#8688=CIRCLE ( 'NONE', #26645, 2.000000000000000000 ) ;
#8689=CARTESIAN_POINT ( 'NONE',  ( 49.99999662536848177, -51.96152422706640550, -5.000000000000000000 ) ) ;
#8690=ORIENTED_EDGE ( 'NONE', *, *, #24013, .T. ) ;
#8691=CIRCLE ( 'NONE', #23060, 2.000000000000001776 ) ;
#8694=EDGE_CURVE ( 'NONE', #5072, #5817, #32648, .T. ) ;
#8695=ORIENTED_EDGE ( 'NONE', *, *, #23248, .T. ) ;
#8696=CYLINDRICAL_SURFACE ( 'NONE', #4805, 2.000000000000001776 ) ;
#8698=FACE_OUTER_BOUND ( 'NONE', #29792, .T. ) ;
#8699=ORIENTED_EDGE ( 'NONE', *, *, #16938, .F. ) ;
#8701=ORIENTED_EDGE ( 'NONE', *, *, #107, .F. ) ;
#8703=CARTESIAN_POINT ( 'NONE',  ( -23.00000337463120559, 77.94228634059957983, -9.999999999999998224 ) ) ;
#8704=CARTESIAN_POINT ( 'NONE',  ( 16.99999662536863454, -77.94228634059960825, 12.50000000000000000 ) ) ;
#8705=APPLICATION_CONTEXT ( 'automotive_design' ) ;
#8706=VERTEX_POINT ( 'NONE', #32389 ) ;
#8707=DIRECTION ( 'NONE',  ( 0.000000000000000000, 0.000000000000000000, 1.000000000000000000 ) ) ;
#8709=DIRECTION ( 'NONE',  ( 0.000000000000000000, 0.000000000000000000, -1.000000000000000000 ) ) ;
#8710=ADVANCED_FACE ( 'NONE', ( #18525 ), #700, .F. ) ;
#8711=CIRCLE ( 'NONE', #12270, 65.00000000000000000 ) ;
#8712=ORIENTED_EDGE ( 'NONE', *, *, #19270, .F. ) ;
#8713=CARTESIAN_POINT ( 'NONE',  ( -70.00000337463100664, -17.32050807568882078, -9.999999999999998224 ) ) ;
#8716=EDGE_CURVE ( 'NONE', #5893, #12977, #8120, .T. ) ;
#8718=DIRECTION ( 'NONE',  ( 0.000000000000000000, 0.000000000000000000, 1.000000000000000000 ) ) ;
#8719=DIRECTION ( 'NONE',  ( 1.000000000000000000, 0.000000000000000000, 0.000000000000000000 ) ) ;
#8720=AXIS2_PLACEMENT_3D ( 'NONE', #33434, #36785, #24998 ) ;
#8721=AXIS2_PLACEMENT_3D ( 'NONE', #1045, #21485, #15106 ) ;
#8723=EDGE_CURVE ( 'NONE', #30459, #17896, #6701, .T. ) ;
#8724=CIRCLE ( 'NONE', #11709, 2.999999999999999556 ) ;
#8725=VERTEX_POINT ( 'NONE', #12505 ) ;
#8727=FACE_OUTER_BOUND ( 'NONE', #35035, .T. ) ;
#8728=DIRECTION ( 'NONE',  ( 1.000000000000000000, 0.000000000000000000, 0.000000000000000000 ) ) ;
#8729=EDGE_CURVE ( 'NONE', #1857, #24169, #5740, .T. ) ;
#8731=AXIS2_PLACEMENT_3D ( 'NONE', #19433, #27508, #1824 ) ;
#8733=ORIENTED_EDGE ( 'NONE', *, *, #34747, .F. ) ;
#8735=CARTESIAN_POINT ( 'NONE',  ( -62.97617850287781494, -4.279621169095772615, -4.999999999999997335 ) ) ;
#8736=CARTESIAN_POINT ( 'NONE',  ( -95.00000000000001421, 1.163414459189985801E-14, -10.00000000000000000 ) ) ;
#8738=AXIS2_PLACEMENT_3D ( 'NONE', #27626, #1379, #35705 ) ;
#8740=EDGE_CURVE ( 'NONE', #10971, #15901, #11104, .T. ) ;
#8741=AXIS2_PLACEMENT_3D ( 'NONE', #4395, #27804, #30453 ) ;
#8742=DIRECTION ( 'NONE',  ( 1.000000000000000000, 0.000000000000000000, 0.000000000000000000 ) ) ;
#8743=ORIENTED_EDGE ( 'NONE', *, *, #11274, .T. ) ;
#8744=EDGE_CURVE ( 'NONE', #8936, #24850, #10258, .T. ) ;
#8745=EDGE_CURVE ( 'NONE', #19466, #5465, #3935, .T. ) ;
#8747=DIRECTION ( 'NONE',  ( 1.000000000000000000, 0.000000000000000000, 0.000000000000000000 ) ) ;
#8749=( GEOMETRIC_REPRESENTATION_CONTEXT ( 3 ) GLOBAL_UNCERTAINTY_ASSIGNED_CONTEXT ( ( #5443 ) ) GLOBAL_UNIT_ASSIGNED_CONTEXT ( ( #4517, #27389, #35348 ) ) REPRESENTATION_CONTEXT ( 'NONE', 'WORKASPACE' ) );
#8750=CARTESIAN_POINT ( 'NONE',  ( 0.000000000000000000, 0.000000000000000000, -5.000000000000000000 ) ) ;
#8752=AXIS2_PLACEMENT_3D ( 'NONE', #34532, #6037, #20824 ) ;
#8753=AXIS2_PLACEMENT_3D ( 'NONE', #10582, #27462, #33078 ) ;
#8754=CIRCLE ( 'NONE', #25541, 2.000000000000001776 ) ;
#8756=DIRECTION ( 'NONE',  ( 0.8660254037844415942, 0.4999999999999949485, 0.000000000000000000 ) ) ;
#8758=CIRCLE ( 'NONE', #33898, 2.000000000000001776 ) ;
#8763=DIRECTION ( 'NONE',  ( 0.000000000000000000, 0.000000000000000000, 1.000000000000000000 ) ) ;
#8765=CARTESIAN_POINT ( 'NONE',  ( 34.99999662536855283, -60.62177826491080168, -9.999999999999998224 ) ) ;
#8767=ORIENTED_EDGE ( 'NONE', *, *, #26741, .T. ) ;
#8768=ORIENTED_EDGE ( 'NONE', *, *, #16334, .T. ) ;
#8772=AXIS2_PLACEMENT_3D ( 'NONE', #25581, #22781, #7957 ) ;
#8774=AXIS2_PLACEMENT_3D ( 'NONE', #5386, #28238, #2555 ) ;
#8775=AXIS2_PLACEMENT_3D ( 'NONE', #32471, #15984, #27033 ) ;
#8776=LINE ( 'NONE', #36908, #26393 ) ;
#8777=AXIS2_PLACEMENT_3D ( 'NONE', #4825, #31048, #36510 ) ;
#8778=CARTESIAN_POINT ( 'NONE',  ( -47.00000337463111322, 60.62177826491077326, 17.49999999999999645 ) ) ;
#8780=CYLINDRICAL_SURFACE ( 'NONE', #12397, 65.00000000000000000 ) ;
#8781=CARTESIAN_POINT ( 'NONE',  ( 6.808388610744110674E-13, 65.00000000000000000, 12.49999999999999822 ) ) ;
#8782=EDGE_LOOP ( 'NONE', ( #24762, #34870, #15490, #31347 ) ) ;
#8783=CIRCLE ( 'NONE', #32708, 2.000000000000001776 ) ;
#8784=VERTEX_POINT ( 'NONE', #10632 ) ;
#8786=CARTESIAN_POINT ( 'NONE',  ( -70.00000337463100664, -17.32050807568882078, -9.999999999999998224 ) ) ;
#8787=EDGE_CURVE ( 'NONE', #27221, #14606, #27308, .T. ) ;
#8788=DIRECTION ( 'NONE',  ( -1.000000000000000000, 0.000000000000000000, 0.000000000000000000 ) ) ;
#8789=VERTEX_POINT ( 'NONE', #36518 ) ;
#8791=CIRCLE ( 'NONE', #29742, 2.000000000000001776 ) ;
#8792=DIRECTION ( 'NONE',  ( 0.000000000000000000, 0.000000000000000000, 1.000000000000000000 ) ) ;
#8793=ORIENTED_EDGE ( 'NONE', *, *, #33830, .F. ) ;
#8794=VERTEX_POINT ( 'NONE', #30675 ) ;
#8795=DIRECTION ( 'NONE',  ( 0.000000000000000000, 0.000000000000000000, 1.000000000000000000 ) ) ;
#8796=EDGE_LOOP ( 'NONE', ( #9766, #35220, #26287, #16667, #25042 ) ) ;
#8799=VECTOR ( 'NONE', #9931, 1000.000000000000000 ) ;
#8801=CIRCLE ( 'NONE', #10010, 2.000000000000001776 ) ;
#8802=CIRCLE ( 'NONE', #15394, 2.000000000000001776 ) ;
#8806=ORIENTED_EDGE ( 'NONE', *, *, #1069, .F. ) ;
#8808=VECTOR ( 'NONE', #31172, 1000.000000000000000 ) ;
#8810=ORIENTED_EDGE ( 'NONE', *, *, #7377, .F. ) ;
#8811=CARTESIAN_POINT ( 'NONE',  ( 0.000000000000000000, 0.000000000000000000, -5.000000000000000000 ) ) ;
#8812=DIRECTION ( 'NONE',  ( 1.000000000000000000, 0.000000000000000000, 0.000000000000000000 ) ) ;
#8813=CYLINDRICAL_SURFACE ( 'NONE', #3504, 2.000000000000001776 ) ;
#8816=ORIENTED_EDGE ( 'NONE', *, *, #9959, .F. ) ;
#8817=DIRECTION ( 'NONE',  ( 0.000000000000000000, -0.000000000000000000, -1.000000000000000000 ) ) ;
#8818=AXIS2_PLACEMENT_3D ( 'NONE', #12584, #35482, #21204 ) ;
#8819=EDGE_CURVE ( 'NONE', #6561, #19630, #24882, .T. ) ;
#8821=CIRCLE ( 'NONE', #21997, 2.000000000000001776 ) ;
#8823=ORIENTED_EDGE ( 'NONE', *, *, #851, .F. ) ;
#8825=LINE ( 'NONE', #20438, #17188 ) ;
#8826=ORIENTED_EDGE ( 'NONE', *, *, #20513, .T. ) ;
#8827=ORIENTED_EDGE ( 'NONE', *, *, #30070, .F. ) ;
#8828=AXIS2_PLACEMENT_3D ( 'NONE', #5533, #8358, #16799 ) ;
#8829=DIRECTION ( 'NONE',  ( 0.000000000000000000, 0.000000000000000000, 1.000000000000000000 ) ) ;
#8830=CARTESIAN_POINT ( 'NONE',  ( -82.00000337463094979, -17.32050807568882078, -5.000000000000000000 ) ) ;
#8831=EDGE_CURVE ( 'NONE', #9651, #20361, #21901, .T. ) ;
#8833=CARTESIAN_POINT ( 'NONE',  ( 21.99999662536862033, -86.60254037844400443, -9.999999999999998224 ) ) ;
#8834=ORIENTED_EDGE ( 'NONE', *, *, #32258, .T. ) ;
#8835=CIRCLE ( 'NONE', #17226, 2.000000000000001776 ) ;
#8836=CARTESIAN_POINT ( 'NONE',  ( -86.45172111230354517, 31.46585318596159553, -49.86348611802629449 ) ) ;
#8837=LINE ( 'NONE', #23279, #22535 ) ;
#8838=CARTESIAN_POINT ( 'NONE',  ( -26.97173872511423198, 77.60723454213314199, 12.50000000000000000 ) ) ;
#8839=AXIS2_PLACEMENT_3D ( 'NONE', #28566, #14333, #20131 ) ;
#8840=VERTEX_POINT ( 'NONE', #7635 ) ;
#8841=AXIS2_PLACEMENT_3D ( 'NONE', #8927, #286, #34258 ) ;
#8842=AXIS2_PLACEMENT_3D ( 'NONE', #27198, #12390, #20847 ) ;
#8844=ORIENTED_EDGE ( 'NONE', *, *, #13415, .F. ) ;
#8845=VERTEX_POINT ( 'NONE', #4642 ) ;
#8847=CIRCLE ( 'NONE', #14232, 2.000000000000001776 ) ;
#8848=EDGE_CURVE ( 'NONE', #15428, #16100, #32038, .T. ) ;
#8850=ORIENTED_EDGE ( 'NONE', *, *, #16174, .T. ) ;
#8851=VERTEX_POINT ( 'NONE', #13624 ) ;
#8852=CARTESIAN_POINT ( 'NONE',  ( 64.99999662536839651, 60.62177826491078747, -9.999999999999998224 ) ) ;
#8853=EDGE_CURVE ( 'NONE', #20458, #36216, #33279, .T. ) ;
#8854=CARTESIAN_POINT ( 'NONE',  ( -52.39915983220772233, -35.19434990244957362, -4.999999999999997335 ) ) ;
#8856=AXIS2_PLACEMENT_3D ( 'NONE', #24582, #9932, #10303 ) ;
#8857=ORIENTED_EDGE ( 'NONE', *, *, #20630, .T. ) ;
#8858=LINE ( 'NONE', #11647, #6971 ) ;
#8859=FACE_BOUND ( 'NONE', #9630, .T. ) ;
#8860=EDGE_CURVE ( 'NONE', #3561, #18462, #313, .T. ) ;
#8861=FACE_OUTER_BOUND ( 'NONE', #28606, .T. ) ;
#8864=CARTESIAN_POINT ( 'NONE',  ( 0.000000000000000000, 0.000000000000000000, -5.000000000000000000 ) ) ;
#8865=DIRECTION ( 'NONE',  ( 0.000000000000000000, 0.000000000000000000, 1.000000000000000000 ) ) ;
#8866=PRODUCT ( 'ventilated rotor', 'ventilated rotor', '', ( #30293 ) ) ;
#8867=DIRECTION ( 'NONE',  ( -0.5000000000000101030, -0.8660254037844328234, 0.000000000000000000 ) ) ;
#8868=EDGE_CURVE ( 'NONE', #27851, #16300, #30853, .T. ) ;
#8869=AXIS2_PLACEMENT_3D ( 'NONE', #33018, #36032, #30388 ) ;
#8871=EDGE_LOOP ( 'NONE', ( #27816, #22008, #34634, #25872 ) ) ;
#8872=CARTESIAN_POINT ( 'NONE',  ( 53.72396900529356145, 62.16182810592437846, 12.50000000000000000 ) ) ;
#8873=VECTOR ( 'NONE', #31022, 1000.000000000000000 ) ;
#8874=CIRCLE ( 'NONE', #29828, 95.00000000000001421 ) ;
#8875=DIRECTION ( 'NONE',  ( 1.000000000000000000, 0.000000000000000000, 0.000000000000000000 ) ) ;
#8876=CARTESIAN_POINT ( 'NONE',  ( -65.00000337463102085, 43.30127018922198801, 12.50000000000000000 ) ) ;
#8877=ORIENTED_EDGE ( 'NONE', *, *, #30157, .T. ) ;
#8878=EDGE_LOOP ( 'NONE', ( #177, #26588 ) ) ;
#8879=EDGE_LOOP ( 'NONE', ( #2520, #12254, #19740, #17577, #9139, #17055 ) ) ;
#8881=DIRECTION ( 'NONE',  ( -1.000000000000000000, 0.000000000000000000, 0.000000000000000000 ) ) ;
#8884=ORIENTED_EDGE ( 'NONE', *, *, #14252, .T. ) ;
#8885=CIRCLE ( 'NONE', #29245, 2.000000000000001776 ) ;
#8886=CARTESIAN_POINT ( 'NONE',  ( 15.97563234535730814, -90.60231327712320137, 12.49999999999999822 ) ) ;
#8887=EDGE_CURVE ( 'NONE', #6244, #18009, #27678, .T. ) ;
#8891=DIRECTION ( 'NONE',  ( 1.000000000000000000, 0.000000000000000000, 0.000000000000000000 ) ) ;
#8892=AXIS2_PLACEMENT_3D ( 'NONE', #33553, #3605, #35991 ) ;
#8893=VERTEX_POINT ( 'NONE', #16431 ) ;
#8894=VERTEX_POINT ( 'NONE', #27859 ) ;
#8895=ADVANCED_FACE ( 'NONE', ( #2182 ), #31865, .F. ) ;
#8896=CARTESIAN_POINT ( 'NONE',  ( 0.000000000000000000, 0.000000000000000000, 0.000000000000000000 ) ) ;
#8898=CIRCLE ( 'NONE', #6494, 2.000000000000000000 ) ;
#8899=ADVANCED_FACE ( 'NONE', ( #28716 ), #29765, .F. ) ;
#8900=DIRECTION ( 'NONE',  ( 0.000000000000000000, 0.000000000000000000, 1.000000000000000000 ) ) ;
#8901=ORIENTED_EDGE ( 'NONE', *, *, #10042, .T. ) ;
#8902=LINE ( 'NONE', #32324, #11312 ) ;
#8903=DIRECTION ( 'NONE',  ( -0.8660254037844449249, -0.4999999999999888423, 0.000000000000000000 ) ) ;
#8904=DIRECTION ( 'NONE',  ( 0.000000000000000000, 0.000000000000000000, 1.000000000000000000 ) ) ;
#8905=AXIS2_PLACEMENT_3D ( 'NONE', #10133, #32610, #32813 ) ;
#8906=ORIENTED_EDGE ( 'NONE', *, *, #29451, .T. ) ;
#8907=DIRECTION ( 'NONE',  ( 0.000000000000000000, -0.000000000000000000, -1.000000000000000000 ) ) ;
#8909=AXIS2_PLACEMENT_3D ( 'NONE', #36287, #31025, #7791 ) ;
#8910=VERTEX_POINT ( 'NONE', #28879 ) ;
#8912=DIRECTION ( 'NONE',  ( 0.000000000000000000, 0.000000000000000000, 1.000000000000000000 ) ) ;
#8914=AXIS2_PLACEMENT_3D ( 'NONE', #2048, #27924, #2249 ) ;
#8916=AXIS2_PLACEMENT_3D ( 'NONE', #20841, #21026, #18202 ) ;
#8917=CARTESIAN_POINT ( 'NONE',  ( 37.99999662536853151, -69.28203230275519786, 17.49999999999999645 ) ) ;
#8918=EDGE_CURVE ( 'NONE', #23562, #4442, #4101, .T. ) ;
#8921=CARTESIAN_POINT ( 'NONE',  ( 24.99999662536859546, -77.94228634059960825, -5.000000000000000000 ) ) ;
#8922=ORIENTED_EDGE ( 'NONE', *, *, #21943, .T. ) ;
#8923=ORIENTED_EDGE ( 'NONE', *, *, #29972, .F. ) ;
#8925=AXIS2_PLACEMENT_3D ( 'NONE', #15347, #12328, #30340 ) ;
#8926=CARTESIAN_POINT ( 'NONE',  ( -58.88972745734155723, 34.00000000000049027, 12.49999999999999822 ) ) ;
#8927=CARTESIAN_POINT ( 'NONE',  ( 59.99999662536842493, 51.96152422706639129, -9.999999999999998224 ) ) ;
#8928=VECTOR ( 'NONE', #16921, 1000.000000000000000 ) ;
#8929=CARTESIAN_POINT ( 'NONE',  ( -65.00000337463102085, 43.30127018922198801, 17.49999999999999645 ) ) ;
#8931=DIRECTION ( 'NONE',  ( -0.000000000000000000, -0.000000000000000000, 1.000000000000000000 ) ) ;
#8932=VERTEX_POINT ( 'NONE', #12001 ) ;
#8933=CIRCLE ( 'NONE', #549, 33.00000000000001421 ) ;
#8934=EDGE_CURVE ( 'NONE', #14791, #16685, #18282, .T. ) ;
#8935=CARTESIAN_POINT ( 'NONE',  ( 39.99999662536853151, 69.28203230275518365, 12.50000000000000000 ) ) ;
#8936=VERTEX_POINT ( 'NONE', #23459 ) ;
#8937=FACE_BOUND ( 'NONE', #12914, .T. ) ;
#8938=AXIS2_PLACEMENT_3D ( 'NONE', #25272, #11188, #2573 ) ;
#8939=ADVANCED_FACE ( 'NONE', ( #18339 ), #25736, .F. ) ;
#8940=AXIS2_PLACEMENT_3D ( 'NONE', #4852, #32969, #27697 ) ;
#8941=DIRECTION ( 'NONE',  ( 0.000000000000000000, 0.000000000000000000, 1.000000000000000000 ) ) ;
#8942=ADVANCED_FACE ( 'NONE', ( #195 ), #5650, .F. ) ;
#8943=CARTESIAN_POINT ( 'NONE',  ( -50.00000337463112032, -51.96152422706641971, 17.49999999999999645 ) ) ;
#8944=AXIS2_PLACEMENT_3D ( 'NONE', #20352, #31772, #6101 ) ;
#8947=CYLINDRICAL_SURFACE ( 'NONE', #288, 2.000000000000001776 ) ;
#8948=CIRCLE ( 'NONE', #28700, 2.000000000000001776 ) ;
#8949=CIRCLE ( 'NONE', #22749, 2.000000000000001776 ) ;
#8951=CARTESIAN_POINT ( 'NONE',  ( -11.64413683707582337, -85.46375806488710225, 12.50000000000000000 ) ) ;
#8952=ORIENTED_EDGE ( 'NONE', *, *, #22400, .F. ) ;
#8955=CARTESIAN_POINT ( 'NONE',  ( 79.99999662536833966, 17.32050807568879236, -9.999999999999998224 ) ) ;
#8956=DIRECTION ( 'NONE',  ( -1.000000000000000000, 0.000000000000000000, 0.000000000000000000 ) ) ;
#8959=EDGE_LOOP ( 'NONE', ( #32351, #5010 ) ) ;
#8960=ORIENTED_EDGE ( 'NONE', *, *, #11879, .F. ) ;
#8961=ADVANCED_FACE ( 'NONE', ( #28522 ), #23278, .T. ) ;
#8963=CARTESIAN_POINT ( 'NONE',  ( 84.99999662536832545, 25.98076211353319565, -9.999999999999998224 ) ) ;
#8964=CIRCLE ( 'NONE', #15552, 2.000000000000001776 ) ;
#8965=CARTESIAN_POINT ( 'NONE',  ( 0.000000000000000000, 0.000000000000000000, 12.49999999999999822 ) ) ;
#8966=AXIS2_PLACEMENT_3D ( 'NONE', #25603, #19960, #37040 ) ;
#8967=AXIS2_PLACEMENT_3D ( 'NONE', #24421, #35862, #1344 ) ;
#8968=DIRECTION ( 'NONE',  ( 0.000000000000000000, 0.000000000000000000, 1.000000000000000000 ) ) ;
#8969=CARTESIAN_POINT ( 'NONE',  ( -86.45172111230354517, 31.46585318596159553, 12.49999999999999822 ) ) ;
#8971=CIRCLE ( 'NONE', #27558, 3.000000000000002665 ) ;
#8972=CARTESIAN_POINT ( 'NONE',  ( -65.00000337463102085, 60.62177826491077326, -9.999999999999998224 ) ) ;
#8973=ORIENTED_EDGE ( 'NONE', *, *, #28616, .F. ) ;
#8974=VERTEX_POINT ( 'NONE', #32045 ) ;
#8975=DIRECTION ( 'NONE',  ( 0.000000000000000000, 0.000000000000000000, -1.000000000000000000 ) ) ;
#8976=EDGE_CURVE ( 'NONE', #23027, #29875, #16526, .T. ) ;
#8977=AXIS2_PLACEMENT_3D ( 'NONE', #26514, #9260, #17902 ) ;
#8979=ADVANCED_FACE ( 'NONE', ( #26274 ), #9024, .F. ) ;
#8981=VERTEX_POINT ( 'NONE', #22905 ) ;
#8982=CIRCLE ( 'NONE', #8400, 2.000000000000001776 ) ;
#8983=CARTESIAN_POINT ( 'NONE',  ( 67.99999662536838230, 34.64101615137758472, 17.49999999999999645 ) ) ;
#8985=EDGE_LOOP ( 'NONE', ( #24021, #564 ) ) ;
#8986=EDGE_CURVE ( 'NONE', #27172, #7448, #20082, .T. ) ;
#8987=CARTESIAN_POINT ( 'NONE',  ( -17.00000337463126243, 77.94228634059957983, 12.50000000000000000 ) ) ;
#8989=AXIS2_PLACEMENT_3D ( 'NONE', #16149, #10499, #30575 ) ;
#8990=DIRECTION ( 'NONE',  ( 0.000000000000000000, 0.000000000000000000, 1.000000000000000000 ) ) ;
#8991=FACE_BOUND ( 'NONE', #27129, .T. ) ;
#8992=VECTOR ( 'NONE', #28863, 1000.000000000000000 ) ;
#8993=EDGE_LOOP ( 'NONE', ( #13235, #35587 ) ) ;
#8995=CIRCLE ( 'NONE', #21592, 2.000000000000001776 ) ;
#8996=ADVANCED_FACE ( 'NONE', ( #11626 ), #34531, .T. ) ;
#8997=VERTEX_POINT ( 'NONE', #5013 ) ;
#8998=EDGE_CURVE ( 'NONE', #10704, #23016, #18311, .T. ) ;
#8999=VERTEX_POINT ( 'NONE', #4664 ) ;
#9000=ORIENTED_EDGE ( 'NONE', *, *, #30048, .T. ) ;
#9001=EDGE_CURVE ( 'NONE', #9038, #3252, #9895, .T. ) ;
#9002=DIRECTION ( 'NONE',  ( 0.5000000000000038858, 0.8660254037844363761, 0.000000000000000000 ) ) ;
#9004=FACE_OUTER_BOUND ( 'NONE', #34136, .T. ) ;
#9007=DIRECTION ( 'NONE',  ( 1.000000000000000000, 0.000000000000000000, 0.000000000000000000 ) ) ;
#9009=DIRECTION ( 'NONE',  ( -1.000000000000000000, 0.000000000000000000, 0.000000000000000000 ) ) ;
#9011=DIRECTION ( 'NONE',  ( 1.000000000000000000, 0.000000000000000000, 0.000000000000000000 ) ) ;
#9012=ORIENTED_EDGE ( 'NONE', *, *, #4776, .F. ) ;
#9013=DIRECTION ( 'NONE',  ( 0.000000000000000000, 0.000000000000000000, 1.000000000000000000 ) ) ;
#9015=ORIENTED_EDGE ( 'NONE', *, *, #30057, .F. ) ;
#9016=ORIENTED_EDGE ( 'NONE', *, *, #28873, .F. ) ;
#9017=CARTESIAN_POINT ( 'NONE',  ( 37.99999662536853151, -69.28203230275519786, -9.999999999999998224 ) ) ;
#9018=CARTESIAN_POINT ( 'NONE',  ( -59.13646009116099833, 70.47608876694653190, -49.22241343995295892 ) ) ;
#9019=AXIS2_PLACEMENT_3D ( 'NONE', #28275, #16303, #22292 ) ;
#9021=CARTESIAN_POINT ( 'NONE',  ( 79.99999662536833966, 34.64101615137759183, -9.999999999999998224 ) ) ;
#9022=ORIENTED_EDGE ( 'NONE', *, *, #20128, .T. ) ;
#9023=ADVANCED_FACE ( 'NONE', ( #24899 ), #33541, .F. ) ;
#9024=CYLINDRICAL_SURFACE ( 'NONE', #5765, 2.000000000000001776 ) ;
#9026=DIRECTION ( 'NONE',  ( 0.000000000000000000, 0.000000000000000000, 1.000000000000000000 ) ) ;
#9028=DIRECTION ( 'NONE',  ( 0.000000000000000000, 0.000000000000000000, 1.000000000000000000 ) ) ;
#9031=LINE ( 'NONE', #29075, #10999 ) ;
#9032=DIRECTION ( 'NONE',  ( 1.000000000000000000, 0.000000000000000000, 0.000000000000000000 ) ) ;
#9035=CARTESIAN_POINT ( 'NONE',  ( 27.99999662536855993, 69.28203230275518365, -5.000000000000000000 ) ) ;
#9037=CYLINDRICAL_SURFACE ( 'NONE', #13707, 2.000000000000001776 ) ;
#9038=VERTEX_POINT ( 'NONE', #1653 ) ;
#9039=DIRECTION ( 'NONE',  ( -1.000000000000000000, 0.000000000000000000, 0.000000000000000000 ) ) ;
#9041=EDGE_CURVE ( 'NONE', #26406, #6520, #19107, .T. ) ;
#9042=FACE_BOUND ( 'NONE', #4929, .T. ) ;
#9043=DIRECTION ( 'NONE',  ( 0.000000000000000000, 0.000000000000000000, 1.000000000000000000 ) ) ;
#9044=CARTESIAN_POINT ( 'NONE',  ( -90.00000337463090716, -1.040834085586084257E-14, 17.49999999999999645 ) ) ;
#9045=LINE ( 'NONE', #1169, #14704 ) ;
#9046=CARTESIAN_POINT ( 'NONE',  ( -27.00000337463121625, -77.94228634059963667, 12.50000000000000000 ) ) ;
#9047=CARTESIAN_POINT ( 'NONE',  ( -80.00000337463094979, -2.428612866367529932E-14, -9.999999999999998224 ) ) ;
#9049=ORIENTED_EDGE ( 'NONE', *, *, #925, .F. ) ;
#9050=DIRECTION ( 'NONE',  ( 0.000000000000000000, 0.000000000000000000, -1.000000000000000000 ) ) ;
#9051=FACE_BOUND ( 'NONE', #32229, .T. ) ;
#9052=DIRECTION ( 'NONE',  ( 1.000000000000000000, 0.000000000000000000, 0.000000000000000000 ) ) ;
#9054=ORIENTED_EDGE ( 'NONE', *, *, #9739, .T. ) ;
#9055=ORIENTED_EDGE ( 'NONE', *, *, #29588, .F. ) ;
#9056=DIRECTION ( 'NONE',  ( 0.000000000000000000, 0.000000000000000000, 1.000000000000000000 ) ) ;
#9057=DIRECTION ( 'NONE',  ( 0.000000000000000000, 0.000000000000000000, 1.000000000000000000 ) ) ;
#9058=DIRECTION ( 'NONE',  ( 0.000000000000000000, 0.000000000000000000, 1.000000000000000000 ) ) ;
#9059=ORIENTED_EDGE ( 'NONE', *, *, #9445, .T. ) ;
#9060=AXIS2_PLACEMENT_3D ( 'NONE', #12165, #15019, #9751 ) ;
#9061=EDGE_CURVE ( 'NONE', #24391, #13923, #8758, .T. ) ;
#9062=CYLINDRICAL_SURFACE ( 'NONE', #25700, 33.00000000000001421 ) ;
#9063=ORIENTED_EDGE ( 'NONE', *, *, #17873, .F. ) ;
#9064=DIRECTION ( 'NONE',  ( 0.000000000000000000, 0.000000000000000000, -1.000000000000000000 ) ) ;
#9066=ORIENTED_EDGE ( 'NONE', *, *, #17790, .T. ) ;
#9067=CARTESIAN_POINT ( 'NONE',  ( 4.999996625368676284, -77.94228634059960825, -9.999999999999998224 ) ) ;
#9068=ORIENTED_EDGE ( 'NONE', *, *, #2210, .T. ) ;
#9069=ORIENTED_EDGE ( 'NONE', *, *, #22572, .F. ) ;
#9070=EDGE_CURVE ( 'NONE', #31694, #26322, #10554, .T. ) ;
#9072=DIRECTION ( 'NONE',  ( -0.000000000000000000, -0.000000000000000000, 1.000000000000000000 ) ) ;
#9073=CARTESIAN_POINT ( 'NONE',  ( -80.00000337463094979, -17.32050807568882078, -9.999999999999998224 ) ) ;
#9075=LINE ( 'NONE', #11693, #15494 ) ;
#9076=FACE_OUTER_BOUND ( 'NONE', #25047, .T. ) ;
#9077=LINE ( 'NONE', #20692, #20261 ) ;
#9078=ORIENTED_EDGE ( 'NONE', *, *, #2624, .F. ) ;
#9079=CARTESIAN_POINT ( 'NONE',  ( 1.999996625368672287, 86.60254037844397601, -5.000000000000000000 ) ) ;
#9081=CIRCLE ( 'NONE', #1893, 2.000000000000001776 ) ;
#9082=ORIENTED_EDGE ( 'NONE', *, *, #12379, .F. ) ;
#9084=CYLINDRICAL_SURFACE ( 'NONE', #23214, 3.000000000000002665 ) ;
#9085=AXIS2_PLACEMENT_3D ( 'NONE', #33985, #28327, #379 ) ;
#9086=CARTESIAN_POINT ( 'NONE',  ( -40.00000337463113453, -69.28203230275519786, 17.49999999999999645 ) ) ;
#9087=CARTESIAN_POINT ( 'NONE',  ( -58.88972745734155723, 34.00000000000049027, -49.22241343995295892 ) ) ;
#9089=LINE ( 'NONE', #18085, #24512 ) ;
#9090=CARTESIAN_POINT ( 'NONE',  ( 62.99999662536842493, 43.30127018922200222, -9.999999999999998224 ) ) ;
#9091=ORIENTED_EDGE ( 'NONE', *, *, #30727, .F. ) ;
#9092=CARTESIAN_POINT ( 'NONE',  ( 76.99999662536836809, 25.98076211353319565, 12.50000000000000000 ) ) ;
#9093=CARTESIAN_POINT ( 'NONE',  ( -63.00000337463102085, 25.98076211353317433, 17.49999999999999645 ) ) ;
#9094=PLANE ( 'NONE',  #12160 ) ;
#9096=EDGE_CURVE ( 'NONE', #14947, #2754, #21532, .T. ) ;
#9097=EDGE_LOOP ( 'NONE', ( #22892, #3010, #35727, #8415 ) ) ;
#9098=ORIENTED_EDGE ( 'NONE', *, *, #34645, .F. ) ;
#9099=EDGE_CURVE ( 'NONE', #9326, #15905, #22517, .T. ) ;
#9100=DIRECTION ( 'NONE',  ( 1.000000000000000000, 0.000000000000000000, 0.000000000000000000 ) ) ;
#9102=LINE ( 'NONE', #9283, #32643 ) ;
#9103=CIRCLE ( 'NONE', #30064, 2.000000000000000000 ) ;
#9104=DIRECTION ( 'NONE',  ( 0.000000000000000000, 0.000000000000000000, 1.000000000000000000 ) ) ;
#9105=ORIENTED_EDGE ( 'NONE', *, *, #7302, .T. ) ;
#9106=DIRECTION ( 'NONE',  ( 0.000000000000000000, 0.000000000000000000, 1.000000000000000000 ) ) ;
#9108=ORIENTED_EDGE ( 'NONE', *, *, #16661, .F. ) ;
#9109=FACE_BOUND ( 'NONE', #20920, .T. ) ;
#9113=EDGE_LOOP ( 'NONE', ( #29560, #541, #25039, #6726, #1858 ) ) ;
#9114=LINE ( 'NONE', #28806, #20631 ) ;
#9116=CARTESIAN_POINT ( 'NONE',  ( 67.99999662536838230, -17.32050807568879947, -9.999999999999998224 ) ) ;
#9117=AXIS2_PLACEMENT_3D ( 'NONE', #35090, #31874, #20834 ) ;
#9118=CIRCLE ( 'NONE', #11527, 2.000000000000001776 ) ;
#9119=DIRECTION ( 'NONE',  ( 0.000000000000000000, 0.000000000000000000, 1.000000000000000000 ) ) ;
#9120=DIRECTION ( 'NONE',  ( 0.000000000000000000, 0.000000000000000000, 1.000000000000000000 ) ) ;
#9121=ORIENTED_EDGE ( 'NONE', *, *, #16543, .T. ) ;
#9122=CYLINDRICAL_SURFACE ( 'NONE', #2232, 2.000000000000001776 ) ;
#9123=DIRECTION ( 'NONE',  ( 0.000000000000000000, 0.000000000000000000, 1.000000000000000000 ) ) ;
#9125=VERTEX_POINT ( 'NONE', #32777 ) ;
#9126=EDGE_CURVE ( 'NONE', #21452, #35244, #24715, .T. ) ;
#9130=CARTESIAN_POINT ( 'NONE',  ( 74.99999662536835388, -25.98076211353319565, -9.999999999999998224 ) ) ;
#9131=EDGE_CURVE ( 'NONE', #24647, #20619, #4567, .T. ) ;
#9133=EDGE_CURVE ( 'NONE', #20202, #16545, #8148, .T. ) ;
#9134=DIRECTION ( 'NONE',  ( 0.000000000000000000, 0.000000000000000000, -1.000000000000000000 ) ) ;
#9135=DIRECTION ( 'NONE',  ( 0.000000000000000000, 0.000000000000000000, -1.000000000000000000 ) ) ;
#9136=CARTESIAN_POINT ( 'NONE',  ( 31.83425564451589196, 89.42901512340320380, -5.000000000000011546 ) ) ;
#9137=CARTESIAN_POINT ( 'NONE',  ( 84.99999662536831124, -25.98076211353319565, -9.999999999999998224 ) ) ;
#9138=EDGE_LOOP ( 'NONE', ( #16835, #29398, #14431, #17781 ) ) ;
#9139=ORIENTED_EDGE ( 'NONE', *, *, #25907, .T. ) ;
#9140=CIRCLE ( 'NONE', #31304, 2.000000000000001776 ) ;
#9141=CARTESIAN_POINT ( 'NONE',  ( -34.60911769017402406, 75.98085615278088767, 12.50000000000000000 ) ) ;
#9143=DIRECTION ( 'NONE',  ( -0.000000000000000000, -0.000000000000000000, 1.000000000000000000 ) ) ;
#9145=EDGE_CURVE ( 'NONE', #16686, #9342, #965, .T. ) ;
#9146=FACE_BOUND ( 'NONE', #20648, .T. ) ;
#9147=EDGE_LOOP ( 'NONE', ( #17328, #36391, #164, #32399 ) ) ;
#9149=ORIENTED_EDGE ( 'NONE', *, *, #27411, .T. ) ;
#9150=CARTESIAN_POINT ( 'NONE',  ( 29.99999662536856349, 69.28203230275518365, -5.000000000000000000 ) ) ;
#9151=ORIENTED_EDGE ( 'NONE', *, *, #34396, .F. ) ;
#9157=AXIS2_PLACEMENT_3D ( 'NONE', #23129, #28375, #19782 ) ;
#9159=VERTEX_POINT ( 'NONE', #1842 ) ;
#9160=AXIS2_PLACEMENT_3D ( 'NONE', #9534, #35781, #35237 ) ;
#9161=EDGE_CURVE ( 'NONE', #34031, #34992, #15937, .T. ) ;
#9162=EDGE_LOOP ( 'NONE', ( #14890, #6265, #11326, #32054 ) ) ;
#9163=DIRECTION ( 'NONE',  ( -0.000000000000000000, -0.000000000000000000, 1.000000000000000000 ) ) ;
#9164=CARTESIAN_POINT ( 'NONE',  ( -20.00000337463122690, 86.60254037844397601, -9.999999999999998224 ) ) ;
#9165=ADVANCED_FACE ( 'NONE', ( #22999 ), #2956, .F. ) ;
#9166=EDGE_LOOP ( 'NONE', ( #29432, #652 ) ) ;
#9167=FACE_OUTER_BOUND ( 'NONE', #16611, .T. ) ;
#9169=DIRECTION ( 'NONE',  ( 0.000000000000000000, 0.000000000000000000, -1.000000000000000000 ) ) ;
#9170=ORIENTED_EDGE ( 'NONE', *, *, #29414, .T. ) ;
#9171=FACE_OUTER_BOUND ( 'NONE', #7441, .T. ) ;
#9172=AXIS2_PLACEMENT_3D ( 'NONE', #2369, #30104, #24865 ) ;
#9173=ADVANCED_FACE ( 'NONE', ( #25827 ), #28625, .F. ) ;
#9175=DIRECTION ( 'NONE',  ( 0.000000000000000000, 0.000000000000000000, 1.000000000000000000 ) ) ;
#9176=ORIENTED_EDGE ( 'NONE', *, *, #22572, .T. ) ;
#9177=CARTESIAN_POINT ( 'NONE',  ( 3.108933952041194271, 78.59334852315024023, 12.50000000000000000 ) ) ;
#9178=EDGE_CURVE ( 'NONE', #19731, #18123, #2755, .T. ) ;
#9179=CARTESIAN_POINT ( 'NONE',  ( -30.00000337463119848, -69.28203230275522628, -9.999999999999998224 ) ) ;
#9180=ADVANCED_FACE ( 'NONE', ( #31251 ), #14384, .T. ) ;
#9181=AXIS2_PLACEMENT_3D ( 'NONE', #31775, #3286, #17180 ) ;
#9183=ORIENTED_EDGE ( 'NONE', *, *, #3045, .T. ) ;
#9185=FACE_OUTER_BOUND ( 'NONE', #13229, .T. ) ;
#9186=CYLINDRICAL_SURFACE ( 'NONE', #7897, 33.00000000000001421 ) ;
#9188=DIRECTION ( 'NONE',  ( 1.000000000000000000, 0.000000000000000000, 0.000000000000000000 ) ) ;
#9189=ORIENTED_EDGE ( 'NONE', *, *, #31314, .T. ) ;
#9190=ADVANCED_FACE ( 'NONE', ( #11383, #33705, #19645, #31428, #25443, #14190, #30872, #11191, #22440, #34091, #25649, #20189, #31617, #5208, #5567, #22268, #5953, #17004, #17384, #2404, #10998, #2204, #13641, #34266, #25102, #13829, #33890, #10838, #8011, #19450, #16646, #5753, #28076, #25275, #8566, #19999, #36700, #5402, #16836, #28254, #2575, #36882, #22643, #8396, #19828, #23193, #3851, #31957, #20534, #12476, #26733, #3300, #32364, #21106, #6296, #15293, #31790, #23383, #6119, #1050, #18104, #6848, #17547, #23942, #12268, #35394, #9679, #32531, #14738, #28803, #11921, #3128, #9109, #14552, #35194, #15110, #34639, #25992, #20726, #20373, #26183, #9500, #294, #11730, #28971, #8937, #499, #17733, #29529, #32162, #34817, #29173, #3681, #3505, #14941, #26372, #678, #12089, #23549, #34993, #9291, #6500, #26542, #17935, #29366, #853, #23744, #20934, #6680, #32727, #16238, #7601, #7416, #19054, #29921, #1411, #13395, #33490, #18290, #15495, #10405, #7053, #7242, #1241, #21842, #10051, #27655, #18675, #21667, #30279, #12658, #29719, #22043, #4053, #24853, #36292, #15676, #4614, #33286, #18856 ), #4804, .T. ) ;
#9191=CARTESIAN_POINT ( 'NONE',  ( 79.99999662536833966, 17.32050807568879236, -9.999999999999998224 ) ) ;
#9192=DIRECTION ( 'NONE',  ( 1.000000000000000000, 0.000000000000000000, 0.000000000000000000 ) ) ;
#9193=EDGE_CURVE ( 'NONE', #29609, #31054, #20133, .T. ) ;
#9195=AXIS2_PLACEMENT_3D ( 'NONE', #18321, #10260, #13255 ) ;
#9196=EDGE_CURVE ( 'NONE', #18736, #8614, #24939, .T. ) ;
#9198=ADVANCED_FACE ( 'NONE', ( #26925 ), #24675, .F. ) ;
#9199=CARTESIAN_POINT ( 'NONE',  ( -85.00000337463092137, -25.98076211353322051, 12.50000000000000000 ) ) ;
#9201=CARTESIAN_POINT ( 'NONE',  ( -72.00000337463100664, 51.96152422706637708, 12.50000000000000000 ) ) ;
#9202=LINE ( 'NONE', #6595, #36175 ) ;
#9203=VECTOR ( 'NONE', #2081, 1000.000000000000000 ) ;
#9204=DIRECTION ( 'NONE',  ( 1.000000000000000000, 0.000000000000000000, 0.000000000000000000 ) ) ;
#9205=ORIENTED_EDGE ( 'NONE', *, *, #25346, .F. ) ;
#9206=VERTEX_POINT ( 'NONE', #27097 ) ;
#9208=LINE ( 'NONE', #20638, #7654 ) ;
#9209=CARTESIAN_POINT ( 'NONE',  ( 62.19434990244977257, -52.39915983220758022, -4.999999999999997335 ) ) ;
#9210=VERTEX_POINT ( 'NONE', #9846 ) ;
#9212=FACE_BOUND ( 'NONE', #36289, .T. ) ;
#9213=DIRECTION ( 'NONE',  ( 1.000000000000000000, 0.000000000000000000, 0.000000000000000000 ) ) ;
#9214=DIRECTION ( 'NONE',  ( -0.000000000000000000, -0.000000000000000000, 1.000000000000000000 ) ) ;
#9215=PLANE ( 'NONE',  #20693 ) ;
#9216=VERTEX_POINT ( 'NONE', #21286 ) ;
#9220=DIRECTION ( 'NONE',  ( 0.000000000000000000, 0.000000000000000000, 1.000000000000000000 ) ) ;
#9221=ORIENTED_EDGE ( 'NONE', *, *, #17457, .T. ) ;
#9223=CARTESIAN_POINT ( 'NONE',  ( 59.99999662536843914, -34.64101615137759893, 12.50000000000000000 ) ) ;
#9224=CARTESIAN_POINT ( 'NONE',  ( 1.999996625368672287, 86.60254037844397601, -9.999999999999998224 ) ) ;
#9225=VECTOR ( 'NONE', #4157, 1000.000000000000000 ) ;
#9227=VERTEX_POINT ( 'NONE', #18499 ) ;
#9228=VERTEX_POINT ( 'NONE', #15852 ) ;
#9229=AXIS2_PLACEMENT_3D ( 'NONE', #30357, #13674, #33166 ) ;
#9230=DIRECTION ( 'NONE',  ( 1.000000000000000000, 0.000000000000000000, 0.000000000000000000 ) ) ;
#9231=FACE_OUTER_BOUND ( 'NONE', #23205, .T. ) ;
#9232=CARTESIAN_POINT ( 'NONE',  ( 82.99999662536832545, 8.660254037844394404, -5.000000000000000000 ) ) ;
#9233=EDGE_LOOP ( 'NONE', ( #930, #8052, #16369, #19779, #12946, #5152 ) ) ;
#9235=ORIENTED_EDGE ( 'NONE', *, *, #4540, .F. ) ;
#9237=LINE ( 'NONE', #11677, #9525 ) ;
#9238=ORIENTED_EDGE ( 'NONE', *, *, #17772, .F. ) ;
#9239=EDGE_CURVE ( 'NONE', #19593, #31910, #29704, .T. ) ;
#9241=AXIS2_PLACEMENT_3D ( 'NONE', #14805, #34503, #9002 ) ;
#9245=EDGE_LOOP ( 'NONE', ( #36968, #14080, #17600, #29572 ) ) ;
#9246=AXIS2_PLACEMENT_3D ( 'NONE', #5050, #13479, #4702 ) ;
#9247=DIRECTION ( 'NONE',  ( 0.000000000000000000, 0.000000000000000000, 1.000000000000000000 ) ) ;
#9248=CYLINDRICAL_SURFACE ( 'NONE', #17221, 33.00000000000001421 ) ;
#9249=LINE ( 'NONE', #26142, #13457 ) ;
#9250=EDGE_LOOP ( 'NONE', ( #7783, #2613 ) ) ;
#9251=ORIENTED_EDGE ( 'NONE', *, *, #24473, .F. ) ;
#9252=DIRECTION ( 'NONE',  ( 0.000000000000000000, 0.000000000000000000, 1.000000000000000000 ) ) ;
#9253=CIRCLE ( 'NONE', #5067, 2.000000000000001776 ) ;
#9254=CARTESIAN_POINT ( 'NONE',  ( 79.99999662536833966, -3.469446951953614189E-15, 12.50000000000000000 ) ) ;
#9255=AXIS2_PLACEMENT_3D ( 'NONE', #19322, #33585, #36581 ) ;
#9256=CARTESIAN_POINT ( 'NONE',  ( -37.00000337463116296, 77.94228634059957983, -9.999999999999998224 ) ) ;
#9257=ORIENTED_EDGE ( 'NONE', *, *, #36264, .T. ) ;
#9258=CIRCLE ( 'NONE', #21849, 27.00000000000001421 ) ;
#9259=DIRECTION ( 'NONE',  ( 1.000000000000000000, 0.000000000000000000, 0.000000000000000000 ) ) ;
#9260=DIRECTION ( 'NONE',  ( 0.000000000000000000, 0.000000000000000000, -1.000000000000000000 ) ) ;
#9262=DIRECTION ( 'NONE',  ( 0.000000000000000000, -0.000000000000000000, -1.000000000000000000 ) ) ;
#9263=DIRECTION ( 'NONE',  ( 0.000000000000000000, 0.000000000000000000, 1.000000000000000000 ) ) ;
#9265=EDGE_CURVE ( 'NONE', #2172, #15620, #1552, .T. ) ;
#9267=DIRECTION ( 'NONE',  ( 0.000000000000000000, 0.000000000000000000, 1.000000000000000000 ) ) ;
#9268=CARTESIAN_POINT ( 'NONE',  ( 79.99999662536832545, -17.32050807568879591, 12.50000000000000000 ) ) ;
#9269=AXIS2_PLACEMENT_3D ( 'NONE', #3131, #20378, #29179 ) ;
#9270=DIRECTION ( 'NONE',  ( 1.000000000000000000, 0.000000000000000000, 0.000000000000000000 ) ) ;
#9271=EDGE_LOOP ( 'NONE', ( #32796, #1010 ) ) ;
#9272=FACE_OUTER_BOUND ( 'NONE', #36067, .T. ) ;
#9273=VECTOR ( 'NONE', #25621, 1000.000000000000000 ) ;
#9274=CARTESIAN_POINT ( 'NONE',  ( -65.00000000000000000, 0.000000000000000000, -4.999999999999997335 ) ) ;
#9275=CARTESIAN_POINT ( 'NONE',  ( 59.99999662536845335, 34.64101615137759893, -9.999999999999998224 ) ) ;
#9276=ORIENTED_EDGE ( 'NONE', *, *, #13251, .F. ) ;
#9277=ADVANCED_FACE ( 'NONE', ( #33095 ), #27279, .F. ) ;
#9278=ORIENTED_EDGE ( 'NONE', *, *, #12739, .T. ) ;
#9279=ORIENTED_EDGE ( 'NONE', *, *, #15092, .T. ) ;
#9282=CARTESIAN_POINT ( 'NONE',  ( 0.000000000000000000, -55.00000000000000000, -5.000000000000000000 ) ) ;
#9283=CARTESIAN_POINT ( 'NONE',  ( 52.99999662536846046, -43.30127018922200222, -9.999999999999998224 ) ) ;
#9284=AXIS2_PLACEMENT_3D ( 'NONE', #29674, #14520, #34781 ) ;
#9285=LINE ( 'NONE', #16866, #8480 ) ;
#9286=DIRECTION ( 'NONE',  ( 0.000000000000000000, 0.000000000000000000, 1.000000000000000000 ) ) ;
#9287=ORIENTED_EDGE ( 'NONE', *, *, #30744, .F. ) ;
#9288=EDGE_CURVE ( 'NONE', #21337, #14745, #2146, .T. ) ;
#9289=CYLINDRICAL_SURFACE ( 'NONE', #11373, 2.000000000000001776 ) ;
#9290=ORIENTED_EDGE ( 'NONE', *, *, #4436, .F. ) ;
#9291=FACE_BOUND ( 'NONE', #25342, .T. ) ;
#9292=CYLINDRICAL_SURFACE ( 'NONE', #17939, 2.000000000000001776 ) ;
#9293=VECTOR ( 'NONE', #5537, 1000.000000000000000 ) ;
#9294=DIRECTION ( 'NONE',  ( 1.000000000000000000, 0.000000000000000000, 0.000000000000000000 ) ) ;
#9295=CIRCLE ( 'NONE', #3332, 2.000000000000001776 ) ;
#9296=EDGE_LOOP ( 'NONE', ( #8283, #3282 ) ) ;
#9297=CARTESIAN_POINT ( 'NONE',  ( 65.00000000000000000, 7.960204194457797252E-15, 17.49999999999999645 ) ) ;
#9299=AXIS2_PLACEMENT_3D ( 'NONE', #36529, #13262, #25438 ) ;
#9301=DIRECTION ( 'NONE',  ( 0.000000000000000000, 0.000000000000000000, 1.000000000000000000 ) ) ;
#9302=CYLINDRICAL_SURFACE ( 'NONE', #20355, 2.000000000000001776 ) ;
#9303=DIRECTION ( 'NONE',  ( 1.000000000000000000, 0.000000000000000000, 0.000000000000000000 ) ) ;
#9304=ADVANCED_FACE ( 'NONE', ( #7796 ), #81, .T. ) ;
#9305=EDGE_LOOP ( 'NONE', ( #25086, #32776, #28388, #26047 ) ) ;
#9306=PLANE ( 'NONE',  #21481 ) ;
#9307=DIRECTION ( 'NONE',  ( 0.000000000000000000, 0.000000000000000000, 1.000000000000000000 ) ) ;
#9308=DIRECTION ( 'NONE',  ( 0.000000000000000000, 0.000000000000000000, 1.000000000000000000 ) ) ;
#9309=EDGE_CURVE ( 'NONE', #6244, #31374, #27887, .T. ) ;
#9310=AXIS2_PLACEMENT_3D ( 'NONE', #6462, #5919, #17351 ) ;
#9311=VECTOR ( 'NONE', #6880, 1000.000000000000000 ) ;
#9312=ORIENTED_EDGE ( 'NONE', *, *, #26552, .F. ) ;
#9313=ORIENTED_EDGE ( 'NONE', *, *, #33435, .T. ) ;
#9314=EDGE_LOOP ( 'NONE', ( #8304, #13299, #22943, #30322, #26776, #2657 ) ) ;
#9315=EDGE_CURVE ( 'NONE', #8449, #4001, #20712, .T. ) ;
#9316=CARTESIAN_POINT ( 'NONE',  ( 16.49657687835809128, -93.55673653615983199, 12.49999999999999822 ) ) ;
#9317=CARTESIAN_POINT ( 'NONE',  ( 44.99999662536849598, -77.94228634059960825, -9.999999999999998224 ) ) ;
#9318=CARTESIAN_POINT ( 'NONE',  ( 7.122621931239992550E-13, 68.00000000000000000, -4.999999999999997335 ) ) ;
#9319=ADVANCED_FACE ( 'NONE', ( #34229 ), #8523, .F. ) ;
#9320=DIRECTION ( 'NONE',  ( 0.000000000000000000, 0.000000000000000000, 1.000000000000000000 ) ) ;
#9321=DIRECTION ( 'NONE',  ( 0.000000000000000000, 0.000000000000000000, -1.000000000000000000 ) ) ;
#9323=CIRCLE ( 'NONE', #23715, 1.999999999999998224 ) ;
#9325=VECTOR ( 'NONE', #24108, 1000.000000000000000 ) ;
#9326=VERTEX_POINT ( 'NONE', #19405 ) ;
#9327=CIRCLE ( 'NONE', #35091, 2.000000000000001776 ) ;
#9329=CYLINDRICAL_SURFACE ( 'NONE', #21271, 1.999999999999998224 ) ;
#9330=CIRCLE ( 'NONE', #7551, 2.000000000000001776 ) ;
#9332=VERTEX_POINT ( 'NONE', #27829 ) ;
#9333=CARTESIAN_POINT ( 'NONE',  ( 74.99999662536836809, 25.98076211353319565, -5.000000000000000000 ) ) ;
#9337=EDGE_CURVE ( 'NONE', #22341, #28072, #17745, .T. ) ;
#9338=FACE_BOUND ( 'NONE', #11328, .T. ) ;
#9339=ORIENTED_EDGE ( 'NONE', *, *, #32051, .F. ) ;
#9340=ORIENTED_EDGE ( 'NONE', *, *, #14181, .F. ) ;
#9341=DIRECTION ( 'NONE',  ( 1.000000000000000000, 0.000000000000000000, 0.000000000000000000 ) ) ;
#9342=VERTEX_POINT ( 'NONE', #28213 ) ;
#9344=AXIS2_PLACEMENT_3D ( 'NONE', #22409, #5722, #7982 ) ;
#9345=ADVANCED_FACE ( 'NONE', ( #25594 ), #10793, .F. ) ;
#9346=FACE_OUTER_BOUND ( 'NONE', #15798, .T. ) ;
#9347=DIRECTION ( 'NONE',  ( 0.000000000000000000, 0.000000000000000000, 1.000000000000000000 ) ) ;
#9348=CARTESIAN_POINT ( 'NONE',  ( 0.000000000000000000, 0.000000000000000000, 12.49999999999999822 ) ) ;
#9349=EDGE_CURVE ( 'NONE', #27267, #10069, #30651, .T. ) ;
#9350=EDGE_LOOP ( 'NONE', ( #12440, #32328 ) ) ;
#9351=ORIENTED_EDGE ( 'NONE', *, *, #268, .T. ) ;
#9353=AXIS2_PLACEMENT_3D ( 'NONE', #5354, #22944, #33655 ) ;
#9355=ORIENTED_EDGE ( 'NONE', *, *, #30818, .T. ) ;
#9356=AXIS2_PLACEMENT_3D ( 'NONE', #29820, #1142, #12932 ) ;
#9358=ORIENTED_EDGE ( 'NONE', *, *, #31702, .T. ) ;
#9359=CIRCLE ( 'NONE', #5758, 2.000000000000001776 ) ;
#9360=ORIENTED_EDGE ( 'NONE', *, *, #36399, .T. ) ;
#9361=CARTESIAN_POINT ( 'NONE',  ( 82.99999662536832545, 8.660254037844394404, -9.999999999999998224 ) ) ;
#9362=DIRECTION ( 'NONE',  ( 0.000000000000000000, 0.000000000000000000, 1.000000000000000000 ) ) ;
#9363=ORIENTED_EDGE ( 'NONE', *, *, #34907, .T. ) ;
#9364=DIRECTION ( 'NONE',  ( 0.000000000000000000, 0.000000000000000000, 1.000000000000000000 ) ) ;
#9365=FACE_OUTER_BOUND ( 'NONE', #8782, .T. ) ;
#9367=EDGE_LOOP ( 'NONE', ( #31206, #11260, #27309, #12425 ) ) ;
#9368=LINE ( 'NONE', #17273, #12848 ) ;
#9369=AXIS2_PLACEMENT_3D ( 'NONE', #34776, #20491, #11681 ) ;
#9371=EDGE_CURVE ( 'NONE', #10781, #5113, #8783, .T. ) ;
#9372=DIRECTION ( 'NONE',  ( 1.000000000000000000, 0.000000000000000000, 0.000000000000000000 ) ) ;
#9374=DIRECTION ( 'NONE',  ( 0.000000000000000000, 0.000000000000000000, 1.000000000000000000 ) ) ;
#9375=DIRECTION ( 'NONE',  ( 0.000000000000000000, 0.000000000000000000, 1.000000000000000000 ) ) ;
#9376=ORIENTED_EDGE ( 'NONE', *, *, #10337, .F. ) ;
#9379=CIRCLE ( 'NONE', #20748, 33.00000000000001421 ) ;
#9380=DIRECTION ( 'NONE',  ( 0.000000000000000000, 0.000000000000000000, 1.000000000000000000 ) ) ;
#9381=CARTESIAN_POINT ( 'NONE',  ( 64.99999662536841072, -25.98076211353320275, -9.999999999999998224 ) ) ;
#9384=ORIENTED_EDGE ( 'NONE', *, *, #1147, .F. ) ;
#9385=VECTOR ( 'NONE', #8550, 1000.000000000000000 ) ;
#9387=CARTESIAN_POINT ( 'NONE',  ( -60.00000337463108480, -51.96152422706641971, 12.50000000000000000 ) ) ;
#9388=AXIS2_PLACEMENT_3D ( 'NONE', #7987, #30305, #5180 ) ;
#9389=EDGE_CURVE ( 'NONE', #26415, #21303, #19598, .T. ) ;
#9390=ORIENTED_EDGE ( 'NONE', *, *, #13295, .T. ) ;
#9391=EDGE_CURVE ( 'NONE', #7069, #30820, #26128, .T. ) ;
#9392=LINE ( 'NONE', #3209, #6397 ) ;
#9393=EDGE_LOOP ( 'NONE', ( #14648, #16085 ) ) ;
#9394=CARTESIAN_POINT ( 'NONE',  ( -3.374631334790434423E-06, 69.28203230275516944, 12.50000000000000000 ) ) ;
#9395=AXIS2_PLACEMENT_3D ( 'NONE', #21751, #29623, #32833 ) ;
#9396=EDGE_CURVE ( 'NONE', #23264, #15061, #31029, .T. ) ;
#9397=DIRECTION ( 'NONE',  ( 1.000000000000000000, 0.000000000000000000, 0.000000000000000000 ) ) ;
#9398=CYLINDRICAL_SURFACE ( 'NONE', #32193, 2.000000000000001776 ) ;
#9399=ORIENTED_EDGE ( 'NONE', *, *, #28684, .F. ) ;
#9400=VERTEX_POINT ( 'NONE', #13790 ) ;
#9401=ADVANCED_FACE ( 'NONE', ( #2705 ), #16795, .F. ) ;
#9402=CIRCLE ( 'NONE', #35177, 2.000000000000000000 ) ;
#9403=EDGE_CURVE ( 'NONE', #24339, #22350, #7586, .T. ) ;
#9404=CIRCLE ( 'NONE', #7628, 2.000000000000001776 ) ;
#9405=CARTESIAN_POINT ( 'NONE',  ( 35.19434990244975126, -52.39915983220758022, 12.49999999999999822 ) ) ;
#9407=AXIS2_PLACEMENT_3D ( 'NONE', #28748, #25935, #5347 ) ;
#9408=ORIENTED_EDGE ( 'NONE', *, *, #32810, .F. ) ;
#9409=DIRECTION ( 'NONE',  ( -1.000000000000000000, 0.000000000000000000, 0.000000000000000000 ) ) ;
#9410=CARTESIAN_POINT ( 'NONE',  ( -3.374631303565411855E-06, -86.60254037844400443, 17.49999999999999645 ) ) ;
#9412=DIRECTION ( 'NONE',  ( 0.000000000000000000, 0.000000000000000000, -1.000000000000000000 ) ) ;
#9414=DIRECTION ( 'NONE',  ( 0.000000000000000000, 0.000000000000000000, 1.000000000000000000 ) ) ;
#9415=ADVANCED_FACE ( 'NONE', ( #30823 ), #5160, .F. ) ;
#9416=AXIS2_PLACEMENT_3D ( 'NONE', #8527, #14142, #25602 ) ;
#9417=ORIENTED_EDGE ( 'NONE', *, *, #27127, .T. ) ;
#9418=DIRECTION ( 'NONE',  ( 0.000000000000000000, 0.000000000000000000, 1.000000000000000000 ) ) ;
#9419=AXIS2_PLACEMENT_3D ( 'NONE', #31108, #2041, #33570 ) ;
#9420=EDGE_CURVE ( 'NONE', #14513, #27693, #12949, .T. ) ;
#9421=CIRCLE ( 'NONE', #17190, 2.000000000000001776 ) ;
#9422=CARTESIAN_POINT ( 'NONE',  ( -43.00000337463112743, -60.62177826491080168, -9.999999999999998224 ) ) ;
#9423=EDGE_CURVE ( 'NONE', #25244, #5952, #2798, .T. ) ;
#9424=DIRECTION ( 'NONE',  ( -1.000000000000000000, 0.000000000000000000, 0.000000000000000000 ) ) ;
#9425=VERTEX_POINT ( 'NONE', #17342 ) ;
#9426=EDGE_CURVE ( 'NONE', #19493, #31662, #442, .T. ) ;
#9427=CARTESIAN_POINT ( 'NONE',  ( 71.99999662536839651, -3.469446951953614189E-15, -9.999999999999998224 ) ) ;
#9428=LINE ( 'NONE', #23489, #27320 ) ;
#9429=DIRECTION ( 'NONE',  ( 0.5000000000000039968, 0.8660254037844363761, 0.000000000000000000 ) ) ;
#9432=EDGE_LOOP ( 'NONE', ( #1280, #24860, #5321, #33944, #7824 ) ) ;
#9434=AXIS2_PLACEMENT_3D ( 'NONE', #8689, #26126, #22783 ) ;
#9435=LINE ( 'NONE', #26317, #35216 ) ;
#9436=CARTESIAN_POINT ( 'NONE',  ( -80.00000337463094979, 17.32050807568878525, -9.999999999999998224 ) ) ;
#9438=EDGE_LOOP ( 'NONE', ( #9543, #33120, #7711, #16413 ) ) ;
#9439=EDGE_LOOP ( 'NONE', ( #10166, #19060 ) ) ;
#9440=CIRCLE ( 'NONE', #20224, 27.00000000000001066 ) ;
#9441=CIRCLE ( 'NONE', #32171, 2.000000000000001776 ) ;
#9442=ORIENTED_EDGE ( 'NONE', *, *, #32948, .T. ) ;
#9443=AXIS2_PLACEMENT_3D ( 'NONE', #11643, #5869, #2669 ) ;
#9444=DIRECTION ( 'NONE',  ( 1.000000000000000000, 0.000000000000000000, 0.000000000000000000 ) ) ;
#9445=EDGE_CURVE ( 'NONE', #36367, #36578, #6994, .T. ) ;
#9446=AXIS2_PLACEMENT_3D ( 'NONE', #18427, #26112, #422 ) ;
#9447=EDGE_LOOP ( 'NONE', ( #9555, #20038, #11595, #31111 ) ) ;
#9448=CARTESIAN_POINT ( 'NONE',  ( -10.00000337463128730, 69.28203230275516944, -9.999999999999998224 ) ) ;
#9449=ORIENTED_EDGE ( 'NONE', *, *, #24022, .F. ) ;
#9450=CARTESIAN_POINT ( 'NONE',  ( -36.97203788308986105, 58.48108235278859013, 12.49999999999999645 ) ) ;
#9451=ORIENTED_EDGE ( 'NONE', *, *, #9878, .F. ) ;
#9452=ORIENTED_EDGE ( 'NONE', *, *, #17058, .F. ) ;
#9453=AXIS2_PLACEMENT_3D ( 'NONE', #24100, #27268, #22033 ) ;
#9454=AXIS2_PLACEMENT_3D ( 'NONE', #15248, #1199, #18066 ) ;
#9457=DIRECTION ( 'NONE',  ( 1.000000000000000000, 0.000000000000000000, 0.000000000000000000 ) ) ;
#9458=VERTEX_POINT ( 'NONE', #6079 ) ;
#9459=EDGE_LOOP ( 'NONE', ( #12655, #4098, #29470, #17836 ) ) ;
#9461=CYLINDRICAL_SURFACE ( 'NONE', #7732, 3.000000000000002665 ) ;
#9462=AXIS2_PLACEMENT_3D ( 'NONE', #37053, #28597, #8174 ) ;
#9463=CARTESIAN_POINT ( 'NONE',  ( -31.46585318596190106, -86.45172111230344569, -4.999999999999997335 ) ) ;
#9464=DIRECTION ( 'NONE',  ( 0.000000000000000000, 0.000000000000000000, 1.000000000000000000 ) ) ;
#9465=CARTESIAN_POINT ( 'NONE',  ( -80.00000337463096400, -34.64101615137762025, 12.50000000000000000 ) ) ;
#9466=EDGE_LOOP ( 'NONE', ( #29547, #14807 ) ) ;
#9467=FACE_OUTER_BOUND ( 'NONE', #29019, .T. ) ;
#9469=AXIS2_PLACEMENT_3D ( 'NONE', #20291, #26457, #26093 ) ;
#9471=FACE_OUTER_BOUND ( 'NONE', #23439, .T. ) ;
#9473=AXIS2_PLACEMENT_3D ( 'NONE', #4345, #18206, #26851 ) ;
#9474=DIRECTION ( 'NONE',  ( 0.000000000000000000, 0.000000000000000000, 1.000000000000000000 ) ) ;
#9475=CARTESIAN_POINT ( 'NONE',  ( -65.00000337463102085, 60.62177826491077326, -9.999999999999998224 ) ) ;
#9476=DIRECTION ( 'NONE',  ( -1.000000000000000000, 0.000000000000000000, 0.000000000000000000 ) ) ;
#9479=FACE_OUTER_BOUND ( 'NONE', #23212, .T. ) ;
#9482=ADVANCED_FACE ( 'NONE', ( #8698 ), #6251, .T. ) ;
#9484=VERTEX_POINT ( 'NONE', #9450 ) ;
#9485=DIRECTION ( 'NONE',  ( -1.000000000000000000, 0.000000000000000000, 0.000000000000000000 ) ) ;
#9488=ORIENTED_EDGE ( 'NONE', *, *, #2306, .F. ) ;
#9489=ORIENTED_EDGE ( 'NONE', *, *, #12289, .F. ) ;
#9490=EDGE_LOOP ( 'NONE', ( #2955, #24895, #14011, #15026 ) ) ;
#9491=DIRECTION ( 'NONE',  ( 0.000000000000000000, 0.000000000000000000, 1.000000000000000000 ) ) ;
#9492=DIRECTION ( 'NONE',  ( 3.469446951953612611E-15, 1.000000000000000000, 0.000000000000000000 ) ) ;
#9493=AXIS2_PLACEMENT_3D ( 'NONE', #127, #23010, #7858 ) ;
#9498=DIRECTION ( 'NONE',  ( 0.000000000000000000, 0.000000000000000000, 1.000000000000000000 ) ) ;
#9499=ORIENTED_EDGE ( 'NONE', *, *, #34088, .T. ) ;
#9500=FACE_BOUND ( 'NONE', #25874, .T. ) ;
#9501=EDGE_CURVE ( 'NONE', #8706, #17922, #35725, .T. ) ;
#9502=AXIS2_PLACEMENT_3D ( 'NONE', #26517, #14909, #32132 ) ;
#9503=AXIS2_PLACEMENT_3D ( 'NONE', #36731, #33568, #19307 ) ;
#9505=DIRECTION ( 'NONE',  ( 0.000000000000000000, 0.000000000000000000, 1.000000000000000000 ) ) ;
#9506=VERTEX_POINT ( 'NONE', #26133 ) ;
#9507=CARTESIAN_POINT ( 'NONE',  ( -12.00000337463125000, -86.60254037844400443, -9.999999999999998224 ) ) ;
#9508=CARTESIAN_POINT ( 'NONE',  ( -45.00000337463111322, 77.94228634059959404, -5.000000000000000000 ) ) ;
#9509=AXIS2_PLACEMENT_3D ( 'NONE', #22553, #28735, #19920 ) ;
#9510=CARTESIAN_POINT ( 'NONE',  ( -55.00000337463109901, -60.62177826491083010, -9.999999999999998224 ) ) ;
#9511=DIRECTION ( 'NONE',  ( 0.000000000000000000, 0.000000000000000000, 1.000000000000000000 ) ) ;
#9513=DIRECTION ( 'NONE',  ( 0.000000000000000000, 0.000000000000000000, 1.000000000000000000 ) ) ;
#9514=DIRECTION ( 'NONE',  ( 0.000000000000000000, 0.000000000000000000, 1.000000000000000000 ) ) ;
#9516=ORIENTED_EDGE ( 'NONE', *, *, #7506, .F. ) ;
#9517=EDGE_LOOP ( 'NONE', ( #26742, #20297, #20612, #15849 ) ) ;
#9518=CIRCLE ( 'NONE', #30473, 2.000000000000000000 ) ;
#9519=EDGE_CURVE ( 'NONE', #8231, #20602, #2205, .T. ) ;
#9520=ORIENTED_EDGE ( 'NONE', *, *, #21087, .F. ) ;
#9521=AXIS2_PLACEMENT_3D ( 'NONE', #7563, #15812, #7378 ) ;
#9522=DIRECTION ( 'NONE',  ( -0.000000000000000000, -0.000000000000000000, -1.000000000000000000 ) ) ;
#9523=DIRECTION ( 'NONE',  ( 0.000000000000000000, 0.000000000000000000, 1.000000000000000000 ) ) ;
#9525=VECTOR ( 'NONE', #28570, 1000.000000000000000 ) ;
#9526=DIRECTION ( 'NONE',  ( 1.000000000000000000, 0.000000000000000000, 0.000000000000000000 ) ) ;
#9530=VERTEX_POINT ( 'NONE', #6448 ) ;
#9532=DIRECTION ( 'NONE',  ( 0.000000000000000000, 0.000000000000000000, 1.000000000000000000 ) ) ;
#9533=AXIS2_PLACEMENT_3D ( 'NONE', #3129, #22646, #8209 ) ;
#9534=CARTESIAN_POINT ( 'NONE',  ( 62.97617850287784336, 4.279621169095339184, 12.49999999999999822 ) ) ;
#9535=EDGE_LOOP ( 'NONE', ( #14279, #18641, #16516, #2473 ) ) ;
#9536=AXIS2_PLACEMENT_3D ( 'NONE', #21082, #18836, #16217 ) ;
#9537=DIRECTION ( 'NONE',  ( 0.000000000000000000, 0.000000000000000000, -1.000000000000000000 ) ) ;
#9540=FACE_BOUND ( 'NONE', #26596, .T. ) ;
#9542=VERTEX_POINT ( 'NONE', #11875 ) ;
#9543=ORIENTED_EDGE ( 'NONE', *, *, #26689, .F. ) ;
#9544=AXIS2_PLACEMENT_3D ( 'NONE', #6908, #35434, #904 ) ;
#9545=DIRECTION ( 'NONE',  ( 1.000000000000000000, 0.000000000000000000, 0.000000000000000000 ) ) ;
#9546=ORIENTED_EDGE ( 'NONE', *, *, #23821, .T. ) ;
#9547=LINE ( 'NONE', #29408, #26628 ) ;
#9548=ADVANCED_FACE ( 'NONE', ( #25952 ), #808, .F. ) ;
#9550=CARTESIAN_POINT ( 'NONE',  ( -30.00000337463119848, -69.28203230275522628, 17.49999999999999645 ) ) ;
#9551=ORIENTED_EDGE ( 'NONE', *, *, #35104, .T. ) ;
#9552=VERTEX_POINT ( 'NONE', #20882 ) ;
#9553=CIRCLE ( 'NONE', #34696, 2.000000000000001776 ) ;
#9554=ORIENTED_EDGE ( 'NONE', *, *, #25927, .T. ) ;
#9555=ORIENTED_EDGE ( 'NONE', *, *, #12389, .F. ) ;
#9556=AXIS2_PLACEMENT_3D ( 'NONE', #1416, #35747, #4619 ) ;
#9557=ORIENTED_EDGE ( 'NONE', *, *, #8140, .T. ) ;
#9558=DIRECTION ( 'NONE',  ( 1.000000000000000000, 0.000000000000000000, 0.000000000000000000 ) ) ;
#9559=ADVANCED_FACE ( 'NONE', ( #23336 ), #20678, .F. ) ;
#9560=DIRECTION ( 'NONE',  ( 1.000000000000000000, 0.000000000000000000, 0.000000000000000000 ) ) ;
#9561=ORIENTED_EDGE ( 'NONE', *, *, #9309, .T. ) ;
#9562=CARTESIAN_POINT ( 'NONE',  ( -10.00000337463128730, 69.28203230275516944, -5.000000000000000000 ) ) ;
#9564=AXIS2_PLACEMENT_3D ( 'NONE', #9410, #20846, #33961 ) ;
#9565=CARTESIAN_POINT ( 'NONE',  ( -85.00000337463092137, 8.660254037844389075, -5.000000000000000000 ) ) ;
#9566=EDGE_LOOP ( 'NONE', ( #35339, #1201 ) ) ;
#9567=DIRECTION ( 'NONE',  ( 1.000000000000000000, 0.000000000000000000, 0.000000000000000000 ) ) ;
#9568=CARTESIAN_POINT ( 'NONE',  ( -22.00000337463122690, 86.60254037844397601, -9.999999999999998224 ) ) ;
#9570=DIRECTION ( 'NONE',  ( 0.000000000000000000, 0.000000000000000000, 1.000000000000000000 ) ) ;
#9571=ORIENTED_EDGE ( 'NONE', *, *, #14257, .T. ) ;
#9572=CARTESIAN_POINT ( 'NONE',  ( -83.00000337463092137, 25.98076211353317433, -9.999999999999998224 ) ) ;
#9573=AXIS2_PLACEMENT_3D ( 'NONE', #28811, #33717, #33900 ) ;
#9574=CARTESIAN_POINT ( 'NONE',  ( 47.99999662536846756, -69.28203230275519786, -9.999999999999998224 ) ) ;
#9575=ORIENTED_EDGE ( 'NONE', *, *, #21476, .T. ) ;
#9576=EDGE_CURVE ( 'NONE', #30221, #32244, #18968, .T. ) ;
#9579=EDGE_CURVE ( 'NONE', #2310, #32307, #5183, .T. ) ;
#9582=DIRECTION ( 'NONE',  ( 0.000000000000000000, 0.000000000000000000, 1.000000000000000000 ) ) ;
#9583=ORIENTED_EDGE ( 'NONE', *, *, #9680, .T. ) ;
#9584=CIRCLE ( 'NONE', #16769, 2.000000000000001776 ) ;
#9587=CARTESIAN_POINT ( 'NONE',  ( -47.00000337463111322, -77.94228634059960825, -5.000000000000000000 ) ) ;
#9588=ORIENTED_EDGE ( 'NONE', *, *, #9951, .T. ) ;
#9589=AXIS2_PLACEMENT_3D ( 'NONE', #23484, #23309, #31728 ) ;
#9590=ADVANCED_FACE ( 'NONE', ( #3456 ), #14889, .F. ) ;
#9591=DIRECTION ( 'NONE',  ( -1.000000000000000000, 0.000000000000000000, 0.000000000000000000 ) ) ;
#9593=VERTEX_POINT ( 'NONE', #20330 ) ;
#9594=CARTESIAN_POINT ( 'NONE',  ( 26.97173338359068850, -77.60724282659606388, -5.000000000000000000 ) ) ;
#9596=EDGE_CURVE ( 'NONE', #30141, #19642, #17175, .T. ) ;
#9597=AXIS2_PLACEMENT_3D ( 'NONE', #3336, #887, #12305 ) ;
#9598=DIRECTION ( 'NONE',  ( 0.000000000000000000, 0.000000000000000000, -1.000000000000000000 ) ) ;
#9599=EDGE_LOOP ( 'NONE', ( #35243, #24708, #18766, #18733 ) ) ;
#9600=ORIENTED_EDGE ( 'NONE', *, *, #19863, .T. ) ;
#9601=AXIS2_PLACEMENT_3D ( 'NONE', #24124, #27293, #4258 ) ;
#9602=LINE ( 'NONE', #34746, #18510 ) ;
#9604=CARTESIAN_POINT ( 'NONE',  ( 0.000000000000000000, 0.000000000000000000, -5.000000000000000000 ) ) ;
#9607=DIRECTION ( 'NONE',  ( 1.000000000000000000, 0.000000000000000000, 0.000000000000000000 ) ) ;
#9608=DIRECTION ( 'NONE',  ( 1.000000000000000000, 0.000000000000000000, 0.000000000000000000 ) ) ;
#9610=VERTEX_POINT ( 'NONE', #21794 ) ;
#9611=DIRECTION ( 'NONE',  ( 0.000000000000000000, 0.000000000000000000, 1.000000000000000000 ) ) ;
#9612=EDGE_CURVE ( 'NONE', #26170, #12792, #21958, .T. ) ;
#9613=CARTESIAN_POINT ( 'NONE',  ( -70.00000337463099243, -2.428612866367529932E-14, 17.49999999999999645 ) ) ;
#9614=AXIS2_PLACEMENT_3D ( 'NONE', #30165, #35626, #29992 ) ;
#9615=DIRECTION ( 'NONE',  ( 1.000000000000000000, 0.000000000000000000, 0.000000000000000000 ) ) ;
#9617=LINE ( 'NONE', #18216, #16648 ) ;
#9618=CARTESIAN_POINT ( 'NONE',  ( 22.99999662536859901, -77.94228634059960825, 17.49999999999999645 ) ) ;
#9619=AXIS2_PLACEMENT_3D ( 'NONE', #7864, #1675, #2032 ) ;
#9620=LINE ( 'NONE', #9224, #20976 ) ;
#9621=ORIENTED_EDGE ( 'NONE', *, *, #35748, .F. ) ;
#9623=EDGE_LOOP ( 'NONE', ( #19320, #27549, #18897, #18229, #3289 ) ) ;
#9624=EDGE_CURVE ( 'NONE', #32853, #20212, #8178, .T. ) ;
#9625=CARTESIAN_POINT ( 'NONE',  ( -35.83991598322101169, -56.52018970185248037, -49.22241343995298024 ) ) ;
#9626=CARTESIAN_POINT ( 'NONE',  ( -85.00000337463092137, -25.98076211353322051, -9.999999999999998224 ) ) ;
#9627=EDGE_CURVE ( 'NONE', #745, #11213, #1548, .T. ) ;
#9628=DIRECTION ( 'NONE',  ( 1.000000000000000000, 0.000000000000000000, 0.000000000000000000 ) ) ;
#9629=ORIENTED_EDGE ( 'NONE', *, *, #7302, .F. ) ;
#9630=EDGE_LOOP ( 'NONE', ( #32891, #31899 ) ) ;
#9631=VERTEX_POINT ( 'NONE', #32673 ) ;
#9632=CYLINDRICAL_SURFACE ( 'NONE', #29039, 2.000000000000001776 ) ;
#9634=ORIENTED_EDGE ( 'NONE', *, *, #33516, .F. ) ;
#9635=DIRECTION ( 'NONE',  ( 1.000000000000000000, 0.000000000000000000, 0.000000000000000000 ) ) ;
#9637=EDGE_LOOP ( 'NONE', ( #28683, #16996, #12678, #28604 ) ) ;
#9638=SURFACE_STYLE_FILL_AREA ( #29487 ) ;
#9639=CARTESIAN_POINT ( 'NONE',  ( 31.27962116909600709, -62.97617850287780072, -49.86561046011506448 ) ) ;
#9640=EDGE_CURVE ( 'NONE', #36079, #18409, #36918, .T. ) ;
#9641=CARTESIAN_POINT ( 'NONE',  ( -86.45172111230354517, 31.46585318596159553, 12.49999999999999822 ) ) ;
#9642=ORIENTED_EDGE ( 'NONE', *, *, #13544, .F. ) ;
#9644=DIRECTION ( 'NONE',  ( 1.000000000000000000, 0.000000000000000000, 0.000000000000000000 ) ) ;
#9645=CARTESIAN_POINT ( 'NONE',  ( 16.99999662536859901, 77.94228634059957983, 12.50000000000000000 ) ) ;
#9646=DIRECTION ( 'NONE',  ( 1.000000000000000000, 0.000000000000000000, 0.000000000000000000 ) ) ;
#9648=ORIENTED_EDGE ( 'NONE', *, *, #2319, .F. ) ;
#9649=DIRECTION ( 'NONE',  ( 0.5000000000000038858, 0.8660254037844362651, 0.000000000000000000 ) ) ;
#9651=VERTEX_POINT ( 'NONE', #26882 ) ;
#9652=CARTESIAN_POINT ( 'NONE',  ( 4.999996625368676284, -77.94228634059960825, 12.50000000000000000 ) ) ;
#9653=PLANE ( 'NONE',  #5826 ) ;
#9654=DIRECTION ( 'NONE',  ( -1.000000000000000000, 0.000000000000000000, 0.000000000000000000 ) ) ;
#9656=EDGE_CURVE ( 'NONE', #13843, #9593, #4600, .T. ) ;
#9657=DIRECTION ( 'NONE',  ( 1.000000000000000000, 0.000000000000000000, 0.000000000000000000 ) ) ;
#9658=DIRECTION ( 'NONE',  ( 1.000000000000000000, 0.000000000000000000, 0.000000000000000000 ) ) ;
#9659=ORIENTED_EDGE ( 'NONE', *, *, #25883, .F. ) ;
#9660=ADVANCED_FACE ( 'NONE', ( #24633 ), #6800, .F. ) ;
#9661=PLANE ( 'NONE',  #11200 ) ;
#9662=CIRCLE ( 'NONE', #28232, 1.999999999999998224 ) ;
#9664=CARTESIAN_POINT ( 'NONE',  ( 36.99999662536855283, -60.62177826491080168, 17.49999999999999645 ) ) ;
#9665=ORIENTED_EDGE ( 'NONE', *, *, #31119, .T. ) ;
#9666=EDGE_CURVE ( 'NONE', #18360, #34031, #14165, .T. ) ;
#9667=EDGE_LOOP ( 'NONE', ( #25694, #4186 ) ) ;
#9668=VERTEX_POINT ( 'NONE', #24067 ) ;
#9669=PLANE ( 'NONE',  #31380 ) ;
#9672=CARTESIAN_POINT ( 'NONE',  ( -27.78182860042817026, -56.67878100130359087, 12.49999999999999822 ) ) ;
#9673=EDGE_CURVE ( 'NONE', #8255, #35883, #21627, .T. ) ;
#9675=CARTESIAN_POINT ( 'NONE',  ( 19.99999662536861678, -86.60254037844400443, -5.000000000000000000 ) ) ;
#9677=CARTESIAN_POINT ( 'NONE',  ( 56.99999662536844625, 43.30127018922198801, -9.999999999999998224 ) ) ;
#9678=ORIENTED_EDGE ( 'NONE', *, *, #8192, .T. ) ;
#9679=FACE_BOUND ( 'NONE', #1897, .T. ) ;
#9680=EDGE_CURVE ( 'NONE', #2691, #14791, #36952, .T. ) ;
#9681=EDGE_CURVE ( 'NONE', #1135, #3002, #33956, .T. ) ;
#9682=CARTESIAN_POINT ( 'NONE',  ( -70.00000337463099243, 17.32050807568877460, 17.49999999999999645 ) ) ;
#9683=LINE ( 'NONE', #35397, #12540 ) ;
#9684=EDGE_CURVE ( 'NONE', #26423, #34827, #18236, .T. ) ;
#9685=CIRCLE ( 'NONE', #8502, 2.000000000000001776 ) ;
#9686=EDGE_CURVE ( 'NONE', #6350, #25578, #12374, .T. ) ;
#9687=DIRECTION ( 'NONE',  ( 0.000000000000000000, 0.000000000000000000, 1.000000000000000000 ) ) ;
#9690=AXIS2_PLACEMENT_3D ( 'NONE', #28876, #31698, #31861 ) ;
#9691=CARTESIAN_POINT ( 'NONE',  ( 56.99999662536844625, -60.62177826491080168, -9.999999999999998224 ) ) ;
#9692=CARTESIAN_POINT ( 'NONE',  ( 83.67710222720857871, -27.48074558388131905, 12.50000000000000000 ) ) ;
#9693=DIRECTION ( 'NONE',  ( 1.000000000000000000, 0.000000000000000000, 0.000000000000000000 ) ) ;
#9694=ORIENTED_EDGE ( 'NONE', *, *, #16503, .T. ) ;
#9695=DIRECTION ( 'NONE',  ( 0.000000000000000000, 0.000000000000000000, 1.000000000000000000 ) ) ;
#9697=DIRECTION ( 'NONE',  ( -0.000000000000000000, -0.000000000000000000, 1.000000000000000000 ) ) ;
#9698=ORIENTED_EDGE ( 'NONE', *, *, #27109, .F. ) ;
#9699=EDGE_LOOP ( 'NONE', ( #31458, #8073, #10912, #142 ) ) ;
#9700=ORIENTED_EDGE ( 'NONE', *, *, #32932, .T. ) ;
#9702=DIRECTION ( 'NONE',  ( -1.000000000000000000, 0.000000000000000000, 0.000000000000000000 ) ) ;
#9704=CIRCLE ( 'NONE', #24081, 2.000000000000001776 ) ;
#9705=DIRECTION ( 'NONE',  ( -1.000000000000000000, 0.000000000000000000, -0.000000000000000000 ) ) ;
#9706=CARTESIAN_POINT ( 'NONE',  ( 46.99999662536849598, 60.62177826491077326, 17.49999999999999645 ) ) ;
#9707=CARTESIAN_POINT ( 'NONE',  ( 39.99999662536853151, -69.28203230275519786, 17.49999999999999645 ) ) ;
#9708=EDGE_LOOP ( 'NONE', ( #3724, #13029 ) ) ;
#9710=DIRECTION ( 'NONE',  ( 0.000000000000000000, 0.000000000000000000, 1.000000000000000000 ) ) ;
#9711=CARTESIAN_POINT ( 'NONE',  ( -33.99999999999945288, 58.88972745734214698, 12.49999999999999822 ) ) ;
#9712=ORIENTED_EDGE ( 'NONE', *, *, #26850, .T. ) ;
#9714=ORIENTED_EDGE ( 'NONE', *, *, #13793, .T. ) ;
#9715=FACE_BOUND ( 'NONE', #28586, .T. ) ;
#9716=EDGE_LOOP ( 'NONE', ( #34718, #33781 ) ) ;
#9717=ORIENTED_EDGE ( 'NONE', *, *, #21432, .F. ) ;
#9718=ADVANCED_FACE ( 'NONE', ( #9992, #18635, #30050, #4371, #15804, #12984, #35885, #33054, #7369 ), #30227, .F. ) ;
#9719=CARTESIAN_POINT ( 'NONE',  ( 69.99999662536839651, -17.32050807568879947, -9.999999999999998224 ) ) ;
#9720=ORIENTED_EDGE ( 'NONE', *, *, #28400, .F. ) ;
#9721=PLANE ( 'NONE',  #23635 ) ;
#9722=CIRCLE ( 'NONE', #30679, 2.000000000000001776 ) ;
#9723=LINE ( 'NONE', #17106, #17927 ) ;
#9725=EDGE_LOOP ( 'NONE', ( #31498, #479 ) ) ;
#9726=VERTEX_POINT ( 'NONE', #5655 ) ;
#9727=EDGE_LOOP ( 'NONE', ( #7912, #16455, #804, #2297 ) ) ;
#9728=EDGE_LOOP ( 'NONE', ( #27335, #11451 ) ) ;
#9729=VERTEX_POINT ( 'NONE', #33622 ) ;
#9730=DIRECTION ( 'NONE',  ( 0.000000000000000000, 0.000000000000000000, -1.000000000000000000 ) ) ;
#9731=DIRECTION ( 'NONE',  ( 1.000000000000000000, 0.000000000000000000, 0.000000000000000000 ) ) ;
#9732=ORIENTED_EDGE ( 'NONE', *, *, #30723, .F. ) ;
#9733=CARTESIAN_POINT ( 'NONE',  ( -37.00000337463116296, 77.94228634059957983, 17.49999999999999645 ) ) ;
#9735=CYLINDRICAL_SURFACE ( 'NONE', #18385, 2.000000000000001776 ) ;
#9736=EDGE_CURVE ( 'NONE', #22407, #1861, #19360, .T. ) ;
#9737=EDGE_LOOP ( 'NONE', ( #4114, #18839, #36151 ) ) ;
#9738=CYLINDRICAL_SURFACE ( 'NONE', #21233, 2.000000000000001776 ) ;
#9739=EDGE_CURVE ( 'NONE', #30643, #26836, #28561, .T. ) ;
#9740=PLANE ( 'NONE',  #14404 ) ;
#9743=FACE_OUTER_BOUND ( 'NONE', #21618, .T. ) ;
#9744=DIRECTION ( 'NONE',  ( 0.000000000000000000, 0.000000000000000000, 1.000000000000000000 ) ) ;
#9745=ORIENTED_EDGE ( 'NONE', *, *, #30074, .F. ) ;
#9746=ORIENTED_EDGE ( 'NONE', *, *, #31394, .T. ) ;
#9747=ADVANCED_FACE ( 'NONE', ( #28171 ), #36986, .F. ) ;
#9748=CARTESIAN_POINT ( 'NONE',  ( 54.99999662536844625, 43.30127018922198801, 17.49999999999999645 ) ) ;
#9749=CIRCLE ( 'NONE', #36126, 2.000000000000001776 ) ;
#9750=DIRECTION ( 'NONE',  ( 0.000000000000000000, 0.000000000000000000, 1.000000000000000000 ) ) ;
#9751=DIRECTION ( 'NONE',  ( 1.000000000000000000, 0.000000000000000000, 0.000000000000000000 ) ) ;
#9752=VECTOR ( 'NONE', #13214, 1000.000000000000000 ) ;
#9755=CARTESIAN_POINT ( 'NONE',  ( -44.13139720814439215, -27.49999999999955591, -10.00000000000000000 ) ) ;
#9756=DIRECTION ( 'NONE',  ( 0.000000000000000000, 0.000000000000000000, 1.000000000000000000 ) ) ;
#9757=ORIENTED_EDGE ( 'NONE', *, *, #6127, .F. ) ;
#9758=EDGE_CURVE ( 'NONE', #15480, #4621, #35752, .T. ) ;
#9759=LINE ( 'NONE', #15952, #35169 ) ;
#9760=AXIS2_PLACEMENT_3D ( 'NONE', #8513, #25944, #14506 ) ;
#9761=VERTEX_POINT ( 'NONE', #36788 ) ;
#9762=DIRECTION ( 'NONE',  ( -1.000000000000000000, 0.000000000000000000, 0.000000000000000000 ) ) ;
#9763=AXIS2_PLACEMENT_3D ( 'NONE', #14627, #23454, #378 ) ;
#9764=CARTESIAN_POINT ( 'NONE',  ( -19.13981058454750794, 60.93295298010998806, 12.49999999999999822 ) ) ;
#9766=ORIENTED_EDGE ( 'NONE', *, *, #13693, .F. ) ;
#9767=ORIENTED_EDGE ( 'NONE', *, *, #3341, .T. ) ;
#9769=CARTESIAN_POINT ( 'NONE',  ( -4.279621169095561228, 62.97617850287782915, -4.999999999999997335 ) ) ;
#9770=AXIS2_PLACEMENT_3D ( 'NONE', #3238, #5885, #11116 ) ;
#9771=EDGE_CURVE ( 'NONE', #7161, #29318, #12980, .T. ) ;
#9772=DIRECTION ( 'NONE',  ( 1.000000000000000000, 0.000000000000000000, 0.000000000000000000 ) ) ;
#9773=FACE_OUTER_BOUND ( 'NONE', #21956, .T. ) ;
#9774=DIRECTION ( 'NONE',  ( -1.000000000000000000, 2.210166206429708225E-14, 0.000000000000000000 ) ) ;
#9775=FACE_OUTER_BOUND ( 'NONE', #5707, .T. ) ;
#9776=VERTEX_POINT ( 'NONE', #8311 ) ;
#9778=CARTESIAN_POINT ( 'NONE',  ( 54.99999662536844625, 60.62177826491077326, -5.000000000000000000 ) ) ;
#9779=CARTESIAN_POINT ( 'NONE',  ( 66.99999662536842493, 43.30127018922200222, -9.999999999999998224 ) ) ;
#9780=ORIENTED_EDGE ( 'NONE', *, *, #29396, .F. ) ;
#9781=CARTESIAN_POINT ( 'NONE',  ( 64.99999662536841072, -25.98076211353320275, -9.999999999999998224 ) ) ;
#9783=CARTESIAN_POINT ( 'NONE',  ( -70.00000337463099243, 51.96152422706637708, -9.999999999999998224 ) ) ;
#9784=CIRCLE ( 'NONE', #34957, 2.000000000000001776 ) ;
#9785=DIRECTION ( 'NONE',  ( 0.000000000000000000, 0.000000000000000000, 1.000000000000000000 ) ) ;
#9786=ORIENTED_EDGE ( 'NONE', *, *, #4171, .F. ) ;
#9788=VERTEX_POINT ( 'NONE', #5110 ) ;
#9789=ADVANCED_FACE ( 'NONE', ( #4927 ), #13739, .T. ) ;
#9790=DIRECTION ( 'NONE',  ( 0.000000000000000000, 0.000000000000000000, 1.000000000000000000 ) ) ;
#9791=DIRECTION ( 'NONE',  ( 1.000000000000000000, 0.000000000000000000, 0.000000000000000000 ) ) ;
#9793=ORIENTED_EDGE ( 'NONE', *, *, #16218, .T. ) ;
#9794=EDGE_LOOP ( 'NONE', ( #22042, #17425, #27504 ) ) ;
#9795=ORIENTED_EDGE ( 'NONE', *, *, #16263, .T. ) ;
#9796=AXIS2_PLACEMENT_3D ( 'NONE', #34353, #8655, #14474 ) ;
#9797=DIRECTION ( 'NONE',  ( 1.000000000000000000, 0.000000000000000000, 0.000000000000000000 ) ) ;
#9798=CIRCLE ( 'NONE', #30755, 33.00000000000001421 ) ;
#9799=ORIENTED_EDGE ( 'NONE', *, *, #2974, .T. ) ;
#9801=DIRECTION ( 'NONE',  ( 0.000000000000000000, 0.000000000000000000, 1.000000000000000000 ) ) ;
#9802=ORIENTED_EDGE ( 'NONE', *, *, #23165, .F. ) ;
#9803=VECTOR ( 'NONE', #28958, 1000.000000000000000 ) ;
#9804=ORIENTED_EDGE ( 'NONE', *, *, #22968, .T. ) ;
#9805=EDGE_CURVE ( 'NONE', #12474, #35136, #34184, .T. ) ;
#9806=CARTESIAN_POINT ( 'NONE',  ( -35.19434990244938888, 52.39915983220783602, 12.49999999999999822 ) ) ;
#9808=ORIENTED_EDGE ( 'NONE', *, *, #13967, .F. ) ;
#9809=EDGE_LOOP ( 'NONE', ( #24748, #31427, #14540, #18811, #33513 ) ) ;
#9810=DIRECTION ( 'NONE',  ( 1.000000000000000000, 0.000000000000000000, 0.000000000000000000 ) ) ;
#9811=CARTESIAN_POINT ( 'NONE',  ( 53.72396900529356145, 62.16182810592437846, -5.000000000000000000 ) ) ;
#9813=DIRECTION ( 'NONE',  ( 0.000000000000000000, 0.000000000000000000, 1.000000000000000000 ) ) ;
#9814=CARTESIAN_POINT ( 'NONE',  ( -12.00000337463127842, -69.28203230275519786, 17.49999999999999645 ) ) ;
#9815=AXIS2_PLACEMENT_3D ( 'NONE', #10436, #21875, #24138 ) ;
#9816=VERTEX_POINT ( 'NONE', #28336 ) ;
#9818=ADVANCED_FACE ( 'NONE', ( #25194 ), #21991, .F. ) ;
#9819=EDGE_LOOP ( 'NONE', ( #29770, #7291, #29920, #18450 ) ) ;
#9820=DIRECTION ( 'NONE',  ( 0.000000000000000000, 0.000000000000000000, 1.000000000000000000 ) ) ;
#9821=CARTESIAN_POINT ( 'NONE',  ( -25.00000337463120914, 77.94228634059957983, -9.999999999999998224 ) ) ;
#9822=DIRECTION ( 'NONE',  ( -0.000000000000000000, -0.000000000000000000, -1.000000000000000000 ) ) ;
#9823=DIRECTION ( 'NONE',  ( 0.4999999999999919509, -0.8660254037844433705, 0.000000000000000000 ) ) ;
#9824=AXIS2_PLACEMENT_3D ( 'NONE', #29447, #1153, #3766 ) ;
#9826=AXIS2_PLACEMENT_3D ( 'NONE', #4135, #569, #35066 ) ;
#9827=CARTESIAN_POINT ( 'NONE',  ( -82.00000337463094979, -2.404119930384582903E-14, -9.999999999999998224 ) ) ;
#9828=VERTEX_POINT ( 'NONE', #19196 ) ;
#9829=CARTESIAN_POINT ( 'NONE',  ( 90.60231327712337190, 15.97563234535636134, -49.86561046011506448 ) ) ;
#9830=DIRECTION ( 'NONE',  ( -1.000000000000000000, 0.000000000000000000, 0.000000000000000000 ) ) ;
#9831=DIRECTION ( 'NONE',  ( 0.000000000000000000, 0.000000000000000000, 1.000000000000000000 ) ) ;
#9832=EDGE_LOOP ( 'NONE', ( #1099, #34502, #13135, #24131 ) ) ;
#9837=PLANE ( 'NONE',  #3261 ) ;
#9839=EDGE_LOOP ( 'NONE', ( #32782, #16693 ) ) ;
#9840=AXIS2_PLACEMENT_3D ( 'NONE', #2291, #32713, #4239 ) ;
#9842=CARTESIAN_POINT ( 'NONE',  ( -80.00000337463094979, 34.64101615137757051, -9.999999999999998224 ) ) ;
#9843=ORIENTED_EDGE ( 'NONE', *, *, #4365, .F. ) ;
#9844=CARTESIAN_POINT ( 'NONE',  ( 34.99999662536855283, -77.94228634059960825, 12.50000000000000000 ) ) ;
#9845=ORIENTED_EDGE ( 'NONE', *, *, #36005, .F. ) ;
#9846=CARTESIAN_POINT ( 'NONE',  ( -18.00000337463123046, 86.60254037844397601, 12.50000000000000000 ) ) ;
#9847=CIRCLE ( 'NONE', #34406, 2.000000000000001776 ) ;
#9848=AXIS2_PLACEMENT_3D ( 'NONE', #9150, #26414, #8440 ) ;
#9849=ADVANCED_FACE ( 'NONE', ( #31333, #2102, #24809, #36241, #10550, #13540, #22184 ), #25002, .F. ) ;
#9851=CARTESIAN_POINT ( 'NONE',  ( -15.97563234535668109, 90.60231327712331506, -4.999999999999997335 ) ) ;
#9852=CIRCLE ( 'NONE', #11052, 2.000000000000001776 ) ;
#9854=EDGE_CURVE ( 'NONE', #17617, #20586, #14776, .T. ) ;
#9856=DIRECTION ( 'NONE',  ( -1.000000000000000000, 0.000000000000000000, 0.000000000000000000 ) ) ;
#9858=EDGE_CURVE ( 'NONE', #17340, #30760, #35085, .T. ) ;
#9859=DIRECTION ( 'NONE',  ( 0.000000000000000000, 0.000000000000000000, 1.000000000000000000 ) ) ;
#9860=VECTOR ( 'NONE', #26193, 1000.000000000000000 ) ;
#9861=FACE_BOUND ( 'NONE', #631, .T. ) ;
#9862=DIRECTION ( 'NONE',  ( -1.000000000000000000, 0.000000000000000000, 0.000000000000000000 ) ) ;
#9863=ORIENTED_EDGE ( 'NONE', *, *, #26805, .F. ) ;
#9865=AXIS2_PLACEMENT_3D ( 'NONE', #3736, #6918, #20990 ) ;
#9866=EDGE_CURVE ( 'NONE', #17624, #8845, #10611, .T. ) ;
#9867=DIRECTION ( 'NONE',  ( 1.000000000000000000, 0.000000000000000000, 0.000000000000000000 ) ) ;
#9868=DIRECTION ( 'NONE',  ( 0.000000000000000000, 0.000000000000000000, -1.000000000000000000 ) ) ;
#9869=EDGE_CURVE ( 'NONE', #22214, #13783, #9392, .T. ) ;
#9871=AXIS2_PLACEMENT_3D ( 'NONE', #8637, #2851, #14458 ) ;
#9872=ORIENTED_EDGE ( 'NONE', *, *, #9627, .F. ) ;
#9873=EDGE_LOOP ( 'NONE', ( #17831, #15098 ) ) ;
#9874=CARTESIAN_POINT ( 'NONE',  ( 13.89091430021463935, 62.33939050065170306, 12.49999999999999822 ) ) ;
#9875=DIRECTION ( 'NONE',  ( 1.000000000000000000, 0.000000000000000000, 0.000000000000000000 ) ) ;
#9876=ADVANCED_FACE ( 'NONE', ( #28722 ), #6591, .F. ) ;
#9877=CIRCLE ( 'NONE', #5094, 2.000000000000000000 ) ;
#9878=EDGE_CURVE ( 'NONE', #12035, #21455, #31551, .T. ) ;
#9879=DIRECTION ( 'NONE',  ( 0.000000000000000000, 0.000000000000000000, -1.000000000000000000 ) ) ;
#9880=ORIENTED_EDGE ( 'NONE', *, *, #23634, .T. ) ;
#9881=EDGE_CURVE ( 'NONE', #10138, #23997, #11765, .T. ) ;
#9882=EDGE_CURVE ( 'NONE', #35412, #15350, #36370, .T. ) ;
#9883=CARTESIAN_POINT ( 'NONE',  ( 74.99999662536836809, 43.30127018922198801, -9.999999999999998224 ) ) ;
#9884=DIRECTION ( 'NONE',  ( -1.000000000000000000, 0.000000000000000000, 0.000000000000000000 ) ) ;
#9887=ORIENTED_EDGE ( 'NONE', *, *, #34978, .T. ) ;
#9888=EDGE_LOOP ( 'NONE', ( #34938, #4416, #29477, #26353 ) ) ;
#9889=FACE_OUTER_BOUND ( 'NONE', #3716, .T. ) ;
#9890=FACE_OUTER_BOUND ( 'NONE', #3015, .T. ) ;
#9891=VERTEX_POINT ( 'NONE', #25904 ) ;
#9892=AXIS2_PLACEMENT_3D ( 'NONE', #467, #32337, #26904 ) ;
#9893=DIRECTION ( 'NONE',  ( 0.000000000000000000, 0.000000000000000000, -1.000000000000000000 ) ) ;
#9894=EDGE_LOOP ( 'NONE', ( #27358, #29494, #11686 ) ) ;
#9895=LINE ( 'NONE', #24342, #33311 ) ;
#9896=AXIS2_PLACEMENT_3D ( 'NONE', #26223, #9710, #29561 ) ;
#9897=FACE_BOUND ( 'NONE', #14378, .T. ) ;
#9898=EDGE_LOOP ( 'NONE', ( #8733, #12983, #19747, #10145 ) ) ;
#9900=DIRECTION ( 'NONE',  ( 1.000000000000000000, 0.000000000000000000, 0.000000000000000000 ) ) ;
#9901=EDGE_LOOP ( 'NONE', ( #17087, #4078, #7981, #23834 ) ) ;
#9902=AXIS2_PLACEMENT_3D ( 'NONE', #17928, #15102, #23542 ) ;
#9903=AXIS2_PLACEMENT_3D ( 'NONE', #27837, #16965, #22404 ) ;
#9904=AXIS2_PLACEMENT_3D ( 'NONE', #13419, #19085, #16084 ) ;
#9906=DIRECTION ( 'NONE',  ( 1.000000000000000000, 0.000000000000000000, 0.000000000000000000 ) ) ;
#9909=DIRECTION ( 'NONE',  ( 1.000000000000000000, 0.000000000000000000, 0.000000000000000000 ) ) ;
#9910=ORIENTED_EDGE ( 'NONE', *, *, #9656, .F. ) ;
#9912=ORIENTED_EDGE ( 'NONE', *, *, #27420, .F. ) ;
#9913=CIRCLE ( 'NONE', #2156, 2.000000000000001776 ) ;
#9914=DIRECTION ( 'NONE',  ( 0.000000000000000000, 0.000000000000000000, 1.000000000000000000 ) ) ;
#9915=CARTESIAN_POINT ( 'NONE',  ( 76.99999662536836809, 43.30127018922198801, -9.999999999999998224 ) ) ;
#9916=ORIENTED_EDGE ( 'NONE', *, *, #32297, .F. ) ;
#9917=AXIS2_PLACEMENT_3D ( 'NONE', #2886, #14316, #28743 ) ;
#9919=CIRCLE ( 'NONE', #23713, 2.000000000000000000 ) ;
#9920=FACE_OUTER_BOUND ( 'NONE', #3993, .T. ) ;
#9921=AXIS2_PLACEMENT_3D ( 'NONE', #27977, #19547, #2485 ) ;
#9922=ORIENTED_EDGE ( 'NONE', *, *, #28649, .T. ) ;
#9923=AXIS2_PLACEMENT_3D ( 'NONE', #12471, #32527, #15848 ) ;
#9925=VECTOR ( 'NONE', #33698, 1000.000000000000000 ) ;
#9929=CARTESIAN_POINT ( 'NONE',  ( -33.00000337463116296, 77.94228634059957983, -5.000000000000000000 ) ) ;
#9931=DIRECTION ( 'NONE',  ( 0.000000000000000000, 0.000000000000000000, 1.000000000000000000 ) ) ;
#9932=DIRECTION ( 'NONE',  ( 0.000000000000000000, 0.000000000000000000, -1.000000000000000000 ) ) ;
#9934=AXIS2_PLACEMENT_3D ( 'NONE', #18714, #27527, #16282 ) ;
#9935=ORIENTED_EDGE ( 'NONE', *, *, #17611, .F. ) ;
#9936=DIRECTION ( 'NONE',  ( 1.000000000000000000, 0.000000000000000000, 0.000000000000000000 ) ) ;
#9937=DIRECTION ( 'NONE',  ( -1.000000000000000000, 0.000000000000000000, 0.000000000000000000 ) ) ;
#9938=CARTESIAN_POINT ( 'NONE',  ( -37.00000337463116296, -60.62177826491080168, -5.000000000000000000 ) ) ;
#9940=ORIENTED_EDGE ( 'NONE', *, *, #19072, .T. ) ;
#9942=AXIS2_PLACEMENT_3D ( 'NONE', #12060, #29141, #28945 ) ;
#9943=DIRECTION ( 'NONE',  ( -1.000000000000000000, 0.000000000000000000, 0.000000000000000000 ) ) ;
#9945=VECTOR ( 'NONE', #30026, 1000.000000000000000 ) ;
#9947=DIRECTION ( 'NONE',  ( -0.000000000000000000, -0.000000000000000000, 1.000000000000000000 ) ) ;
#9948=ORIENTED_EDGE ( 'NONE', *, *, #28219, .T. ) ;
#9951=EDGE_CURVE ( 'NONE', #15962, #29981, #16583, .T. ) ;
#9952=DIRECTION ( 'NONE',  ( 0.000000000000000000, 0.000000000000000000, 1.000000000000000000 ) ) ;
#9954=FACE_OUTER_BOUND ( 'NONE', #32291, .T. ) ;
#9955=AXIS2_PLACEMENT_3D ( 'NONE', #8223, #4864, #5226 ) ;
#9956=DIRECTION ( 'NONE',  ( 0.000000000000000000, 0.000000000000000000, 1.000000000000000000 ) ) ;
#9957=ORIENTED_EDGE ( 'NONE', *, *, #4506, .T. ) ;
#9959=EDGE_CURVE ( 'NONE', #25333, #33312, #3595, .T. ) ;
#9960=ORIENTED_EDGE ( 'NONE', *, *, #34747, .T. ) ;
#9961=DIRECTION ( 'NONE',  ( 0.000000000000000000, 0.000000000000000000, 1.000000000000000000 ) ) ;
#9963=DIRECTION ( 'NONE',  ( 1.000000000000000000, 0.000000000000000000, 0.000000000000000000 ) ) ;
#9967=LINE ( 'NONE', #19174, #10451 ) ;
#9968=AXIS2_PLACEMENT_3D ( 'NONE', #604, #28737, #23103 ) ;
#9969=CARTESIAN_POINT ( 'NONE',  ( 4.220257619726806020, 79.78402657284750887, 12.50000000000000000 ) ) ;
#9970=AXIS2_PLACEMENT_3D ( 'NONE', #3375, #14811, #26251 ) ;
#9971=EDGE_CURVE ( 'NONE', #12428, #5388, #395, .T. ) ;
#9973=DIRECTION ( 'NONE',  ( -0.000000000000000000, -0.000000000000000000, 1.000000000000000000 ) ) ;
#9975=CYLINDRICAL_SURFACE ( 'NONE', #20755, 27.00000000000001421 ) ;
#9976=CIRCLE ( 'NONE', #14764, 2.000000000000001776 ) ;
#9977=VECTOR ( 'NONE', #24696, 1000.000000000000000 ) ;
#9978=ORIENTED_EDGE ( 'NONE', *, *, #5679, .T. ) ;
#9980=ORIENTED_EDGE ( 'NONE', *, *, #36064, .T. ) ;
#9981=AXIS2_PLACEMENT_3D ( 'NONE', #6694, #9308, #32945 ) ;
#9982=LINE ( 'NONE', #28326, #12697 ) ;
#9983=CYLINDRICAL_SURFACE ( 'NONE', #5587, 2.000000000000001776 ) ;
#9985=ORIENTED_EDGE ( 'NONE', *, *, #7972, .F. ) ;
#9986=VERTEX_POINT ( 'NONE', #15025 ) ;
#9987=ORIENTED_EDGE ( 'NONE', *, *, #1203, .F. ) ;
#9988=DIRECTION ( 'NONE',  ( -1.000000000000000000, 0.000000000000000000, 0.000000000000000000 ) ) ;
#9989=ORIENTED_EDGE ( 'NONE', *, *, #19738, .F. ) ;
#9991=VERTEX_POINT ( 'NONE', #11828 ) ;
#9992=FACE_BOUND ( 'NONE', #22072, .T. ) ;
#9993=VERTEX_POINT ( 'NONE', #760 ) ;
#9994=EDGE_CURVE ( 'NONE', #34620, #8381, #4623, .T. ) ;
#9995=AXIS2_PLACEMENT_3D ( 'NONE', #9604, #12951, #3968 ) ;
#9996=ORIENTED_EDGE ( 'NONE', *, *, #10957, .F. ) ;
#9997=FACE_OUTER_BOUND ( 'NONE', #3194, .T. ) ;
#9998=CIRCLE ( 'NONE', #6408, 2.000000000000000000 ) ;
#9999=CLOSED_SHELL ( 'NONE', ( #35667, #28786, #32791, #17591, #30964, #31218, #29280, #10725, #22495, #18607, #10225, #27325, #27485, #3148, #8996, #24589, #35538, #23841, #22946, #26638, #4191, #16734, #21097, #14097, #17544, #21055, #6169, #29486, #34571, #13784, #9277, #32424, #6388, #1603, #1763, #28680, #22595, #25690, #19671, #9319, #34371, #3050, #20215, #16436, #25737, #32140, #35534, #7151, #34609, #23797, #6379, #25913, #18431, #24293, #10322, #17034, #13775, #24694, #21351, #24401, #27177, #22422, #773, #30232, #9559, #27752, #4392, #22251, #25725, #24661, #36160, #10960, #28940, #5343, #5834, #2701, #24904, #12696, #34164, #23961, #31968, #8466, #21488, #17960, #13033, #25824, #32432, #13887, #14105, #9876, #5312, #13346, #23438, #22801, #32814, #5963, #12847, #8593, #3086, #13898, #8522, #2076, #2371, #29107, #6897, #15018, #17265, #29807, #8939, #7722, #22955, #5516, #33511, #25436, #13350, #36268, #29536, #11825, #14145, #25931, #33917, #34074, #14459, #13724, #29012, #17460, #25014, #34860, #12871, #30215, #1324, #12124, #34735, #14607, #390, #2984, #3848, #10613, #3463, #7753, #1064, #7969, #13943, #947, #14454, #16392, #12782, #3682, #33027, #12180, #28396, #29436, #28528, #9198, #25175, #6235, #14797, #23342, #27958, #12671, #33921, #4847, #33645, #31201, #11108, #10496, #16082, #36568, #1455, #15859, #2732, #36009, #10053, #15235, #3014, #9023, #14625, #26050, #1418, #5672, #10465, #13728, #8266, #1686, #12752, #20019, #32343, #24501, #23572, #16083, #25336, #31777, #20418, #27165, #35346, #29053, #27304, #24920, #27938, #28194, #19765, #22635, #3885, #8410, #33535, #25925, #32775, #7612, #5326, #10684, #20001, #11939, #23589, #26185, #20394, #7021, #9747, #4187, #15317, #26381, #22629, #26173, #16653, #33040, #12122, #26916, #21036, #159, #10413, #3594, #13113, #17571, #10325, #17712, #32681, #30828, #29569, #19665, #5535, #33373, #12335, #24941, #7495, #14975, #33531, #1160, #34421, #35541, #36020, #2777, #32031, #19436, #23605, #14708, #11893, #11019, #36724, #27296, #28669, #10950, #10201, #35888, #756, #3169, #21517, #11172, #30734, #33835, #20075, #29133, #4552, #15169, #14772, #26041, #21733, #1144, #4389, #13449, #12749, #27536, #16514, #4865, #34627, #26025, #2999, #2500, #27591, #21281, #23740, #37021, #3442, #15443, #28634, #5073, #30747, #4853, #5404, #33962, #14690, #7803, #4301, #32542, #34066, #30631, #17777, #33179, #33044, #11636, #25513, #24322, #15655, #8576, #4512, #9849, #9718, #11057, #13307, #23303, #10033, #20865, #9190, #22053, #2345, #17462, #18694, #1194, #1343, #5090, #842, #23853, #15808, #25676, #20555, #21683, #4048, #16895, #25093, #19374, #30652, #24680, #8292, #13502, #32248, #7536, #21256, #35743, #7136, #36943, #35123, #7332, #8450, #14701, #13983, #12411, #32503, #19356, #36416, #17373, #17783, #15337, #16701, #36948, #23260, #35652, #13370, #31460, #24710, #263, #7605, #35226, #9173, #1096, #9165, #29328, #14366, #12816, #4726, #36725, #4386, #2713, #6572, #6470, #33469, #36914, #30895, #25586, #24195, #29993, #31205, #6009, #33397, #30416, #10012, #25402, #26790, #34508, #5309, #10262, #8525, #25846, #1838, #27627, #22029, #15387, #26361, #18825, #21727, #21335, #6919, #25580, #35734, #20454, #34208, #11663, #14416, #25723, #10894, #30939, #29490, #26160, #28054, #25073, #10002, #14008, #15639, #26111, #35708, #30644, #2762, #7286, #12625, #26060, #6541, #10832, #478, #26933, #33244, #14325, #6286, #6771, #5775, #24103, #24602, #35855, #13412, #5693, #17194, #19220, #30134, #22215, #1958, #29717, #9548, #25406, #23190, #3116, #21892, #24670, #30280, #24541, #35327, #24096, #1351, #14000, #19531, #8272, #23186, #6806, #1687, #5224, #14822, #6630, #36060, #9345, #13565, #16925, #3710, #22226, #23323, #25245, #35569, #26035, #28853, #28721, #20983, #15398, #18281, #32357, #27548, #23356, #12506, #23847, #11015, #35600, #18134, #15507, #33272, #32559, #17419, #16470, #16608, #36024, #12927, #23064, #8899, #9590, #28007, #22897, #6114, #33465, #8061, #1501, #30511, #11608, #15034, #13348, #18329, #20899, #25046, #6804, #23225, #28132, #36675, #20946, #36037, #5995, #26575, #25807, #9401, #27897, #8051, #29740, #18870, #6646, #19163, #2775, #17449, #17083, #18934, #16039, #25240, #18625, #1895, #34997, #27805, #9818, #15194, #4452, #34862, #24638, #7079, #18286, #19257, #19913, #33483, #13108, #9660, #29707, #15752, #11139, #31780, #15989, #37070, #7153, #8895, #25053, #32764, #23729, #3621, #26866, #10242, #10144, #4163, #16621, #23110, #32270, #19398, #34326, #10698, #24842, #30944, #8294, #7716, #2549, #1417, #24327, #34783, #17524, #31544, #25615, #10587, #14931, #6766, #5317, #8942, #30411, #14500, #33659, #37099, #8979, #30595, #31823, #8008, #8435, #29206, #3512, #6163, #31678, #17406, #22293, #4588, #27220, #18130, #12541, #31636, #36580, #8341, #28752, #7258, #28009, #10552, #17661, #30485, #7253, #34563, #11928, #9180, #22681, #9304, #1286, #7134, #31284, #11924, #32446, #23026, #5412, #17822, #1161, #17938, #18538, #15611, #26591, #21327, #19279, #19749, #9482, #2554, #21625, #31622, #8479, #10992, #20876, #12632, #33185, #21664, #8961, #27779, #27523, #17291, #27449, #17659, #2486, #31211, #22620, #21214, #27007, #20285, #31158, #14699, #17916, #15951, #6447, #10111, #28220, #34670, #29472, #14486, #28999, #28817, #28353, #7051, #17595, #36250, #17311, #21239, #15677, #3642, #14439, #20263, #1756, #24773, #31184, #13936, #5872, #33298, #34837, #30689, #17432, #26722, #8474, #19546, #17267, #32788, #35358, #35289, #15656, #28324, #3379, #6905, #5630, #9789, #36661, #20663, #36478, #13970, #29767, #30533, #2066, #27398, #10457, #4382, #24275, #15651, #25993, #23868, #22334, #30662, #36496, #24992, #12043, #34267, #24736, #10134, #21820, #25465, #29949, #23101, #34555, #36177, #14067, #9415, #31608, #7703, #31299, #12017, #17892, #13894, #29819, #36492, #23339, #16005, #5037, #8710, #21815, #12873, #7995, #12437, #29061, #14590, #10788, #25306 ) ) ;
#10000=CYLINDRICAL_SURFACE ( 'NONE', #14864, 2.000000000000001776 ) ;
#10001=ORIENTED_EDGE ( 'NONE', *, *, #12609, .F. ) ;
#10002=ADVANCED_FACE ( 'NONE', ( #34732 ), #34349, .F. ) ;
#10003=ORIENTED_EDGE ( 'NONE', *, *, #10930, .F. ) ;
#10004=AXIS2_PLACEMENT_3D ( 'NONE', #4246, #30277, #4611 ) ;
#10006=DIRECTION ( 'NONE',  ( 0.000000000000000000, 0.000000000000000000, 1.000000000000000000 ) ) ;
#10007=CIRCLE ( 'NONE', #13595, 1.999999999999998224 ) ;
#10008=LINE ( 'NONE', #15456, #12661 ) ;
#10009=DIRECTION ( 'NONE',  ( 0.000000000000000000, 0.000000000000000000, 1.000000000000000000 ) ) ;
#10010=AXIS2_PLACEMENT_3D ( 'NONE', #2816, #17048, #16705 ) ;
#10011=AXIS2_PLACEMENT_3D ( 'NONE', #6099, #31770, #25620 ) ;
#10012=ADVANCED_FACE ( 'NONE', ( #10152 ), #21194, .F. ) ;
#10013=EDGE_LOOP ( 'NONE', ( #30779, #7060 ) ) ;
#10014=DIRECTION ( 'NONE',  ( 1.000000000000000000, 0.000000000000000000, 0.000000000000000000 ) ) ;
#10015=ORIENTED_EDGE ( 'NONE', *, *, #14703, .T. ) ;
#10017=LINE ( 'NONE', #35369, #25618 ) ;
#10018=CARTESIAN_POINT ( 'NONE',  ( -85.00000337463092137, 25.98076211353317433, -9.999999999999998224 ) ) ;
#10019=CIRCLE ( 'NONE', #36422, 2.000000000000001776 ) ;
#10020=DIRECTION ( 'NONE',  ( 0.000000000000000000, 0.000000000000000000, 1.000000000000000000 ) ) ;
#10021=FACE_OUTER_BOUND ( 'NONE', #12677, .T. ) ;
#10024=EDGE_CURVE ( 'NONE', #12218, #22555, #25577, .T. ) ;
#10025=DIRECTION ( 'NONE',  ( 0.000000000000000000, 0.000000000000000000, -1.000000000000000000 ) ) ;
#10027=DIRECTION ( 'NONE',  ( 0.000000000000000000, 0.000000000000000000, 1.000000000000000000 ) ) ;
#10028=AXIS2_PLACEMENT_3D ( 'NONE', #13366, #5335, #31189 ) ;
#10030=FACE_OUTER_BOUND ( 'NONE', #30036, .T. ) ;
#10031=AXIS2_PLACEMENT_3D ( 'NONE', #3061, #601, #23473 ) ;
#10032=EDGE_LOOP ( 'NONE', ( #17468, #32434, #28410, #31277 ) ) ;
#10033=ADVANCED_FACE ( 'NONE', ( #7154 ), #35472, .T. ) ;
#10036=AXIS2_PLACEMENT_3D ( 'NONE', #30716, #25125, #4876 ) ;
#10038=CYLINDRICAL_SURFACE ( 'NONE', #30181, 2.000000000000001776 ) ;
#10039=CARTESIAN_POINT ( 'NONE',  ( -3.000003374631269981, -77.94228634059960825, 12.50000000000000000 ) ) ;
#10040=ORIENTED_EDGE ( 'NONE', *, *, #33222, .T. ) ;
#10042=EDGE_CURVE ( 'NONE', #20202, #29611, #9759, .T. ) ;
#10044=AXIS2_PLACEMENT_3D ( 'NONE', #1927, #21995, #24812 ) ;
#10047=VERTEX_POINT ( 'NONE', #15762 ) ;
#10048=EDGE_CURVE ( 'NONE', #21760, #8155, #26635, .T. ) ;
#10050=VERTEX_POINT ( 'NONE', #23843 ) ;
#10051=FACE_BOUND ( 'NONE', #23451, .T. ) ;
#10052=CIRCLE ( 'NONE', #14833, 3.000000000000002665 ) ;
#10053=ADVANCED_FACE ( 'NONE', ( #3950 ), #18764, .F. ) ;
#10054=LINE ( 'NONE', #18500, #36359 ) ;
#10055=CARTESIAN_POINT ( 'NONE',  ( -50.00000337463109190, 51.96152422706637708, 17.49999999999999645 ) ) ;
#10056=AXIS2_PLACEMENT_3D ( 'NONE', #18533, #29955, #18706 ) ;
#10057=EDGE_CURVE ( 'NONE', #2026, #12842, #32625, .T. ) ;
#10058=EDGE_LOOP ( 'NONE', ( #25206, #5998, #30213, #3648 ) ) ;
#10059=DIRECTION ( 'NONE',  ( 0.000000000000000000, 0.000000000000000000, -1.000000000000000000 ) ) ;
#10060=AXIS2_PLACEMENT_3D ( 'NONE', #36326, #5391, #27512 ) ;
#10061=VECTOR ( 'NONE', #20645, 1000.000000000000000 ) ;
#10063=AXIS2_PLACEMENT_3D ( 'NONE', #28093, #25457, #36549 ) ;
#10064=CARTESIAN_POINT ( 'NONE',  ( -18.00000337463123756, -86.60254037844400443, -5.000000000000000000 ) ) ;
#10066=VECTOR ( 'NONE', #10939, 1000.000000000000000 ) ;
#10067=FACE_OUTER_BOUND ( 'NONE', #15193, .T. ) ;
#10068=FACE_OUTER_BOUND ( 'NONE', #32880, .T. ) ;
#10069=VERTEX_POINT ( 'NONE', #18399 ) ;
#10070=FACE_OUTER_BOUND ( 'NONE', #6116, .T. ) ;
#10071=DIRECTION ( 'NONE',  ( -1.000000000000000000, 0.000000000000000000, 0.000000000000000000 ) ) ;
#10072=CARTESIAN_POINT ( 'NONE',  ( -60.00000337463108480, -51.96152422706641971, 12.50000000000000000 ) ) ;
#10073=VECTOR ( 'NONE', #2042, 1000.000000000000000 ) ;
#10075=ORIENTED_EDGE ( 'NONE', *, *, #13539, .T. ) ;
#10076=CARTESIAN_POINT ( 'NONE',  ( -42.00000337463114164, 69.28203230275516944, 17.49999999999999645 ) ) ;
#10077=AXIS2_PLACEMENT_3D ( 'NONE', #14007, #2969, #8221 ) ;
#10079=CARTESIAN_POINT ( 'NONE',  ( 66.99999662536839651, 60.62177826491078747, -9.999999999999998224 ) ) ;
#10083=CARTESIAN_POINT ( 'NONE',  ( 74.99999662536836809, 25.98076211353319565, -9.999999999999998224 ) ) ;
#10085=AXIS2_PLACEMENT_3D ( 'NONE', #22511, #33963, #31144 ) ;
#10086=DIRECTION ( 'NONE',  ( 0.000000000000000000, 0.000000000000000000, 1.000000000000000000 ) ) ;
#10087=FACE_OUTER_BOUND ( 'NONE', #11529, .T. ) ;
#10088=ORIENTED_EDGE ( 'NONE', *, *, #30556, .F. ) ;
#10089=AXIS2_PLACEMENT_3D ( 'NONE', #9086, #14531, #32334 ) ;
#10090=EDGE_CURVE ( 'NONE', #25333, #520, #1644, .T. ) ;
#10091=ORIENTED_EDGE ( 'NONE', *, *, #24087, .F. ) ;
#10094=DIRECTION ( 'NONE',  ( 1.000000000000000000, 0.000000000000000000, 0.000000000000000000 ) ) ;
#10095=ORIENTED_EDGE ( 'NONE', *, *, #22834, .T. ) ;
#10096=EDGE_CURVE ( 'NONE', #4290, #17808, #1148, .T. ) ;
#10097=CARTESIAN_POINT ( 'NONE',  ( 84.99999662536832545, 25.98076211353319565, -5.000000000000000000 ) ) ;
#10098=EDGE_CURVE ( 'NONE', #13035, #15480, #21396, .T. ) ;
#10100=DIRECTION ( 'NONE',  ( 1.000000000000000000, 0.000000000000000000, 0.000000000000000000 ) ) ;
#10101=CIRCLE ( 'NONE', #29327, 27.00000000000001776 ) ;
#10103=DIRECTION ( 'NONE',  ( -0.8660254037844453689, -0.4999999999999882871, 0.000000000000000000 ) ) ;
#10106=DIRECTION ( 'NONE',  ( 0.000000000000000000, 0.000000000000000000, 1.000000000000000000 ) ) ;
#10108=AXIS2_PLACEMENT_3D ( 'NONE', #23760, #9513, #3317 ) ;
#10110=CARTESIAN_POINT ( 'NONE',  ( -10.00000337463128197, 86.60254037844397601, 12.50000000000000000 ) ) ;
#10111=ADVANCED_FACE ( 'NONE', ( #33011 ), #6758, .T. ) ;
#10112=CIRCLE ( 'NONE', #6519, 2.000000000000001776 ) ;
#10113=CYLINDRICAL_SURFACE ( 'NONE', #23304, 2.000000000000001776 ) ;
#10114=LINE ( 'NONE', #21715, #21508 ) ;
#10115=ORIENTED_EDGE ( 'NONE', *, *, #26643, .T. ) ;
#10116=CARTESIAN_POINT ( 'NONE',  ( -20.00000337463123756, -69.28203230275522628, 17.49999999999999645 ) ) ;
#10117=FACE_OUTER_BOUND ( 'NONE', #5709, .T. ) ;
#10119=ORIENTED_EDGE ( 'NONE', *, *, #15165, .F. ) ;
#10121=DIRECTION ( 'NONE',  ( 0.000000000000000000, 0.000000000000000000, -1.000000000000000000 ) ) ;
#10123=DIRECTION ( 'NONE',  ( 0.000000000000000000, 0.000000000000000000, 1.000000000000000000 ) ) ;
#10124=ORIENTED_EDGE ( 'NONE', *, *, #7829, .F. ) ;
#10125=DIRECTION ( 'NONE',  ( 0.000000000000000000, 0.000000000000000000, 1.000000000000000000 ) ) ;
#10127=CIRCLE ( 'NONE', #23286, 2.000000000000001776 ) ;
#10128=VERTEX_POINT ( 'NONE', #24027 ) ;
#10130=CARTESIAN_POINT ( 'NONE',  ( 62.33939050065184517, -13.89091430021398565, 12.49999999999999822 ) ) ;
#10131=EDGE_CURVE ( 'NONE', #2314, #9400, #7507, .T. ) ;
#10133=CARTESIAN_POINT ( 'NONE',  ( 49.99999662536846756, 51.96152422706637708, -9.999999999999998224 ) ) ;
#10134=ADVANCED_FACE ( 'NONE', ( #21392 ), #29444, .T. ) ;
#10135=CARTESIAN_POINT ( 'NONE',  ( 69.99999662536839651, 17.32050807568879236, -9.999999999999998224 ) ) ;
#10136=DIRECTION ( 'NONE',  ( -0.000000000000000000, -0.000000000000000000, 1.000000000000000000 ) ) ;
#10137=ORIENTED_EDGE ( 'NONE', *, *, #10816, .T. ) ;
#10138=VERTEX_POINT ( 'NONE', #21018 ) ;
#10140=CIRCLE ( 'NONE', #22103, 2.000000000000001776 ) ;
#10141=CARTESIAN_POINT ( 'NONE',  ( 79.99999662536832545, -34.64101615137759183, -9.999999999999998224 ) ) ;
#10142=DIRECTION ( 'NONE',  ( 0.000000000000000000, 0.000000000000000000, 1.000000000000000000 ) ) ;
#10143=CARTESIAN_POINT ( 'NONE',  ( 22.99999662536859901, -77.94228634059960825, -9.999999999999998224 ) ) ;
#10144=ADVANCED_FACE ( 'NONE', ( #22142 ), #11244, .F. ) ;
#10145=ORIENTED_EDGE ( 'NONE', *, *, #1047, .F. ) ;
#10146=AXIS2_PLACEMENT_3D ( 'NONE', #32586, #15346, #1287 ) ;
#10148=DIRECTION ( 'NONE',  ( -1.000000000000000000, 0.000000000000000000, 0.000000000000000000 ) ) ;
#10150=ORIENTED_EDGE ( 'NONE', *, *, #7960, .T. ) ;
#10151=CIRCLE ( 'NONE', #6553, 2.000000000000000000 ) ;
#10152=FACE_OUTER_BOUND ( 'NONE', #23566, .T. ) ;
#10153=ORIENTED_EDGE ( 'NONE', *, *, #35245, .T. ) ;
#10154=AXIS2_PLACEMENT_3D ( 'NONE', #19826, #22639, #22438 ) ;
#10156=CARTESIAN_POINT ( 'NONE',  ( 69.99999662536839651, -3.469446951953614189E-15, -9.999999999999998224 ) ) ;
#10158=DIRECTION ( 'NONE',  ( 1.000000000000000000, 0.000000000000000000, 0.000000000000000000 ) ) ;
#10160=EDGE_CURVE ( 'NONE', #17753, #4797, #10502, .T. ) ;
#10163=VERTEX_POINT ( 'NONE', #25150 ) ;
#10164=AXIS2_PLACEMENT_3D ( 'NONE', #24262, #24471, #33259 ) ;
#10165=VERTEX_POINT ( 'NONE', #13868 ) ;
#10166=ORIENTED_EDGE ( 'NONE', *, *, #7266, .T. ) ;
#10167=CYLINDRICAL_SURFACE ( 'NONE', #8213, 2.000000000000000000 ) ;
#10169=FACE_BOUND ( 'NONE', #967, .T. ) ;
#10170=CIRCLE ( 'NONE', #25145, 2.000000000000000000 ) ;
#10171=FACE_OUTER_BOUND ( 'NONE', #15164, .T. ) ;
#10174=ORIENTED_EDGE ( 'NONE', *, *, #2765, .T. ) ;
#10176=DIRECTION ( 'NONE',  ( 0.000000000000000000, 0.000000000000000000, 1.000000000000000000 ) ) ;
#10178=VERTEX_POINT ( 'NONE', #2259 ) ;
#10179=CARTESIAN_POINT ( 'NONE',  ( -33.00000337463116296, -60.62177826491080168, 17.49999999999999645 ) ) ;
#10180=DIRECTION ( 'NONE',  ( -0.000000000000000000, -0.000000000000000000, 1.000000000000000000 ) ) ;
#10182=EDGE_LOOP ( 'NONE', ( #13300, #14436, #18773, #14727, #31929, #32613 ) ) ;
#10183=VERTEX_POINT ( 'NONE', #28125 ) ;
#10184=DIRECTION ( 'NONE',  ( 0.000000000000000000, 0.000000000000000000, 1.000000000000000000 ) ) ;
#10185=CIRCLE ( 'NONE', #19185, 2.000000000000001776 ) ;
#10186=CARTESIAN_POINT ( 'NONE',  ( 35.83991598322140248, 56.52018970185221036, 12.49999999999999645 ) ) ;
#10188=ORIENTED_EDGE ( 'NONE', *, *, #21206, .T. ) ;
#10190=ORIENTED_EDGE ( 'NONE', *, *, #15142, .T. ) ;
#10191=CARTESIAN_POINT ( 'NONE',  ( -37.00000337463117717, -77.94228634059963667, -9.999999999999998224 ) ) ;
#10193=EDGE_LOOP ( 'NONE', ( #11352, #30043, #36019, #34318, #23338 ) ) ;
#10194=EDGE_LOOP ( 'NONE', ( #28525, #32967, #26259, #7898 ) ) ;
#10195=CIRCLE ( 'NONE', #9, 27.00000000000001421 ) ;
#10196=CARTESIAN_POINT ( 'NONE',  ( 56.67878100130369035, -27.78182860042797131, -4.999999999999997335 ) ) ;
#10197=ORIENTED_EDGE ( 'NONE', *, *, #20216, .T. ) ;
#10198=ORIENTED_EDGE ( 'NONE', *, *, #28772, .F. ) ;
#10200=DIRECTION ( 'NONE',  ( 1.000000000000000000, 0.000000000000000000, 0.000000000000000000 ) ) ;
#10201=ADVANCED_FACE ( 'NONE', ( #36935 ), #19693, .F. ) ;
#10202=EDGE_LOOP ( 'NONE', ( #11078, #12611 ) ) ;
#10203=VECTOR ( 'NONE', #3624, 1000.000000000000000 ) ;
#10205=CARTESIAN_POINT ( 'NONE',  ( 19.99999662536858835, 69.28203230275516944, 17.49999999999999645 ) ) ;
#10207=CIRCLE ( 'NONE', #25180, 2.000000000000001776 ) ;
#10208=DIRECTION ( 'NONE',  ( -1.000000000000000000, 0.000000000000000000, 0.000000000000000000 ) ) ;
#10209=CARTESIAN_POINT ( 'NONE',  ( 11.99999662536862566, 86.60254037844397601, -5.000000000000000000 ) ) ;
#10210=ORIENTED_EDGE ( 'NONE', *, *, #131, .T. ) ;
#10211=DIRECTION ( 'NONE',  ( 0.000000000000000000, 0.000000000000000000, 1.000000000000000000 ) ) ;
#10212=ORIENTED_EDGE ( 'NONE', *, *, #35368, .T. ) ;
#10213=DIRECTION ( 'NONE',  ( 1.000000000000000000, 0.000000000000000000, 0.000000000000000000 ) ) ;
#10214=CARTESIAN_POINT ( 'NONE',  ( 34.99999662536855283, -77.94228634059960825, -9.999999999999998224 ) ) ;
#10215=AXIS2_PLACEMENT_3D ( 'NONE', #35620, #26803, #9560 ) ;
#10216=FACE_BOUND ( 'NONE', #10740, .T. ) ;
#10217=DIRECTION ( 'NONE',  ( 0.000000000000000000, 0.000000000000000000, 1.000000000000000000 ) ) ;
#10220=DIRECTION ( 'NONE',  ( 0.000000000000000000, 0.000000000000000000, -1.000000000000000000 ) ) ;
#10221=ORIENTED_EDGE ( 'NONE', *, *, #6007, .T. ) ;
#10223=FACE_OUTER_BOUND ( 'NONE', #4342, .T. ) ;
#10224=CARTESIAN_POINT ( 'NONE',  ( -7.000003374631269537, -77.94228634059960825, -9.999999999999998224 ) ) ;
#10225=ADVANCED_FACE ( 'NONE', ( #2449 ), #27742, .T. ) ;
#10227=ORIENTED_EDGE ( 'NONE', *, *, #18809, .F. ) ;
#10229=ORIENTED_EDGE ( 'NONE', *, *, #26970, .T. ) ;
#10234=EDGE_CURVE ( 'NONE', #9552, #32504, #26630, .T. ) ;
#10235=DIRECTION ( 'NONE',  ( 0.000000000000000000, 0.000000000000000000, 1.000000000000000000 ) ) ;
#10236=ORIENTED_EDGE ( 'NONE', *, *, #21954, .T. ) ;
#10238=ORIENTED_EDGE ( 'NONE', *, *, #16117, .F. ) ;
#10239=CARTESIAN_POINT ( 'NONE',  ( -35.00000337463116296, 77.94228634059957983, -5.000000000000000000 ) ) ;
#10240=DIRECTION ( 'NONE',  ( 0.000000000000000000, 0.000000000000000000, 1.000000000000000000 ) ) ;
#10241=CARTESIAN_POINT ( 'NONE',  ( 36.97203788309026606, -58.48108235278833433, 12.49999999999999645 ) ) ;
#10242=ADVANCED_FACE ( 'NONE', ( #1885 ), #24956, .F. ) ;
#10243=VERTEX_POINT ( 'NONE', #22491 ) ;
#10244=DIRECTION ( 'NONE',  ( -0.000000000000000000, -0.000000000000000000, 1.000000000000000000 ) ) ;
#10247=FACE_BOUND ( 'NONE', #36315, .T. ) ;
#10248=CARTESIAN_POINT ( 'NONE',  ( 47.99999662536846756, 69.28203230275516944, -9.999999999999998224 ) ) ;
#10250=LINE ( 'NONE', #21680, #17795 ) ;
#10251=LINE ( 'NONE', #29939, #24439 ) ;
#10252=DIRECTION ( 'NONE',  ( -1.000000000000000000, 0.000000000000000000, -0.000000000000000000 ) ) ;
#10255=VERTEX_POINT ( 'NONE', #21945 ) ;
#10256=DIRECTION ( 'NONE',  ( -0.000000000000000000, -0.000000000000000000, 1.000000000000000000 ) ) ;
#10257=LINE ( 'NONE', #21688, #21181 ) ;
#10258=LINE ( 'NONE', #36321, #22487 ) ;
#10259=ORIENTED_EDGE ( 'NONE', *, *, #15734, .F. ) ;
#10260=DIRECTION ( 'NONE',  ( -0.000000000000000000, -0.000000000000000000, -1.000000000000000000 ) ) ;
#10262=ADVANCED_FACE ( 'NONE', ( #30739 ), #30577, .F. ) ;
#10263=CARTESIAN_POINT ( 'NONE',  ( 17.99999662536858835, 69.28203230275516944, -9.999999999999998224 ) ) ;
#10264=DIRECTION ( 'NONE',  ( 0.000000000000000000, 0.000000000000000000, 1.000000000000000000 ) ) ;
#10265=VERTEX_POINT ( 'NONE', #13695 ) ;
#10266=ORIENTED_EDGE ( 'NONE', *, *, #9001, .F. ) ;
#10267=CARTESIAN_POINT ( 'NONE',  ( 11.99999662536865763, -69.28203230275519786, -9.999999999999998224 ) ) ;
#10268=EDGE_CURVE ( 'NONE', #12416, #7360, #17628, .T. ) ;
#10269=DIRECTION ( 'NONE',  ( -1.000000000000000000, 0.000000000000000000, -0.000000000000000000 ) ) ;
#10270=VERTEX_POINT ( 'NONE', #10874 ) ;
#10271=FACE_OUTER_BOUND ( 'NONE', #9894, .T. ) ;
#10272=ORIENTED_EDGE ( 'NONE', *, *, #233, .F. ) ;
#10273=AXIS2_PLACEMENT_3D ( 'NONE', #19316, #10309, #1877 ) ;
#10275=CARTESIAN_POINT ( 'NONE',  ( -55.00000337463107059, 43.30127018922197379, 17.49999999999999645 ) ) ;
#10276=ORIENTED_EDGE ( 'NONE', *, *, #23273, .F. ) ;
#10277=DIRECTION ( 'NONE',  ( 0.000000000000000000, 0.000000000000000000, 1.000000000000000000 ) ) ;
#10278=ORIENTED_EDGE ( 'NONE', *, *, #31637, .F. ) ;
#10280=DIRECTION ( 'NONE',  ( 0.000000000000000000, 0.000000000000000000, -1.000000000000000000 ) ) ;
#10282=LINE ( 'NONE', #33146, #29913 ) ;
#10283=CARTESIAN_POINT ( 'NONE',  ( 76.99999662536836809, 8.660254037844394404, -9.999999999999998224 ) ) ;
#10285=DIRECTION ( 'NONE',  ( 1.000000000000000000, 0.000000000000000000, 0.000000000000000000 ) ) ;
#10286=CARTESIAN_POINT ( 'NONE',  ( 59.99999662536842493, -51.96152422706639840, -9.999999999999998224 ) ) ;
#10287=FACE_OUTER_BOUND ( 'NONE', #11127, .T. ) ;
#10288=ORIENTED_EDGE ( 'NONE', *, *, #22430, .T. ) ;
#10289=EDGE_CURVE ( 'NONE', #33284, #32298, #29587, .T. ) ;
#10290=EDGE_LOOP ( 'NONE', ( #15965, #17816, #35140, #17300 ) ) ;
#10292=VECTOR ( 'NONE', #25369, 1000.000000000000000 ) ;
#10293=EDGE_CURVE ( 'NONE', #15817, #27467, #17050, .T. ) ;
#10294=DIRECTION ( 'NONE',  ( 0.000000000000000000, 0.000000000000000000, -1.000000000000000000 ) ) ;
#10295=ORIENTED_EDGE ( 'NONE', *, *, #2915, .T. ) ;
#10297=CARTESIAN_POINT ( 'NONE',  ( -60.93295298010992411, -19.13981058454771755, 12.49999999999999822 ) ) ;
#10298=CARTESIAN_POINT ( 'NONE',  ( 27.99999662536855993, 69.28203230275518365, -9.999999999999998224 ) ) ;
#10299=DIRECTION ( 'NONE',  ( 1.000000000000000000, 0.000000000000000000, 0.000000000000000000 ) ) ;
#10300=DIRECTION ( 'NONE',  ( 1.000000000000000000, 0.000000000000000000, 0.000000000000000000 ) ) ;
#10303=DIRECTION ( 'NONE',  ( -1.000000000000000000, 0.000000000000000000, 0.000000000000000000 ) ) ;
#10304=VERTEX_POINT ( 'NONE', #8987 ) ;
#10305=ORIENTED_EDGE ( 'NONE', *, *, #30442, .T. ) ;
#10306=DIRECTION ( 'NONE',  ( 0.000000000000000000, -0.000000000000000000, -1.000000000000000000 ) ) ;
#10307=EDGE_CURVE ( 'NONE', #15870, #26836, #14047, .T. ) ;
#10309=DIRECTION ( 'NONE',  ( 0.000000000000000000, 0.000000000000000000, 1.000000000000000000 ) ) ;
#10310=CYLINDRICAL_SURFACE ( 'NONE', #13705, 2.000000000000001776 ) ;
#10311=ORIENTED_EDGE ( 'NONE', *, *, #9612, .T. ) ;
#10312=DIRECTION ( 'NONE',  ( -0.000000000000000000, -0.000000000000000000, -1.000000000000000000 ) ) ;
#10313=CARTESIAN_POINT ( 'NONE',  ( 74.99999662536836809, 25.98076211353319565, 12.50000000000000000 ) ) ;
#10314=DIRECTION ( 'NONE',  ( 0.000000000000000000, 0.000000000000000000, 1.000000000000000000 ) ) ;
#10318=ORIENTED_EDGE ( 'NONE', *, *, #8383, .T. ) ;
#10322=ADVANCED_FACE ( 'NONE', ( #14985 ), #31665, .F. ) ;
#10323=CARTESIAN_POINT ( 'NONE',  ( -65.00000337463106348, -60.62177826491083010, 12.50000000000000000 ) ) ;
#10324=ORIENTED_EDGE ( 'NONE', *, *, #34444, .F. ) ;
#10325=ADVANCED_FACE ( 'NONE', ( #12129 ), #11587, .F. ) ;
#10326=ORIENTED_EDGE ( 'NONE', *, *, #32068, .F. ) ;
#10327=FACE_OUTER_BOUND ( 'NONE', #36354, .T. ) ;
#10329=CIRCLE ( 'NONE', #18114, 2.000000000000001776 ) ;
#10330=ORIENTED_EDGE ( 'NONE', *, *, #13858, .T. ) ;
#10331=DIRECTION ( 'NONE',  ( 0.000000000000000000, 0.000000000000000000, 1.000000000000000000 ) ) ;
#10332=CYLINDRICAL_SURFACE ( 'NONE', #30532, 2.000000000000001776 ) ;
#10334=DIRECTION ( 'NONE',  ( -1.000000000000000000, 0.000000000000000000, 0.000000000000000000 ) ) ;
#10335=DIRECTION ( 'NONE',  ( -0.5000000000000098810, -0.8660254037844328234, 0.000000000000000000 ) ) ;
#10336=DIRECTION ( 'NONE',  ( 0.000000000000000000, 0.000000000000000000, 1.000000000000000000 ) ) ;
#10337=EDGE_CURVE ( 'NONE', #5470, #20921, #23637, .T. ) ;
#10338=VERTEX_POINT ( 'NONE', #20041 ) ;
#10340=DIRECTION ( 'NONE',  ( 0.000000000000000000, 0.000000000000000000, 1.000000000000000000 ) ) ;
#10341=AXIS2_PLACEMENT_3D ( 'NONE', #36594, #19522, #11265 ) ;
#10342=DIRECTION ( 'NONE',  ( 1.000000000000000000, 0.000000000000000000, 0.000000000000000000 ) ) ;
#10343=ORIENTED_EDGE ( 'NONE', *, *, #20735, .T. ) ;
#10345=DIRECTION ( 'NONE',  ( 0.000000000000000000, 0.000000000000000000, 1.000000000000000000 ) ) ;
#10346=FACE_OUTER_BOUND ( 'NONE', #9809, .T. ) ;
#10347=EDGE_CURVE ( 'NONE', #10265, #15896, #26234, .T. ) ;
#10348=ORIENTED_EDGE ( 'NONE', *, *, #16519, .T. ) ;
#10349=EDGE_CURVE ( 'NONE', #10338, #27157, #19868, .T. ) ;
#10350=VERTEX_POINT ( 'NONE', #25695 ) ;
#10352=EDGE_CURVE ( 'NONE', #2354, #10426, #3003, .T. ) ;
#10353=CARTESIAN_POINT ( 'NONE',  ( -55.00000337463109901, -60.62177826491083010, -9.999999999999998224 ) ) ;
#10354=DIRECTION ( 'NONE',  ( -0.000000000000000000, -0.000000000000000000, 1.000000000000000000 ) ) ;
#10356=ORIENTED_EDGE ( 'NONE', *, *, #29143, .T. ) ;
#10357=ORIENTED_EDGE ( 'NONE', *, *, #5444, .F. ) ;
#10359=DIRECTION ( 'NONE',  ( 0.000000000000000000, 0.000000000000000000, 1.000000000000000000 ) ) ;
#10360=CIRCLE ( 'NONE', #19331, 2.000000000000001776 ) ;
#10361=ORIENTED_EDGE ( 'NONE', *, *, #31081, .F. ) ;
#10362=CARTESIAN_POINT ( 'NONE',  ( -85.00000337463092137, -25.98076211353322051, 17.49999999999999645 ) ) ;
#10364=ORIENTED_EDGE ( 'NONE', *, *, #4087, .T. ) ;
#10365=DIRECTION ( 'NONE',  ( 0.000000000000000000, 0.000000000000000000, -1.000000000000000000 ) ) ;
#10366=VECTOR ( 'NONE', #21263, 1000.000000000000000 ) ;
#10367=CARTESIAN_POINT ( 'NONE',  ( -75.00000337463097821, 25.98076211353318854, -9.999999999999998224 ) ) ;
#10368=ORIENTED_EDGE ( 'NONE', *, *, #6912, .T. ) ;
#10369=VERTEX_POINT ( 'NONE', #341 ) ;
#10370=DIRECTION ( 'NONE',  ( 0.000000000000000000, 0.000000000000000000, 1.000000000000000000 ) ) ;
#10371=DIRECTION ( 'NONE',  ( 0.000000000000000000, 0.000000000000000000, -1.000000000000000000 ) ) ;
#10372=DIRECTION ( 'NONE',  ( 1.000000000000000000, 0.000000000000000000, 0.000000000000000000 ) ) ;
#10373=DIRECTION ( 'NONE',  ( 1.000000000000000000, 0.000000000000000000, 0.000000000000000000 ) ) ;
#10374=ORIENTED_EDGE ( 'NONE', *, *, #1242, .F. ) ;
#10375=DIRECTION ( 'NONE',  ( 1.000000000000000000, 0.000000000000000000, 0.000000000000000000 ) ) ;
#10376=ORIENTED_EDGE ( 'NONE', *, *, #9680, .F. ) ;
#10377=DIRECTION ( 'NONE',  ( -0.4999999999999977796, 0.8660254037844398178, 0.000000000000000000 ) ) ;
#10379=DIRECTION ( 'NONE',  ( 0.000000000000000000, 0.000000000000000000, -1.000000000000000000 ) ) ;
#10382=AXIS2_PLACEMENT_3D ( 'NONE', #14977, #11416, #5800 ) ;
#10383=DIRECTION ( 'NONE',  ( 0.000000000000000000, 0.000000000000000000, -1.000000000000000000 ) ) ;
#10385=ORIENTED_EDGE ( 'NONE', *, *, #18561, .F. ) ;
#10386=CARTESIAN_POINT ( 'NONE',  ( -42.00000337463114164, 69.28203230275516944, 12.50000000000000000 ) ) ;
#10387=DIRECTION ( 'NONE',  ( 1.000000000000000000, 0.000000000000000000, 0.000000000000000000 ) ) ;
#10388=DIRECTION ( 'NONE',  ( -1.000000000000000000, 0.000000000000000000, 0.000000000000000000 ) ) ;
#10391=EDGE_LOOP ( 'NONE', ( #17413, #13662, #3326, #16586, #12076, #1322 ) ) ;
#10392=EDGE_LOOP ( 'NONE', ( #30815, #15757, #22689, #15811, #9629 ) ) ;
#10393=AXIS2_PLACEMENT_3D ( 'NONE', #22566, #34024, #8334 ) ;
#10394=EDGE_CURVE ( 'NONE', #16962, #15109, #25864, .T. ) ;
#10395=DIRECTION ( 'NONE',  ( 0.000000000000000000, 0.000000000000000000, 1.000000000000000000 ) ) ;
#10396=DIRECTION ( 'NONE',  ( 1.000000000000000000, 0.000000000000000000, 0.000000000000000000 ) ) ;
#10398=CIRCLE ( 'NONE', #13980, 2.000000000000000000 ) ;
#10400=DIRECTION ( 'NONE',  ( 1.000000000000000000, 0.000000000000000000, 0.000000000000000000 ) ) ;
#10401=DIRECTION ( 'NONE',  ( 1.000000000000000000, 0.000000000000000000, 0.000000000000000000 ) ) ;
#10403=DIRECTION ( 'NONE',  ( 0.000000000000000000, 0.000000000000000000, -1.000000000000000000 ) ) ;
#10404=ORIENTED_EDGE ( 'NONE', *, *, #28790, .T. ) ;
#10405=FACE_BOUND ( 'NONE', #31060, .T. ) ;
#10406=AXIS2_PLACEMENT_3D ( 'NONE', #16434, #30858, #22820 ) ;
#10409=DIRECTION ( 'NONE',  ( 0.000000000000000000, 0.000000000000000000, 1.000000000000000000 ) ) ;
#10410=ORIENTED_EDGE ( 'NONE', *, *, #36470, .T. ) ;
#10411=FACE_OUTER_BOUND ( 'NONE', #29858, .T. ) ;
#10413=ADVANCED_FACE ( 'NONE', ( #34488 ), #5999, .F. ) ;
#10414=VECTOR ( 'NONE', #25411, 1000.000000000000000 ) ;
#10416=CARTESIAN_POINT ( 'NONE',  ( 44.99999662536849598, -77.94228634059960825, 12.50000000000000000 ) ) ;
#10417=VERTEX_POINT ( 'NONE', #3166 ) ;
#10420=DIRECTION ( 'NONE',  ( 0.000000000000000000, 0.000000000000000000, 1.000000000000000000 ) ) ;
#10421=EDGE_LOOP ( 'NONE', ( #35731, #2288 ) ) ;
#10422=DIRECTION ( 'NONE',  ( 1.000000000000000000, 0.000000000000000000, 0.000000000000000000 ) ) ;
#10423=CYLINDRICAL_SURFACE ( 'NONE', #31618, 2.000000000000001776 ) ;
#10424=DIRECTION ( 'NONE',  ( -1.000000000000000000, 0.000000000000000000, 0.000000000000000000 ) ) ;
#10425=EDGE_CURVE ( 'NONE', #23671, #4724, #7475, .T. ) ;
#10426=VERTEX_POINT ( 'NONE', #18721 ) ;
#10427=ORIENTED_EDGE ( 'NONE', *, *, #36172, .T. ) ;
#10430=DIRECTION ( 'NONE',  ( 0.000000000000000000, 0.000000000000000000, -1.000000000000000000 ) ) ;
#10432=CARTESIAN_POINT ( 'NONE',  ( 62.97617850287784336, 4.279621169095339184, 12.49999999999999822 ) ) ;
#10433=ORIENTED_EDGE ( 'NONE', *, *, #33507, .T. ) ;
#10434=EDGE_LOOP ( 'NONE', ( #11400, #28658 ) ) ;
#10435=EDGE_CURVE ( 'NONE', #29294, #545, #4480, .T. ) ;
#10436=CARTESIAN_POINT ( 'NONE',  ( -60.00000337463104216, 34.64101615137757051, 12.50000000000000000 ) ) ;
#10437=CARTESIAN_POINT ( 'NONE',  ( -77.00000337463099243, -25.98076211353322051, -5.000000000000000000 ) ) ;
#10438=CARTESIAN_POINT ( 'NONE',  ( -10.00000337463127842, -69.28203230275519786, -9.999999999999998224 ) ) ;
#10439=CARTESIAN_POINT ( 'NONE',  ( -38.00000337463113453, 69.28203230275516944, -9.999999999999998224 ) ) ;
#10442=VERTEX_POINT ( 'NONE', #15904 ) ;
#10443=DIRECTION ( 'NONE',  ( 0.000000000000000000, 0.000000000000000000, 1.000000000000000000 ) ) ;
#10444=VECTOR ( 'NONE', #36179, 1000.000000000000000 ) ;
#10445=CYLINDRICAL_SURFACE ( 'NONE', #17680, 2.000000000000001776 ) ;
#10447=DIRECTION ( 'NONE',  ( 0.4999999999999919509, -0.8660254037844432595, 0.000000000000000000 ) ) ;
#10448=EDGE_LOOP ( 'NONE', ( #31940, #20240, #30044, #17670 ) ) ;
#10449=DIRECTION ( 'NONE',  ( 0.000000000000000000, 0.000000000000000000, 1.000000000000000000 ) ) ;
#10451=VECTOR ( 'NONE', #21966, 1000.000000000000000 ) ;
#10456=ORIENTED_EDGE ( 'NONE', *, *, #33227, .F. ) ;
#10457=ADVANCED_FACE ( 'NONE', ( #23985 ), #15720, .T. ) ;
#10459=AXIS2_PLACEMENT_3D ( 'NONE', #7494, #18752, #27372 ) ;
#10461=CYLINDRICAL_SURFACE ( 'NONE', #36515, 2.000000000000001776 ) ;
#10462=DIRECTION ( 'NONE',  ( -1.000000000000000000, 0.000000000000000000, 0.000000000000000000 ) ) ;
#10463=EDGE_LOOP ( 'NONE', ( #5030, #19390, #4833, #1705 ) ) ;
#10464=CARTESIAN_POINT ( 'NONE',  ( -47.00000337463111322, -77.94228634059960825, -9.999999999999998224 ) ) ;
#10465=ADVANCED_FACE ( 'NONE', ( #6548 ), #4289, .F. ) ;
#10466=LINE ( 'NONE', #36897, #5861 ) ;
#10468=VERTEX_POINT ( 'NONE', #15154 ) ;
#10469=AXIS2_PLACEMENT_3D ( 'NONE', #22275, #11391, #16840 ) ;
#10470=VERTEX_POINT ( 'NONE', #15544 ) ;
#10471=EDGE_CURVE ( 'NONE', #6640, #12600, #35036, .T. ) ;
#10472=VERTEX_POINT ( 'NONE', #12527 ) ;
#10473=AXIS2_PLACEMENT_3D ( 'NONE', #15866, #27291, #18866 ) ;
#10474=CARTESIAN_POINT ( 'NONE',  ( 47.04203867989577503, -43.19957991610382919, 12.49999999999999822 ) ) ;
#10477=DIRECTION ( 'NONE',  ( 0.000000000000000000, 0.000000000000000000, 1.000000000000000000 ) ) ;
#10478=DIRECTION ( 'NONE',  ( 0.8660254037844344888, -0.5000000000000071054, 0.000000000000000000 ) ) ;
#10479=VECTOR ( 'NONE', #15117, 1000.000000000000000 ) ;
#10480=LINE ( 'NONE', #10680, #20021 ) ;
#10481=LINE ( 'NONE', #29806, #2925 ) ;
#10483=AXIS2_PLACEMENT_3D ( 'NONE', #27250, #33073, #15652 ) ;
#10484=CARTESIAN_POINT ( 'NONE',  ( -10.00000337463125000, -86.60254037844400443, -9.999999999999998224 ) ) ;
#10487=CIRCLE ( 'NONE', #302, 2.000000000000001776 ) ;
#10488=ORIENTED_EDGE ( 'NONE', *, *, #3481, .F. ) ;
#10489=EDGE_CURVE ( 'NONE', #36483, #357, #13429, .T. ) ;
#10490=DIRECTION ( 'NONE',  ( 0.000000000000000000, 0.000000000000000000, -1.000000000000000000 ) ) ;
#10491=CARTESIAN_POINT ( 'NONE',  ( 44.99999662536849598, -77.94228634059960825, -9.999999999999998224 ) ) ;
#10492=FACE_OUTER_BOUND ( 'NONE', #28592, .T. ) ;
#10493=DIRECTION ( 'NONE',  ( 0.000000000000000000, 0.000000000000000000, 1.000000000000000000 ) ) ;
#10495=AXIS2_PLACEMENT_3D ( 'NONE', #9508, #23393, #17746 ) ;
#10496=ADVANCED_FACE ( 'NONE', ( #15341 ), #21152, .F. ) ;
#10497=VECTOR ( 'NONE', #24637, 1000.000000000000000 ) ;
#10498=DIRECTION ( 'NONE',  ( -1.000000000000000000, 6.167905692361977800E-15, 0.000000000000000000 ) ) ;
#10499=DIRECTION ( 'NONE',  ( 0.000000000000000000, 0.000000000000000000, 1.000000000000000000 ) ) ;
#10500=ORIENTED_EDGE ( 'NONE', *, *, #884, .F. ) ;
#10501=EDGE_CURVE ( 'NONE', #16545, #716, #20779, .T. ) ;
#10502=LINE ( 'NONE', #30926, #19607 ) ;
#10503=ORIENTED_EDGE ( 'NONE', *, *, #20570, .F. ) ;
#10504=( LENGTH_UNIT ( ) NAMED_UNIT ( * ) SI_UNIT ( .MILLI., .METRE. ) );
#10505=CYLINDRICAL_SURFACE ( 'NONE', #34710, 2.000000000000001776 ) ;
#10506=DIRECTION ( 'NONE',  ( -0.000000000000000000, -0.000000000000000000, -1.000000000000000000 ) ) ;
#10507=CIRCLE ( 'NONE', #29031, 2.000000000000001776 ) ;
#10509=EDGE_LOOP ( 'NONE', ( #29195, #35874, #10410, #5192 ) ) ;
#10510=CIRCLE ( 'NONE', #917, 2.000000000000001776 ) ;
#10512=CIRCLE ( 'NONE', #18299, 2.000000000000001776 ) ;
#10514=CIRCLE ( 'NONE', #12917, 2.000000000000000000 ) ;
#10515=EDGE_CURVE ( 'NONE', #27674, #21403, #19442, .T. ) ;
#10516=ORIENTED_EDGE ( 'NONE', *, *, #7266, .F. ) ;
#10517=DIRECTION ( 'NONE',  ( 0.000000000000000000, 0.000000000000000000, 1.000000000000000000 ) ) ;
#10518=FACE_OUTER_BOUND ( 'NONE', #13380, .T. ) ;
#10519=DIRECTION ( 'NONE',  ( 0.000000000000000000, 0.000000000000000000, -1.000000000000000000 ) ) ;
#10521=CARTESIAN_POINT ( 'NONE',  ( -47.63139720814438505, -27.49999999999955591, -10.00000000000000000 ) ) ;
#10523=FACE_OUTER_BOUND ( 'NONE', #11982, .T. ) ;
#10524=AXIS2_PLACEMENT_3D ( 'NONE', #7080, #27120, #1436 ) ;
#10525=CYLINDRICAL_SURFACE ( 'NONE', #11973, 2.000000000000000000 ) ;
#10526=( NAMED_UNIT ( * ) PLANE_ANGLE_UNIT ( ) SI_UNIT ( $, .RADIAN. ) );
#10527=ORIENTED_EDGE ( 'NONE', *, *, #6352, .F. ) ;
#10531=ORIENTED_EDGE ( 'NONE', *, *, #18213, .F. ) ;
#10533=AXIS2_PLACEMENT_3D ( 'NONE', #2331, #20110, #31352 ) ;
#10534=CARTESIAN_POINT ( 'NONE',  ( 86.99999662536831124, -25.98076211353319565, -9.999999999999998224 ) ) ;
#10535=DIRECTION ( 'NONE',  ( 1.000000000000000000, 0.000000000000000000, 0.000000000000000000 ) ) ;
#10536=EDGE_CURVE ( 'NONE', #28869, #16509, #30800, .T. ) ;
#10537=VECTOR ( 'NONE', #14271, 1000.000000000000000 ) ;
#10539=ORIENTED_EDGE ( 'NONE', *, *, #910, .F. ) ;
#10540=ORIENTED_EDGE ( 'NONE', *, *, #3387, .F. ) ;
#10541=ORIENTED_EDGE ( 'NONE', *, *, #23134, .T. ) ;
#10543=VECTOR ( 'NONE', #21838, 1000.000000000000000 ) ;
#10546=DIRECTION ( 'NONE',  ( 1.000000000000000000, 0.000000000000000000, 0.000000000000000000 ) ) ;
#10547=CIRCLE ( 'NONE', #23720, 2.000000000000001776 ) ;
#10548=VERTEX_POINT ( 'NONE', #20977 ) ;
#10549=EDGE_CURVE ( 'NONE', #36402, #8583, #24223, .T. ) ;
#10550=FACE_BOUND ( 'NONE', #5691, .T. ) ;
#10551=ORIENTED_EDGE ( 'NONE', *, *, #9349, .T. ) ;
#10552=ADVANCED_FACE ( 'NONE', ( #29574 ), #3899, .T. ) ;
#10554=CIRCLE ( 'NONE', #18937, 2.000000000000001776 ) ;
#10555=DIRECTION ( 'NONE',  ( 1.000000000000000000, 0.000000000000000000, 0.000000000000000000 ) ) ;
#10556=CARTESIAN_POINT ( 'NONE',  ( 17.14523346298344109, -93.36492675454773860, -49.86561046011506448 ) ) ;
#10558=ORIENTED_EDGE ( 'NONE', *, *, #35657, .F. ) ;
#10559=DIRECTION ( 'NONE',  ( 0.000000000000000000, 0.000000000000000000, 1.000000000000000000 ) ) ;
#10560=CARTESIAN_POINT ( 'NONE',  ( 79.99999662536832545, -34.64101615137759183, -9.999999999999998224 ) ) ;
#10561=EDGE_CURVE ( 'NONE', #31248, #10841, #11050, .T. ) ;
#10562=CIRCLE ( 'NONE', #31499, 2.000000000000001776 ) ;
#10564=EDGE_CURVE ( 'NONE', #3670, #16140, #3295, .T. ) ;
#10565=CARTESIAN_POINT ( 'NONE',  ( -10.00000337463127842, -69.28203230275519786, -9.999999999999998224 ) ) ;
#10566=EDGE_CURVE ( 'NONE', #36232, #3839, #9877, .T. ) ;
#10569=DIRECTION ( 'NONE',  ( 1.000000000000000000, 0.000000000000000000, 0.000000000000000000 ) ) ;
#10570=FACE_BOUND ( 'NONE', #4418, .T. ) ;
#10571=CARTESIAN_POINT ( 'NONE',  ( 39.99999662536853151, -69.28203230275519786, -5.000000000000000000 ) ) ;
#10572=DIRECTION ( 'NONE',  ( 1.000000000000000000, 0.000000000000000000, 0.000000000000000000 ) ) ;
#10574=AXIS2_PLACEMENT_3D ( 'NONE', #27237, #35897, #29883 ) ;
#10575=CARTESIAN_POINT ( 'NONE',  ( 44.13139720814401556, -27.50000000000022737, -10.00000000000000178 ) ) ;
#10577=CIRCLE ( 'NONE', #14184, 2.000000000000001776 ) ;
#10578=DIRECTION ( 'NONE',  ( 0.000000000000000000, 0.000000000000000000, 1.000000000000000000 ) ) ;
#10579=DIRECTION ( 'NONE',  ( 0.000000000000000000, 0.000000000000000000, 1.000000000000000000 ) ) ;
#10580=ORIENTED_EDGE ( 'NONE', *, *, #30354, .F. ) ;
#10582=CARTESIAN_POINT ( 'NONE',  ( -80.00000337463094979, 17.32050807568878525, -9.999999999999998224 ) ) ;
#10583=CARTESIAN_POINT ( 'NONE',  ( -70.00000337463102085, -34.64101615137762025, -9.999999999999998224 ) ) ;
#10584=ORIENTED_EDGE ( 'NONE', *, *, #29111, .T. ) ;
#10585=AXIS2_PLACEMENT_3D ( 'NONE', #18810, #15445, #36065 ) ;
#10586=EDGE_LOOP ( 'NONE', ( #12559, #28465 ) ) ;
#10587=ADVANCED_FACE ( 'NONE', ( #27698 ), #27534, .F. ) ;
#10588=ORIENTED_EDGE ( 'NONE', *, *, #26453, .F. ) ;
#10589=CARTESIAN_POINT ( 'NONE',  ( 77.99999662536832545, -34.64101615137759183, -5.000000000000000000 ) ) ;
#10591=EDGE_CURVE ( 'NONE', #19789, #22214, #30240, .T. ) ;
#10592=VERTEX_POINT ( 'NONE', #7850 ) ;
#10593=CIRCLE ( 'NONE', #26136, 2.000000000000001776 ) ;
#10595=AXIS2_PLACEMENT_3D ( 'NONE', #27717, #8234, #30900 ) ;
#10596=CYLINDRICAL_SURFACE ( 'NONE', #36278, 95.00000000000001421 ) ;
#10597=EDGE_LOOP ( 'NONE', ( #29312, #34213, #23452, #15789 ) ) ;
#10599=ORIENTED_EDGE ( 'NONE', *, *, #1281, .F. ) ;
#10600=EDGE_CURVE ( 'NONE', #35595, #14986, #31575, .T. ) ;
#10601=DIRECTION ( 'NONE',  ( 0.000000000000000000, 0.000000000000000000, -1.000000000000000000 ) ) ;
#10602=AXIS2_PLACEMENT_3D ( 'NONE', #4268, #18697, #1261 ) ;
#10603=AXIS2_PLACEMENT_3D ( 'NONE', #24581, #23826, #26997 ) ;
#10604=AXIS2_PLACEMENT_3D ( 'NONE', #9475, #32133, #35529 ) ;
#10607=DIRECTION ( 'NONE',  ( 0.000000000000000000, 0.000000000000000000, 1.000000000000000000 ) ) ;
#10609=DIRECTION ( 'NONE',  ( 0.000000000000000000, 0.000000000000000000, 1.000000000000000000 ) ) ;
#10611=CIRCLE ( 'NONE', #34576, 2.000000000000001776 ) ;
#10612=DIRECTION ( 'NONE',  ( -1.000000000000000000, 0.000000000000000000, 0.000000000000000000 ) ) ;
#10613=ADVANCED_FACE ( 'NONE', ( #4854 ), #13442, .F. ) ;
#10614=DIRECTION ( 'NONE',  ( 0.000000000000000000, 0.000000000000000000, 1.000000000000000000 ) ) ;
#10615=EDGE_CURVE ( 'NONE', #36125, #35067, #6291, .T. ) ;
#10616=ORIENTED_EDGE ( 'NONE', *, *, #15856, .T. ) ;
#10617=DIRECTION ( 'NONE',  ( -0.000000000000000000, -0.000000000000000000, 1.000000000000000000 ) ) ;
#10620=ORIENTED_EDGE ( 'NONE', *, *, #34389, .F. ) ;
#10621=DIRECTION ( 'NONE',  ( 1.000000000000000000, 0.000000000000000000, 0.000000000000000000 ) ) ;
#10622=AXIS2_PLACEMENT_3D ( 'NONE', #10214, #15466, #21642 ) ;
#10623=CARTESIAN_POINT ( 'NONE',  ( 19.13981058454793072, -60.93295298010985306, 12.49999999999999822 ) ) ;
#10626=ORIENTED_EDGE ( 'NONE', *, *, #7074, .F. ) ;
#10627=CIRCLE ( 'NONE', #31561, 2.000000000000000000 ) ;
#10629=CARTESIAN_POINT ( 'NONE',  ( -7.000003374631307729, 77.94228634059957983, 12.50000000000000000 ) ) ;
#10630=DIRECTION ( 'NONE',  ( 0.000000000000000000, 0.000000000000000000, 1.000000000000000000 ) ) ;
#10631=AXIS2_PLACEMENT_3D ( 'NONE', #24843, #13219, #7040 ) ;
#10632=CARTESIAN_POINT ( 'NONE',  ( -73.00000337463097821, 8.660254037844374864, 17.49999999999999645 ) ) ;
#10633=CIRCLE ( 'NONE', #31571, 3.000000000000002665 ) ;
#10634=VERTEX_POINT ( 'NONE', #8704 ) ;
#10635=VERTEX_POINT ( 'NONE', #36347 ) ;
#10639=CARTESIAN_POINT ( 'NONE',  ( -73.90204618161054384, 6.988581222280664917, 12.50000000000000000 ) ) ;
#10640=AXIS2_PLACEMENT_3D ( 'NONE', #26556, #20203, #5968 ) ;
#10642=EDGE_CURVE ( 'NONE', #23924, #18775, #16467, .T. ) ;
#10643=VERTEX_POINT ( 'NONE', #8014 ) ;
#10646=AXIS2_PLACEMENT_3D ( 'NONE', #15058, #32305, #18226 ) ;
#10647=DIRECTION ( 'NONE',  ( 0.000000000000000000, 0.000000000000000000, 1.000000000000000000 ) ) ;
#10648=VERTEX_POINT ( 'NONE', #1845 ) ;
#10649=CARTESIAN_POINT ( 'NONE',  ( 64.99999662536839651, -43.30127018922199511, 12.50000000000000000 ) ) ;
#10651=CIRCLE ( 'NONE', #16060, 1.999999999999998224 ) ;
#10652=CIRCLE ( 'NONE', #31588, 95.00000000000000000 ) ;
#10653=DIRECTION ( 'NONE',  ( 1.000000000000000000, 0.000000000000000000, 0.000000000000000000 ) ) ;
#10654=CIRCLE ( 'NONE', #22027, 2.000000000000001776 ) ;
#10655=AXIS2_PLACEMENT_3D ( 'NONE', #13166, #27209, #19179 ) ;
#10657=CARTESIAN_POINT ( 'NONE',  ( -75.00000337463097821, -8.660254037844422825, 12.50000000000000000 ) ) ;
#10658=ORIENTED_EDGE ( 'NONE', *, *, #2747, .F. ) ;
#10659=DIRECTION ( 'NONE',  ( 0.000000000000000000, 0.000000000000000000, 1.000000000000000000 ) ) ;
#10660=AXIS2_PLACEMENT_3D ( 'NONE', #30725, #7878, #18935 ) ;
#10661=CARTESIAN_POINT ( 'NONE',  ( -62.00000337463104927, 34.64101615137757051, -9.999999999999998224 ) ) ;
#10662=DIRECTION ( 'NONE',  ( 1.000000000000000000, 0.000000000000000000, 0.000000000000000000 ) ) ;
#10664=ORIENTED_EDGE ( 'NONE', *, *, #15903, .T. ) ;
#10665=DIRECTION ( 'NONE',  ( 0.000000000000000000, 0.000000000000000000, -1.000000000000000000 ) ) ;
#10666=CARTESIAN_POINT ( 'NONE',  ( 62.99999662536841072, -25.98076211353320275, -9.999999999999998224 ) ) ;
#10667=CIRCLE ( 'NONE', #14246, 2.000000000000000000 ) ;
#10668=DIRECTION ( 'NONE',  ( 1.000000000000000000, 0.000000000000000000, 0.000000000000000000 ) ) ;
#10670=EDGE_LOOP ( 'NONE', ( #13191, #35125 ) ) ;
#10671=VERTEX_POINT ( 'NONE', #11514 ) ;
#10672=AXIS2_PLACEMENT_3D ( 'NONE', #15961, #6958, #12945 ) ;
#10674=EDGE_LOOP ( 'NONE', ( #19878, #31690 ) ) ;
#10675=AXIS2_PLACEMENT_3D ( 'NONE', #16042, #7591, #19588 ) ;
#10677=LINE ( 'NONE', #34114, #1594 ) ;
#10678=FACE_OUTER_BOUND ( 'NONE', #36048, .T. ) ;
#10679=CIRCLE ( 'NONE', #23849, 2.000000000000001776 ) ;
#10680=CARTESIAN_POINT ( 'NONE',  ( 57.99999662536843914, -34.64101615137759893, -9.999999999999998224 ) ) ;
#10682=FACE_OUTER_BOUND ( 'NONE', #32593, .T. ) ;
#10683=CARTESIAN_POINT ( 'NONE',  ( 69.99999662536839651, 17.32050807568879236, 12.50000000000000000 ) ) ;
#10684=ADVANCED_FACE ( 'NONE', ( #22961 ), #30333, .F. ) ;
#10685=DIRECTION ( 'NONE',  ( 1.000000000000000000, 0.000000000000000000, 0.000000000000000000 ) ) ;
#10686=ORIENTED_EDGE ( 'NONE', *, *, #2290, .T. ) ;
#10689=AXIS2_PLACEMENT_3D ( 'NONE', #30444, #4772, #27624 ) ;
#10690=CARTESIAN_POINT ( 'NONE',  ( 44.99999662536851019, 77.94228634059959404, -9.999999999999998224 ) ) ;
#10691=CARTESIAN_POINT ( 'NONE',  ( -56.67878100130369035, 27.78182860042797131, 12.49999999999999822 ) ) ;
#10692=LINE ( 'NONE', #15942, #3688 ) ;
#10696=CIRCLE ( 'NONE', #29844, 2.000000000000001776 ) ;
#10697=CARTESIAN_POINT ( 'NONE',  ( 32.99999662536855283, -60.62177826491080168, 17.49999999999999645 ) ) ;
#10698=ADVANCED_FACE ( 'NONE', ( #6807 ), #18242, .F. ) ;
#10699=DIRECTION ( 'NONE',  ( -0.000000000000000000, -0.000000000000000000, 1.000000000000000000 ) ) ;
#10700=CIRCLE ( 'NONE', #31641, 3.000000000000004885 ) ;
#10701=EDGE_LOOP ( 'NONE', ( #29239, #28918, #18844, #2588 ) ) ;
#10702=AXIS2_PLACEMENT_3D ( 'NONE', #8943, #14556, #20377 ) ;
#10703=DIRECTION ( 'NONE',  ( 1.000000000000000000, 0.000000000000000000, 0.000000000000000000 ) ) ;
#10704=VERTEX_POINT ( 'NONE', #1008 ) ;
#10706=DIRECTION ( 'NONE',  ( 0.000000000000000000, 0.000000000000000000, 1.000000000000000000 ) ) ;
#10709=EDGE_CURVE ( 'NONE', #1395, #21235, #289, .T. ) ;
#10710=ORIENTED_EDGE ( 'NONE', *, *, #15734, .T. ) ;
#10711=ORIENTED_EDGE ( 'NONE', *, *, #18929, .T. ) ;
#10712=CIRCLE ( 'NONE', #28078, 2.000000000000001776 ) ;
#10713=AXIS2_PLACEMENT_3D ( 'NONE', #5328, #10924, #50 ) ;
#10714=ORIENTED_EDGE ( 'NONE', *, *, #1746, .T. ) ;
#10716=DIRECTION ( 'NONE',  ( 1.000000000000000000, 0.000000000000000000, 0.000000000000000000 ) ) ;
#10717=CARTESIAN_POINT ( 'NONE',  ( 36.99999662536853862, 77.94228634059959404, 17.49999999999999645 ) ) ;
#10718=DIRECTION ( 'NONE',  ( 0.000000000000000000, 0.000000000000000000, 1.000000000000000000 ) ) ;
#10720=EDGE_LOOP ( 'NONE', ( #15586, #21992 ) ) ;
#10721=LINE ( 'NONE', #34162, #11727 ) ;
#10723=CYLINDRICAL_SURFACE ( 'NONE', #28771, 2.000000000000001776 ) ;
#10724=CIRCLE ( 'NONE', #8925, 2.000000000000001776 ) ;
#10725=ADVANCED_FACE ( 'NONE', ( #6084 ), #31919, .T. ) ;
#10726=DIRECTION ( 'NONE',  ( 0.000000000000000000, 0.000000000000000000, -1.000000000000000000 ) ) ;
#10728=DIRECTION ( 'NONE',  ( 0.000000000000000000, 0.000000000000000000, 1.000000000000000000 ) ) ;
#10729=AXIS2_PLACEMENT_3D ( 'NONE', #23427, #18354, #9906 ) ;
#10732=EDGE_CURVE ( 'NONE', #29318, #22484, #30825, .T. ) ;
#10733=VERTEX_POINT ( 'NONE', #23144 ) ;
#10734=DIRECTION ( 'NONE',  ( 1.000000000000000000, 0.000000000000000000, 0.000000000000000000 ) ) ;
#10735=CIRCLE ( 'NONE', #17318, 27.00000000000001421 ) ;
#10736=LINE ( 'NONE', #19350, #34883 ) ;
#10739=EDGE_CURVE ( 'NONE', #19789, #28708, #21063, .T. ) ;
#10740=EDGE_LOOP ( 'NONE', ( #30846, #10295 ) ) ;
#10742=CARTESIAN_POINT ( 'NONE',  ( -12.00000337463127842, -69.28203230275519786, -9.999999999999998224 ) ) ;
#10743=VECTOR ( 'NONE', #2406, 1000.000000000000000 ) ;
#10744=EDGE_CURVE ( 'NONE', #25550, #30229, #35641, .T. ) ;
#10746=AXIS2_PLACEMENT_3D ( 'NONE', #30550, #5233, #33159 ) ;
#10747=CARTESIAN_POINT ( 'NONE',  ( -56.67878100130369035, 27.78182860042797131, -4.999999999999997335 ) ) ;
#10749=ORIENTED_EDGE ( 'NONE', *, *, #3301, .F. ) ;
#10750=CIRCLE ( 'NONE', #7754, 3.000000000000002665 ) ;
#10751=DIRECTION ( 'NONE',  ( 0.000000000000000000, 0.000000000000000000, -1.000000000000000000 ) ) ;
#10753=PLANE ( 'NONE',  #19663 ) ;
#10754=EDGE_LOOP ( 'NONE', ( #30911, #4849, #31524, #4252 ) ) ;
#10755=VERTEX_POINT ( 'NONE', #12223 ) ;
#10757=CIRCLE ( 'NONE', #28705, 33.00000000000001421 ) ;
#10759=DIRECTION ( 'NONE',  ( 0.000000000000000000, 0.000000000000000000, -1.000000000000000000 ) ) ;
#10760=DIRECTION ( 'NONE',  ( 1.000000000000000000, 0.000000000000000000, 0.000000000000000000 ) ) ;
#10762=EDGE_LOOP ( 'NONE', ( #22896, #16590 ) ) ;
#10763=FACE_OUTER_BOUND ( 'NONE', #23840, .T. ) ;
#10764=FACE_BOUND ( 'NONE', #4723, .T. ) ;
#10765=CARTESIAN_POINT ( 'NONE',  ( -32.00000337463118427, 69.28203230275516944, -9.999999999999998224 ) ) ;
#10766=FACE_BOUND ( 'NONE', #11368, .T. ) ;
#10767=FACE_OUTER_BOUND ( 'NONE', #14917, .T. ) ;
#10770=CIRCLE ( 'NONE', #35911, 2.000000000000001776 ) ;
#10771=DIRECTION ( 'NONE',  ( -1.000000000000000000, 0.000000000000000000, 0.000000000000000000 ) ) ;
#10772=EDGE_CURVE ( 'NONE', #2346, #35442, #35040, .T. ) ;
#10773=DIRECTION ( 'NONE',  ( 1.000000000000000000, 0.000000000000000000, 0.000000000000000000 ) ) ;
#10775=CARTESIAN_POINT ( 'NONE',  ( -82.00000337463094979, 17.32050807568878525, 12.50000000000000000 ) ) ;
#10776=CARTESIAN_POINT ( 'NONE',  ( -77.00000337463097821, 25.98076211353318854, -9.999999999999998224 ) ) ;
#10777=AXIS2_PLACEMENT_3D ( 'NONE', #29841, #35483, #35310 ) ;
#10778=DIRECTION ( 'NONE',  ( 1.000000000000000000, 0.000000000000000000, 0.000000000000000000 ) ) ;
#10780=ORIENTED_EDGE ( 'NONE', *, *, #24704, .T. ) ;
#10781=VERTEX_POINT ( 'NONE', #20889 ) ;
#10782=AXIS2_PLACEMENT_3D ( 'NONE', #24869, #2542, #33676 ) ;
#10783=CARTESIAN_POINT ( 'NONE',  ( 24.99999662536859546, -77.94228634059960825, -9.999999999999998224 ) ) ;
#10784=DIRECTION ( 'NONE',  ( 1.000000000000000000, 0.000000000000000000, 0.000000000000000000 ) ) ;
#10785=AXIS2_PLACEMENT_3D ( 'NONE', #30538, #18727, #22104 ) ;
#10786=ORIENTED_EDGE ( 'NONE', *, *, #31871, .F. ) ;
#10787=DIRECTION ( 'NONE',  ( -1.000000000000000000, 0.000000000000000000, 0.000000000000000000 ) ) ;
#10788=ADVANCED_FACE ( 'NONE', ( #23513 ), #32116, .F. ) ;
#10789=DIRECTION ( 'NONE',  ( 0.000000000000000000, 0.000000000000000000, 1.000000000000000000 ) ) ;
#10790=ORIENTED_EDGE ( 'NONE', *, *, #31373, .T. ) ;
#10791=DIRECTION ( 'NONE',  ( 1.000000000000000000, 0.000000000000000000, 0.000000000000000000 ) ) ;
#10792=EDGE_LOOP ( 'NONE', ( #3731, #30810, #31638, #22259 ) ) ;
#10793=CYLINDRICAL_SURFACE ( 'NONE', #19555, 45.00000000000000711 ) ;
#10794=DIRECTION ( 'NONE',  ( 0.000000000000000000, 0.000000000000000000, 1.000000000000000000 ) ) ;
#10795=CARTESIAN_POINT ( 'NONE',  ( -12.00000337463128197, 86.60254037844397601, -9.999999999999998224 ) ) ;
#10796=CIRCLE ( 'NONE', #3593, 2.000000000000001776 ) ;
#10797=ORIENTED_EDGE ( 'NONE', *, *, #28990, .T. ) ;
#10798=DIRECTION ( 'NONE',  ( -1.000000000000000000, 0.000000000000000000, 0.000000000000000000 ) ) ;
#10799=AXIS2_PLACEMENT_3D ( 'NONE', #31486, #14266, #34703 ) ;
#10801=DIRECTION ( 'NONE',  ( 0.000000000000000000, 0.000000000000000000, 1.000000000000000000 ) ) ;
#10803=CIRCLE ( 'NONE', #3017, 2.000000000000000000 ) ;
#10804=EDGE_LOOP ( 'NONE', ( #5177, #87 ) ) ;
#10808=EDGE_CURVE ( 'NONE', #6666, #22417, #32008, .T. ) ;
#10809=FACE_OUTER_BOUND ( 'NONE', #11245, .T. ) ;
#10810=FACE_OUTER_BOUND ( 'NONE', #3363, .T. ) ;
#10811=DIRECTION ( 'NONE',  ( 0.000000000000000000, 0.000000000000000000, -1.000000000000000000 ) ) ;
#10813=EDGE_CURVE ( 'NONE', #13352, #7527, #9249, .T. ) ;
#10814=EDGE_LOOP ( 'NONE', ( #4525, #10875 ) ) ;
#10815=EDGE_LOOP ( 'NONE', ( #1257, #7931 ) ) ;
#10816=EDGE_CURVE ( 'NONE', #31233, #5893, #31757, .T. ) ;
#10818=DIRECTION ( 'NONE',  ( 0.000000000000000000, 0.000000000000000000, -1.000000000000000000 ) ) ;
#10819=EDGE_CURVE ( 'NONE', #33663, #5095, #36256, .T. ) ;
#10820=DIRECTION ( 'NONE',  ( 0.000000000000000000, 0.000000000000000000, 1.000000000000000000 ) ) ;
#10821=EDGE_LOOP ( 'NONE', ( #36685, #16428, #11054, #21144 ) ) ;
#10822=VERTEX_POINT ( 'NONE', #7757 ) ;
#10823=CIRCLE ( 'NONE', #32361, 2.000000000000001776 ) ;
#10826=DIRECTION ( 'NONE',  ( 0.000000000000000000, 0.000000000000000000, -1.000000000000000000 ) ) ;
#10827=EDGE_CURVE ( 'NONE', #2100, #33319, #24814, .T. ) ;
#10828=VERTEX_POINT ( 'NONE', #1370 ) ;
#10829=EDGE_CURVE ( 'NONE', #23537, #30130, #33443, .T. ) ;
#10830=ORIENTED_EDGE ( 'NONE', *, *, #2572, .F. ) ;
#10831=CARTESIAN_POINT ( 'NONE',  ( 56.67878100130369035, -27.78182860042797131, -4.999999999999997335 ) ) ;
#10832=ADVANCED_FACE ( 'NONE', ( #36247 ), #35696, .F. ) ;
#10833=DIRECTION ( 'NONE',  ( 0.000000000000000000, 0.000000000000000000, -1.000000000000000000 ) ) ;
#10835=EDGE_CURVE ( 'NONE', #4001, #10128, #15809, .T. ) ;
#10837=ORIENTED_EDGE ( 'NONE', *, *, #16106, .F. ) ;
#10838=FACE_BOUND ( 'NONE', #11862, .T. ) ;
#10839=DIRECTION ( 'NONE',  ( 1.000000000000000000, 0.000000000000000000, 0.000000000000000000 ) ) ;
#10840=DIRECTION ( 'NONE',  ( 1.000000000000000000, 0.000000000000000000, 0.000000000000000000 ) ) ;
#10841=VERTEX_POINT ( 'NONE', #4569 ) ;
#10844=DIRECTION ( 'NONE',  ( -1.000000000000000000, 0.000000000000000000, 0.000000000000000000 ) ) ;
#10846=CIRCLE ( 'NONE', #34782, 2.000000000000001776 ) ;
#10848=CARTESIAN_POINT ( 'NONE',  ( 81.99999662536833966, -3.469446951953614189E-15, 12.50000000000000000 ) ) ;
#10849=DIRECTION ( 'NONE',  ( 1.000000000000000000, 0.000000000000000000, 0.000000000000000000 ) ) ;
#10850=DIRECTION ( 'NONE',  ( 1.000000000000000000, 0.000000000000000000, 0.000000000000000000 ) ) ;
#10851=VERTEX_POINT ( 'NONE', #21998 ) ;
#10853=DIRECTION ( 'NONE',  ( 0.000000000000000000, 0.000000000000000000, 1.000000000000000000 ) ) ;
#10855=LINE ( 'NONE', #19667, #22333 ) ;
#10856=DIRECTION ( 'NONE',  ( 0.000000000000000000, 0.000000000000000000, 1.000000000000000000 ) ) ;
#10857=CARTESIAN_POINT ( 'NONE',  ( -70.00000337463100664, -17.32050807568882078, -5.000000000000000000 ) ) ;
#10861=AXIS2_PLACEMENT_3D ( 'NONE', #8249, #13861, #32157 ) ;
#10863=DIRECTION ( 'NONE',  ( 0.000000000000000000, 0.000000000000000000, 1.000000000000000000 ) ) ;
#10864=ORIENTED_EDGE ( 'NONE', *, *, #25000, .T. ) ;
#10865=ORIENTED_EDGE ( 'NONE', *, *, #3894, .F. ) ;
#10866=DIRECTION ( 'NONE',  ( -1.000000000000000000, 0.000000000000000000, 0.000000000000000000 ) ) ;
#10867=EDGE_CURVE ( 'NONE', #4612, #11022, #21871, .T. ) ;
#10868=CARTESIAN_POINT ( 'NONE',  ( 79.99999662536832545, -34.64101615137759183, -5.000000000000000000 ) ) ;
#10872=ORIENTED_EDGE ( 'NONE', *, *, #12902, .F. ) ;
#10873=ORIENTED_EDGE ( 'NONE', *, *, #4436, .T. ) ;
#10874=CARTESIAN_POINT ( 'NONE',  ( 56.29165124598892334, 32.49999999999928235, 12.49999999999999822 ) ) ;
#10875=ORIENTED_EDGE ( 'NONE', *, *, #17637, .T. ) ;
#10876=DIRECTION ( 'NONE',  ( 1.000000000000000000, 0.000000000000000000, 0.000000000000000000 ) ) ;
#10879=ORIENTED_EDGE ( 'NONE', *, *, #2027, .F. ) ;
#10880=EDGE_LOOP ( 'NONE', ( #15177, #28707, #8877, #22152 ) ) ;
#10881=AXIS2_PLACEMENT_3D ( 'NONE', #6194, #23455, #29614 ) ;
#10882=EDGE_CURVE ( 'NONE', #35287, #11413, #4006, .T. ) ;
#10883=ORIENTED_EDGE ( 'NONE', *, *, #27259, .F. ) ;
#10884=EDGE_CURVE ( 'NONE', #13905, #32112, #15450, .T. ) ;
#10885=EDGE_LOOP ( 'NONE', ( #28736, #4372, #6622, #11267 ) ) ;
#10886=CARTESIAN_POINT ( 'NONE',  ( -80.00000337463096400, -34.64101615137762025, -9.999999999999998224 ) ) ;
#10887=DIRECTION ( 'NONE',  ( 0.000000000000000000, 0.000000000000000000, 1.000000000000000000 ) ) ;
#10888=CARTESIAN_POINT ( 'NONE',  ( -70.00000337463102085, -34.64101615137762025, -5.000000000000000000 ) ) ;
#10889=DIRECTION ( 'NONE',  ( 0.000000000000000000, 0.000000000000000000, 1.000000000000000000 ) ) ;
#10890=LINE ( 'NONE', #5828, #3357 ) ;
#10893=FACE_OUTER_BOUND ( 'NONE', #23231, .T. ) ;
#10894=ADVANCED_FACE ( 'NONE', ( #21631 ), #27618, .F. ) ;
#10896=ORIENTED_EDGE ( 'NONE', *, *, #2626, .F. ) ;
#10898=CARTESIAN_POINT ( 'NONE',  ( 9.999996625368625658, 86.60254037844397601, 12.50000000000000000 ) ) ;
#10899=ORIENTED_EDGE ( 'NONE', *, *, #11380, .T. ) ;
#10900=ORIENTED_EDGE ( 'NONE', *, *, #21083, .F. ) ;
#10901=DIRECTION ( 'NONE',  ( -0.000000000000000000, 0.000000000000000000, -1.000000000000000000 ) ) ;
#10902=AXIS2_PLACEMENT_3D ( 'NONE', #9044, #3971, #9608 ) ;
#10907=ORIENTED_EDGE ( 'NONE', *, *, #23248, .F. ) ;
#10908=ORIENTED_EDGE ( 'NONE', *, *, #26107, .T. ) ;
#10909=DIRECTION ( 'NONE',  ( 0.000000000000000000, 0.000000000000000000, 1.000000000000000000 ) ) ;
#10910=ORIENTED_EDGE ( 'NONE', *, *, #5860, .T. ) ;
#10911=DIRECTION ( 'NONE',  ( 1.000000000000000000, 0.000000000000000000, 0.000000000000000000 ) ) ;
#10912=ORIENTED_EDGE ( 'NONE', *, *, #30515, .T. ) ;
#10913=ORIENTED_EDGE ( 'NONE', *, *, #1881, .F. ) ;
#10914=VECTOR ( 'NONE', #30012, 1000.000000000000000 ) ;
#10916=CARTESIAN_POINT ( 'NONE',  ( 54.99999662536844625, 43.30127018922198801, -5.000000000000000000 ) ) ;
#10918=DIRECTION ( 'NONE',  ( 0.000000000000000000, 0.000000000000000000, -1.000000000000000000 ) ) ;
#10919=VERTEX_POINT ( 'NONE', #24072 ) ;
#10921=CARTESIAN_POINT ( 'NONE',  ( -37.00000337463116296, -60.62177826491080168, -9.999999999999998224 ) ) ;
#10922=LINE ( 'NONE', #7762, #36905 ) ;
#10923=CARTESIAN_POINT ( 'NONE',  ( -58.00000337463108480, -51.96152422706641971, -5.000000000000000000 ) ) ;
#10924=DIRECTION ( 'NONE',  ( 0.000000000000000000, 0.000000000000000000, 1.000000000000000000 ) ) ;
#10925=EDGE_LOOP ( 'NONE', ( #24624, #5894 ) ) ;
#10926=DIRECTION ( 'NONE',  ( 0.000000000000000000, 0.000000000000000000, 1.000000000000000000 ) ) ;
#10928=AXIS2_PLACEMENT_3D ( 'NONE', #21963, #30590, #4908 ) ;
#10929=FACE_BOUND ( 'NONE', #13281, .T. ) ;
#10930=EDGE_CURVE ( 'NONE', #14423, #3735, #18250, .T. ) ;
#10931=CARTESIAN_POINT ( 'NONE',  ( -31.46585318596190106, -86.45172111230344569, -4.999999999999997335 ) ) ;
#10932=FACE_OUTER_BOUND ( 'NONE', #1272, .T. ) ;
#10933=DIRECTION ( 'NONE',  ( -1.000000000000000000, 0.000000000000000000, 0.000000000000000000 ) ) ;
#10934=DIRECTION ( 'NONE',  ( -1.000000000000000000, 0.000000000000000000, 0.000000000000000000 ) ) ;
#10935=CARTESIAN_POINT ( 'NONE',  ( 79.99999662536833966, 34.64101615137759183, -9.999999999999998224 ) ) ;
#10937=CARTESIAN_POINT ( 'NONE',  ( -70.00000337463100664, -17.32050807568882078, 17.49999999999999645 ) ) ;
#10938=VERTEX_POINT ( 'NONE', #4209 ) ;
#10939=DIRECTION ( 'NONE',  ( 0.000000000000000000, 0.000000000000000000, 1.000000000000000000 ) ) ;
#10940=DIRECTION ( 'NONE',  ( 0.000000000000000000, 0.000000000000000000, 1.000000000000000000 ) ) ;
#10941=FACE_OUTER_BOUND ( 'NONE', #9699, .T. ) ;
#10942=ORIENTED_EDGE ( 'NONE', *, *, #28199, .T. ) ;
#10943=CIRCLE ( 'NONE', #12719, 33.00000000000002132 ) ;
#10944=ORIENTED_EDGE ( 'NONE', *, *, #32012, .T. ) ;
#10945=ORIENTED_EDGE ( 'NONE', *, *, #20381, .T. ) ;
#10946=CARTESIAN_POINT ( 'NONE',  ( -70.00000337463099243, 34.64101615137758472, 12.50000000000000000 ) ) ;
#10947=DIRECTION ( 'NONE',  ( 1.000000000000000000, 0.000000000000000000, 0.000000000000000000 ) ) ;
#10949=DIRECTION ( 'NONE',  ( 0.000000000000000000, 0.000000000000000000, -1.000000000000000000 ) ) ;
#10950=ADVANCED_FACE ( 'NONE', ( #24451 ), #10000, .F. ) ;
#10952=VERTEX_POINT ( 'NONE', #27233 ) ;
#10953=CIRCLE ( 'NONE', #31887, 2.000000000000001776 ) ;
#10954=CARTESIAN_POINT ( 'NONE',  ( -81.86307664143558327, 18.04780306571548820, 12.50000000000000000 ) ) ;
#10956=DIRECTION ( 'NONE',  ( 0.000000000000000000, 0.000000000000000000, -1.000000000000000000 ) ) ;
#10957=EDGE_CURVE ( 'NONE', #18409, #36079, #34049, .T. ) ;
#10958=FACE_OUTER_BOUND ( 'NONE', #16418, .T. ) ;
#10959=CARTESIAN_POINT ( 'NONE',  ( 52.39915983220795681, 35.19434990244919703, -4.999999999999997335 ) ) ;
#10960=ADVANCED_FACE ( 'NONE', ( #33058 ), #19557, .F. ) ;
#10961=ORIENTED_EDGE ( 'NONE', *, *, #32538, .F. ) ;
#10962=FACE_OUTER_BOUND ( 'NONE', #24810, .T. ) ;
#10963=AXIS2_PLACEMENT_3D ( 'NONE', #22217, #27470, #10396 ) ;
#10966=CARTESIAN_POINT ( 'NONE',  ( -73.00000337463099243, -25.98076211353322051, -9.999999999999998224 ) ) ;
#10967=AXIS2_PLACEMENT_3D ( 'NONE', #8430, #16690, #19859 ) ;
#10968=ORIENTED_EDGE ( 'NONE', *, *, #71, .T. ) ;
#10969=DIRECTION ( 'NONE',  ( -1.000000000000000000, 0.000000000000000000, 0.000000000000000000 ) ) ;
#10970=DIRECTION ( 'NONE',  ( -1.000000000000000000, 0.000000000000000000, 0.000000000000000000 ) ) ;
#10971=VERTEX_POINT ( 'NONE', #2493 ) ;
#10972=CARTESIAN_POINT ( 'NONE',  ( 91.99999662536828282, 0.000000000000000000, 17.49999999999999645 ) ) ;
#10973=CARTESIAN_POINT ( 'NONE',  ( -45.00000337463112743, -60.62177826491080168, 17.49999999999999645 ) ) ;
#10974=DIRECTION ( 'NONE',  ( 0.000000000000000000, 0.000000000000000000, 1.000000000000000000 ) ) ;
#10975=CYLINDRICAL_SURFACE ( 'NONE', #15274, 2.000000000000001776 ) ;
#10976=ORIENTED_EDGE ( 'NONE', *, *, #25814, .T. ) ;
#10978=VECTOR ( 'NONE', #12766, 1000.000000000000000 ) ;
#10980=CARTESIAN_POINT ( 'NONE',  ( 64.99999662536839651, 60.62177826491078747, -9.999999999999998224 ) ) ;
#10981=CARTESIAN_POINT ( 'NONE',  ( -62.00000337463104927, 34.64101615137757051, 17.49999999999999645 ) ) ;
#10983=ORIENTED_EDGE ( 'NONE', *, *, #11948, .F. ) ;
#10984=DIRECTION ( 'NONE',  ( 0.000000000000000000, 0.000000000000000000, 1.000000000000000000 ) ) ;
#10988=EDGE_LOOP ( 'NONE', ( #24205, #31700 ) ) ;
#10989=EDGE_LOOP ( 'NONE', ( #24792, #8922, #8827, #29600, #5442, #10908, #3742, #19947, #16552, #5685, #17826, #13386, #22607, #23115, #23947, #2896, #7205, #6444, #23096, #34545, #6301, #21013, #1177, #24295 ) ) ;
#10990=CIRCLE ( 'NONE', #34960, 27.00000000000001066 ) ;
#10991=DIRECTION ( 'NONE',  ( -0.000000000000000000, -0.000000000000000000, -1.000000000000000000 ) ) ;
#10992=ADVANCED_FACE ( 'NONE', ( #36624 ), #10753, .F. ) ;
#10993=CYLINDRICAL_SURFACE ( 'NONE', #17096, 2.000000000000001776 ) ;
#10994=ORIENTED_EDGE ( 'NONE', *, *, #27526, .T. ) ;
#10995=EDGE_CURVE ( 'NONE', #11751, #27540, #31034, .T. ) ;
#10996=CARTESIAN_POINT ( 'NONE',  ( -8.000003374631281972, 86.60254037844397601, 12.50000000000000000 ) ) ;
#10997=VERTEX_POINT ( 'NONE', #34190 ) ;
#10998=FACE_BOUND ( 'NONE', #20947, .T. ) ;
#10999=VECTOR ( 'NONE', #14845, 1000.000000000000000 ) ;
#11000=EDGE_CURVE ( 'NONE', #27568, #11237, #17860, .T. ) ;
#11001=CARTESIAN_POINT ( 'NONE',  ( 84.99999662536831124, -25.98076211353319565, 12.50000000000000000 ) ) ;
#11002=CIRCLE ( 'NONE', #207, 2.000000000000001776 ) ;
#11003=EDGE_CURVE ( 'NONE', #4892, #8845, #33800, .T. ) ;
#11004=ORIENTED_EDGE ( 'NONE', *, *, #14187, .F. ) ;
#11005=EDGE_CURVE ( 'NONE', #26527, #23588, #5116, .T. ) ;
#11007=DIRECTION ( 'NONE',  ( 0.000000000000000000, 0.000000000000000000, 1.000000000000000000 ) ) ;
#11008=DIRECTION ( 'NONE',  ( 0.000000000000000000, 0.000000000000000000, 1.000000000000000000 ) ) ;
#11009=DIRECTION ( 'NONE',  ( 0.000000000000000000, 0.000000000000000000, 1.000000000000000000 ) ) ;
#11010=ORIENTED_EDGE ( 'NONE', *, *, #1277, .F. ) ;
#11011=DIRECTION ( 'NONE',  ( 0.000000000000000000, 0.000000000000000000, 1.000000000000000000 ) ) ;
#11012=CYLINDRICAL_SURFACE ( 'NONE', #10063, 27.00000000000001066 ) ;
#11013=DIRECTION ( 'NONE',  ( 0.000000000000000000, 0.000000000000000000, 1.000000000000000000 ) ) ;
#11014=EDGE_CURVE ( 'NONE', #27066, #20492, #14253, .T. ) ;
#11015=ADVANCED_FACE ( 'NONE', ( #28175 ), #13546, .F. ) ;
#11016=ORIENTED_EDGE ( 'NONE', *, *, #35796, .T. ) ;
#11018=VERTEX_POINT ( 'NONE', #25549 ) ;
#11019=ADVANCED_FACE ( 'NONE', ( #2313 ), #36793, .F. ) ;
#11020=EDGE_CURVE ( 'NONE', #2812, #23997, #11097, .T. ) ;
#11021=DIRECTION ( 'NONE',  ( 0.000000000000000000, 0.000000000000000000, 1.000000000000000000 ) ) ;
#11022=VERTEX_POINT ( 'NONE', #7930 ) ;
#11024=CARTESIAN_POINT ( 'NONE',  ( 4.279621169095998212, -62.97617850287780072, 12.49999999999999822 ) ) ;
#11026=CIRCLE ( 'NONE', #17599, 3.499999999999989342 ) ;
#11028=VECTOR ( 'NONE', #29428, 1000.000000000000000 ) ;
#11029=DIRECTION ( 'NONE',  ( 0.000000000000000000, 0.000000000000000000, 1.000000000000000000 ) ) ;
#11031=CARTESIAN_POINT ( 'NONE',  ( 77.99999662536833966, -3.224517592124143893E-15, -9.999999999999998224 ) ) ;
#11033=CARTESIAN_POINT ( 'NONE',  ( 81.99999662536832545, -34.64101615137759183, -9.999999999999998224 ) ) ;
#11034=ORIENTED_EDGE ( 'NONE', *, *, #27473, .T. ) ;
#11035=VERTEX_POINT ( 'NONE', #22545 ) ;
#11037=CARTESIAN_POINT ( 'NONE',  ( -51.13139720814380240, 27.50000000000055422, -10.00000000000000000 ) ) ;
#11038=DIRECTION ( 'NONE',  ( 0.000000000000000000, 0.000000000000000000, 1.000000000000000000 ) ) ;
#11039=AXIS2_PLACEMENT_3D ( 'NONE', #15556, #18565, #1118 ) ;
#11040=DIRECTION ( 'NONE',  ( 1.000000000000000000, 0.000000000000000000, 0.000000000000000000 ) ) ;
#11042=CIRCLE ( 'NONE', #15846, 2.000000000000001776 ) ;
#11043=FACE_OUTER_BOUND ( 'NONE', #14030, .T. ) ;
#11044=ORIENTED_EDGE ( 'NONE', *, *, #25361, .F. ) ;
#11045=ORIENTED_EDGE ( 'NONE', *, *, #35695, .T. ) ;
#11046=DIRECTION ( 'NONE',  ( 1.000000000000000000, 0.000000000000000000, 0.000000000000000000 ) ) ;
#11047=ORIENTED_EDGE ( 'NONE', *, *, #34446, .T. ) ;
#11049=AXIS2_PLACEMENT_3D ( 'NONE', #32009, #31829, #17593 ) ;
#11050=CIRCLE ( 'NONE', #31982, 2.000000000000001776 ) ;
#11052=AXIS2_PLACEMENT_3D ( 'NONE', #2983, #5241, #16678 ) ;
#11053=CARTESIAN_POINT ( 'NONE',  ( -73.00000337463097821, 43.30127018922197379, -9.999999999999998224 ) ) ;
#11054=ORIENTED_EDGE ( 'NONE', *, *, #7335, .T. ) ;
#11055=ORIENTED_EDGE ( 'NONE', *, *, #2306, .T. ) ;
#11056=ORIENTED_EDGE ( 'NONE', *, *, #20907, .T. ) ;
#11057=ADVANCED_FACE ( 'NONE', ( #14095, #36992, #2871, #5661, #30615, #4931, #16367 ), #13746, .F. ) ;
#11060=EDGE_CURVE ( 'NONE', #13754, #17529, #13068, .T. ) ;
#11062=CARTESIAN_POINT ( 'NONE',  ( 7.999996625368656744, -69.28203230275519786, -9.999999999999998224 ) ) ;
#11063=EDGE_CURVE ( 'NONE', #11374, #26778, #3499, .T. ) ;
#11064=DIRECTION ( 'NONE',  ( 0.000000000000000000, 0.000000000000000000, 1.000000000000000000 ) ) ;
#11066=FACE_OUTER_BOUND ( 'NONE', #19392, .T. ) ;
#11067=LINE ( 'NONE', #3022, #13925 ) ;
#11069=ORIENTED_EDGE ( 'NONE', *, *, #19768, .F. ) ;
#11070=CARTESIAN_POINT ( 'NONE',  ( 69.99999662536839651, -3.469446951953614189E-15, 17.49999999999999645 ) ) ;
#11071=AXIS2_PLACEMENT_3D ( 'NONE', #35633, #13682, #19682 ) ;
#11073=DIRECTION ( 'NONE',  ( 1.000000000000000000, 0.000000000000000000, 0.000000000000000000 ) ) ;
#11074=EDGE_LOOP ( 'NONE', ( #11303, #32331, #22218, #19318 ) ) ;
#11075=DIRECTION ( 'NONE',  ( -0.000000000000000000, -0.000000000000000000, -1.000000000000000000 ) ) ;
#11076=DIRECTION ( 'NONE',  ( 0.000000000000000000, 0.000000000000000000, 1.000000000000000000 ) ) ;
#11077=AXIS2_PLACEMENT_3D ( 'NONE', #34649, #508, #11933 ) ;
#11078=ORIENTED_EDGE ( 'NONE', *, *, #27206, .T. ) ;
#11079=ORIENTED_EDGE ( 'NONE', *, *, #23159, .F. ) ;
#11081=CARTESIAN_POINT ( 'NONE',  ( -20.00000337463124112, 69.28203230275516944, -9.999999999999998224 ) ) ;
#11082=DIRECTION ( 'NONE',  ( -0.000000000000000000, -0.000000000000000000, 1.000000000000000000 ) ) ;
#11083=DIRECTION ( 'NONE',  ( 0.000000000000000000, 0.000000000000000000, 1.000000000000000000 ) ) ;
#11085=ORIENTED_EDGE ( 'NONE', *, *, #945, .T. ) ;
#11086=EDGE_CURVE ( 'NONE', #11561, #10755, #208, .T. ) ;
#11087=CARTESIAN_POINT ( 'NONE',  ( -75.00000337463097821, 43.30127018922197379, -9.999999999999998224 ) ) ;
#11088=CIRCLE ( 'NONE', #35648, 27.00000000000001421 ) ;
#11089=ORIENTED_EDGE ( 'NONE', *, *, #26872, .F. ) ;
#11091=CARTESIAN_POINT ( 'NONE',  ( -83.00000337463092137, -25.98076211353322051, -9.999999999999998224 ) ) ;
#11092=EDGE_LOOP ( 'NONE', ( #19579, #6386, #30856, #24424 ) ) ;
#11093=VECTOR ( 'NONE', #34728, 1000.000000000000000 ) ;
#11097=LINE ( 'NONE', #28342, #31609 ) ;
#11099=ORIENTED_EDGE ( 'NONE', *, *, #13246, .F. ) ;
#11103=LINE ( 'NONE', #2115, #23463 ) ;
#11104=CIRCLE ( 'NONE', #14103, 2.000000000000000000 ) ;
#11105=DIRECTION ( 'NONE',  ( 0.000000000000000000, 0.000000000000000000, 1.000000000000000000 ) ) ;
#11106=ORIENTED_EDGE ( 'NONE', *, *, #35027, .T. ) ;
#11107=DIRECTION ( 'NONE',  ( 1.000000000000000000, 0.000000000000000000, 0.000000000000000000 ) ) ;
#11108=ADVANCED_FACE ( 'NONE', ( #32062 ), #23850, .F. ) ;
#11109=FACE_BOUND ( 'NONE', #31736, .T. ) ;
#11110=DIRECTION ( 'NONE',  ( 1.000000000000000000, 0.000000000000000000, 0.000000000000000000 ) ) ;
#11111=DIRECTION ( 'NONE',  ( 1.000000000000000000, 0.000000000000000000, 0.000000000000000000 ) ) ;
#11112=CYLINDRICAL_SURFACE ( 'NONE', #16504, 2.000000000000001776 ) ;
#11113=DIRECTION ( 'NONE',  ( 0.000000000000000000, 0.000000000000000000, 1.000000000000000000 ) ) ;
#11114=CARTESIAN_POINT ( 'NONE',  ( 43.19957991610432657, 47.04203867989531318, 12.49999999999999822 ) ) ;
#11116=DIRECTION ( 'NONE',  ( 1.000000000000000000, 0.000000000000000000, 0.000000000000000000 ) ) ;
#11117=ORIENTED_EDGE ( 'NONE', *, *, #10160, .F. ) ;
#11118=DIRECTION ( 'NONE',  ( 0.000000000000000000, 0.000000000000000000, 1.000000000000000000 ) ) ;
#11119=AXIS2_PLACEMENT_3D ( 'NONE', #4177, #24784, #27202 ) ;
#11120=FACE_OUTER_BOUND ( 'NONE', #21957, .T. ) ;
#11121=CARTESIAN_POINT ( 'NONE',  ( 45.00000000000000711, 0.000000000000000000, -10.00000000000000000 ) ) ;
#11123=AXIS2_PLACEMENT_3D ( 'NONE', #20956, #30117, #9875 ) ;
#11124=AXIS2_PLACEMENT_3D ( 'NONE', #27824, #16047, #28027 ) ;
#11125=EDGE_LOOP ( 'NONE', ( #8258, #30095, #35405, #17176 ) ) ;
#11126=CIRCLE ( 'NONE', #14718, 2.000000000000001776 ) ;
#11127=EDGE_LOOP ( 'NONE', ( #15442, #21978, #4469, #8084 ) ) ;
#11128=ORIENTED_EDGE ( 'NONE', *, *, #3705, .T. ) ;
#11130=FACE_OUTER_BOUND ( 'NONE', #8796, .T. ) ;
#11132=EDGE_LOOP ( 'NONE', ( #18921, #15429 ) ) ;
#11134=EDGE_CURVE ( 'NONE', #24333, #719, #22636, .T. ) ;
#11135=AXIS2_PLACEMENT_3D ( 'NONE', #8154, #10956, #36833 ) ;
#11136=LINE ( 'NONE', #36655, #19127 ) ;
#11137=EDGE_LOOP ( 'NONE', ( #27876, #27777 ) ) ;
#11139=ADVANCED_FACE ( 'NONE', ( #31713 ), #9398, .F. ) ;
#11140=ORIENTED_EDGE ( 'NONE', *, *, #11528, .F. ) ;
#11141=DIRECTION ( 'NONE',  ( -0.000000000000000000, -0.000000000000000000, 1.000000000000000000 ) ) ;
#11142=EDGE_LOOP ( 'NONE', ( #3726, #5525, #34998, #32602 ) ) ;
#11144=CARTESIAN_POINT ( 'NONE',  ( -72.00000337463100664, 51.96152422706637708, -9.999999999999998224 ) ) ;
#11145=CARTESIAN_POINT ( 'NONE',  ( 84.99999662536832545, 8.660254037844394404, 17.49999999999999645 ) ) ;
#11147=ORIENTED_EDGE ( 'NONE', *, *, #8202, .T. ) ;
#11149=DIRECTION ( 'NONE',  ( 0.000000000000000000, 0.000000000000000000, -1.000000000000000000 ) ) ;
#11151=AXIS2_PLACEMENT_3D ( 'NONE', #22550, #28179, #5496 ) ;
#11153=CIRCLE ( 'NONE', #35124, 2.000000000000001776 ) ;
#11154=DIRECTION ( 'NONE',  ( -0.000000000000000000, -0.000000000000000000, 1.000000000000000000 ) ) ;
#11156=AXIS2_PLACEMENT_3D ( 'NONE', #36164, #21909, #27708 ) ;
#11157=EDGE_LOOP ( 'NONE', ( #20669, #1568 ) ) ;
#11158=CARTESIAN_POINT ( 'NONE',  ( 56.67878100130369035, -27.78182860042797131, -4.999999999999997335 ) ) ;
#11159=CARTESIAN_POINT ( 'NONE',  ( -60.00000337463104216, 34.64101615137757051, -9.999999999999998224 ) ) ;
#11160=ORIENTED_EDGE ( 'NONE', *, *, #7129, .T. ) ;
#11161=EDGE_CURVE ( 'NONE', #23429, #7967, #11851, .T. ) ;
#11162=DIRECTION ( 'NONE',  ( -1.000000000000000000, 0.000000000000000000, 0.000000000000000000 ) ) ;
#11164=DIRECTION ( 'NONE',  ( 0.000000000000000000, 0.000000000000000000, 1.000000000000000000 ) ) ;
#11166=AXIS2_PLACEMENT_3D ( 'NONE', #23507, #34946, #8891 ) ;
#11167=ORIENTED_EDGE ( 'NONE', *, *, #437, .F. ) ;
#11168=ORIENTED_EDGE ( 'NONE', *, *, #25462, .F. ) ;
#11170=DIRECTION ( 'NONE',  ( 1.000000000000000000, 0.000000000000000000, 0.000000000000000000 ) ) ;
#11171=AXIS2_PLACEMENT_3D ( 'NONE', #3064, #5874, #14655 ) ;
#11172=ADVANCED_FACE ( 'NONE', ( #29448 ), #15205, .F. ) ;
#11173=EDGE_LOOP ( 'NONE', ( #23237, #9717, #12773, #23059, #20293 ) ) ;
#11175=EDGE_CURVE ( 'NONE', #3360, #630, #24462, .T. ) ;
#11178=DIRECTION ( 'NONE',  ( 0.000000000000000000, 0.000000000000000000, 1.000000000000000000 ) ) ;
#11180=AXIS2_PLACEMENT_3D ( 'NONE', #19259, #26948, #17179 ) ;
#11181=ORIENTED_EDGE ( 'NONE', *, *, #14853, .T. ) ;
#11182=VECTOR ( 'NONE', #17488, 1000.000000000000000 ) ;
#11183=ORIENTED_EDGE ( 'NONE', *, *, #531, .F. ) ;
#11184=DIRECTION ( 'NONE',  ( 1.000000000000000000, 0.000000000000000000, 0.000000000000000000 ) ) ;
#11185=AXIS2_PLACEMENT_3D ( 'NONE', #10072, #13059, #35008 ) ;
#11186=CYLINDRICAL_SURFACE ( 'NONE', #14089, 3.000000000000006217 ) ;
#11187=ORIENTED_EDGE ( 'NONE', *, *, #34431, .F. ) ;
#11188=DIRECTION ( 'NONE',  ( 0.000000000000000000, 0.000000000000000000, 1.000000000000000000 ) ) ;
#11190=ORIENTED_EDGE ( 'NONE', *, *, #2357, .F. ) ;
#11191=FACE_BOUND ( 'NONE', #10674, .T. ) ;
#11192=AXIS2_PLACEMENT_3D ( 'NONE', #17094, #25355, #14086 ) ;
#11193=EDGE_CURVE ( 'NONE', #5840, #17343, #16055, .T. ) ;
#11194=CARTESIAN_POINT ( 'NONE',  ( 9.999996625368618552, 69.28203230275516944, -9.999999999999998224 ) ) ;
#11200=AXIS2_PLACEMENT_3D ( 'NONE', #29344, #12071, #32344 ) ;
#11202=DIRECTION ( 'NONE',  ( -1.000000000000000000, 0.000000000000000000, 0.000000000000000000 ) ) ;
#11203=ORIENTED_EDGE ( 'NONE', *, *, #36146, .T. ) ;
#11204=CARTESIAN_POINT ( 'NONE',  ( 79.99999662536832545, -17.32050807568879591, 17.49999999999999645 ) ) ;
#11205=CARTESIAN_POINT ( 'NONE',  ( -79.83584802575171580, -32.64776428033012934, 12.50000000000000000 ) ) ;
#11207=AXIS2_PLACEMENT_3D ( 'NONE', #31214, #13955, #36662 ) ;
#11209=EDGE_LOOP ( 'NONE', ( #27750, #35234, #31095, #21229 ) ) ;
#11210=CIRCLE ( 'NONE', #19601, 2.999999999999999556 ) ;
#11211=EDGE_CURVE ( 'NONE', #27018, #1819, #11638, .T. ) ;
#11212=ORIENTED_EDGE ( 'NONE', *, *, #29687, .T. ) ;
#11213=VERTEX_POINT ( 'NONE', #23291 ) ;
#11214=CARTESIAN_POINT ( 'NONE',  ( 67.99999662536838230, -3.224517592124143893E-15, 12.50000000000000000 ) ) ;
#11215=AXIS2_PLACEMENT_3D ( 'NONE', #29735, #15871, #30109 ) ;
#11216=CARTESIAN_POINT ( 'NONE',  ( -5.000003374631269537, -77.94228634059960825, -9.999999999999998224 ) ) ;
#11217=VECTOR ( 'NONE', #12742, 1000.000000000000000 ) ;
#11219=CARTESIAN_POINT ( 'NONE',  ( -78.00000337463094979, -17.32050807568882078, 17.49999999999999645 ) ) ;
#11221=CARTESIAN_POINT ( 'NONE',  ( 42.99999662536848888, 60.62177826491077326, 17.49999999999999645 ) ) ;
#11222=EDGE_CURVE ( 'NONE', #16746, #8683, #25641, .T. ) ;
#11225=EDGE_CURVE ( 'NONE', #4653, #3063, #11833, .T. ) ;
#11227=AXIS2_PLACEMENT_3D ( 'NONE', #23914, #24649, #32506 ) ;
#11229=EDGE_LOOP ( 'NONE', ( #13880, #1557, #18690, #20093 ) ) ;
#11233=AXIS2_PLACEMENT_3D ( 'NONE', #6976, #29096, #12198 ) ;
#11235=DIRECTION ( 'NONE',  ( 0.000000000000000000, 0.000000000000000000, 1.000000000000000000 ) ) ;
#11237=VERTEX_POINT ( 'NONE', #6210 ) ;
#11238=AXIS2_PLACEMENT_3D ( 'NONE', #20564, #26019, #26216 ) ;
#11239=CIRCLE ( 'NONE', #21441, 2.000000000000001776 ) ;
#11241=FACE_BOUND ( 'NONE', #4677, .T. ) ;
#11242=ORIENTED_EDGE ( 'NONE', *, *, #415, .F. ) ;
#11243=ORIENTED_EDGE ( 'NONE', *, *, #16368, .F. ) ;
#11244=CYLINDRICAL_SURFACE ( 'NONE', #3438, 2.000000000000001776 ) ;
#11245=EDGE_LOOP ( 'NONE', ( #15225, #27223, #5867, #30666 ) ) ;
#11246=AXIS2_PLACEMENT_3D ( 'NONE', #18650, #32895, #23913 ) ;
#11248=DIRECTION ( 'NONE',  ( -1.000000000000000000, 0.000000000000000000, 0.000000000000000000 ) ) ;
#11250=CARTESIAN_POINT ( 'NONE',  ( -55.00000337463110611, -43.30127018922202353, 12.50000000000000000 ) ) ;
#11253=EDGE_LOOP ( 'NONE', ( #24364, #12459, #4499, #3912 ) ) ;
#11255=CIRCLE ( 'NONE', #8841, 2.000000000000001776 ) ;
#11256=ORIENTED_EDGE ( 'NONE', *, *, #19467, .T. ) ;
#11259=AXIS2_PLACEMENT_3D ( 'NONE', #28154, #16529, #8289 ) ;
#11260=ORIENTED_EDGE ( 'NONE', *, *, #16531, .T. ) ;
#11261=DIRECTION ( 'NONE',  ( 1.000000000000000000, 0.000000000000000000, 0.000000000000000000 ) ) ;
#11262=FACE_OUTER_BOUND ( 'NONE', #10194, .T. ) ;
#11263=EDGE_CURVE ( 'NONE', #18862, #5705, #12443, .T. ) ;
#11264=CARTESIAN_POINT ( 'NONE',  ( -70.00000337463099243, -2.428612866367529932E-14, -9.999999999999998224 ) ) ;
#11265=DIRECTION ( 'NONE',  ( 1.000000000000000000, 0.000000000000000000, 0.000000000000000000 ) ) ;
#11266=DIRECTION ( 'NONE',  ( 0.000000000000000000, 0.000000000000000000, 1.000000000000000000 ) ) ;
#11267=ORIENTED_EDGE ( 'NONE', *, *, #22872, .T. ) ;
#11268=DIRECTION ( 'NONE',  ( 0.000000000000000000, 0.000000000000000000, 1.000000000000000000 ) ) ;
#11270=DIRECTION ( 'NONE',  ( 1.000000000000000000, 0.000000000000000000, 0.000000000000000000 ) ) ;
#11271=CARTESIAN_POINT ( 'NONE',  ( 68.00000000000000000, 0.000000000000000000, 12.49999999999999822 ) ) ;
#11272=VERTEX_POINT ( 'NONE', #12579 ) ;
#11274=EDGE_CURVE ( 'NONE', #31389, #3917, #15461, .T. ) ;
#11275=DIRECTION ( 'NONE',  ( 1.000000000000000000, 0.000000000000000000, 0.000000000000000000 ) ) ;
#11276=CIRCLE ( 'NONE', #34657, 2.000000000000001776 ) ;
#11278=ORIENTED_EDGE ( 'NONE', *, *, #13653, .F. ) ;
#11279=CARTESIAN_POINT ( 'NONE',  ( 62.99999662536839651, -60.62177826491080168, -9.999999999999998224 ) ) ;
#11280=AXIS2_PLACEMENT_3D ( 'NONE', #32631, #13147, #27016 ) ;
#11281=FACE_OUTER_BOUND ( 'NONE', #12709, .T. ) ;
#11282=LINE ( 'NONE', #20274, #25850 ) ;
#11284=ORIENTED_EDGE ( 'NONE', *, *, #27545, .T. ) ;
#11285=ORIENTED_EDGE ( 'NONE', *, *, #8533, .F. ) ;
#11286=AXIS2_PLACEMENT_3D ( 'NONE', #34819, #14945, #682 ) ;
#11287=EDGE_CURVE ( 'NONE', #18742, #18793, #26832, .T. ) ;
#11290=CARTESIAN_POINT ( 'NONE',  ( 62.97617850287784336, 4.279621169095339184, -4.999999999999997335 ) ) ;
#11291=EDGE_CURVE ( 'NONE', #9788, #23537, #25058, .T. ) ;
#11292=ORIENTED_EDGE ( 'NONE', *, *, #13286, .T. ) ;
#11293=EDGE_CURVE ( 'NONE', #28140, #1125, #1894, .T. ) ;
#11295=ORIENTED_EDGE ( 'NONE', *, *, #34804, .T. ) ;
#11297=ORIENTED_EDGE ( 'NONE', *, *, #14236, .T. ) ;
#11298=CIRCLE ( 'NONE', #22679, 2.000000000000001776 ) ;
#11299=DIRECTION ( 'NONE',  ( 0.000000000000000000, 0.000000000000000000, 1.000000000000000000 ) ) ;
#11300=DIRECTION ( 'NONE',  ( 1.000000000000000000, 0.000000000000000000, 0.000000000000000000 ) ) ;
#11301=CARTESIAN_POINT ( 'NONE',  ( -65.00000337463102085, 43.30127018922198801, -9.999999999999998224 ) ) ;
#11302=ORIENTED_EDGE ( 'NONE', *, *, #20595, .T. ) ;
#11303=ORIENTED_EDGE ( 'NONE', *, *, #16749, .F. ) ;
#11304=CARTESIAN_POINT ( 'NONE',  ( -25.00000337463120914, 77.94228634059957983, 17.49999999999999645 ) ) ;
#11305=CARTESIAN_POINT ( 'NONE',  ( -12.00000337463128908, 69.28203230275516944, 17.49999999999999645 ) ) ;
#11306=DIRECTION ( 'NONE',  ( 0.000000000000000000, 0.000000000000000000, 1.000000000000000000 ) ) ;
#11308=ORIENTED_EDGE ( 'NONE', *, *, #6007, .F. ) ;
#11309=DIRECTION ( 'NONE',  ( 0.000000000000000000, 0.000000000000000000, 1.000000000000000000 ) ) ;
#11310=CIRCLE ( 'NONE', #23300, 3.000000000000002665 ) ;
#11311=FACE_BOUND ( 'NONE', #9873, .T. ) ;
#11312=VECTOR ( 'NONE', #23700, 1000.000000000000000 ) ;
#11313=CARTESIAN_POINT ( 'NONE',  ( -67.00000337463106348, -60.62177826491083010, 12.50000000000000000 ) ) ;
#11315=DIRECTION ( 'NONE',  ( 0.000000000000000000, 0.000000000000000000, -1.000000000000000000 ) ) ;
#11316=EDGE_CURVE ( 'NONE', #10338, #4318, #34077, .T. ) ;
#11317=PLANE ( 'NONE',  #23085 ) ;
#11319=AXIS2_PLACEMENT_3D ( 'NONE', #12610, #21622, #24064 ) ;
#11320=DIRECTION ( 'NONE',  ( -1.000000000000000000, 0.000000000000000000, 0.000000000000000000 ) ) ;
#11321=VERTEX_POINT ( 'NONE', #6763 ) ;
#11325=ORIENTED_EDGE ( 'NONE', *, *, #11619, .T. ) ;
#11326=ORIENTED_EDGE ( 'NONE', *, *, #17334, .T. ) ;
#11327=CIRCLE ( 'NONE', #35882, 2.000000000000001776 ) ;
#11328=EDGE_LOOP ( 'NONE', ( #728, #5886 ) ) ;
#11329=DIRECTION ( 'NONE',  ( 0.000000000000000000, 0.000000000000000000, 1.000000000000000000 ) ) ;
#11330=DIRECTION ( 'NONE',  ( 0.000000000000000000, 0.000000000000000000, 1.000000000000000000 ) ) ;
#11331=PLANE ( 'NONE',  #35815 ) ;
#11332=ORIENTED_EDGE ( 'NONE', *, *, #34984, .T. ) ;
#11333=CARTESIAN_POINT ( 'NONE',  ( -45.00000000000000711, 5.510910596163090344E-15, -10.00000000000000000 ) ) ;
#11334=CIRCLE ( 'NONE', #29877, 2.000000000000001776 ) ;
#11335=ORIENTED_EDGE ( 'NONE', *, *, #10471, .F. ) ;
#11338=ORIENTED_EDGE ( 'NONE', *, *, #31624, .F. ) ;
#11339=DIRECTION ( 'NONE',  ( -1.000000000000000000, 0.000000000000000000, 0.000000000000000000 ) ) ;
#11340=EDGE_LOOP ( 'NONE', ( #16202, #27600, #27231, #32825 ) ) ;
#11341=VERTEX_POINT ( 'NONE', #4722 ) ;
#11342=CARTESIAN_POINT ( 'NONE',  ( -80.00000337463094979, 34.64101615137757051, -5.000000000000000000 ) ) ;
#11343=CARTESIAN_POINT ( 'NONE',  ( -84.88770934388888634, 10.65709906204123492, -5.000000000000000000 ) ) ;
#11344=VERTEX_POINT ( 'NONE', #21596 ) ;
#11346=CARTESIAN_POINT ( 'NONE',  ( -65.00000000000000000, 0.000000000000000000, 17.49999999999999645 ) ) ;
#11350=DIRECTION ( 'NONE',  ( 1.000000000000000000, 0.000000000000000000, 0.000000000000000000 ) ) ;
#11351=DIRECTION ( 'NONE',  ( -1.000000000000000000, 0.000000000000000000, -0.000000000000000000 ) ) ;
#11352=ORIENTED_EDGE ( 'NONE', *, *, #24031, .F. ) ;
#11353=DIRECTION ( 'NONE',  ( 0.000000000000000000, 0.000000000000000000, 1.000000000000000000 ) ) ;
#11355=AXIS2_PLACEMENT_3D ( 'NONE', #14058, #29033, #28854 ) ;
#11356=CARTESIAN_POINT ( 'NONE',  ( 84.99999662536831124, -25.98076211353319565, -9.999999999999998224 ) ) ;
#11357=EDGE_CURVE ( 'NONE', #2055, #35706, #35476, .T. ) ;
#11358=EDGE_CURVE ( 'NONE', #4900, #35883, #17893, .T. ) ;
#11359=CARTESIAN_POINT ( 'NONE',  ( -8.000003374631278419, -69.28203230275519786, -9.999999999999998224 ) ) ;
#11360=ORIENTED_EDGE ( 'NONE', *, *, #29264, .T. ) ;
#11361=AXIS2_PLACEMENT_3D ( 'NONE', #35755, #28045, #19612 ) ;
#11362=ORIENTED_EDGE ( 'NONE', *, *, #24487, .F. ) ;
#11363=EDGE_CURVE ( 'NONE', #14483, #34280, #7108, .T. ) ;
#11364=CIRCLE ( 'NONE', #35926, 2.000000000000001776 ) ;
#11366=DIRECTION ( 'NONE',  ( 1.000000000000000000, 0.000000000000000000, 0.000000000000000000 ) ) ;
#11367=EDGE_CURVE ( 'NONE', #27049, #20566, #28062, .T. ) ;
#11368=EDGE_LOOP ( 'NONE', ( #16712, #352 ) ) ;
#11369=EDGE_LOOP ( 'NONE', ( #29425, #27256, #36711, #12000, #34283 ) ) ;
#11370=DIRECTION ( 'NONE',  ( 0.000000000000000000, 0.000000000000000000, 1.000000000000000000 ) ) ;
#11371=DIRECTION ( 'NONE',  ( 0.000000000000000000, 0.000000000000000000, -1.000000000000000000 ) ) ;
#11372=CARTESIAN_POINT ( 'NONE',  ( -23.00000337463120559, 77.94228634059957983, 17.49999999999999645 ) ) ;
#11373=AXIS2_PLACEMENT_3D ( 'NONE', #11919, #9106, #20532 ) ;
#11374=VERTEX_POINT ( 'NONE', #4336 ) ;
#11375=ORIENTED_EDGE ( 'NONE', *, *, #2801, .T. ) ;
#11377=CARTESIAN_POINT ( 'NONE',  ( -12.00000337463127842, -69.28203230275519786, -9.999999999999998224 ) ) ;
#11378=VERTEX_POINT ( 'NONE', #18771 ) ;
#11380=EDGE_CURVE ( 'NONE', #30265, #3561, #16087, .T. ) ;
#11381=CARTESIAN_POINT ( 'NONE',  ( -82.00000337463096400, -34.64101615137762025, 17.49999999999999645 ) ) ;
#11382=EDGE_LOOP ( 'NONE', ( #16954, #28259, #25314, #19815, #26681, #24608, #22857, #11665, #11829, #24564, #20985, #33398, #33557 ) ) ;
#11383=FACE_BOUND ( 'NONE', #7301, .T. ) ;
#11384=AXIS2_PLACEMENT_3D ( 'NONE', #19167, #11064, #5461 ) ;
#11385=DIRECTION ( 'NONE',  ( 0.000000000000000000, 0.000000000000000000, -1.000000000000000000 ) ) ;
#11386=AXIS2_PLACEMENT_3D ( 'NONE', #29205, #6530, #23222 ) ;
#11388=CIRCLE ( 'NONE', #14981, 2.000000000000001776 ) ;
#11389=VERTEX_POINT ( 'NONE', #24603 ) ;
#11391=DIRECTION ( 'NONE',  ( 0.000000000000000000, 0.000000000000000000, 1.000000000000000000 ) ) ;
#11392=DIRECTION ( 'NONE',  ( -1.000000000000000000, 0.000000000000000000, 0.000000000000000000 ) ) ;
#11393=CARTESIAN_POINT ( 'NONE',  ( 27.78182860042856461, 56.67878100130339902, 12.49999999999999822 ) ) ;
#11395=ORIENTED_EDGE ( 'NONE', *, *, #6674, .F. ) ;
#11396=AXIS2_PLACEMENT_3D ( 'NONE', #32294, #1180, #21043 ) ;
#11397=DIRECTION ( 'NONE',  ( 0.000000000000000000, 0.000000000000000000, 1.000000000000000000 ) ) ;
#11398=DIRECTION ( 'NONE',  ( 0.5000000000000039968, 0.8660254037844363761, 0.000000000000000000 ) ) ;
#11399=FACE_OUTER_BOUND ( 'NONE', #16823, .T. ) ;
#11400=ORIENTED_EDGE ( 'NONE', *, *, #34548, .T. ) ;
#11401=EDGE_LOOP ( 'NONE', ( #25189, #11910, #27171, #11770 ) ) ;
#11403=ORIENTED_EDGE ( 'NONE', *, *, #28846, .F. ) ;
#11404=EDGE_CURVE ( 'NONE', #33595, #35934, #14282, .T. ) ;
#11406=FACE_OUTER_BOUND ( 'NONE', #14447, .T. ) ;
#11408=DIRECTION ( 'NONE',  ( 1.000000000000000000, 0.000000000000000000, 0.000000000000000000 ) ) ;
#11412=DIRECTION ( 'NONE',  ( 0.000000000000000000, 0.000000000000000000, -1.000000000000000000 ) ) ;
#11413=VERTEX_POINT ( 'NONE', #22498 ) ;
#11414=ORIENTED_EDGE ( 'NONE', *, *, #4254, .T. ) ;
#11415=DIRECTION ( 'NONE',  ( 1.000000000000000000, 0.000000000000000000, 0.000000000000000000 ) ) ;
#11416=DIRECTION ( 'NONE',  ( 0.000000000000000000, 0.000000000000000000, 1.000000000000000000 ) ) ;
#11417=LINE ( 'NONE', #26536, #13853 ) ;
#11420=EDGE_CURVE ( 'NONE', #36248, #30244, #11882, .T. ) ;
#11421=DIRECTION ( 'NONE',  ( 0.000000000000000000, 0.000000000000000000, 1.000000000000000000 ) ) ;
#11422=ORIENTED_EDGE ( 'NONE', *, *, #33414, .F. ) ;
#11423=ORIENTED_EDGE ( 'NONE', *, *, #35981, .T. ) ;
#11424=CARTESIAN_POINT ( 'NONE',  ( -15.00000337463125710, -77.94228634059960825, -5.000000000000000000 ) ) ;
#11425=ORIENTED_EDGE ( 'NONE', *, *, #15211, .F. ) ;
#11426=CARTESIAN_POINT ( 'NONE',  ( 86.99999662536831124, -8.660254037844397956, -9.999999999999998224 ) ) ;
#11427=EDGE_CURVE ( 'NONE', #25842, #29105, #17284, .T. ) ;
#11428=CARTESIAN_POINT ( 'NONE',  ( 51.99999662536847467, 51.96152422706637708, -5.000000000000000000 ) ) ;
#11429=LINE ( 'NONE', #23046, #519 ) ;
#11430=EDGE_CURVE ( 'NONE', #16632, #3771, #23869, .T. ) ;
#11431=ORIENTED_EDGE ( 'NONE', *, *, #4806, .F. ) ;
#11433=EDGE_LOOP ( 'NONE', ( #9176, #9575 ) ) ;
#11434=ORIENTED_EDGE ( 'NONE', *, *, #23617, .F. ) ;
#11435=VERTEX_POINT ( 'NONE', #30583 ) ;
#11436=PLANE ( 'NONE',  #29607 ) ;
#11438=CIRCLE ( 'NONE', #18659, 2.000000000000000000 ) ;
#11440=LINE ( 'NONE', #30946, #11513 ) ;
#11443=DIRECTION ( 'NONE',  ( -0.000000000000000000, -0.000000000000000000, 1.000000000000000000 ) ) ;
#11444=DIRECTION ( 'NONE',  ( 0.000000000000000000, 0.000000000000000000, -1.000000000000000000 ) ) ;
#11445=EDGE_CURVE ( 'NONE', #30112, #29105, #12470, .T. ) ;
#11446=CARTESIAN_POINT ( 'NONE',  ( -22.00000337463124112, -69.28203230275522628, 12.50000000000000000 ) ) ;
#11447=ORIENTED_EDGE ( 'NONE', *, *, #25883, .T. ) ;
#11449=DIRECTION ( 'NONE',  ( 0.000000000000000000, 0.000000000000000000, 1.000000000000000000 ) ) ;
#11450=VERTEX_POINT ( 'NONE', #25499 ) ;
#11451=ORIENTED_EDGE ( 'NONE', *, *, #11951, .T. ) ;
#11452=DIRECTION ( 'NONE',  ( 0.000000000000000000, 0.000000000000000000, 1.000000000000000000 ) ) ;
#11457=ORIENTED_EDGE ( 'NONE', *, *, #1156, .T. ) ;
#11458=DIRECTION ( 'NONE',  ( 1.000000000000000000, 0.000000000000000000, 0.000000000000000000 ) ) ;
#11459=DIRECTION ( 'NONE',  ( 1.000000000000000000, 0.000000000000000000, 0.000000000000000000 ) ) ;
#11464=AXIS2_PLACEMENT_3D ( 'NONE', #21577, #13685, #36571 ) ;
#11465=DIRECTION ( 'NONE',  ( -1.000000000000000000, 0.000000000000000000, 0.000000000000000000 ) ) ;
#11466=ORIENTED_EDGE ( 'NONE', *, *, #13781, .T. ) ;
#11468=EDGE_CURVE ( 'NONE', #18680, #22239, #13497, .T. ) ;
#11469=DIRECTION ( 'NONE',  ( 0.000000000000000000, 0.000000000000000000, 1.000000000000000000 ) ) ;
#11473=EDGE_CURVE ( 'NONE', #20787, #32385, #5272, .T. ) ;
#11475=EDGE_CURVE ( 'NONE', #21946, #4196, #37041, .T. ) ;
#11476=CARTESIAN_POINT ( 'NONE',  ( 54.99999662536844625, -60.62177826491080168, -9.999999999999998224 ) ) ;
#11477=CARTESIAN_POINT ( 'NONE',  ( -2.000003374631289521, -69.28203230275519786, 12.50000000000000000 ) ) ;
#11478=ORIENTED_EDGE ( 'NONE', *, *, #21431, .T. ) ;
#11479=DIRECTION ( 'NONE',  ( 0.000000000000000000, 0.000000000000000000, 1.000000000000000000 ) ) ;
#11480=FACE_BOUND ( 'NONE', #28370, .T. ) ;
#11482=DIRECTION ( 'NONE',  ( 0.000000000000000000, 0.000000000000000000, 1.000000000000000000 ) ) ;
#11483=CARTESIAN_POINT ( 'NONE',  ( 84.99999662536831124, -25.98076211353319565, -5.000000000000000000 ) ) ;
#11484=EDGE_CURVE ( 'NONE', #17803, #5817, #7894, .T. ) ;
#11487=DIRECTION ( 'NONE',  ( 0.000000000000000000, 0.000000000000000000, 1.000000000000000000 ) ) ;
#11488=EDGE_CURVE ( 'NONE', #21436, #5553, #22687, .T. ) ;
#11489=VECTOR ( 'NONE', #1517, 1000.000000000000000 ) ;
#11490=EDGE_CURVE ( 'NONE', #3670, #16108, #10700, .T. ) ;
#11491=DIRECTION ( 'NONE',  ( 0.000000000000000000, 0.000000000000000000, 1.000000000000000000 ) ) ;
#11492=EDGE_LOOP ( 'NONE', ( #9012, #9489 ) ) ;
#11494=DIRECTION ( 'NONE',  ( 1.000000000000000000, 0.000000000000000000, 0.000000000000000000 ) ) ;
#11496=CARTESIAN_POINT ( 'NONE',  ( -68.00000337463102085, -51.96152422706641971, -9.999999999999998224 ) ) ;
#11497=ORIENTED_EDGE ( 'NONE', *, *, #33699, .T. ) ;
#11498=ORIENTED_EDGE ( 'NONE', *, *, #28790, .F. ) ;
#11501=DIRECTION ( 'NONE',  ( 0.000000000000000000, 0.000000000000000000, 1.000000000000000000 ) ) ;
#11502=DIRECTION ( 'NONE',  ( -1.000000000000000000, 0.000000000000000000, 0.000000000000000000 ) ) ;
#11503=EDGE_LOOP ( 'NONE', ( #11045, #8504 ) ) ;
#11504=CYLINDRICAL_SURFACE ( 'NONE', #21495, 2.000000000000001776 ) ;
#11505=ORIENTED_EDGE ( 'NONE', *, *, #8019, .T. ) ;
#11506=CARTESIAN_POINT ( 'NONE',  ( 69.99999662536838230, -34.64101615137759183, 17.49999999999999645 ) ) ;
#11507=ORIENTED_EDGE ( 'NONE', *, *, #12224, .T. ) ;
#11508=DIRECTION ( 'NONE',  ( -1.000000000000000000, 0.000000000000000000, 0.000000000000000000 ) ) ;
#11509=ORIENTED_EDGE ( 'NONE', *, *, #32186, .T. ) ;
#11510=ORIENTED_EDGE ( 'NONE', *, *, #36946, .F. ) ;
#11511=DIRECTION ( 'NONE',  ( -0.000000000000000000, -0.000000000000000000, 1.000000000000000000 ) ) ;
#11512=CARTESIAN_POINT ( 'NONE',  ( 54.99999662536846046, -43.30127018922200222, -5.000000000000000000 ) ) ;
#11513=VECTOR ( 'NONE', #10889, 1000.000000000000000 ) ;
#11514=CARTESIAN_POINT ( 'NONE',  ( -48.00000337463109190, 51.96152422706637708, 17.49999999999999645 ) ) ;
#11516=DIRECTION ( 'NONE',  ( 0.000000000000000000, 0.000000000000000000, 1.000000000000000000 ) ) ;
#11519=EDGE_LOOP ( 'NONE', ( #21486, #32285 ) ) ;
#11520=CARTESIAN_POINT ( 'NONE',  ( 74.99999662536836809, 25.98076211353319565, -5.000000000000000000 ) ) ;
#11521=CYLINDRICAL_SURFACE ( 'NONE', #19780, 3.499999999999996003 ) ;
#11523=CARTESIAN_POINT ( 'NONE',  ( -34.00000000000027711, -58.88972745734168512, 12.49999999999999822 ) ) ;
#11524=CARTESIAN_POINT ( 'NONE',  ( 79.99999662536833966, -3.469446951953614189E-15, -9.999999999999998224 ) ) ;
#11525=DIRECTION ( 'NONE',  ( -0.000000000000000000, -0.000000000000000000, 1.000000000000000000 ) ) ;
#11526=CARTESIAN_POINT ( 'NONE',  ( 58.88972745734179171, -34.00000000000007105, -4.999999999999997335 ) ) ;
#11527=AXIS2_PLACEMENT_3D ( 'NONE', #27774, #4919, #36429 ) ;
#11528=EDGE_CURVE ( 'NONE', #12630, #3592, #31298, .T. ) ;
#11529=EDGE_LOOP ( 'NONE', ( #9621, #19724, #7759, #24870 ) ) ;
#11531=CARTESIAN_POINT ( 'NONE',  ( -3.374631327851540519E-06, 86.60254037844397601, -9.999999999999998224 ) ) ;
#11532=EDGE_LOOP ( 'NONE', ( #11944, #3653, #28754, #11904, #13037, #3372 ) ) ;
#11535=AXIS2_PLACEMENT_3D ( 'NONE', #33733, #13846, #25292 ) ;
#11536=LINE ( 'NONE', #25819, #7651 ) ;
#11537=AXIS2_PLACEMENT_3D ( 'NONE', #27463, #4598, #13773 ) ;
#11538=CARTESIAN_POINT ( 'NONE',  ( -32.00000337463118427, 69.28203230275516944, -9.999999999999998224 ) ) ;
#11539=VERTEX_POINT ( 'NONE', #36203 ) ;
#11540=CARTESIAN_POINT ( 'NONE',  ( 6.999996625368676284, -77.94228634059960825, -5.000000000000000000 ) ) ;
#11541=EDGE_LOOP ( 'NONE', ( #21019, #24890, #33226, #21610 ) ) ;
#11543=FACE_OUTER_BOUND ( 'NONE', #11841, .T. ) ;
#11544=ORIENTED_EDGE ( 'NONE', *, *, #17408, .T. ) ;
#11545=DIRECTION ( 'NONE',  ( 0.000000000000000000, 0.000000000000000000, 1.000000000000000000 ) ) ;
#11547=VECTOR ( 'NONE', #30174, 1000.000000000000000 ) ;
#11549=FACE_BOUND ( 'NONE', #17559, .T. ) ;
#11552=CARTESIAN_POINT ( 'NONE',  ( 54.99999662536844625, 43.30127018922198801, -9.999999999999998224 ) ) ;
#11553=EDGE_CURVE ( 'NONE', #8910, #25432, #11429, .T. ) ;
#11554=AXIS2_PLACEMENT_3D ( 'NONE', #25032, #10220, #8131 ) ;
#11556=CARTESIAN_POINT ( 'NONE',  ( 71.99999662536838230, -51.96152422706639840, 12.50000000000000000 ) ) ;
#11557=ORIENTED_EDGE ( 'NONE', *, *, #10835, .F. ) ;
#11558=CARTESIAN_POINT ( 'NONE',  ( -22.00000337463122690, 86.60254037844397601, 17.49999999999999645 ) ) ;
#11559=DIRECTION ( 'NONE',  ( 0.000000000000000000, 0.000000000000000000, 1.000000000000000000 ) ) ;
#11560=CARTESIAN_POINT ( 'NONE',  ( 49.99999662536846756, 69.28203230275516944, 12.50000000000000000 ) ) ;
#11561=VERTEX_POINT ( 'NONE', #22875 ) ;
#11564=ORIENTED_EDGE ( 'NONE', *, *, #5568, .T. ) ;
#11565=CIRCLE ( 'NONE', #10382, 2.000000000000001776 ) ;
#11568=CARTESIAN_POINT ( 'NONE',  ( -10.00000337463128197, 86.60254037844397601, 17.49999999999999645 ) ) ;
#11570=FACE_OUTER_BOUND ( 'NONE', #33701, .T. ) ;
#11572=VERTEX_POINT ( 'NONE', #34865 ) ;
#11573=CIRCLE ( 'NONE', #28952, 2.000000000000001776 ) ;
#11574=ORIENTED_EDGE ( 'NONE', *, *, #19844, .F. ) ;
#11575=CARTESIAN_POINT ( 'NONE',  ( -7.000003374631307729, 77.94228634059957983, -9.999999999999998224 ) ) ;
#11576=VECTOR ( 'NONE', #25382, 1000.000000000000000 ) ;
#11577=EDGE_CURVE ( 'NONE', #28556, #14157, #8898, .T. ) ;
#11578=CARTESIAN_POINT ( 'NONE',  ( 74.99999662536836809, 8.660254037844394404, -9.999999999999998224 ) ) ;
#11579=DIRECTION ( 'NONE',  ( 1.000000000000000000, 0.000000000000000000, 0.000000000000000000 ) ) ;
#11580=VERTEX_POINT ( 'NONE', #8612 ) ;
#11582=AXIS2_PLACEMENT_3D ( 'NONE', #35176, #32908, #34977 ) ;
#11583=DIRECTION ( 'NONE',  ( 1.000000000000000000, 0.000000000000000000, 0.000000000000000000 ) ) ;
#11586=EDGE_CURVE ( 'NONE', #10997, #21808, #27446, .T. ) ;
#11587=CYLINDRICAL_SURFACE ( 'NONE', #21845, 2.000000000000001776 ) ;
#11588=EDGE_LOOP ( 'NONE', ( #14516, #14141 ) ) ;
#11590=AXIS2_PLACEMENT_3D ( 'NONE', #23968, #30314, #15524 ) ;
#11592=EDGE_CURVE ( 'NONE', #27431, #31117, #10112, .T. ) ;
#11593=FACE_OUTER_BOUND ( 'NONE', #5747, .T. ) ;
#11594=ORIENTED_EDGE ( 'NONE', *, *, #30380, .T. ) ;
#11595=ORIENTED_EDGE ( 'NONE', *, *, #26535, .T. ) ;
#11597=AXIS2_PLACEMENT_3D ( 'NONE', #9764, #30386, #24963 ) ;
#11598=ORIENTED_EDGE ( 'NONE', *, *, #489, .F. ) ;
#11599=ORIENTED_EDGE ( 'NONE', *, *, #11222, .T. ) ;
#11600=CARTESIAN_POINT ( 'NONE',  ( 34.99999662536853862, 77.94228634059959404, -9.999999999999998224 ) ) ;
#11601=MECHANICAL_DESIGN_GEOMETRIC_PRESENTATION_REPRESENTATION('',(#20571),#29563);
#11603=CARTESIAN_POINT ( 'NONE',  ( 57.99999662536842493, 51.96152422706639129, -9.999999999999998224 ) ) ;
#11604=CARTESIAN_POINT ( 'NONE',  ( -65.00000337463106348, -60.62177826491083010, -9.999999999999998224 ) ) ;
#11606=ORIENTED_EDGE ( 'NONE', *, *, #21588, .T. ) ;
#11608=ADVANCED_FACE ( 'NONE', ( #28681 ), #3171, .F. ) ;
#11610=FACE_OUTER_BOUND ( 'NONE', #19736, .T. ) ;
#11611=VERTEX_POINT ( 'NONE', #6349 ) ;
#11612=CARTESIAN_POINT ( 'NONE',  ( 29.99999662536857770, -69.28203230275519786, -5.000000000000000000 ) ) ;
#11614=ORIENTED_EDGE ( 'NONE', *, *, #11086, .F. ) ;
#11615=EDGE_CURVE ( 'NONE', #16140, #11035, #31061, .T. ) ;
#11617=EDGE_LOOP ( 'NONE', ( #25794, #23049, #24632, #26068 ) ) ;
#11619=EDGE_CURVE ( 'NONE', #32887, #17624, #26238, .T. ) ;
#11620=DIRECTION ( 'NONE',  ( 0.000000000000000000, 0.000000000000000000, 1.000000000000000000 ) ) ;
#11623=ORIENTED_EDGE ( 'NONE', *, *, #13549, .F. ) ;
#11624=VERTEX_POINT ( 'NONE', #25699 ) ;
#11625=AXIS2_PLACEMENT_3D ( 'NONE', #7287, #24158, #30537 ) ;
#11626=FACE_OUTER_BOUND ( 'NONE', #16115, .T. ) ;
#11627=DIRECTION ( 'NONE',  ( 1.000000000000000000, 0.000000000000000000, 0.000000000000000000 ) ) ;
#11628=AXIS2_PLACEMENT_3D ( 'NONE', #21340, #10106, #9341 ) ;
#11630=AXIS2_PLACEMENT_3D ( 'NONE', #18004, #35455, #26994 ) ;
#11633=ORIENTED_EDGE ( 'NONE', *, *, #20060, .F. ) ;
#11636=ADVANCED_FACE ( 'NONE', ( #8991, #17792, #20419, #14430, #29227, #3557, #11593 ), #35044, .F. ) ;
#11637=VECTOR ( 'NONE', #35452, 1000.000000000000000 ) ;
#11638=LINE ( 'NONE', #397, #17254 ) ;
#11639=VERTEX_POINT ( 'NONE', #6006 ) ;
#11641=VERTEX_POINT ( 'NONE', #32223 ) ;
#11642=LINE ( 'NONE', #2875, #31634 ) ;
#11643=CARTESIAN_POINT ( 'NONE',  ( 64.99999662536841072, -25.98076211353320275, -9.999999999999998224 ) ) ;
#11644=CARTESIAN_POINT ( 'NONE',  ( 68.17080445151383117, -51.15278694518232072, 12.50000000000000000 ) ) ;
#11645=AXIS2_PLACEMENT_3D ( 'NONE', #29054, #11996, #6579 ) ;
#11647=CARTESIAN_POINT ( 'NONE',  ( -17.00000337463125533, -77.94228634059960825, -9.999999999999998224 ) ) ;
#11648=FACE_BOUND ( 'NONE', #10762, .T. ) ;
#11649=CYLINDRICAL_SURFACE ( 'NONE', #16061, 2.000000000000001776 ) ;
#11651=LINE ( 'NONE', #34560, #5136 ) ;
#11652=CARTESIAN_POINT ( 'NONE',  ( 0.000000000000000000, 0.000000000000000000, -5.000000000000000000 ) ) ;
#11656=DIRECTION ( 'NONE',  ( 0.000000000000000000, 0.000000000000000000, 1.000000000000000000 ) ) ;
#11657=EDGE_LOOP ( 'NONE', ( #18495, #16845 ) ) ;
#11660=FACE_BOUND ( 'NONE', #22903, .T. ) ;
#11661=DIRECTION ( 'NONE',  ( 0.000000000000000000, 0.000000000000000000, -1.000000000000000000 ) ) ;
#11662=ORIENTED_EDGE ( 'NONE', *, *, #6901, .F. ) ;
#11663=ADVANCED_FACE ( 'NONE', ( #23241 ), #31831, .F. ) ;
#11664=ORIENTED_EDGE ( 'NONE', *, *, #24969, .F. ) ;
#11665=ORIENTED_EDGE ( 'NONE', *, *, #932, .F. ) ;
#11666=AXIS2_PLACEMENT_3D ( 'NONE', #4813, #30487, #13047 ) ;
#11667=EDGE_CURVE ( 'NONE', #18343, #24428, #13690, .T. ) ;
#11668=FACE_OUTER_BOUND ( 'NONE', #9901, .T. ) ;
#11669=CARTESIAN_POINT ( 'NONE',  ( -90.00000337463090716, -1.040834085586084257E-14, -9.999999999999998224 ) ) ;
#11670=AXIS2_PLACEMENT_3D ( 'NONE', #16817, #5548, #16977 ) ;
#11671=EDGE_CURVE ( 'NONE', #31731, #7037, #15909, .T. ) ;
#11672=CARTESIAN_POINT ( 'NONE',  ( 67.99999662536838230, 34.64101615137758472, -9.999999999999998224 ) ) ;
#11673=ORIENTED_EDGE ( 'NONE', *, *, #31399, .F. ) ;
#11674=EDGE_CURVE ( 'NONE', #27674, #14720, #10114, .T. ) ;
#11675=AXIS2_PLACEMENT_3D ( 'NONE', #25642, #3296, #31247 ) ;
#11677=CARTESIAN_POINT ( 'NONE',  ( 37.99999662536853151, 69.28203230275518365, -9.999999999999998224 ) ) ;
#11678=ORIENTED_EDGE ( 'NONE', *, *, #19482, .F. ) ;
#11680=ORIENTED_EDGE ( 'NONE', *, *, #27848, .T. ) ;
#11681=DIRECTION ( 'NONE',  ( 1.000000000000000000, 0.000000000000000000, 0.000000000000000000 ) ) ;
#11682=AXIS2_PLACEMENT_3D ( 'NONE', #9672, #12652, #9492 ) ;
#11683=EDGE_LOOP ( 'NONE', ( #32747, #32569, #23400, #19443 ) ) ;
#11684=EDGE_CURVE ( 'NONE', #17723, #22036, #25110, .T. ) ;
#11685=CIRCLE ( 'NONE', #14101, 2.000000000000001776 ) ;
#11686=ORIENTED_EDGE ( 'NONE', *, *, #36830, .T. ) ;
#11688=EDGE_CURVE ( 'NONE', #22983, #16313, #18910, .T. ) ;
#11689=FACE_OUTER_BOUND ( 'NONE', #12583, .T. ) ;
#11690=EDGE_CURVE ( 'NONE', #7273, #10178, #10724, .T. ) ;
#11691=DIRECTION ( 'NONE',  ( 1.000000000000000000, 0.000000000000000000, 0.000000000000000000 ) ) ;
#11692=VERTEX_POINT ( 'NONE', #26976 ) ;
#11693=CARTESIAN_POINT ( 'NONE',  ( -13.00000337463126066, 77.94228634059957983, -9.999999999999998224 ) ) ;
#11695=CARTESIAN_POINT ( 'NONE',  ( 26.99999662536859546, -77.94228634059960825, 12.50000000000000000 ) ) ;
#11696=CIRCLE ( 'NONE', #25498, 2.000000000000001776 ) ;
#11698=DIRECTION ( 'NONE',  ( 0.4999999999999919509, -0.8660254037844433705, 0.000000000000000000 ) ) ;
#11701=CARTESIAN_POINT ( 'NONE',  ( 3.108933952041194271, 78.59334852315024023, -5.000000000000000000 ) ) ;
#11702=AXIS2_PLACEMENT_3D ( 'NONE', #5134, #28359, #5880 ) ;
#11703=CARTESIAN_POINT ( 'NONE',  ( -60.00000337463104216, 51.96152422706639129, -9.999999999999998224 ) ) ;
#11704=DIRECTION ( 'NONE',  ( -0.4999999999999968359, 0.8660254037844404840, 0.000000000000000000 ) ) ;
#11706=VECTOR ( 'NONE', #36061, 1000.000000000000000 ) ;
#11707=CIRCLE ( 'NONE', #4558, 2.000000000000000000 ) ;
#11708=FACE_OUTER_BOUND ( 'NONE', #28053, .T. ) ;
#11709=AXIS2_PLACEMENT_3D ( 'NONE', #6484, #20356, #3285 ) ;
#11710=EDGE_CURVE ( 'NONE', #35393, #4661, #19115, .T. ) ;
#11712=ORIENTED_EDGE ( 'NONE', *, *, #1865, .F. ) ;
#11715=CARTESIAN_POINT ( 'NONE',  ( -83.45172111230354517, 31.46585318596159553, -49.86348611802629449 ) ) ;
#11717=ORIENTED_EDGE ( 'NONE', *, *, #29987, .F. ) ;
#11718=VERTEX_POINT ( 'NONE', #27342 ) ;
#11719=DIRECTION ( 'NONE',  ( -1.000000000000000000, 0.000000000000000000, 0.000000000000000000 ) ) ;
#11721=EDGE_CURVE ( 'NONE', #12419, #13800, #35254, .T. ) ;
#11722=CARTESIAN_POINT ( 'NONE',  ( 4.279621169095998212, -62.97617850287780072, -4.999999999999997335 ) ) ;
#11724=AXIS2_PLACEMENT_3D ( 'NONE', #18833, #10020, #7573 ) ;
#11725=DIRECTION ( 'NONE',  ( 0.000000000000000000, 0.000000000000000000, 1.000000000000000000 ) ) ;
#11726=ORIENTED_EDGE ( 'NONE', *, *, #21070, .F. ) ;
#11727=VECTOR ( 'NONE', #22331, 1000.000000000000000 ) ;
#11728=DIRECTION ( 'NONE',  ( 0.000000000000000000, 0.000000000000000000, 1.000000000000000000 ) ) ;
#11730=FACE_BOUND ( 'NONE', #13483, .T. ) ;
#11731=EDGE_CURVE ( 'NONE', #15417, #32452, #11310, .T. ) ;
#11732=AXIS2_PLACEMENT_3D ( 'NONE', #35467, #32828, #4509 ) ;
#11733=AXIS2_PLACEMENT_3D ( 'NONE', #26713, #12457, #23926 ) ;
#11736=EDGE_CURVE ( 'NONE', #8155, #23009, #27503, .T. ) ;
#11737=EDGE_CURVE ( 'NONE', #8275, #16746, #6544, .T. ) ;
#11738=LINE ( 'NONE', #25654, #5917 ) ;
#11739=LINE ( 'NONE', #9507, #17061 ) ;
#11742=CARTESIAN_POINT ( 'NONE',  ( -12.00000337463125000, -86.60254037844400443, 12.50000000000000000 ) ) ;
#11743=FACE_OUTER_BOUND ( 'NONE', #18573, .T. ) ;
#11744=CARTESIAN_POINT ( 'NONE',  ( -12.00000337463128197, 86.60254037844397601, -9.999999999999998224 ) ) ;
#11745=EDGE_LOOP ( 'NONE', ( #15513, #5385, #5061 ) ) ;
#11746=CARTESIAN_POINT ( 'NONE',  ( 27.99999662536857414, -69.28203230275519786, -9.999999999999998224 ) ) ;
#11747=DIRECTION ( 'NONE',  ( 0.000000000000000000, 0.000000000000000000, 1.000000000000000000 ) ) ;
#11748=CYLINDRICAL_SURFACE ( 'NONE', #26120, 2.000000000000001776 ) ;
#11749=CIRCLE ( 'NONE', #2806, 27.00000000000001421 ) ;
#11751=VERTEX_POINT ( 'NONE', #32587 ) ;
#11755=AXIS2_PLACEMENT_3D ( 'NONE', #9682, #21107, #16053 ) ;
#11756=EDGE_CURVE ( 'NONE', #24284, #698, #31660, .T. ) ;
#11757=CIRCLE ( 'NONE', #31514, 2.000000000000001776 ) ;
#11758=DIRECTION ( 'NONE',  ( 1.000000000000000000, 0.000000000000000000, 0.000000000000000000 ) ) ;
#11760=CARTESIAN_POINT ( 'NONE',  ( -43.00000337463111322, -77.94228634059960825, -5.000000000000000000 ) ) ;
#11762=DIRECTION ( 'NONE',  ( -0.000000000000000000, -0.000000000000000000, -1.000000000000000000 ) ) ;
#11764=EDGE_LOOP ( 'NONE', ( #9499, #9712 ) ) ;
#11765=CIRCLE ( 'NONE', #13604, 2.000000000000001776 ) ;
#11766=ORIENTED_EDGE ( 'NONE', *, *, #7083, .T. ) ;
#11767=LINE ( 'NONE', #14778, #26059 ) ;
#11768=CARTESIAN_POINT ( 'NONE',  ( -55.00000337463107059, 60.62177826491078747, 17.49999999999999645 ) ) ;
#11769=CARTESIAN_POINT ( 'NONE',  ( 56.99999662536844625, -60.62177826491080168, 17.49999999999999645 ) ) ;
#11770=ORIENTED_EDGE ( 'NONE', *, *, #873, .T. ) ;
#11771=AXIS2_PLACEMENT_3D ( 'NONE', #13289, #7125, #29797 ) ;
#11772=FACE_BOUND ( 'NONE', #26523, .T. ) ;
#11773=ORIENTED_EDGE ( 'NONE', *, *, #3439, .T. ) ;
#11774=ORIENTED_EDGE ( 'NONE', *, *, #1532, .T. ) ;
#11776=EDGE_CURVE ( 'NONE', #32947, #14483, #33484, .T. ) ;
#11778=ORIENTED_EDGE ( 'NONE', *, *, #30057, .T. ) ;
#11781=AXIS2_PLACEMENT_3D ( 'NONE', #9179, #29047, #14621 ) ;
#11782=DIRECTION ( 'NONE',  ( 0.000000000000000000, 0.000000000000000000, 1.000000000000000000 ) ) ;
#11787=CIRCLE ( 'NONE', #11215, 2.000000000000001776 ) ;
#11789=AXIS2_PLACEMENT_3D ( 'NONE', #30780, #36619, #36438 ) ;
#11791=ORIENTED_EDGE ( 'NONE', *, *, #11943, .F. ) ;
#11792=FACE_OUTER_BOUND ( 'NONE', #2559, .T. ) ;
#11793=CARTESIAN_POINT ( 'NONE',  ( 9.999996625368655856, -69.28203230275519786, 12.50000000000000000 ) ) ;
#11794=PLANE ( 'NONE',  #28038 ) ;
#11795=AXIS2_PLACEMENT_3D ( 'NONE', #36636, #13928, #25375 ) ;
#11797=CYLINDRICAL_SURFACE ( 'NONE', #7005, 2.000000000000001776 ) ;
#11799=ORIENTED_EDGE ( 'NONE', *, *, #12880, .F. ) ;
#11801=CIRCLE ( 'NONE', #33401, 2.000000000000001776 ) ;
#11803=CIRCLE ( 'NONE', #35182, 2.000000000000001776 ) ;
#11804=DIRECTION ( 'NONE',  ( 0.000000000000000000, 0.000000000000000000, -1.000000000000000000 ) ) ;
#11805=ORIENTED_EDGE ( 'NONE', *, *, #8517, .F. ) ;
#11806=DIRECTION ( 'NONE',  ( 0.000000000000000000, 0.000000000000000000, 1.000000000000000000 ) ) ;
#11807=CYLINDRICAL_SURFACE ( 'NONE', #35767, 2.000000000000000000 ) ;
#11809=CIRCLE ( 'NONE', #31570, 1.999999999999998224 ) ;
#11810=ORIENTED_EDGE ( 'NONE', *, *, #10057, .T. ) ;
#11811=AXIS2_PLACEMENT_3D ( 'NONE', #7202, #33442, #27232 ) ;
#11812=EDGE_CURVE ( 'NONE', #26888, #6282, #27146, .T. ) ;
#11814=CYLINDRICAL_SURFACE ( 'NONE', #19940, 3.000000000000002665 ) ;
#11819=CIRCLE ( 'NONE', #9462, 2.000000000000001776 ) ;
#11820=DIRECTION ( 'NONE',  ( 0.000000000000000000, 0.000000000000000000, 1.000000000000000000 ) ) ;
#11821=DIRECTION ( 'NONE',  ( 0.000000000000000000, 0.000000000000000000, 1.000000000000000000 ) ) ;
#11823=AXIS2_PLACEMENT_3D ( 'NONE', #19188, #27607, #7543 ) ;
#11824=ORIENTED_EDGE ( 'NONE', *, *, #19470, .F. ) ;
#11825=ADVANCED_FACE ( 'NONE', ( #32977 ), #7289, .F. ) ;
#11826=CIRCLE ( 'NONE', #16645, 2.000000000000001776 ) ;
#11827=CIRCLE ( 'NONE', #32803, 3.499999999999996003 ) ;
#11828=CARTESIAN_POINT ( 'NONE',  ( 21.99999662536857770, 86.60254037844397601, -5.000000000000000000 ) ) ;
#11829=ORIENTED_EDGE ( 'NONE', *, *, #2245, .F. ) ;
#11830=DIRECTION ( 'NONE',  ( -0.8660254037844379305, 0.5000000000000011102, 0.000000000000000000 ) ) ;
#11831=DIRECTION ( 'NONE',  ( 1.000000000000000000, 0.000000000000000000, 0.000000000000000000 ) ) ;
#11833=LINE ( 'NONE', #34740, #21454 ) ;
#11836=DIRECTION ( 'NONE',  ( 1.000000000000000000, 0.000000000000000000, 0.000000000000000000 ) ) ;
#11837=EDGE_CURVE ( 'NONE', #3733, #29631, #32883, .T. ) ;
#11838=CYLINDRICAL_SURFACE ( 'NONE', #9443, 2.000000000000001776 ) ;
#11839=DIRECTION ( 'NONE',  ( 0.000000000000000000, 0.000000000000000000, 1.000000000000000000 ) ) ;
#11840=CIRCLE ( 'NONE', #7073, 2.000000000000001776 ) ;
#11841=EDGE_LOOP ( 'NONE', ( #33422, #24014 ) ) ;
#11842=DIRECTION ( 'NONE',  ( -1.000000000000000000, 0.000000000000000000, 0.000000000000000000 ) ) ;
#11843=EDGE_CURVE ( 'NONE', #10369, #17775, #25692, .T. ) ;
#11844=FACE_BOUND ( 'NONE', #31953, .T. ) ;
#11845=CARTESIAN_POINT ( 'NONE',  ( -85.00000337463092137, 25.98076211353317433, -9.999999999999998224 ) ) ;
#11846=DIRECTION ( 'NONE',  ( 0.000000000000000000, 0.000000000000000000, -1.000000000000000000 ) ) ;
#11847=CIRCLE ( 'NONE', #2287, 2.000000000000001776 ) ;
#11848=CARTESIAN_POINT ( 'NONE',  ( 79.99999662536833966, -3.469446951953614189E-15, -9.999999999999998224 ) ) ;
#11849=LINE ( 'NONE', #6776, #14711 ) ;
#11850=CYLINDRICAL_SURFACE ( 'NONE', #26952, 2.000000000000001776 ) ;
#11851=CIRCLE ( 'NONE', #490, 2.000000000000001776 ) ;
#11852=DIRECTION ( 'NONE',  ( 1.000000000000000000, 0.000000000000000000, 0.000000000000000000 ) ) ;
#11853=ORIENTED_EDGE ( 'NONE', *, *, #8723, .T. ) ;
#11854=DIRECTION ( 'NONE',  ( 1.000000000000000000, 0.000000000000000000, 0.000000000000000000 ) ) ;
#11856=CIRCLE ( 'NONE', #17258, 2.000000000000000000 ) ;
#11857=AXIS2_PLACEMENT_3D ( 'NONE', #26249, #561, #20599 ) ;
#11858=CARTESIAN_POINT ( 'NONE',  ( -50.00000337463110611, -69.28203230275519786, 17.49999999999999645 ) ) ;
#11859=CARTESIAN_POINT ( 'NONE',  ( -93.55673653615988883, -16.49657687835776088, -5.000000000000000000 ) ) ;
#11860=AXIS2_PLACEMENT_3D ( 'NONE', #16617, #31047, #35166 ) ;
#11861=EDGE_LOOP ( 'NONE', ( #27965, #30912, #35650 ) ) ;
#11862=EDGE_LOOP ( 'NONE', ( #29221, #22870 ) ) ;
#11863=ORIENTED_EDGE ( 'NONE', *, *, #27065, .F. ) ;
#11864=EDGE_CURVE ( 'NONE', #16326, #10952, #11334, .T. ) ;
#11865=CIRCLE ( 'NONE', #32839, 2.000000000000001776 ) ;
#11867=CARTESIAN_POINT ( 'NONE',  ( 89.99999662536828282, 0.000000000000000000, -9.999999999999998224 ) ) ;
#11868=CARTESIAN_POINT ( 'NONE',  ( 64.99999662536841072, 25.98076211353318854, -9.999999999999998224 ) ) ;
#11869=VERTEX_POINT ( 'NONE', #16842 ) ;
#11870=AXIS2_PLACEMENT_3D ( 'NONE', #32619, #6942, #4147 ) ;
#11871=FACE_OUTER_BOUND ( 'NONE', #31738, .T. ) ;
#11872=EDGE_LOOP ( 'NONE', ( #30373, #7204, #15152 ) ) ;
#11875=CARTESIAN_POINT ( 'NONE',  ( -38.00000337463113453, 69.28203230275516944, 12.50000000000000000 ) ) ;
#11876=AXIS2_PLACEMENT_3D ( 'NONE', #25284, #11011, #22452 ) ;
#11877=ORIENTED_EDGE ( 'NONE', *, *, #25560, .F. ) ;
#11878=ORIENTED_EDGE ( 'NONE', *, *, #6677, .T. ) ;
#11879=EDGE_CURVE ( 'NONE', #35442, #2346, #9518, .T. ) ;
#11880=DIRECTION ( 'NONE',  ( 1.000000000000000000, 0.000000000000000000, 0.000000000000000000 ) ) ;
#11882=CIRCLE ( 'NONE', #28644, 2.000000000000001776 ) ;
#11884=EDGE_LOOP ( 'NONE', ( #20139, #26600, #8010, #11909 ) ) ;
#11886=EDGE_CURVE ( 'NONE', #6247, #24313, #13131, .T. ) ;
#11888=DIRECTION ( 'NONE',  ( -0.8660254037844379305, 0.5000000000000011102, 0.000000000000000000 ) ) ;
#11889=ORIENTED_EDGE ( 'NONE', *, *, #18079, .T. ) ;
#11890=CARTESIAN_POINT ( 'NONE',  ( 17.99999662536858835, 69.28203230275516944, -9.999999999999998224 ) ) ;
#11891=DIRECTION ( 'NONE',  ( -1.000000000000000000, 0.000000000000000000, 0.000000000000000000 ) ) ;
#11892=AXIS2_PLACEMENT_3D ( 'NONE', #7193, #18632, #23888 ) ;
#11893=ADVANCED_FACE ( 'NONE', ( #19837 ), #30885, .F. ) ;
#11894=EDGE_LOOP ( 'NONE', ( #27035, #1366, #11606, #15672 ) ) ;
#11895=DIRECTION ( 'NONE',  ( 1.000000000000000000, 0.000000000000000000, 0.000000000000000000 ) ) ;
#11896=DIRECTION ( 'NONE',  ( 1.000000000000000000, 0.000000000000000000, 0.000000000000000000 ) ) ;
#11897=FACE_OUTER_BOUND ( 'NONE', #23466, .T. ) ;
#11898=AXIS2_PLACEMENT_3D ( 'NONE', #14235, #17037, #2609 ) ;
#11901=CIRCLE ( 'NONE', #31676, 2.000000000000000000 ) ;
#11902=CARTESIAN_POINT ( 'NONE',  ( -92.00000337463090716, -1.016341149603137227E-14, -9.999999999999998224 ) ) ;
#11903=FACE_OUTER_BOUND ( 'NONE', #36632, .T. ) ;
#11904=ORIENTED_EDGE ( 'NONE', *, *, #26839, .F. ) ;
#11905=CARTESIAN_POINT ( 'NONE',  ( -52.00000337463109190, 69.28203230275518365, 12.50000000000000000 ) ) ;
#11907=DIRECTION ( 'NONE',  ( 0.000000000000000000, 0.000000000000000000, -1.000000000000000000 ) ) ;
#11909=ORIENTED_EDGE ( 'NONE', *, *, #20216, .F. ) ;
#11910=ORIENTED_EDGE ( 'NONE', *, *, #35205, .F. ) ;
#11914=CARTESIAN_POINT ( 'NONE',  ( -40.00000337463113453, 69.28203230275516944, -9.999999999999998224 ) ) ;
#11916=CARTESIAN_POINT ( 'NONE',  ( -58.88972745734203329, -33.99999999999965894, -4.999999999999997335 ) ) ;
#11917=ORIENTED_EDGE ( 'NONE', *, *, #21914, .T. ) ;
#11918=VECTOR ( 'NONE', #4414, 1000.000000000000000 ) ;
#11919=CARTESIAN_POINT ( 'NONE',  ( -35.00000337463117717, -77.94228634059963667, -9.999999999999998224 ) ) ;
#11920=ORIENTED_EDGE ( 'NONE', *, *, #29566, .F. ) ;
#11921=FACE_BOUND ( 'NONE', #18344, .T. ) ;
#11922=VECTOR ( 'NONE', #23546, 1000.000000000000000 ) ;
#11923=VECTOR ( 'NONE', #3896, 1000.000000000000000 ) ;
#11924=ADVANCED_FACE ( 'NONE', ( #36894 ), #16114, .T. ) ;
#11925=DIRECTION ( 'NONE',  ( 1.000000000000000000, 0.000000000000000000, 0.000000000000000000 ) ) ;
#11926=FACE_OUTER_BOUND ( 'NONE', #36614, .T. ) ;
#11927=AXIS2_PLACEMENT_3D ( 'NONE', #15269, #17713, #12243 ) ;
#11928=ADVANCED_FACE ( 'NONE', ( #30704 ), #22105, .T. ) ;
#11930=DIRECTION ( 'NONE',  ( 0.000000000000000000, 0.000000000000000000, 1.000000000000000000 ) ) ;
#11933=DIRECTION ( 'NONE',  ( 1.000000000000000000, 0.000000000000000000, 0.000000000000000000 ) ) ;
#11936=CARTESIAN_POINT ( 'NONE',  ( -33.00000337463117006, -77.94228634059963667, 17.49999999999999645 ) ) ;
#11938=DIRECTION ( 'NONE',  ( 0.000000000000000000, 0.000000000000000000, 1.000000000000000000 ) ) ;
#11939=ADVANCED_FACE ( 'NONE', ( #22277 ), #22653, .F. ) ;
#11941=DIRECTION ( 'NONE',  ( 0.000000000000000000, 0.000000000000000000, -1.000000000000000000 ) ) ;
#11942=CARTESIAN_POINT ( 'NONE',  ( -20.00000337463122690, 86.60254037844397601, 17.49999999999999645 ) ) ;
#11943=EDGE_CURVE ( 'NONE', #182, #2651, #26295, .T. ) ;
#11944=ORIENTED_EDGE ( 'NONE', *, *, #22881, .F. ) ;
#11945=ORIENTED_EDGE ( 'NONE', *, *, #34418, .T. ) ;
#11946=ORIENTED_EDGE ( 'NONE', *, *, #23576, .F. ) ;
#11948=EDGE_CURVE ( 'NONE', #23292, #21544, #36710, .T. ) ;
#11950=CARTESIAN_POINT ( 'NONE',  ( 61.06482292022111125, -72.77422209630303485, 12.49999999999999822 ) ) ;
#11951=EDGE_CURVE ( 'NONE', #731, #1473, #10140, .T. ) ;
#11952=EDGE_CURVE ( 'NONE', #27432, #29824, #22450, .T. ) ;
#11954=CARTESIAN_POINT ( 'NONE',  ( -47.00000337463111322, 77.94228634059959404, 12.50000000000000000 ) ) ;
#11957=DIRECTION ( 'NONE',  ( 1.000000000000000000, 0.000000000000000000, 0.000000000000000000 ) ) ;
#11958=ORIENTED_EDGE ( 'NONE', *, *, #16444, .T. ) ;
#11959=ORIENTED_EDGE ( 'NONE', *, *, #6342, .F. ) ;
#11960=CARTESIAN_POINT ( 'NONE',  ( -25.00000337463121980, -77.94228634059963667, -9.999999999999998224 ) ) ;
#11962=CYLINDRICAL_SURFACE ( 'NONE', #790, 1.999999999999998224 ) ;
#11965=FACE_OUTER_BOUND ( 'NONE', #13897, .T. ) ;
#11966=VERTEX_POINT ( 'NONE', #14005 ) ;
#11967=VERTEX_POINT ( 'NONE', #14394 ) ;
#11968=CARTESIAN_POINT ( 'NONE',  ( -20.00000337463122690, 86.60254037844397601, -9.999999999999998224 ) ) ;
#11969=ORIENTED_EDGE ( 'NONE', *, *, #22037, .T. ) ;
#11973=AXIS2_PLACEMENT_3D ( 'NONE', #27957, #2282, #13717 ) ;
#11975=EDGE_LOOP ( 'NONE', ( #30278, #30445, #637, #1852 ) ) ;
#11978=ORIENTED_EDGE ( 'NONE', *, *, #8345, .T. ) ;
#11979=ORIENTED_EDGE ( 'NONE', *, *, #22255, .F. ) ;
#11982=EDGE_LOOP ( 'NONE', ( #23986, #10385, #32227, #34775 ) ) ;
#11983=DIRECTION ( 'NONE',  ( -1.000000000000000000, 0.000000000000000000, 0.000000000000000000 ) ) ;
#11986=ORIENTED_EDGE ( 'NONE', *, *, #18735, .F. ) ;
#11987=DIRECTION ( 'NONE',  ( 0.000000000000000000, 0.000000000000000000, -1.000000000000000000 ) ) ;
#11988=DIRECTION ( 'NONE',  ( -1.000000000000000000, 0.000000000000000000, 0.000000000000000000 ) ) ;
#11989=EDGE_CURVE ( 'NONE', #9816, #2403, #7727, .T. ) ;
#11990=CARTESIAN_POINT ( 'NONE',  ( 29.99999662536857770, -69.28203230275519786, 17.49999999999999645 ) ) ;
#11991=ORIENTED_EDGE ( 'NONE', *, *, #9396, .T. ) ;
#11992=CYLINDRICAL_SURFACE ( 'NONE', #3483, 33.00000000000001421 ) ;
#11993=LINE ( 'NONE', #23450, #20182 ) ;
#11995=EDGE_LOOP ( 'NONE', ( #6765, #16265, #2087, #6650, #12994, #11774, #33230, #6684, #1699, #31557, #8619, #3995, #7644, #34834, #22086, #14413 ) ) ;
#11996=DIRECTION ( 'NONE',  ( 0.000000000000000000, 0.000000000000000000, 1.000000000000000000 ) ) ;
#11997=DIRECTION ( 'NONE',  ( 0.000000000000000000, 0.000000000000000000, 1.000000000000000000 ) ) ;
#11998=CARTESIAN_POINT ( 'NONE',  ( -59.13646009116099833, 70.47608876694653190, 12.49999999999999822 ) ) ;
#11999=CARTESIAN_POINT ( 'NONE',  ( 11.99999662536862566, 86.60254037844397601, -9.999999999999998224 ) ) ;
#12000=ORIENTED_EDGE ( 'NONE', *, *, #28654, .F. ) ;
#12001=CARTESIAN_POINT ( 'NONE',  ( -2.778182860042079927, 69.13212189986968781, 12.49999999999999645 ) ) ;
#12002=CARTESIAN_POINT ( 'NONE',  ( 17.99999662536861678, -69.28203230275519786, 17.49999999999999645 ) ) ;
#12004=VERTEX_POINT ( 'NONE', #17011 ) ;
#12005=DIRECTION ( 'NONE',  ( 0.000000000000000000, 0.000000000000000000, 1.000000000000000000 ) ) ;
#12006=VERTEX_POINT ( 'NONE', #11556 ) ;
#12008=EDGE_CURVE ( 'NONE', #9986, #18803, #18519, .T. ) ;
#12009=CARTESIAN_POINT ( 'NONE',  ( 93.36492675454790913, 17.14523346298246409, -49.86561046011506448 ) ) ;
#12012=EDGE_LOOP ( 'NONE', ( #2149, #26729 ) ) ;
#12013=ORIENTED_EDGE ( 'NONE', *, *, #10564, .F. ) ;
#12014=DIRECTION ( 'NONE',  ( 0.000000000000000000, 0.000000000000000000, 1.000000000000000000 ) ) ;
#12015=CYLINDRICAL_SURFACE ( 'NONE', #26813, 2.000000000000001776 ) ;
#12016=CYLINDRICAL_SURFACE ( 'NONE', #36471, 2.000000000000001776 ) ;
#12017=ADVANCED_FACE ( 'NONE', ( #31257 ), #34274, .T. ) ;
#12018=ORIENTED_EDGE ( 'NONE', *, *, #7145, .T. ) ;
#12019=CARTESIAN_POINT ( 'NONE',  ( 6.999996625368645198, 77.94228634059957983, -9.999999999999998224 ) ) ;
#12020=CIRCLE ( 'NONE', #13838, 27.00000000000001421 ) ;
#12021=FACE_BOUND ( 'NONE', #9439, .T. ) ;
#12022=DIRECTION ( 'NONE',  ( 1.000000000000000000, 0.000000000000000000, 0.000000000000000000 ) ) ;
#12024=CARTESIAN_POINT ( 'NONE',  ( 24.99999662536857059, 77.94228634059957983, -5.000000000000000000 ) ) ;
#12029=ORIENTED_EDGE ( 'NONE', *, *, #23290, .F. ) ;
#12030=DIRECTION ( 'NONE',  ( 0.000000000000000000, 0.000000000000000000, 1.000000000000000000 ) ) ;
#12031=DIRECTION ( 'NONE',  ( 1.000000000000000000, 0.000000000000000000, 0.000000000000000000 ) ) ;
#12032=DIRECTION ( 'NONE',  ( 0.000000000000000000, 0.000000000000000000, 1.000000000000000000 ) ) ;
#12033=VERTEX_POINT ( 'NONE', #3136 ) ;
#12034=ORIENTED_EDGE ( 'NONE', *, *, #24255, .F. ) ;
#12035=VERTEX_POINT ( 'NONE', #8951 ) ;
#12036=LINE ( 'NONE', #20319, #13321 ) ;
#12037=CARTESIAN_POINT ( 'NONE',  ( -63.00000337463104927, -43.30127018922202353, 12.50000000000000000 ) ) ;
#12039=AXIS2_PLACEMENT_3D ( 'NONE', #6493, #11038, #17929 ) ;
#12040=VERTEX_POINT ( 'NONE', #31798 ) ;
#12041=CARTESIAN_POINT ( 'NONE',  ( 21.99999662536859191, 69.28203230275516944, 12.50000000000000000 ) ) ;
#12042=ORIENTED_EDGE ( 'NONE', *, *, #13792, .T. ) ;
#12043=ADVANCED_FACE ( 'NONE', ( #25660 ), #20201, .T. ) ;
#12044=CARTESIAN_POINT ( 'NONE',  ( -60.00000337463108480, -51.96152422706641971, -9.999999999999998224 ) ) ;
#12045=EDGE_LOOP ( 'NONE', ( #28100, #33624, #25149, #32296 ) ) ;
#12046=DIRECTION ( 'NONE',  ( -1.000000000000000000, 0.000000000000000000, 0.000000000000000000 ) ) ;
#12047=VERTEX_POINT ( 'NONE', #5966 ) ;
#12048=EDGE_CURVE ( 'NONE', #24238, #7448, #4169, .T. ) ;
#12049=ORIENTED_EDGE ( 'NONE', *, *, #1639, .T. ) ;
#12050=DIRECTION ( 'NONE',  ( 0.000000000000000000, 0.000000000000000000, -1.000000000000000000 ) ) ;
#12051=LINE ( 'NONE', #9639, #29778 ) ;
#12052=DIRECTION ( 'NONE',  ( 0.000000000000000000, 0.000000000000000000, 1.000000000000000000 ) ) ;
#12053=EDGE_CURVE ( 'NONE', #7932, #20086, #1785, .T. ) ;
#12054=ORIENTED_EDGE ( 'NONE', *, *, #30685, .F. ) ;
#12056=CARTESIAN_POINT ( 'NONE',  ( 46.99999662536851019, -60.62177826491080168, 17.49999999999999645 ) ) ;
#12057=DIRECTION ( 'NONE',  ( 0.000000000000000000, 0.000000000000000000, 1.000000000000000000 ) ) ;
#12058=EDGE_CURVE ( 'NONE', #7909, #8784, #14563, .T. ) ;
#12059=EDGE_LOOP ( 'NONE', ( #19361, #12888, #15259 ) ) ;
#12060=CARTESIAN_POINT ( 'NONE',  ( -10.00000337463125000, -86.60254037844400443, -5.000000000000000000 ) ) ;
#12061=DIRECTION ( 'NONE',  ( -1.000000000000000000, 0.000000000000000000, -0.000000000000000000 ) ) ;
#12062=VECTOR ( 'NONE', #17696, 1000.000000000000000 ) ;
#12063=ORIENTED_EDGE ( 'NONE', *, *, #33017, .T. ) ;
#12065=DIRECTION ( 'NONE',  ( 0.000000000000000000, 0.000000000000000000, 1.000000000000000000 ) ) ;
#12066=DIRECTION ( 'NONE',  ( 1.000000000000000000, 0.000000000000000000, 0.000000000000000000 ) ) ;
#12067=LINE ( 'NONE', #23528, #21862 ) ;
#12068=DIRECTION ( 'NONE',  ( -0.000000000000000000, -0.000000000000000000, 1.000000000000000000 ) ) ;
#12069=CARTESIAN_POINT ( 'NONE',  ( 15.97563234535730814, -90.60231327712320137, -4.999999999999997335 ) ) ;
#12070=ORIENTED_EDGE ( 'NONE', *, *, #16308, .T. ) ;
#12071=DIRECTION ( 'NONE',  ( 0.000000000000000000, -0.000000000000000000, -1.000000000000000000 ) ) ;
#12073=CARTESIAN_POINT ( 'NONE',  ( 4.279621169095998212, -62.97617850287780072, -49.86561046011506448 ) ) ;
#12074=VERTEX_POINT ( 'NONE', #28982 ) ;
#12075=EDGE_CURVE ( 'NONE', #4901, #33, #20010, .T. ) ;
#12076=ORIENTED_EDGE ( 'NONE', *, *, #16488, .T. ) ;
#12079=CARTESIAN_POINT ( 'NONE',  ( 52.99999662536846046, -43.30127018922200222, 17.49999999999999645 ) ) ;
#12080=CARTESIAN_POINT ( 'NONE',  ( 49.99999662536846756, 69.28203230275516944, -5.000000000000000000 ) ) ;
#12081=EDGE_CURVE ( 'NONE', #29077, #12832, #20923, .T. ) ;
#12083=VECTOR ( 'NONE', #9214, 1000.000000000000000 ) ;
#12084=CARTESIAN_POINT ( 'NONE',  ( 36.97203788309026606, -58.48108235278833433, -49.86561046011506448 ) ) ;
#12085=EDGE_LOOP ( 'NONE', ( #15458, #34363 ) ) ;
#12087=FACE_OUTER_BOUND ( 'NONE', #12499, .T. ) ;
#12088=ORIENTED_EDGE ( 'NONE', *, *, #5610, .T. ) ;
#12089=FACE_BOUND ( 'NONE', #30586, .T. ) ;
#12091=FACE_BOUND ( 'NONE', #32015, .T. ) ;
#12092=ORIENTED_EDGE ( 'NONE', *, *, #23902, .F. ) ;
#12093=CARTESIAN_POINT ( 'NONE',  ( 69.99999662536838230, -34.64101615137759183, 12.50000000000000000 ) ) ;
#12095=DIRECTION ( 'NONE',  ( 0.000000000000000000, 0.000000000000000000, 1.000000000000000000 ) ) ;
#12097=DIRECTION ( 'NONE',  ( 1.000000000000000000, 0.000000000000000000, 0.000000000000000000 ) ) ;
#12098=CARTESIAN_POINT ( 'NONE',  ( 51.99999662536847467, 69.28203230275516944, -9.999999999999998224 ) ) ;
#12099=VERTEX_POINT ( 'NONE', #11936 ) ;
#12100=DIRECTION ( 'NONE',  ( 1.000000000000000000, 0.000000000000000000, 0.000000000000000000 ) ) ;
#12101=CARTESIAN_POINT ( 'NONE',  ( 86.99999662536832545, 8.660254037844394404, -9.999999999999998224 ) ) ;
#12102=DIRECTION ( 'NONE',  ( 0.000000000000000000, 0.000000000000000000, -1.000000000000000000 ) ) ;
#12104=ORIENTED_EDGE ( 'NONE', *, *, #12463, .T. ) ;
#12106=ORIENTED_EDGE ( 'NONE', *, *, #19655, .T. ) ;
#12107=DIRECTION ( 'NONE',  ( -1.000000000000000000, 0.000000000000000000, 0.000000000000000000 ) ) ;
#12108=CARTESIAN_POINT ( 'NONE',  ( 60.93295298011005201, 19.13981058454729123, 12.49999999999999822 ) ) ;
#12109=EDGE_CURVE ( 'NONE', #16919, #29590, #16754, .T. ) ;
#12110=ORIENTED_EDGE ( 'NONE', *, *, #11615, .F. ) ;
#12112=CARTESIAN_POINT ( 'NONE',  ( 29.99999662536856349, 69.28203230275518365, -9.999999999999998224 ) ) ;
#12113=EDGE_CURVE ( 'NONE', #22424, #9206, #6309, .T. ) ;
#12114=DIRECTION ( 'NONE',  ( -1.000000000000000000, 0.000000000000000000, 0.000000000000000000 ) ) ;
#12115=ORIENTED_EDGE ( 'NONE', *, *, #14435, .F. ) ;
#12116=EDGE_CURVE ( 'NONE', #26437, #17529, #3520, .T. ) ;
#12117=VERTEX_POINT ( 'NONE', #15121 ) ;
#12118=VECTOR ( 'NONE', #23831, 1000.000000000000000 ) ;
#12120=CYLINDRICAL_SURFACE ( 'NONE', #5590, 2.000000000000001776 ) ;
#12121=CYLINDRICAL_SURFACE ( 'NONE', #22144, 2.000000000000001776 ) ;
#12122=ADVANCED_FACE ( 'NONE', ( #29934 ), #18512, .F. ) ;
#12123=ORIENTED_EDGE ( 'NONE', *, *, #18122, .T. ) ;
#12124=ADVANCED_FACE ( 'NONE', ( #10068 ), #32741, .F. ) ;
#12125=FACE_BOUND ( 'NONE', #30740, .T. ) ;
#12126=ORIENTED_EDGE ( 'NONE', *, *, #12138, .F. ) ;
#12127=CIRCLE ( 'NONE', #11535, 2.000000000000001776 ) ;
#12129=FACE_OUTER_BOUND ( 'NONE', #5818, .T. ) ;
#12130=ORIENTED_EDGE ( 'NONE', *, *, #33840, .F. ) ;
#12131=EDGE_CURVE ( 'NONE', #5193, #20137, #30505, .T. ) ;
#12132=EDGE_CURVE ( 'NONE', #14960, #4180, #2965, .T. ) ;
#12133=DIRECTION ( 'NONE',  ( 1.000000000000000000, 0.000000000000000000, 0.000000000000000000 ) ) ;
#12134=EDGE_CURVE ( 'NONE', #25177, #5895, #24545, .T. ) ;
#12135=CYLINDRICAL_SURFACE ( 'NONE', #10729, 2.000000000000001776 ) ;
#12136=CARTESIAN_POINT ( 'NONE',  ( -50.00000337463112032, -51.96152422706641971, -9.999999999999998224 ) ) ;
#12137=ORIENTED_EDGE ( 'NONE', *, *, #4776, .T. ) ;
#12138=EDGE_CURVE ( 'NONE', #34610, #25842, #26748, .T. ) ;
#12141=ORIENTED_EDGE ( 'NONE', *, *, #15567, .F. ) ;
#12142=ORIENTED_EDGE ( 'NONE', *, *, #29965, .F. ) ;
#12144=EDGE_LOOP ( 'NONE', ( #4021, #30065, #2578, #2862, #33670 ) ) ;
#12145=CARTESIAN_POINT ( 'NONE',  ( -55.00000337463109901, -60.62177826491083010, 12.50000000000000000 ) ) ;
#12146=CARTESIAN_POINT ( 'NONE',  ( 48.49678893472093932, 67.96280274017779277, -5.000000000000000000 ) ) ;
#12148=DIRECTION ( 'NONE',  ( 0.000000000000000000, 0.000000000000000000, 1.000000000000000000 ) ) ;
#12150=CARTESIAN_POINT ( 'NONE',  ( -33.00000337463117006, -77.94228634059963667, -5.000000000000000000 ) ) ;
#12152=DIRECTION ( 'NONE',  ( 0.000000000000000000, 0.000000000000000000, 1.000000000000000000 ) ) ;
#12153=VECTOR ( 'NONE', #13404, 1000.000000000000000 ) ;
#12154=LINE ( 'NONE', #23618, #21589 ) ;
#12155=CIRCLE ( 'NONE', #21766, 27.00000000000001421 ) ;
#12156=CARTESIAN_POINT ( 'NONE',  ( -47.04203867989546950, 43.19957991610416315, 12.49999999999999822 ) ) ;
#12158=CARTESIAN_POINT ( 'NONE',  ( 51.99999662536848888, -51.96152422706640550, -9.999999999999998224 ) ) ;
#12159=FACE_OUTER_BOUND ( 'NONE', #4821, .T. ) ;
#12160=AXIS2_PLACEMENT_3D ( 'NONE', #19813, #28608, #17532 ) ;
#12161=ORIENTED_EDGE ( 'NONE', *, *, #29511, .F. ) ;
#12163=DIRECTION ( 'NONE',  ( 0.000000000000000000, 0.000000000000000000, 1.000000000000000000 ) ) ;
#12164=DIRECTION ( 'NONE',  ( 0.000000000000000000, 0.000000000000000000, 1.000000000000000000 ) ) ;
#12165=CARTESIAN_POINT ( 'NONE',  ( 14.99999662536859901, 77.94228634059957983, -9.999999999999998224 ) ) ;
#12166=CARTESIAN_POINT ( 'NONE',  ( 79.99999662536832545, -17.32050807568879591, -9.999999999999998224 ) ) ;
#12168=AXIS2_PLACEMENT_3D ( 'NONE', #24626, #1738, #22344 ) ;
#12169=DIRECTION ( 'NONE',  ( 0.000000000000000000, 0.000000000000000000, 1.000000000000000000 ) ) ;
#12170=CARTESIAN_POINT ( 'NONE',  ( 4.279621169095998212, -62.97617850287780072, 12.49999999999999822 ) ) ;
#12172=EDGE_LOOP ( 'NONE', ( #3493, #35782, #32609, #10945 ) ) ;
#12173=CARTESIAN_POINT ( 'NONE',  ( -75.00000337463100664, -43.30127018922202353, -5.000000000000000000 ) ) ;
#12174=ORIENTED_EDGE ( 'NONE', *, *, #8558, .F. ) ;
#12175=DIRECTION ( 'NONE',  ( 1.000000000000000000, 0.000000000000000000, 0.000000000000000000 ) ) ;
#12176=EDGE_CURVE ( 'NONE', #18535, #35393, #5964, .T. ) ;
#12177=DIRECTION ( 'NONE',  ( 0.000000000000000000, 0.000000000000000000, 1.000000000000000000 ) ) ;
#12180=ADVANCED_FACE ( 'NONE', ( #4259 ), #30107, .F. ) ;
#12183=CARTESIAN_POINT ( 'NONE',  ( 57.99999662536842493, -51.96152422706639840, -5.000000000000000000 ) ) ;
#12184=CARTESIAN_POINT ( 'NONE',  ( -52.00000337463110611, -69.28203230275519786, -9.999999999999998224 ) ) ;
#12185=CARTESIAN_POINT ( 'NONE',  ( 39.99999662536853151, 69.28203230275518365, 12.50000000000000000 ) ) ;
#12186=ORIENTED_EDGE ( 'NONE', *, *, #5766, .T. ) ;
#12187=DIRECTION ( 'NONE',  ( 1.000000000000000000, 0.000000000000000000, 0.000000000000000000 ) ) ;
#12188=FACE_BOUND ( 'NONE', #8878, .T. ) ;
#12190=DIRECTION ( 'NONE',  ( -1.000000000000000000, 0.000000000000000000, 0.000000000000000000 ) ) ;
#12191=FACE_OUTER_BOUND ( 'NONE', #16652, .T. ) ;
#12192=EDGE_LOOP ( 'NONE', ( #26699, #18227 ) ) ;
#12193=FACE_OUTER_BOUND ( 'NONE', #7670, .T. ) ;
#12194=VECTOR ( 'NONE', #35384, 1000.000000000000000 ) ;
#12196=CYLINDRICAL_SURFACE ( 'NONE', #16419, 2.000000000000001776 ) ;
#12198=DIRECTION ( 'NONE',  ( -1.000000000000000000, 0.000000000000000000, 0.000000000000000000 ) ) ;
#12199=DIRECTION ( 'NONE',  ( 0.000000000000000000, 0.000000000000000000, -1.000000000000000000 ) ) ;
#12200=DIRECTION ( 'NONE',  ( -0.000000000000000000, -0.000000000000000000, 1.000000000000000000 ) ) ;
#12201=EDGE_CURVE ( 'NONE', #18462, #3561, #22132, .T. ) ;
#12202=AXIS2_PLACEMENT_3D ( 'NONE', #33759, #31471, #16502 ) ;
#12203=ORIENTED_EDGE ( 'NONE', *, *, #21038, .F. ) ;
#12204=ORIENTED_EDGE ( 'NONE', *, *, #22353, .F. ) ;
#12205=ORIENTED_EDGE ( 'NONE', *, *, #22229, .T. ) ;
#12206=CIRCLE ( 'NONE', #12811, 2.000000000000001776 ) ;
#12207=DIRECTION ( 'NONE',  ( 1.000000000000000000, 0.000000000000000000, 0.000000000000000000 ) ) ;
#12209=DIRECTION ( 'NONE',  ( 1.000000000000000000, 0.000000000000000000, 0.000000000000000000 ) ) ;
#12210=ORIENTED_EDGE ( 'NONE', *, *, #4799, .T. ) ;
#12212=EDGE_LOOP ( 'NONE', ( #33674, #26585, #7879, #3058 ) ) ;
#12213=CYLINDRICAL_SURFACE ( 'NONE', #23089, 27.00000000000001421 ) ;
#12214=ORIENTED_EDGE ( 'NONE', *, *, #1396, .F. ) ;
#12215=CARTESIAN_POINT ( 'NONE',  ( -30.00000337463119848, -69.28203230275522628, 17.49999999999999645 ) ) ;
#12216=ORIENTED_EDGE ( 'NONE', *, *, #2525, .F. ) ;
#12217=DIRECTION ( 'NONE',  ( 1.000000000000000000, 0.000000000000000000, 0.000000000000000000 ) ) ;
#12218=VERTEX_POINT ( 'NONE', #27108 ) ;
#12219=EDGE_LOOP ( 'NONE', ( #3465, #17884, #2501, #36816, #27778, #204 ) ) ;
#12220=CIRCLE ( 'NONE', #33836, 33.00000000000001421 ) ;
#12221=DIRECTION ( 'NONE',  ( -1.000000000000000000, 0.000000000000000000, 0.000000000000000000 ) ) ;
#12222=CARTESIAN_POINT ( 'NONE',  ( 42.99999662536850309, 77.94228634059959404, 12.50000000000000000 ) ) ;
#12223=CARTESIAN_POINT ( 'NONE',  ( -53.00000337463106348, 60.62177826491078747, 17.49999999999999645 ) ) ;
#12224=EDGE_CURVE ( 'NONE', #18123, #10426, #8949, .T. ) ;
#12225=VERTEX_POINT ( 'NONE', #6690 ) ;
#12226=VERTEX_POINT ( 'NONE', #35951 ) ;
#12227=CARTESIAN_POINT ( 'NONE',  ( -35.00000337463117717, -77.94228634059963667, -9.999999999999998224 ) ) ;
#12229=CIRCLE ( 'NONE', #27807, 2.000000000000001776 ) ;
#12230=CYLINDRICAL_SURFACE ( 'NONE', #36053, 2.000000000000001776 ) ;
#12231=AXIS2_PLACEMENT_3D ( 'NONE', #27141, #26587, #29772 ) ;
#12232=DIRECTION ( 'NONE',  ( 0.000000000000000000, 0.000000000000000000, -1.000000000000000000 ) ) ;
#12233=AXIS2_PLACEMENT_3D ( 'NONE', #11722, #5746, #110 ) ;
#12236=CARTESIAN_POINT ( 'NONE',  ( 9.999996625368655856, -86.60254037844400443, -9.999999999999998224 ) ) ;
#12238=EDGE_LOOP ( 'NONE', ( #32588, #30639, #32742, #23995 ) ) ;
#12239=DIRECTION ( 'NONE',  ( 1.000000000000000000, 0.000000000000000000, 0.000000000000000000 ) ) ;
#12240=CARTESIAN_POINT ( 'NONE',  ( -18.00000337463124467, 69.28203230275516944, -9.999999999999998224 ) ) ;
#12241=FACE_OUTER_BOUND ( 'NONE', #28200, .T. ) ;
#12242=DIRECTION ( 'NONE',  ( 0.000000000000000000, 0.000000000000000000, 1.000000000000000000 ) ) ;
#12243=DIRECTION ( 'NONE',  ( -1.000000000000000000, 0.000000000000000000, 0.000000000000000000 ) ) ;
#12244=AXIS2_PLACEMENT_3D ( 'NONE', #18001, #23445, #28698 ) ;
#12245=EDGE_CURVE ( 'NONE', #11213, #8789, #14951, .T. ) ;
#12246=CARTESIAN_POINT ( 'NONE',  ( 79.99999662536833966, 17.32050807568879236, -9.999999999999998224 ) ) ;
#12247=ORIENTED_EDGE ( 'NONE', *, *, #4357, .F. ) ;
#12248=DIRECTION ( 'NONE',  ( 0.000000000000000000, 0.000000000000000000, 1.000000000000000000 ) ) ;
#12251=CYLINDRICAL_SURFACE ( 'NONE', #6802, 2.000000000000001776 ) ;
#12252=EDGE_CURVE ( 'NONE', #10165, #7561, #16165, .T. ) ;
#12253=VERTEX_POINT ( 'NONE', #12850 ) ;
#12254=ORIENTED_EDGE ( 'NONE', *, *, #13188, .F. ) ;
#12256=DIRECTION ( 'NONE',  ( 0.000000000000000000, 0.000000000000000000, 1.000000000000000000 ) ) ;
#12259=CARTESIAN_POINT ( 'NONE',  ( 12.99999662536859901, 77.94228634059957983, -9.999999999999998224 ) ) ;
#12260=AXIS2_PLACEMENT_3D ( 'NONE', #5767, #6508, #17208 ) ;
#12261=AXIS2_PLACEMENT_3D ( 'NONE', #4669, #19111, #35350 ) ;
#12262=DIRECTION ( 'NONE',  ( 0.000000000000000000, 0.000000000000000000, -1.000000000000000000 ) ) ;
#12263=EDGE_CURVE ( 'NONE', #22983, #21984, #6571, .T. ) ;
#12265=VERTEX_POINT ( 'NONE', #12670 ) ;
#12266=LINE ( 'NONE', #9677, #4184 ) ;
#12267=ORIENTED_EDGE ( 'NONE', *, *, #9579, .F. ) ;
#12268=FACE_BOUND ( 'NONE', #14098, .T. ) ;
#12269=DIRECTION ( 'NONE',  ( 0.000000000000000000, 0.000000000000000000, 1.000000000000000000 ) ) ;
#12270=AXIS2_PLACEMENT_3D ( 'NONE', #14349, #88, #17158 ) ;
#12271=CARTESIAN_POINT ( 'NONE',  ( -3.000003374631308173, 77.94228634059957983, -9.999999999999998224 ) ) ;
#12274=ORIENTED_EDGE ( 'NONE', *, *, #26122, .T. ) ;
#12275=CARTESIAN_POINT ( 'NONE',  ( -50.00000337463110611, -69.28203230275519786, 12.50000000000000000 ) ) ;
#12276=AXIS2_PLACEMENT_3D ( 'NONE', #22537, #27612, #13347 ) ;
#12278=CIRCLE ( 'NONE', #3310, 1.999999999999998224 ) ;
#12280=CARTESIAN_POINT ( 'NONE',  ( 64.99999662536842493, 43.30127018922200222, -5.000000000000000000 ) ) ;
#12281=AXIS2_PLACEMENT_3D ( 'NONE', #26637, #34903, #9762 ) ;
#12282=CARTESIAN_POINT ( 'NONE',  ( 11.99999662536861855, 69.28203230275516944, 17.49999999999999645 ) ) ;
#12284=ORIENTED_EDGE ( 'NONE', *, *, #1833, .F. ) ;
#12285=DIRECTION ( 'NONE',  ( 1.000000000000000000, 0.000000000000000000, 0.000000000000000000 ) ) ;
#12286=CARTESIAN_POINT ( 'NONE',  ( 69.99999662536838230, -51.96152422706639840, -5.000000000000000000 ) ) ;
#12287=DIRECTION ( 'NONE',  ( 0.000000000000000000, 0.000000000000000000, 1.000000000000000000 ) ) ;
#12288=CIRCLE ( 'NONE', #19495, 2.000000000000001776 ) ;
#12289=EDGE_CURVE ( 'NONE', #12365, #24912, #33514, .T. ) ;
#12291=ORIENTED_EDGE ( 'NONE', *, *, #26211, .F. ) ;
#12292=ORIENTED_EDGE ( 'NONE', *, *, #7798, .F. ) ;
#12294=EDGE_LOOP ( 'NONE', ( #11302, #34900 ) ) ;
#12295=CARTESIAN_POINT ( 'NONE',  ( -60.00000337463104216, 51.96152422706639129, 12.50000000000000000 ) ) ;
#12296=DIRECTION ( 'NONE',  ( 1.000000000000000000, 0.000000000000000000, 0.000000000000000000 ) ) ;
#12298=DIRECTION ( 'NONE',  ( 1.000000000000000000, 0.000000000000000000, 0.000000000000000000 ) ) ;
#12299=CARTESIAN_POINT ( 'NONE',  ( 54.99999662536844625, -60.62177826491080168, -5.000000000000000000 ) ) ;
#12300=DIRECTION ( 'NONE',  ( -1.000000000000000000, 0.000000000000000000, 0.000000000000000000 ) ) ;
#12301=AXIS2_PLACEMENT_3D ( 'NONE', #27028, #30203, #15781 ) ;
#12302=EDGE_CURVE ( 'NONE', #5493, #35478, #13745, .T. ) ;
#12303=CIRCLE ( 'NONE', #35087, 2.000000000000001776 ) ;
#12304=VECTOR ( 'NONE', #2050, 1000.000000000000000 ) ;
#12305=DIRECTION ( 'NONE',  ( 1.000000000000000000, 0.000000000000000000, 0.000000000000000000 ) ) ;
#12308=ORIENTED_EDGE ( 'NONE', *, *, #18350, .F. ) ;
#12309=DIRECTION ( 'NONE',  ( -1.000000000000000000, 0.000000000000000000, 0.000000000000000000 ) ) ;
#12310=CIRCLE ( 'NONE', #24337, 2.000000000000001776 ) ;
#12312=CARTESIAN_POINT ( 'NONE',  ( -50.00000337463109190, 51.96152422706637708, 17.49999999999999645 ) ) ;
#12313=VERTEX_POINT ( 'NONE', #18869 ) ;
#12315=VERTEX_POINT ( 'NONE', #4628 ) ;
#12316=AXIS2_PLACEMENT_3D ( 'NONE', #19083, #10430, #31058 ) ;
#12317=VECTOR ( 'NONE', #22094, 1000.000000000000000 ) ;
#12318=FACE_BOUND ( 'NONE', #9466, .T. ) ;
#12319=ORIENTED_EDGE ( 'NONE', *, *, #13517, .F. ) ;
#12320=ORIENTED_EDGE ( 'NONE', *, *, #26400, .F. ) ;
#12321=CARTESIAN_POINT ( 'NONE',  ( 84.99999662536831124, -8.660254037844397956, -9.999999999999998224 ) ) ;
#12322=ORIENTED_EDGE ( 'NONE', *, *, #12344, .F. ) ;
#12323=CIRCLE ( 'NONE', #23109, 2.000000000000000000 ) ;
#12324=CYLINDRICAL_SURFACE ( 'NONE', #2681, 2.000000000000001776 ) ;
#12325=EDGE_CURVE ( 'NONE', #21059, #20978, #5383, .T. ) ;
#12326=VECTOR ( 'NONE', #29845, 1000.000000000000000 ) ;
#12328=DIRECTION ( 'NONE',  ( 0.000000000000000000, 0.000000000000000000, -1.000000000000000000 ) ) ;
#12329=VERTEX_POINT ( 'NONE', #19250 ) ;
#12330=ORIENTED_EDGE ( 'NONE', *, *, #17378, .T. ) ;
#12331=AXIS2_PLACEMENT_3D ( 'NONE', #10783, #11329, #19943 ) ;
#12332=AXIS2_PLACEMENT_3D ( 'NONE', #19752, #30789, #25202 ) ;
#12333=ORIENTED_EDGE ( 'NONE', *, *, #7980, .T. ) ;
#12334=CIRCLE ( 'NONE', #21949, 27.00000000000001421 ) ;
#12335=ADVANCED_FACE ( 'NONE', ( #22410 ), #7621, .F. ) ;
#12337=ORIENTED_EDGE ( 'NONE', *, *, #4254, .F. ) ;
#12338=AXIS2_PLACEMENT_3D ( 'NONE', #18693, #4263, #15692 ) ;
#12339=VERTEX_POINT ( 'NONE', #22237 ) ;
#12340=CARTESIAN_POINT ( 'NONE',  ( 69.99999662536841072, 51.96152422706640550, -9.999999999999998224 ) ) ;
#12341=EDGE_CURVE ( 'NONE', #23885, #10643, #19143, .T. ) ;
#12342=CYLINDRICAL_SURFACE ( 'NONE', #35, 3.000000000000002665 ) ;
#12343=ORIENTED_EDGE ( 'NONE', *, *, #19145, .T. ) ;
#12344=EDGE_CURVE ( 'NONE', #18489, #3043, #19070, .T. ) ;
#12345=DIRECTION ( 'NONE',  ( 0.000000000000000000, 0.000000000000000000, 1.000000000000000000 ) ) ;
#12348=ORIENTED_EDGE ( 'NONE', *, *, #31420, .F. ) ;
#12349=CARTESIAN_POINT ( 'NONE',  ( -55.00000337463109901, -60.62177826491083010, 12.50000000000000000 ) ) ;
#12350=AXIS2_PLACEMENT_3D ( 'NONE', #9067, #18062, #31914 ) ;
#12353=VERTEX_POINT ( 'NONE', #25414 ) ;
#12354=CARTESIAN_POINT ( 'NONE',  ( 34.99999662536855283, 60.62177826491078747, 12.50000000000000000 ) ) ;
#12355=DIRECTION ( 'NONE',  ( 1.000000000000000000, 0.000000000000000000, 0.000000000000000000 ) ) ;
#12359=EDGE_CURVE ( 'NONE', #8015, #22987, #26324, .T. ) ;
#12360=CIRCLE ( 'NONE', #8188, 2.000000000000000000 ) ;
#12361=DIRECTION ( 'NONE',  ( 0.000000000000000000, 0.000000000000000000, 1.000000000000000000 ) ) ;
#12362=DIRECTION ( 'NONE',  ( -0.000000000000000000, -0.000000000000000000, 1.000000000000000000 ) ) ;
#12364=ORIENTED_EDGE ( 'NONE', *, *, #36802, .T. ) ;
#12365=VERTEX_POINT ( 'NONE', #5176 ) ;
#12366=VECTOR ( 'NONE', #10240, 1000.000000000000000 ) ;
#12369=CIRCLE ( 'NONE', #24396, 1.999999999999998224 ) ;
#12370=ORIENTED_EDGE ( 'NONE', *, *, #30074, .T. ) ;
#12371=DIRECTION ( 'NONE',  ( 0.000000000000000000, -0.000000000000000000, -1.000000000000000000 ) ) ;
#12372=ORIENTED_EDGE ( 'NONE', *, *, #2210, .F. ) ;
#12373=DIRECTION ( 'NONE',  ( 0.000000000000000000, 0.000000000000000000, -1.000000000000000000 ) ) ;
#12374=CIRCLE ( 'NONE', #7616, 2.000000000000001776 ) ;
#12375=DIRECTION ( 'NONE',  ( 0.000000000000000000, 0.000000000000000000, -1.000000000000000000 ) ) ;
#12376=EDGE_CURVE ( 'NONE', #26527, #15313, #33544, .T. ) ;
#12377=DIRECTION ( 'NONE',  ( 0.000000000000000000, 0.000000000000000000, 1.000000000000000000 ) ) ;
#12379=EDGE_CURVE ( 'NONE', #23662, #29469, #13966, .T. ) ;
#12380=ORIENTED_EDGE ( 'NONE', *, *, #4639, .F. ) ;
#12381=VECTOR ( 'NONE', #16379, 1000.000000000000000 ) ;
#12382=CIRCLE ( 'NONE', #8818, 2.000000000000001776 ) ;
#12383=DIRECTION ( 'NONE',  ( 0.000000000000000000, 0.000000000000000000, 1.000000000000000000 ) ) ;
#12385=AXIS2_PLACEMENT_3D ( 'NONE', #11216, #7867, #19304 ) ;
#12386=ORIENTED_EDGE ( 'NONE', *, *, #7220, .T. ) ;
#12387=DIRECTION ( 'NONE',  ( 1.000000000000000000, 0.000000000000000000, 0.000000000000000000 ) ) ;
#12388=DIRECTION ( 'NONE',  ( 1.000000000000000000, 0.000000000000000000, 0.000000000000000000 ) ) ;
#12389=EDGE_CURVE ( 'NONE', #2324, #7804, #35949, .T. ) ;
#12390=DIRECTION ( 'NONE',  ( -0.000000000000000000, -0.000000000000000000, 1.000000000000000000 ) ) ;
#12391=DIRECTION ( 'NONE',  ( 0.000000000000000000, 0.000000000000000000, -1.000000000000000000 ) ) ;
#12392=CARTESIAN_POINT ( 'NONE',  ( -35.00000337463116296, 60.62177826491077326, -9.999999999999998224 ) ) ;
#12393=EDGE_CURVE ( 'NONE', #14572, #20117, #29932, .T. ) ;
#12394=AXIS2_PLACEMENT_3D ( 'NONE', #4973, #10794, #13397 ) ;
#12395=EDGE_LOOP ( 'NONE', ( #27862, #23503 ) ) ;
#12396=DIRECTION ( 'NONE',  ( -0.000000000000000000, -0.000000000000000000, 1.000000000000000000 ) ) ;
#12397=AXIS2_PLACEMENT_3D ( 'NONE', #20223, #15839, #18485 ) ;
#12398=CIRCLE ( 'NONE', #29193, 2.000000000000001776 ) ;
#12399=DIRECTION ( 'NONE',  ( -1.000000000000000000, 0.000000000000000000, 0.000000000000000000 ) ) ;
#12400=ORIENTED_EDGE ( 'NONE', *, *, #21686, .F. ) ;
#12401=CYLINDRICAL_SURFACE ( 'NONE', #19044, 2.000000000000001776 ) ;
#12403=CARTESIAN_POINT ( 'NONE',  ( 46.99999662536851019, 77.94228634059959404, 17.49999999999999645 ) ) ;
#12404=AXIS2_PLACEMENT_3D ( 'NONE', #5726, #33857, #31395 ) ;
#12407=EDGE_CURVE ( 'NONE', #6635, #36626, #17971, .T. ) ;
#12408=VERTEX_POINT ( 'NONE', #33304 ) ;
#12410=VECTOR ( 'NONE', #6243, 1000.000000000000000 ) ;
#12411=ADVANCED_FACE ( 'NONE', ( #5723 ), #23352, .F. ) ;
#12413=DIRECTION ( 'NONE',  ( 0.000000000000000000, 0.000000000000000000, 1.000000000000000000 ) ) ;
#12414=DIRECTION ( 'NONE',  ( 1.000000000000000000, 0.000000000000000000, 0.000000000000000000 ) ) ;
#12415=VERTEX_POINT ( 'NONE', #31392 ) ;
#12416=VERTEX_POINT ( 'NONE', #14159 ) ;
#12417=AXIS2_PLACEMENT_3D ( 'NONE', #23178, #34629, #14176 ) ;
#12418=CIRCLE ( 'NONE', #30392, 33.00000000000001421 ) ;
#12419=VERTEX_POINT ( 'NONE', #3473 ) ;
#12420=AXIS2_PLACEMENT_3D ( 'NONE', #8854, #22756, #20295 ) ;
#12421=DIRECTION ( 'NONE',  ( 0.000000000000000000, 0.000000000000000000, 1.000000000000000000 ) ) ;
#12422=CIRCLE ( 'NONE', #1655, 27.00000000000001421 ) ;
#12423=ORIENTED_EDGE ( 'NONE', *, *, #36629, .F. ) ;
#12424=DIRECTION ( 'NONE',  ( 0.000000000000000000, 0.000000000000000000, 1.000000000000000000 ) ) ;
#12425=ORIENTED_EDGE ( 'NONE', *, *, #71, .F. ) ;
#12426=CARTESIAN_POINT ( 'NONE',  ( 69.99999662536839651, -3.469446951953614189E-15, -9.999999999999998224 ) ) ;
#12427=EDGE_LOOP ( 'NONE', ( #33547, #6482 ) ) ;
#12428=VERTEX_POINT ( 'NONE', #25802 ) ;
#12430=FACE_OUTER_BOUND ( 'NONE', #13272, .T. ) ;
#12431=DIRECTION ( 'NONE',  ( -0.000000000000000000, -0.000000000000000000, -1.000000000000000000 ) ) ;
#12432=VERTEX_POINT ( 'NONE', #37051 ) ;
#12434=CYLINDRICAL_SURFACE ( 'NONE', #28065, 2.000000000000001776 ) ;
#12437=ADVANCED_FACE ( 'NONE', ( #22974 ), #11521, .F. ) ;
#12438=CARTESIAN_POINT ( 'NONE',  ( 72.99999662536836809, 8.660254037844394404, 12.50000000000000000 ) ) ;
#12440=ORIENTED_EDGE ( 'NONE', *, *, #18723, .T. ) ;
#12441=DIRECTION ( 'NONE',  ( 0.000000000000000000, 0.000000000000000000, 1.000000000000000000 ) ) ;
#12442=DIRECTION ( 'NONE',  ( 0.000000000000000000, 0.000000000000000000, 1.000000000000000000 ) ) ;
#12443=CIRCLE ( 'NONE', #33423, 1.999999999999998224 ) ;
#12444=ORIENTED_EDGE ( 'NONE', *, *, #15982, .F. ) ;
#12445=CARTESIAN_POINT ( 'NONE',  ( -60.00000337463104216, 51.96152422706639129, -9.999999999999998224 ) ) ;
#12447=AXIS2_PLACEMENT_3D ( 'NONE', #8497, #776, #12022 ) ;
#12448=DIRECTION ( 'NONE',  ( 0.000000000000000000, 0.000000000000000000, 1.000000000000000000 ) ) ;
#12449=FACE_OUTER_BOUND ( 'NONE', #35860, .T. ) ;
#12450=DIRECTION ( 'NONE',  ( 0.000000000000000000, 0.000000000000000000, -1.000000000000000000 ) ) ;
#12451=AXIS2_PLACEMENT_3D ( 'NONE', #16662, #13841, #28442 ) ;
#12452=CARTESIAN_POINT ( 'NONE',  ( 71.99999662536839651, 34.64101615137758472, -9.999999999999998224 ) ) ;
#12453=AXIS2_PLACEMENT_3D ( 'NONE', #31691, #3192, #17446 ) ;
#12455=VERTEX_POINT ( 'NONE', #34791 ) ;
#12457=DIRECTION ( 'NONE',  ( 0.000000000000000000, 0.000000000000000000, 1.000000000000000000 ) ) ;
#12459=ORIENTED_EDGE ( 'NONE', *, *, #16052, .T. ) ;
#12460=VECTOR ( 'NONE', #21806, 1000.000000000000000 ) ;
#12461=ORIENTED_EDGE ( 'NONE', *, *, #6240, .T. ) ;
#12463=EDGE_CURVE ( 'NONE', #20714, #12474, #32938, .T. ) ;
#12464=DIRECTION ( 'NONE',  ( 1.000000000000000000, 0.000000000000000000, 0.000000000000000000 ) ) ;
#12465=CARTESIAN_POINT ( 'NONE',  ( 18.03952607653389961, -86.20686977408767859, -5.000000000000000000 ) ) ;
#12466=DIRECTION ( 'NONE',  ( 1.000000000000000000, 0.000000000000000000, 0.000000000000000000 ) ) ;
#12467=CIRCLE ( 'NONE', #8892, 2.000000000000001776 ) ;
#12470=CIRCLE ( 'NONE', #19689, 27.00000000000001776 ) ;
#12471=CARTESIAN_POINT ( 'NONE',  ( -35.00000337463117717, -77.94228634059963667, 12.50000000000000000 ) ) ;
#12472=VERTEX_POINT ( 'NONE', #36849 ) ;
#12473=DIRECTION ( 'NONE',  ( 0.000000000000000000, 0.000000000000000000, 1.000000000000000000 ) ) ;
#12474=VERTEX_POINT ( 'NONE', #19803 ) ;
#12475=AXIS2_PLACEMENT_3D ( 'NONE', #16720, #28145, #13158 ) ;
#12476=FACE_BOUND ( 'NONE', #35886, .T. ) ;
#12477=CIRCLE ( 'NONE', #11860, 2.000000000000000000 ) ;
#12479=AXIS2_PLACEMENT_3D ( 'NONE', #16680, #31450, #31271 ) ;
#12480=DIRECTION ( 'NONE',  ( 0.000000000000000000, 0.000000000000000000, 1.000000000000000000 ) ) ;
#12481=DIRECTION ( 'NONE',  ( 1.000000000000000000, 0.000000000000000000, 0.000000000000000000 ) ) ;
#12483=CARTESIAN_POINT ( 'NONE',  ( 56.99999662536844625, 60.62177826491077326, 17.49999999999999645 ) ) ;
#12488=CARTESIAN_POINT ( 'NONE',  ( -15.97563234535668109, 90.60231327712331506, -4.999999999999997335 ) ) ;
#12489=AXIS2_PLACEMENT_3D ( 'NONE', #10565, #33633, #33450 ) ;
#12491=CARTESIAN_POINT ( 'NONE',  ( -55.00000337463107059, 43.30127018922197379, -9.999999999999998224 ) ) ;
#12494=EDGE_CURVE ( 'NONE', #17074, #6836, #7194, .T. ) ;
#12498=EDGE_CURVE ( 'NONE', #9458, #8382, #20353, .T. ) ;
#12499=EDGE_LOOP ( 'NONE', ( #12247, #27128, #1198, #16461 ) ) ;
#12503=CARTESIAN_POINT ( 'NONE',  ( 72.99999662536836809, 43.30127018922198801, -9.999999999999998224 ) ) ;
#12504=DIRECTION ( 'NONE',  ( 0.000000000000000000, 0.000000000000000000, 1.000000000000000000 ) ) ;
#12505=CARTESIAN_POINT ( 'NONE',  ( -16.49657687835744113, 93.55673653615994567, -5.000000000000000000 ) ) ;
#12506=ADVANCED_FACE ( 'NONE', ( #31584 ), #31928, .F. ) ;
#12507=DIRECTION ( 'NONE',  ( 0.000000000000000000, 0.000000000000000000, -1.000000000000000000 ) ) ;
#12510=DIRECTION ( 'NONE',  ( 0.000000000000000000, 0.000000000000000000, 1.000000000000000000 ) ) ;
#12511=ORIENTED_EDGE ( 'NONE', *, *, #28005, .T. ) ;
#12512=VERTEX_POINT ( 'NONE', #25966 ) ;
#12515=CARTESIAN_POINT ( 'NONE',  ( -70.00000337463100664, -17.32050807568882078, 17.49999999999999645 ) ) ;
#12516=EDGE_LOOP ( 'NONE', ( #22063, #17136, #21178, #19865, #23960 ) ) ;
#12517=CIRCLE ( 'NONE', #20986, 2.000000000000001776 ) ;
#12518=DIRECTION ( 'NONE',  ( -0.000000000000000000, -0.000000000000000000, 1.000000000000000000 ) ) ;
#12519=ORIENTED_EDGE ( 'NONE', *, *, #20197, .F. ) ;
#12520=CIRCLE ( 'NONE', #26913, 2.000000000000001776 ) ;
#12522=AXIS2_PLACEMENT_3D ( 'NONE', #35403, #32177, #32546 ) ;
#12523=ORIENTED_EDGE ( 'NONE', *, *, #23362, .F. ) ;
#12524=ORIENTED_EDGE ( 'NONE', *, *, #6887, .T. ) ;
#12526=VECTOR ( 'NONE', #6551, 1000.000000000000000 ) ;
#12527=CARTESIAN_POINT ( 'NONE',  ( 56.99999662536844625, 43.30127018922198801, 17.49999999999999645 ) ) ;
#12528=ORIENTED_EDGE ( 'NONE', *, *, #9882, .F. ) ;
#12531=CARTESIAN_POINT ( 'NONE',  ( -80.00000337463094979, 17.32050807568878525, 12.50000000000000000 ) ) ;
#12532=CARTESIAN_POINT ( 'NONE',  ( 35.19434990244975126, -52.39915983220758022, -4.999999999999997335 ) ) ;
#12535=ORIENTED_EDGE ( 'NONE', *, *, #22497, .F. ) ;
#12536=EDGE_CURVE ( 'NONE', #25059, #29874, #16191, .T. ) ;
#12537=CIRCLE ( 'NONE', #29298, 2.000000000000001776 ) ;
#12538=ORIENTED_EDGE ( 'NONE', *, *, #27063, .T. ) ;
#12539=VERTEX_POINT ( 'NONE', #14528 ) ;
#12540=VECTOR ( 'NONE', #12480, 1000.000000000000000 ) ;
#12541=ADVANCED_FACE ( 'NONE', ( #16971 ), #6093, .T. ) ;
#12543=LINE ( 'NONE', #32799, #33802 ) ;
#12545=EDGE_LOOP ( 'NONE', ( #4605, #7622 ) ) ;
#12546=CYLINDRICAL_SURFACE ( 'NONE', #32832, 2.000000000000001776 ) ;
#12549=CARTESIAN_POINT ( 'NONE',  ( 87.99999662536828282, 2.449293598294703949E-16, -9.999999999999998224 ) ) ;
#12550=ORIENTED_EDGE ( 'NONE', *, *, #21405, .F. ) ;
#12551=DIRECTION ( 'NONE',  ( 0.000000000000000000, 0.000000000000000000, -1.000000000000000000 ) ) ;
#12552=DIRECTION ( 'NONE',  ( 1.000000000000000000, 0.000000000000000000, 0.000000000000000000 ) ) ;
#12555=VERTEX_POINT ( 'NONE', #23157 ) ;
#12556=CYLINDRICAL_SURFACE ( 'NONE', #1090, 2.000000000000001776 ) ;
#12557=AXIS2_PLACEMENT_3D ( 'NONE', #2769, #14202, #11392 ) ;
#12559=ORIENTED_EDGE ( 'NONE', *, *, #26571, .T. ) ;
#12560=ORIENTED_EDGE ( 'NONE', *, *, #5687, .F. ) ;
#12561=EDGE_CURVE ( 'NONE', #23429, #24999, #22806, .T. ) ;
#12562=CARTESIAN_POINT ( 'NONE',  ( -55.00000337463107059, 60.62177826491078747, 12.50000000000000000 ) ) ;
#12563=CARTESIAN_POINT ( 'NONE',  ( -15.97563234535668109, 90.60231327712331506, 12.49999999999999822 ) ) ;
#12564=FACE_OUTER_BOUND ( 'NONE', #13666, .T. ) ;
#12567=EDGE_CURVE ( 'NONE', #17104, #28322, #3272, .T. ) ;
#12570=VERTEX_POINT ( 'NONE', #15460 ) ;
#12572=AXIS2_PLACEMENT_3D ( 'NONE', #9047, #20470, #31892 ) ;
#12575=ORIENTED_EDGE ( 'NONE', *, *, #32520, .T. ) ;
#12576=DIRECTION ( 'NONE',  ( 0.000000000000000000, 0.000000000000000000, 1.000000000000000000 ) ) ;
#12577=DIRECTION ( 'NONE',  ( 0.000000000000000000, 0.000000000000000000, 1.000000000000000000 ) ) ;
#12578=CIRCLE ( 'NONE', #33566, 2.000000000000001776 ) ;
#12579=CARTESIAN_POINT ( 'NONE',  ( -47.00000337463112743, -60.62177826491080168, 12.50000000000000000 ) ) ;
#12580=EDGE_LOOP ( 'NONE', ( #1431, #36659, #10968, #20502 ) ) ;
#12581=ORIENTED_EDGE ( 'NONE', *, *, #6238, .T. ) ;
#12583=EDGE_LOOP ( 'NONE', ( #26130, #23615, #4644, #16869 ) ) ;
#12584=CARTESIAN_POINT ( 'NONE',  ( -55.00000337463110611, -43.30127018922202353, -5.000000000000000000 ) ) ;
#12585=FACE_BOUND ( 'NONE', #17140, .T. ) ;
#12586=AXIS2_PLACEMENT_3D ( 'NONE', #34029, #3243, #9052 ) ;
#12588=DIRECTION ( 'NONE',  ( 0.000000000000000000, 0.000000000000000000, 1.000000000000000000 ) ) ;
#12589=CYLINDRICAL_SURFACE ( 'NONE', #20115, 2.000000000000001776 ) ;
#12591=CARTESIAN_POINT ( 'NONE',  ( -3.374631289687624047E-06, -69.28203230275519786, -9.999999999999998224 ) ) ;
#12592=DIRECTION ( 'NONE',  ( 0.000000000000000000, 0.000000000000000000, 1.000000000000000000 ) ) ;
#12593=AXIS2_PLACEMENT_3D ( 'NONE', #27764, #19888, #25335 ) ;
#12595=VERTEX_POINT ( 'NONE', #26896 ) ;
#12596=CYLINDRICAL_SURFACE ( 'NONE', #19622, 2.000000000000001776 ) ;
#12597=PLANE ( 'NONE',  #8775 ) ;
#12598=DIRECTION ( 'NONE',  ( 0.000000000000000000, 0.000000000000000000, 1.000000000000000000 ) ) ;
#12599=VERTEX_POINT ( 'NONE', #26344 ) ;
#12600=VERTEX_POINT ( 'NONE', #21763 ) ;
#12601=EDGE_CURVE ( 'NONE', #19493, #23515, #5989, .T. ) ;
#12602=FACE_OUTER_BOUND ( 'NONE', #18144, .T. ) ;
#12603=DIRECTION ( 'NONE',  ( 0.000000000000000000, 0.000000000000000000, 1.000000000000000000 ) ) ;
#12607=EDGE_LOOP ( 'NONE', ( #1665, #27230, #2914, #6865, #28013, #11557, #6341, #1751 ) ) ;
#12609=EDGE_CURVE ( 'NONE', #36868, #10255, #26936, .T. ) ;
#12610=CARTESIAN_POINT ( 'NONE',  ( -52.39915983220772233, -35.19434990244957362, -4.999999999999997335 ) ) ;
#12611=ORIENTED_EDGE ( 'NONE', *, *, #35342, .T. ) ;
#12612=VERTEX_POINT ( 'NONE', #29502 ) ;
#12613=EDGE_CURVE ( 'NONE', #17979, #8132, #27588, .T. ) ;
#12614=DIRECTION ( 'NONE',  ( -1.000000000000000000, 1.066533692637591978E-14, 0.000000000000000000 ) ) ;
#12616=EDGE_CURVE ( 'NONE', #25448, #13993, #4020, .T. ) ;
#12617=ORIENTED_EDGE ( 'NONE', *, *, #35879, .T. ) ;
#12618=DIRECTION ( 'NONE',  ( 0.000000000000000000, 0.000000000000000000, 1.000000000000000000 ) ) ;
#12620=CIRCLE ( 'NONE', #17423, 2.000000000000001776 ) ;
#12621=ORIENTED_EDGE ( 'NONE', *, *, #33840, .T. ) ;
#12622=ORIENTED_EDGE ( 'NONE', *, *, #16881, .T. ) ;
#12623=CARTESIAN_POINT ( 'NONE',  ( -47.00000337463111322, -77.94228634059960825, 12.50000000000000000 ) ) ;
#12625=ADVANCED_FACE ( 'NONE', ( #18256 ), #1718, .F. ) ;
#12626=DIRECTION ( 'NONE',  ( -1.000000000000000000, 0.000000000000000000, 0.000000000000000000 ) ) ;
#12629=EDGE_CURVE ( 'NONE', #6799, #17677, #31141, .T. ) ;
#12630=VERTEX_POINT ( 'NONE', #32330 ) ;
#12631=CARTESIAN_POINT ( 'NONE',  ( -68.00000337463099243, -2.428612866367529932E-14, -9.999999999999998224 ) ) ;
#12632=ADVANCED_FACE ( 'NONE', ( #10327 ), #7518, .T. ) ;
#12633=ORIENTED_EDGE ( 'NONE', *, *, #36634, .F. ) ;
#12634=DIRECTION ( 'NONE',  ( 1.000000000000000000, 0.000000000000000000, 0.000000000000000000 ) ) ;
#12635=EDGE_CURVE ( 'NONE', #18828, #32378, #20943, .T. ) ;
#12636=CARTESIAN_POINT ( 'NONE',  ( 62.99999662536841072, -25.98076211353320275, 12.50000000000000000 ) ) ;
#12637=CYLINDRICAL_SURFACE ( 'NONE', #1634, 3.499999999999989342 ) ;
#12638=CARTESIAN_POINT ( 'NONE',  ( -2.269462870248036555E-13, -65.00000000000000000, 12.49999999999999822 ) ) ;
#12639=DIRECTION ( 'NONE',  ( 0.000000000000000000, 0.000000000000000000, 1.000000000000000000 ) ) ;
#12641=EDGE_LOOP ( 'NONE', ( #20873, #444 ) ) ;
#12642=DIRECTION ( 'NONE',  ( -0.000000000000000000, -0.000000000000000000, -1.000000000000000000 ) ) ;
#12643=CIRCLE ( 'NONE', #10273, 2.000000000000001776 ) ;
#12644=CYLINDRICAL_SURFACE ( 'NONE', #8166, 3.499999999999991562 ) ;
#12645=DIRECTION ( 'NONE',  ( -0.000000000000000000, -0.000000000000000000, 1.000000000000000000 ) ) ;
#12646=ORIENTED_EDGE ( 'NONE', *, *, #19549, .F. ) ;
#12649=DIRECTION ( 'NONE',  ( 1.000000000000000000, 0.000000000000000000, 0.000000000000000000 ) ) ;
#12650=CARTESIAN_POINT ( 'NONE',  ( -72.00000337463100664, -17.32050807568882078, -9.999999999999998224 ) ) ;
#12651=CARTESIAN_POINT ( 'NONE',  ( 83.10590767357027175, -8.018049208621958357, 12.50000000000000000 ) ) ;
#12652=DIRECTION ( 'NONE',  ( 0.000000000000000000, -0.000000000000000000, -1.000000000000000000 ) ) ;
#12653=CARTESIAN_POINT ( 'NONE',  ( 59.29837256189581041, 31.02796211690887418, -4.999999999999997335 ) ) ;
#12654=CARTESIAN_POINT ( 'NONE',  ( 61.99999662536842493, -51.96152422706639840, -9.999999999999998224 ) ) ;
#12655=ORIENTED_EDGE ( 'NONE', *, *, #19270, .T. ) ;
#12656=PLANE ( 'NONE',  #10004 ) ;
#12658=FACE_BOUND ( 'NONE', #36987, .T. ) ;
#12659=DIRECTION ( 'NONE',  ( 0.000000000000000000, 0.000000000000000000, -1.000000000000000000 ) ) ;
#12661=VECTOR ( 'NONE', #9464, 1000.000000000000000 ) ;
#12662=DIRECTION ( 'NONE',  ( 1.000000000000000000, 0.000000000000000000, 0.000000000000000000 ) ) ;
#12663=ORIENTED_EDGE ( 'NONE', *, *, #3240, .T. ) ;
#12665=AXIS2_PLACEMENT_3D ( 'NONE', #17622, #29437, #3755 ) ;
#12667=PLANE ( 'NONE',  #32036 ) ;
#12668=EDGE_CURVE ( 'NONE', #19047, #14960, #36036, .T. ) ;
#12669=FACE_BOUND ( 'NONE', #27643, .T. ) ;
#12670=CARTESIAN_POINT ( 'NONE',  ( 66.99999662536841072, -25.98076211353320275, -5.000000000000000000 ) ) ;
#12671=ADVANCED_FACE ( 'NONE', ( #4727 ), #6329, .F. ) ;
#12673=DIRECTION ( 'NONE',  ( 1.000000000000000000, 0.000000000000000000, 0.000000000000000000 ) ) ;
#12676=ORIENTED_EDGE ( 'NONE', *, *, #9193, .F. ) ;
#12677=EDGE_LOOP ( 'NONE', ( #4437, #33561, #193, #32415 ) ) ;
#12678=ORIENTED_EDGE ( 'NONE', *, *, #35531, .F. ) ;
#12679=CARTESIAN_POINT ( 'NONE',  ( -60.00000337463104216, 34.64101615137757051, 12.50000000000000000 ) ) ;
#12680=DIRECTION ( 'NONE',  ( -1.000000000000000000, 0.000000000000000000, 0.000000000000000000 ) ) ;
#12681=DIRECTION ( 'NONE',  ( 0.000000000000000000, 0.000000000000000000, 1.000000000000000000 ) ) ;
#12682=AXIS2_PLACEMENT_3D ( 'NONE', #18207, #27025, #29640 ) ;
#12683=DIRECTION ( 'NONE',  ( 1.000000000000000000, 0.000000000000000000, 0.000000000000000000 ) ) ;
#12684=CARTESIAN_POINT ( 'NONE',  ( -57.00000337463107059, 43.30127018922197379, -9.999999999999998224 ) ) ;
#12686=EDGE_CURVE ( 'NONE', #13489, #22972, #28142, .T. ) ;
#12687=ORIENTED_EDGE ( 'NONE', *, *, #9501, .F. ) ;
#12690=CARTESIAN_POINT ( 'NONE',  ( -22.00000337463124112, 69.28203230275516944, -5.000000000000000000 ) ) ;
#12691=EDGE_LOOP ( 'NONE', ( #5212, #2645 ) ) ;
#12692=DIRECTION ( 'NONE',  ( -1.000000000000000000, 0.000000000000000000, 0.000000000000000000 ) ) ;
#12695=AXIS2_PLACEMENT_3D ( 'NONE', #14296, #23846, #15027 ) ;
#12696=ADVANCED_FACE ( 'NONE', ( #35023 ), #26404, .F. ) ;
#12697=VECTOR ( 'NONE', #13901, 1000.000000000000000 ) ;
#12698=FACE_BOUND ( 'NONE', #11503, .T. ) ;
#12699=VERTEX_POINT ( 'NONE', #32392 ) ;
#12701=CARTESIAN_POINT ( 'NONE',  ( 69.99999662536839651, -17.32050807568879947, -9.999999999999998224 ) ) ;
#12702=ORIENTED_EDGE ( 'NONE', *, *, #20644, .T. ) ;
#12703=DIRECTION ( 'NONE',  ( -0.000000000000000000, -0.000000000000000000, 1.000000000000000000 ) ) ;
#12705=PLANE ( 'NONE',  #35311 ) ;
#12708=ORIENTED_EDGE ( 'NONE', *, *, #25836, .T. ) ;
#12709=EDGE_LOOP ( 'NONE', ( #19141, #841, #2663, #19604 ) ) ;
#12711=ORIENTED_EDGE ( 'NONE', *, *, #3656, .F. ) ;
#12712=CARTESIAN_POINT ( 'NONE',  ( -80.00000337463094979, 17.32050807568878525, -5.000000000000000000 ) ) ;
#12713=CARTESIAN_POINT ( 'NONE',  ( -75.00000337463097821, 25.98076211353318854, 12.50000000000000000 ) ) ;
#12714=ORIENTED_EDGE ( 'NONE', *, *, #36011, .T. ) ;
#12716=CARTESIAN_POINT ( 'NONE',  ( -50.00000337463110611, -69.28203230275519786, -9.999999999999998224 ) ) ;
#12718=DIRECTION ( 'NONE',  ( 1.000000000000000000, 0.000000000000000000, 0.000000000000000000 ) ) ;
#12719=AXIS2_PLACEMENT_3D ( 'NONE', #4145, #12731, #9937 ) ;
#12722=DIRECTION ( 'NONE',  ( 0.8660254037844344888, -0.5000000000000069944, 0.000000000000000000 ) ) ;
#12723=ORIENTED_EDGE ( 'NONE', *, *, #25735, .F. ) ;
#12724=CARTESIAN_POINT ( 'NONE',  ( -63.00000337463104927, -25.98076211353322051, 17.49999999999999645 ) ) ;
#12725=CARTESIAN_POINT ( 'NONE',  ( -70.00000337463102085, -34.64101615137762025, -9.999999999999998224 ) ) ;
#12726=EDGE_CURVE ( 'NONE', #25226, #11378, #10803, .T. ) ;
#12727=VERTEX_POINT ( 'NONE', #20762 ) ;
#12730=AXIS2_PLACEMENT_3D ( 'NONE', #29898, #15657, #23722 ) ;
#12731=DIRECTION ( 'NONE',  ( 0.000000000000000000, 0.000000000000000000, -1.000000000000000000 ) ) ;
#12732=DIRECTION ( 'NONE',  ( 0.000000000000000000, 0.000000000000000000, -1.000000000000000000 ) ) ;
#12733=AXIS2_PLACEMENT_3D ( 'NONE', #19582, #1781, #4403 ) ;
#12734=CYLINDRICAL_SURFACE ( 'NONE', #14965, 2.000000000000001776 ) ;
#12735=EDGE_CURVE ( 'NONE', #625, #24999, #35374, .T. ) ;
#12736=ORIENTED_EDGE ( 'NONE', *, *, #26397, .F. ) ;
#12739=EDGE_CURVE ( 'NONE', #20566, #27049, #23975, .T. ) ;
#12742=DIRECTION ( 'NONE',  ( 0.000000000000000000, 0.000000000000000000, 1.000000000000000000 ) ) ;
#12745=DIRECTION ( 'NONE',  ( 0.000000000000000000, 0.000000000000000000, -1.000000000000000000 ) ) ;
#12746=CIRCLE ( 'NONE', #34931, 2.000000000000001776 ) ;
#12748=DIRECTION ( 'NONE',  ( 0.000000000000000000, 0.000000000000000000, -1.000000000000000000 ) ) ;
#12749=ADVANCED_FACE ( 'NONE', ( #31816 ), #26020, .F. ) ;
#12750=ORIENTED_EDGE ( 'NONE', *, *, #10024, .T. ) ;
#12751=ORIENTED_EDGE ( 'NONE', *, *, #30736, .T. ) ;
#12752=ADVANCED_FACE ( 'NONE', ( #15137 ), #17576, .F. ) ;
#12753=ORIENTED_EDGE ( 'NONE', *, *, #25679, .T. ) ;
#12756=DIRECTION ( 'NONE',  ( 0.000000000000000000, 0.000000000000000000, 1.000000000000000000 ) ) ;
#12757=DIRECTION ( 'NONE',  ( -1.000000000000000000, 0.000000000000000000, 0.000000000000000000 ) ) ;
#12759=CARTESIAN_POINT ( 'NONE',  ( 69.99999662536838230, -51.96152422706639840, -9.999999999999998224 ) ) ;
#12760=VERTEX_POINT ( 'NONE', #23410 ) ;
#12762=EDGE_CURVE ( 'NONE', #18228, #34831, #36560, .T. ) ;
#12764=DIRECTION ( 'NONE',  ( 1.000000000000000000, 0.000000000000000000, 0.000000000000000000 ) ) ;
#12766=DIRECTION ( 'NONE',  ( 0.000000000000000000, 0.000000000000000000, 1.000000000000000000 ) ) ;
#12767=EDGE_LOOP ( 'NONE', ( #3297, #34605, #10318, #33696 ) ) ;
#12770=CIRCLE ( 'NONE', #17567, 3.000000000000003553 ) ;
#12771=ORIENTED_EDGE ( 'NONE', *, *, #9315, .T. ) ;
#12772=AXIS2_PLACEMENT_3D ( 'NONE', #19089, #35416, #35588 ) ;
#12773=ORIENTED_EDGE ( 'NONE', *, *, #15903, .F. ) ;
#12774=CARTESIAN_POINT ( 'NONE',  ( -60.00000337463104216, 51.96152422706639129, -9.999999999999998224 ) ) ;
#12775=CARTESIAN_POINT ( 'NONE',  ( 2.999996625368676728, -77.94228634059960825, 17.49999999999999645 ) ) ;
#12777=ORIENTED_EDGE ( 'NONE', *, *, #25113, .F. ) ;
#12778=ORIENTED_EDGE ( 'NONE', *, *, #24117, .T. ) ;
#12779=ORIENTED_EDGE ( 'NONE', *, *, #30269, .T. ) ;
#12780=VECTOR ( 'NONE', #14298, 1000.000000000000000 ) ;
#12781=CARTESIAN_POINT ( 'NONE',  ( -63.10544949267008974, -59.98094631475026262, 12.50000000000000000 ) ) ;
#12782=ADVANCED_FACE ( 'NONE', ( #15325 ), #529, .F. ) ;
#12784=ORIENTED_EDGE ( 'NONE', *, *, #11134, .F. ) ;
#12785=ORIENTED_EDGE ( 'NONE', *, *, #4118, .F. ) ;
#12786=DIRECTION ( 'NONE',  ( 1.000000000000000000, 0.000000000000000000, 0.000000000000000000 ) ) ;
#12787=EDGE_LOOP ( 'NONE', ( #35047, #32710, #15889, #29917, #35592, #36917, #26796, #18696 ) ) ;
#12788=ORIENTED_EDGE ( 'NONE', *, *, #24324, .T. ) ;
#12790=DIRECTION ( 'NONE',  ( 1.000000000000000000, 0.000000000000000000, 0.000000000000000000 ) ) ;
#12791=ORIENTED_EDGE ( 'NONE', *, *, #12134, .F. ) ;
#12792=VERTEX_POINT ( 'NONE', #34843 ) ;
#12793=FACE_OUTER_BOUND ( 'NONE', #9147, .T. ) ;
#12795=DIRECTION ( 'NONE',  ( -0.000000000000000000, -0.000000000000000000, -1.000000000000000000 ) ) ;
#12796=DIRECTION ( 'NONE',  ( 1.000000000000000000, 0.000000000000000000, 0.000000000000000000 ) ) ;
#12797=AXIS2_PLACEMENT_3D ( 'NONE', #36426, #25183, #32522 ) ;
#12798=EDGE_CURVE ( 'NONE', #630, #1054, #22182, .T. ) ;
#12799=ORIENTED_EDGE ( 'NONE', *, *, #26435, .F. ) ;
#12800=CARTESIAN_POINT ( 'NONE',  ( -65.00000337463102085, 60.62177826491077326, 12.50000000000000000 ) ) ;
#12801=ORIENTED_EDGE ( 'NONE', *, *, #27757, .T. ) ;
#12802=EDGE_CURVE ( 'NONE', #10592, #7368, #12578, .T. ) ;
#12804=DIRECTION ( 'NONE',  ( 0.000000000000000000, 0.000000000000000000, 1.000000000000000000 ) ) ;
#12805=CYLINDRICAL_SURFACE ( 'NONE', #7606, 33.00000000000001421 ) ;
#12806=DIRECTION ( 'NONE',  ( 0.000000000000000000, 0.000000000000000000, 1.000000000000000000 ) ) ;
#12807=DIRECTION ( 'NONE',  ( 0.000000000000000000, 0.000000000000000000, 1.000000000000000000 ) ) ;
#12809=EDGE_CURVE ( 'NONE', #26240, #17105, #18887, .T. ) ;
#12810=CYLINDRICAL_SURFACE ( 'NONE', #10164, 2.000000000000001776 ) ;
#12811=AXIS2_PLACEMENT_3D ( 'NONE', #7684, #18930, #22122 ) ;
#12812=EDGE_CURVE ( 'NONE', #126, #17536, #22084, .T. ) ;
#12813=CARTESIAN_POINT ( 'NONE',  ( 57.99999662536843914, -34.64101615137759893, -5.000000000000000000 ) ) ;
#12814=VERTEX_POINT ( 'NONE', #13073 ) ;
#12815=FACE_OUTER_BOUND ( 'NONE', #12045, .T. ) ;
#12816=ADVANCED_FACE ( 'NONE', ( #10087 ), #35775, .F. ) ;
#12817=CARTESIAN_POINT ( 'NONE',  ( -83.00000337463092137, -25.98076211353322051, 17.49999999999999645 ) ) ;
#12819=ORIENTED_EDGE ( 'NONE', *, *, #33451, .T. ) ;
#12820=EDGE_LOOP ( 'NONE', ( #24492, #27044 ) ) ;
#12822=CARTESIAN_POINT ( 'NONE',  ( 19.99999662536858835, 69.28203230275516944, 12.50000000000000000 ) ) ;
#12823=FACE_OUTER_BOUND ( 'NONE', #1268, .T. ) ;
#12825=CIRCLE ( 'NONE', #5079, 2.000000000000001776 ) ;
#12826=EDGE_LOOP ( 'NONE', ( #8559, #26232, #28123, #28697, #15599, #9694, #4379, #14040, #27546, #1778, #28871, #26884 ) ) ;
#12828=EDGE_CURVE ( 'NONE', #17978, #10472, #6015, .T. ) ;
#12829=DIRECTION ( 'NONE',  ( 0.000000000000000000, 0.000000000000000000, 1.000000000000000000 ) ) ;
#12831=CARTESIAN_POINT ( 'NONE',  ( 69.99999662536839651, -3.469446951953614189E-15, -9.999999999999998224 ) ) ;
#12832=VERTEX_POINT ( 'NONE', #15527 ) ;
#12833=CYLINDRICAL_SURFACE ( 'NONE', #21547, 2.000000000000001776 ) ;
#12834=ORIENTED_EDGE ( 'NONE', *, *, #13082, .F. ) ;
#12836=AXIS2_PLACEMENT_3D ( 'NONE', #8611, #20046, #20783 ) ;
#12837=AXIS2_PLACEMENT_3D ( 'NONE', #4106, #26972, #1282 ) ;
#12839=CARTESIAN_POINT ( 'NONE',  ( 86.99999662536831124, -8.660254037844397956, 17.49999999999999645 ) ) ;
#12840=CIRCLE ( 'NONE', #3270, 2.000000000000000000 ) ;
#12841=DIRECTION ( 'NONE',  ( 0.000000000000000000, 0.000000000000000000, -1.000000000000000000 ) ) ;
#12842=VERTEX_POINT ( 'NONE', #26957 ) ;
#12846=DIRECTION ( 'NONE',  ( 0.4999999999999919509, -0.8660254037844433705, 0.000000000000000000 ) ) ;
#12847=ADVANCED_FACE ( 'NONE', ( #1267 ), #21320, .F. ) ;
#12848=VECTOR ( 'NONE', #6569, 1000.000000000000000 ) ;
#12850=CARTESIAN_POINT ( 'NONE',  ( -13.00000337463125710, -77.94228634059960825, 17.49999999999999645 ) ) ;
#12851=ORIENTED_EDGE ( 'NONE', *, *, #5571, .F. ) ;
#12852=EDGE_CURVE ( 'NONE', #11966, #24803, #14838, .T. ) ;
#12854=CIRCLE ( 'NONE', #34449, 33.00000000000001421 ) ;
#12856=DIRECTION ( 'NONE',  ( 0.000000000000000000, 0.000000000000000000, 1.000000000000000000 ) ) ;
#12857=CIRCLE ( 'NONE', #27204, 2.000000000000001776 ) ;
#12860=EDGE_CURVE ( 'NONE', #33375, #30431, #20219, .T. ) ;
#12861=CARTESIAN_POINT ( 'NONE',  ( 69.99999662536838230, -34.64101615137759183, -9.999999999999998224 ) ) ;
#12862=DIRECTION ( 'NONE',  ( 0.000000000000000000, 0.000000000000000000, 1.000000000000000000 ) ) ;
#12863=AXIS2_PLACEMENT_3D ( 'NONE', #13446, #13651, #33899 ) ;
#12865=DIRECTION ( 'NONE',  ( 0.000000000000000000, 0.000000000000000000, 1.000000000000000000 ) ) ;
#12867=PLANE ( 'NONE',  #21192 ) ;
#12871=ADVANCED_FACE ( 'NONE', ( #15887 ), #27316, .F. ) ;
#12872=VERTEX_POINT ( 'NONE', #33126 ) ;
#12873=ADVANCED_FACE ( 'NONE', ( #7445 ), #11331, .F. ) ;
#12874=VERTEX_POINT ( 'NONE', #5698 ) ;
#12875=DIRECTION ( 'NONE',  ( 1.000000000000000000, 0.000000000000000000, 0.000000000000000000 ) ) ;
#12877=VECTOR ( 'NONE', #19605, 1000.000000000000000 ) ;
#12878=DIRECTION ( 'NONE',  ( -1.000000000000000000, 0.000000000000000000, 0.000000000000000000 ) ) ;
#12879=VERTEX_POINT ( 'NONE', #20321 ) ;
#12880=EDGE_CURVE ( 'NONE', #21760, #4105, #4656, .T. ) ;
#12881=AXIS2_PLACEMENT_3D ( 'NONE', #20469, #9611, #28905 ) ;
#12883=EDGE_LOOP ( 'NONE', ( #25287, #21103, #6555, #2708 ) ) ;
#12884=DIRECTION ( 'NONE',  ( -1.000000000000000000, 0.000000000000000000, 0.000000000000000000 ) ) ;
#12885=AXIS2_PLACEMENT_3D ( 'NONE', #4845, #22637, #36144 ) ;
#12886=AXIS2_PLACEMENT_3D ( 'NONE', #3340, #3541, #332 ) ;
#12888=ORIENTED_EDGE ( 'NONE', *, *, #32650, .T. ) ;
#12889=EDGE_LOOP ( 'NONE', ( #1306, #28563 ) ) ;
#12890=CARTESIAN_POINT ( 'NONE',  ( -60.00000337463104216, 51.96152422706639129, -5.000000000000000000 ) ) ;
#12891=ORIENTED_EDGE ( 'NONE', *, *, #29672, .F. ) ;
#12892=CIRCLE ( 'NONE', #16493, 2.000000000000001776 ) ;
#12894=CIRCLE ( 'NONE', #22486, 2.000000000000001776 ) ;
#12895=CARTESIAN_POINT ( 'NONE',  ( -52.39915983220772233, -35.19434990244957362, 12.49999999999999822 ) ) ;
#12896=FACE_OUTER_BOUND ( 'NONE', #19963, .T. ) ;
#12899=FACE_OUTER_BOUND ( 'NONE', #11861, .T. ) ;
#12900=DIRECTION ( 'NONE',  ( 0.000000000000000000, 0.000000000000000000, 1.000000000000000000 ) ) ;
#12901=ORIENTED_EDGE ( 'NONE', *, *, #7768, .F. ) ;
#12902=EDGE_CURVE ( 'NONE', #36225, #14998, #25612, .T. ) ;
#12903=ORIENTED_EDGE ( 'NONE', *, *, #1192, .T. ) ;
#12905=AXIS2_PLACEMENT_3D ( 'NONE', #12024, #17854, #18037 ) ;
#12906=FACE_OUTER_BOUND ( 'NONE', #24816, .T. ) ;
#12907=DIRECTION ( 'NONE',  ( 1.000000000000000000, 0.000000000000000000, 0.000000000000000000 ) ) ;
#12908=EDGE_LOOP ( 'NONE', ( #5361, #15251, #12753, #33363, #1726, #30429 ) ) ;
#12909=VECTOR ( 'NONE', #974, 1000.000000000000000 ) ;
#12911=AXIS2_PLACEMENT_3D ( 'NONE', #8969, #9321, #20761 ) ;
#12912=CARTESIAN_POINT ( 'NONE',  ( 47.99999662536846756, 69.28203230275516944, -5.000000000000000000 ) ) ;
#12913=AXIS2_PLACEMENT_3D ( 'NONE', #7699, #15947, #33385 ) ;
#12914=EDGE_LOOP ( 'NONE', ( #33726, #6008 ) ) ;
#12915=CIRCLE ( 'NONE', #9923, 2.000000000000001776 ) ;
#12916=DIRECTION ( 'NONE',  ( 0.000000000000000000, 0.000000000000000000, 1.000000000000000000 ) ) ;
#12917=AXIS2_PLACEMENT_3D ( 'NONE', #1646, #36336, #1835 ) ;
#12918=DIRECTION ( 'NONE',  ( -1.000000000000000000, 0.000000000000000000, 0.000000000000000000 ) ) ;
#12919=CARTESIAN_POINT ( 'NONE',  ( 31.02796211690949235, -59.29837256189548356, -49.86561046011506448 ) ) ;
#12920=CARTESIAN_POINT ( 'NONE',  ( -3.000003374631308173, 77.94228634059957983, 17.49999999999999645 ) ) ;
#12923=VERTEX_POINT ( 'NONE', #9232 ) ;
#12925=LINE ( 'NONE', #4320, #3288 ) ;
#12926=CARTESIAN_POINT ( 'NONE',  ( 34.99999662536855283, 60.62177826491078747, -5.000000000000000000 ) ) ;
#12927=ADVANCED_FACE ( 'NONE', ( #34387 ), #3251, .F. ) ;
#12928=CARTESIAN_POINT ( 'NONE',  ( -60.00000337463104216, 51.96152422706639129, -9.999999999999998224 ) ) ;
#12929=DIRECTION ( 'NONE',  ( 0.000000000000000000, 0.000000000000000000, -1.000000000000000000 ) ) ;
#12930=ORIENTED_EDGE ( 'NONE', *, *, #21090, .F. ) ;
#12931=AXIS2_PLACEMENT_3D ( 'NONE', #23351, #34790, #6648 ) ;
#12932=DIRECTION ( 'NONE',  ( 1.000000000000000000, 0.000000000000000000, 0.000000000000000000 ) ) ;
#12933=CARTESIAN_POINT ( 'NONE',  ( 64.99999662536839651, 60.62177826491078747, -5.000000000000000000 ) ) ;
#12935=ORIENTED_EDGE ( 'NONE', *, *, #18683, .T. ) ;
#12937=CARTESIAN_POINT ( 'NONE',  ( 91.99999662536828282, 0.000000000000000000, -9.999999999999998224 ) ) ;
#12938=ORIENTED_EDGE ( 'NONE', *, *, #14475, .F. ) ;
#12939=AXIS2_PLACEMENT_3D ( 'NONE', #2347, #13583, #17329 ) ;
#12940=AXIS2_PLACEMENT_3D ( 'NONE', #876, #6319, #12107 ) ;
#12941=CARTESIAN_POINT ( 'NONE',  ( 27.78182860042856461, 56.67878100130339902, 12.49999999999999822 ) ) ;
#12943=CARTESIAN_POINT ( 'NONE',  ( -62.00000337463104927, 51.96152422706639129, 12.50000000000000000 ) ) ;
#12944=AXIS2_PLACEMENT_3D ( 'NONE', #7669, #36357, #10668 ) ;
#12945=DIRECTION ( 'NONE',  ( 1.000000000000000000, 0.000000000000000000, 0.000000000000000000 ) ) ;
#12946=ORIENTED_EDGE ( 'NONE', *, *, #33435, .F. ) ;
#12947=ORIENTED_EDGE ( 'NONE', *, *, #23510, .T. ) ;
#12949=CIRCLE ( 'NONE', #1585, 27.00000000000001421 ) ;
#12950=VERTEX_POINT ( 'NONE', #5004 ) ;
#12951=DIRECTION ( 'NONE',  ( 0.000000000000000000, 0.000000000000000000, -1.000000000000000000 ) ) ;
#12952=DIRECTION ( 'NONE',  ( 0.000000000000000000, 0.000000000000000000, 1.000000000000000000 ) ) ;
#12954=DIRECTION ( 'NONE',  ( 0.000000000000000000, 0.000000000000000000, 1.000000000000000000 ) ) ;
#12955=LINE ( 'NONE', #18609, #28292 ) ;
#12958=CARTESIAN_POINT ( 'NONE',  ( -82.00000337463096400, -34.64101615137762025, 12.50000000000000000 ) ) ;
#12959=AXIS2_PLACEMENT_3D ( 'NONE', #29454, #3420, #9409 ) ;
#12961=EDGE_CURVE ( 'NONE', #25364, #30431, #27393, .T. ) ;
#12964=VERTEX_POINT ( 'NONE', #25092 ) ;
#12965=CARTESIAN_POINT ( 'NONE',  ( 64.99999662536842493, 43.30127018922200222, -9.999999999999998224 ) ) ;
#12967=DIRECTION ( 'NONE',  ( 0.000000000000000000, 0.000000000000000000, 1.000000000000000000 ) ) ;
#12968=CIRCLE ( 'NONE', #21948, 2.000000000000000000 ) ;
#12969=ORIENTED_EDGE ( 'NONE', *, *, #30072, .F. ) ;
#12970=CIRCLE ( 'NONE', #18960, 3.000000000000006217 ) ;
#12972=CIRCLE ( 'NONE', #2199, 2.000000000000000000 ) ;
#12973=DIRECTION ( 'NONE',  ( 0.000000000000000000, 0.000000000000000000, -1.000000000000000000 ) ) ;
#12976=CARTESIAN_POINT ( 'NONE',  ( 31.99999662536856704, 69.28203230275518365, -9.999999999999998224 ) ) ;
#12977=VERTEX_POINT ( 'NONE', #26320 ) ;
#12978=ORIENTED_EDGE ( 'NONE', *, *, #10501, .F. ) ;
#12979=ORIENTED_EDGE ( 'NONE', *, *, #27891, .T. ) ;
#12980=CIRCLE ( 'NONE', #22574, 3.000000000000002665 ) ;
#12983=ORIENTED_EDGE ( 'NONE', *, *, #6192, .F. ) ;
#12984=FACE_BOUND ( 'NONE', #20414, .T. ) ;
#12985=ORIENTED_EDGE ( 'NONE', *, *, #8603, .F. ) ;
#12987=AXIS2_PLACEMENT_3D ( 'NONE', #7715, #8078, #36210 ) ;
#12989=DIRECTION ( 'NONE',  ( 0.000000000000000000, 0.000000000000000000, -1.000000000000000000 ) ) ;
#12992=EDGE_CURVE ( 'NONE', #15625, #5415, #14879, .T. ) ;
#12993=CARTESIAN_POINT ( 'NONE',  ( 19.99999662536861678, -69.28203230275519786, 17.49999999999999645 ) ) ;
#12994=ORIENTED_EDGE ( 'NONE', *, *, #5235, .T. ) ;
#12995=ORIENTED_EDGE ( 'NONE', *, *, #11886, .F. ) ;
#12996=CYLINDRICAL_SURFACE ( 'NONE', #27505, 2.000000000000001776 ) ;
#12997=CARTESIAN_POINT ( 'NONE',  ( -65.00000337463102085, 60.62177826491077326, 17.49999999999999645 ) ) ;
#12998=AXIS2_PLACEMENT_3D ( 'NONE', #22047, #33666, #28217 ) ;
#13000=CARTESIAN_POINT ( 'NONE',  ( -80.00000337463096400, -34.64101615137762025, 12.50000000000000000 ) ) ;
#13001=CARTESIAN_POINT ( 'NONE',  ( 32.99999662536853862, 77.94228634059959404, -9.999999999999998224 ) ) ;
#13002=CIRCLE ( 'NONE', #16017, 2.000000000000001776 ) ;
#13003=EDGE_LOOP ( 'NONE', ( #21203, #937, #11332, #36995 ) ) ;
#13004=CARTESIAN_POINT ( 'NONE',  ( -70.00000337463099243, 17.32050807568877460, -9.999999999999998224 ) ) ;
#13006=CARTESIAN_POINT ( 'NONE',  ( -10.00000337463128197, 86.60254037844397601, -9.999999999999998224 ) ) ;
#13007=EDGE_CURVE ( 'NONE', #11624, #23282, #28594, .T. ) ;
#13008=DIRECTION ( 'NONE',  ( 0.000000000000000000, 0.000000000000000000, -1.000000000000000000 ) ) ;
#13009=CARTESIAN_POINT ( 'NONE',  ( 4.999996625368676284, -77.94228634059960825, -5.000000000000000000 ) ) ;
#13013=DIRECTION ( 'NONE',  ( -0.5000000000000098810, -0.8660254037844328234, 0.000000000000000000 ) ) ;
#13014=EDGE_CURVE ( 'NONE', #2540, #11374, #8515, .T. ) ;
#13015=AXIS2_PLACEMENT_3D ( 'NONE', #15433, #6436, #1356 ) ;
#13016=CARTESIAN_POINT ( 'NONE',  ( -66.50936994187880202, 41.98909163213660634, -5.000000000000000000 ) ) ;
#13018=DIRECTION ( 'NONE',  ( 1.000000000000000000, 0.000000000000000000, 0.000000000000000000 ) ) ;
#13019=AXIS2_PLACEMENT_3D ( 'NONE', #9821, #12448, #32896 ) ;
#13021=LINE ( 'NONE', #27640, #9752 ) ;
#13022=CIRCLE ( 'NONE', #4064, 2.000000000000001776 ) ;
#13023=VERTEX_POINT ( 'NONE', #31905 ) ;
#13024=ORIENTED_EDGE ( 'NONE', *, *, #26092, .F. ) ;
#13026=CIRCLE ( 'NONE', #9446, 33.00000000000001421 ) ;
#13027=CARTESIAN_POINT ( 'NONE',  ( 51.13139720814399425, -27.50000000000022737, -10.00000000000000178 ) ) ;
#13028=DIRECTION ( 'NONE',  ( 1.000000000000000000, 0.000000000000000000, 0.000000000000000000 ) ) ;
#13029=ORIENTED_EDGE ( 'NONE', *, *, #20590, .T. ) ;
#13031=CIRCLE ( 'NONE', #34011, 2.000000000000001776 ) ;
#13032=DIRECTION ( 'NONE',  ( 1.000000000000000000, 0.000000000000000000, 0.000000000000000000 ) ) ;
#13033=ADVANCED_FACE ( 'NONE', ( #17139 ), #20483, .F. ) ;
#13035=VERTEX_POINT ( 'NONE', #14507 ) ;
#13036=DIRECTION ( 'NONE',  ( 0.000000000000000000, 0.000000000000000000, 1.000000000000000000 ) ) ;
#13037=ORIENTED_EDGE ( 'NONE', *, *, #35053, .F. ) ;
#13038=DIRECTION ( 'NONE',  ( 0.000000000000000000, 0.000000000000000000, 1.000000000000000000 ) ) ;
#13039=CIRCLE ( 'NONE', #34017, 27.00000000000001776 ) ;
#13040=EDGE_CURVE ( 'NONE', #11692, #14483, #34607, .T. ) ;
#13044=EDGE_CURVE ( 'NONE', #14998, #36225, #8263, .T. ) ;
#13046=EDGE_LOOP ( 'NONE', ( #8660, #16285, #28530, #5062 ) ) ;
#13047=DIRECTION ( 'NONE',  ( 1.000000000000000000, 0.000000000000000000, 0.000000000000000000 ) ) ;
#13048=CIRCLE ( 'NONE', #34612, 2.000000000000001776 ) ;
#13049=AXIS2_PLACEMENT_3D ( 'NONE', #2073, #7524, #4907 ) ;
#13050=CIRCLE ( 'NONE', #25650, 2.000000000000001776 ) ;
#13051=DIRECTION ( 'NONE',  ( 0.000000000000000000, 0.000000000000000000, 1.000000000000000000 ) ) ;
#13053=VECTOR ( 'NONE', #24218, 1000.000000000000000 ) ;
#13054=CARTESIAN_POINT ( 'NONE',  ( 81.99999662536833966, -3.469446951953614189E-15, -9.999999999999998224 ) ) ;
#13055=DIRECTION ( 'NONE',  ( 0.000000000000000000, 0.000000000000000000, 1.000000000000000000 ) ) ;
#13056=ORIENTED_EDGE ( 'NONE', *, *, #23273, .T. ) ;
#13057=DIRECTION ( 'NONE',  ( 0.000000000000000000, 0.000000000000000000, -1.000000000000000000 ) ) ;
#13058=CARTESIAN_POINT ( 'NONE',  ( 74.99999662536835388, -25.98076211353319565, -9.999999999999998224 ) ) ;
#13059=DIRECTION ( 'NONE',  ( 0.000000000000000000, 0.000000000000000000, 1.000000000000000000 ) ) ;
#13061=EDGE_CURVE ( 'NONE', #5447, #21544, #29198, .T. ) ;
#13062=ORIENTED_EDGE ( 'NONE', *, *, #13007, .T. ) ;
#13063=CYLINDRICAL_SURFACE ( 'NONE', #31539, 2.000000000000001776 ) ;
#13064=AXIS2_PLACEMENT_3D ( 'NONE', #19839, #16846, #22840 ) ;
#13065=DIRECTION ( 'NONE',  ( 0.000000000000000000, 0.000000000000000000, 1.000000000000000000 ) ) ;
#13067=ORIENTED_EDGE ( 'NONE', *, *, #8140, .F. ) ;
#13068=CIRCLE ( 'NONE', #8298, 2.000000000000001776 ) ;
#13070=DIRECTION ( 'NONE',  ( 0.000000000000000000, 0.000000000000000000, -1.000000000000000000 ) ) ;
#13071=CIRCLE ( 'NONE', #13668, 2.000000000000001776 ) ;
#13073=CARTESIAN_POINT ( 'NONE',  ( 77.99999662536833966, 17.32050807568879236, -5.000000000000000000 ) ) ;
#13074=ORIENTED_EDGE ( 'NONE', *, *, #6106, .F. ) ;
#13075=CIRCLE ( 'NONE', #19669, 2.000000000000001776 ) ;
#13076=ORIENTED_EDGE ( 'NONE', *, *, #3782, .T. ) ;
#13077=DIRECTION ( 'NONE',  ( 1.000000000000000000, 0.000000000000000000, 0.000000000000000000 ) ) ;
#13080=DIRECTION ( 'NONE',  ( 0.000000000000000000, 0.000000000000000000, -1.000000000000000000 ) ) ;
#13082=EDGE_CURVE ( 'NONE', #28140, #24230, #23216, .T. ) ;
#13084=ORIENTED_EDGE ( 'NONE', *, *, #732, .T. ) ;
#13085=CARTESIAN_POINT ( 'NONE',  ( -75.00000337463097821, 8.660254037844374864, -9.999999999999998224 ) ) ;
#13088=EDGE_CURVE ( 'NONE', #24516, #14569, #22605, .T. ) ;
#13089=AXIS2_PLACEMENT_3D ( 'NONE', #820, #12232, #20898 ) ;
#13090=CARTESIAN_POINT ( 'NONE',  ( -77.00000337463100664, -43.30127018922202353, 12.50000000000000000 ) ) ;
#13091=ORIENTED_EDGE ( 'NONE', *, *, #19334, .T. ) ;
#13094=ORIENTED_EDGE ( 'NONE', *, *, #16661, .T. ) ;
#13095=EDGE_CURVE ( 'NONE', #34413, #3514, #24228, .T. ) ;
#13098=FACE_OUTER_BOUND ( 'NONE', #11745, .T. ) ;
#13099=AXIS2_PLACEMENT_3D ( 'NONE', #10323, #24202, #1155 ) ;
#13100=CARTESIAN_POINT ( 'NONE',  ( 81.99999662536833966, 17.32050807568879236, -5.000000000000000000 ) ) ;
#13101=DIRECTION ( 'NONE',  ( 0.8660254037844413721, 0.4999999999999950595, 0.000000000000000000 ) ) ;
#13102=EDGE_LOOP ( 'NONE', ( #3732, #15535, #19998, #33957 ) ) ;
#13103=DIRECTION ( 'NONE',  ( 0.000000000000000000, 0.000000000000000000, -1.000000000000000000 ) ) ;
#13105=LINE ( 'NONE', #1669, #21326 ) ;
#13107=EDGE_LOOP ( 'NONE', ( #29517, #24362 ) ) ;
#13108=ADVANCED_FACE ( 'NONE', ( #18628 ), #35331, .F. ) ;
#13109=EDGE_LOOP ( 'NONE', ( #23864, #17598, #22813, #3568 ) ) ;
#13110=ORIENTED_EDGE ( 'NONE', *, *, #31522, .F. ) ;
#13111=EDGE_CURVE ( 'NONE', #29187, #14423, #1053, .T. ) ;
#13112=DIRECTION ( 'NONE',  ( -1.000000000000000000, 0.000000000000000000, 0.000000000000000000 ) ) ;
#13113=ADVANCED_FACE ( 'NONE', ( #29657 ), #27041, .F. ) ;
#13114=CIRCLE ( 'NONE', #33493, 2.000000000000001776 ) ;
#13115=DIRECTION ( 'NONE',  ( 0.000000000000000000, 0.000000000000000000, -1.000000000000000000 ) ) ;
#13116=VERTEX_POINT ( 'NONE', #35679 ) ;
#13117=CARTESIAN_POINT ( 'NONE',  ( 0.000000000000000000, -55.00000000000000000, -10.00000000000000178 ) ) ;
#13118=CARTESIAN_POINT ( 'NONE',  ( -32.00000337463119848, -69.28203230275522628, -9.999999999999998224 ) ) ;
#13121=CYLINDRICAL_SURFACE ( 'NONE', #53, 2.000000000000001776 ) ;
#13123=DIRECTION ( 'NONE',  ( -1.000000000000000000, 1.798972493605577187E-15, 0.000000000000000000 ) ) ;
#13124=AXIS2_PLACEMENT_3D ( 'NONE', #9268, #31937, #6479 ) ;
#13125=CARTESIAN_POINT ( 'NONE',  ( 79.99999662536833966, 17.32050807568879236, -9.999999999999998224 ) ) ;
#13126=DIRECTION ( 'NONE',  ( -0.000000000000000000, -0.000000000000000000, 1.000000000000000000 ) ) ;
#13127=FACE_OUTER_BOUND ( 'NONE', #29253, .T. ) ;
#13129=ORIENTED_EDGE ( 'NONE', *, *, #25447, .T. ) ;
#13131=CIRCLE ( 'NONE', #20299, 2.000000000000001776 ) ;
#13132=CARTESIAN_POINT ( 'NONE',  ( -68.00000337463099243, 17.32050807568877460, 17.49999999999999645 ) ) ;
#13133=CARTESIAN_POINT ( 'NONE',  ( 19.99999662536857770, 86.60254037844397601, -5.000000000000000000 ) ) ;
#13134=DIRECTION ( 'NONE',  ( 0.000000000000000000, 0.000000000000000000, 1.000000000000000000 ) ) ;
#13135=ORIENTED_EDGE ( 'NONE', *, *, #22868, .T. ) ;
#13137=DIRECTION ( 'NONE',  ( 0.000000000000000000, 0.000000000000000000, 1.000000000000000000 ) ) ;
#13138=DIRECTION ( 'NONE',  ( -1.000000000000000000, 0.000000000000000000, 0.000000000000000000 ) ) ;
#13139=FACE_OUTER_BOUND ( 'NONE', #34678, .T. ) ;
#13142=ORIENTED_EDGE ( 'NONE', *, *, #16907, .T. ) ;
#13143=CIRCLE ( 'NONE', #35909, 2.000000000000001776 ) ;
#13146=AXIS2_PLACEMENT_3D ( 'NONE', #28804, #24116, #23553 ) ;
#13147=DIRECTION ( 'NONE',  ( 0.000000000000000000, 0.000000000000000000, -1.000000000000000000 ) ) ;
#13148=ORIENTED_EDGE ( 'NONE', *, *, #11989, .T. ) ;
#13150=VERTEX_POINT ( 'NONE', #12976 ) ;
#13151=DIRECTION ( 'NONE',  ( 0.000000000000000000, 0.000000000000000000, 1.000000000000000000 ) ) ;
#13154=AXIS2_PLACEMENT_3D ( 'NONE', #29542, #15869, #26554 ) ;
#13155=EDGE_CURVE ( 'NONE', #14823, #32711, #36983, .T. ) ;
#13156=FACE_BOUND ( 'NONE', #25727, .T. ) ;
#13158=DIRECTION ( 'NONE',  ( -1.000000000000000000, 0.000000000000000000, 0.000000000000000000 ) ) ;
#13159=CARTESIAN_POINT ( 'NONE',  ( 29.99999662536856349, 69.28203230275518365, 12.50000000000000000 ) ) ;
#13160=CARTESIAN_POINT ( 'NONE',  ( 16.99999662536859901, 77.94228634059957983, -9.999999999999998224 ) ) ;
#13161=EDGE_LOOP ( 'NONE', ( #31661, #34069 ) ) ;
#13163=CARTESIAN_POINT ( 'NONE',  ( 56.99999662536844625, 60.62177826491077326, -9.999999999999998224 ) ) ;
#13164=FACE_OUTER_BOUND ( 'NONE', #22283, .T. ) ;
#13165=VERTEX_POINT ( 'NONE', #17877 ) ;
#13166=CARTESIAN_POINT ( 'NONE',  ( 84.99999662536831124, -8.660254037844397956, 12.50000000000000000 ) ) ;
#13167=LINE ( 'NONE', #24621, #32123 ) ;
#13168=VECTOR ( 'NONE', #1795, 1000.000000000000000 ) ;
#13170=ORIENTED_EDGE ( 'NONE', *, *, #1479, .F. ) ;
#13171=VECTOR ( 'NONE', #36231, 1000.000000000000000 ) ;
#13172=DIRECTION ( 'NONE',  ( 1.000000000000000000, 0.000000000000000000, 0.000000000000000000 ) ) ;
#13176=ORIENTED_EDGE ( 'NONE', *, *, #1079, .F. ) ;
#13177=ORIENTED_EDGE ( 'NONE', *, *, #11404, .T. ) ;
#13178=AXIS2_PLACEMENT_3D ( 'NONE', #969, #26652, #12388 ) ;
#13179=VERTEX_POINT ( 'NONE', #29306 ) ;
#13186=VERTEX_POINT ( 'NONE', #32478 ) ;
#13187=ORIENTED_EDGE ( 'NONE', *, *, #21206, .F. ) ;
#13188=EDGE_CURVE ( 'NONE', #30738, #8351, #36400, .T. ) ;
#13189=CARTESIAN_POINT ( 'NONE',  ( 59.99999662536843914, -34.64101615137759893, -9.999999999999998224 ) ) ;
#13190=CARTESIAN_POINT ( 'NONE',  ( -73.00000337463100664, -43.30127018922202353, -9.999999999999998224 ) ) ;
#13191=ORIENTED_EDGE ( 'NONE', *, *, #17832, .T. ) ;
#13194=CARTESIAN_POINT ( 'NONE',  ( -75.00000337463100664, -43.30127018922202353, -9.999999999999998224 ) ) ;
#13195=DIRECTION ( 'NONE',  ( 1.000000000000000000, 0.000000000000000000, 0.000000000000000000 ) ) ;
#13196=CARTESIAN_POINT ( 'NONE',  ( -75.00000337463097821, 43.30127018922197379, -9.999999999999998224 ) ) ;
#13197=FACE_OUTER_BOUND ( 'NONE', #16220, .T. ) ;
#13199=CARTESIAN_POINT ( 'NONE',  ( 42.99999662536848888, -77.94228634059960825, -5.000000000000000000 ) ) ;
#13201=VECTOR ( 'NONE', #17811, 1000.000000000000000 ) ;
#13205=AXIS2_PLACEMENT_3D ( 'NONE', #12713, #27156, #12907 ) ;
#13206=DIRECTION ( 'NONE',  ( 1.000000000000000000, 0.000000000000000000, 0.000000000000000000 ) ) ;
#13207=CYLINDRICAL_SURFACE ( 'NONE', #23704, 2.000000000000001776 ) ;
#13208=DIRECTION ( 'NONE',  ( 0.000000000000000000, 0.000000000000000000, 1.000000000000000000 ) ) ;
#13209=CARTESIAN_POINT ( 'NONE',  ( 86.45172111230354517, -31.46585318596159553, -4.999999999999997335 ) ) ;
#13210=DIRECTION ( 'NONE',  ( 1.000000000000000000, 0.000000000000000000, 0.000000000000000000 ) ) ;
#13212=CARTESIAN_POINT ( 'NONE',  ( -45.00000337463112743, -60.62177826491080168, 17.49999999999999645 ) ) ;
#13213=DIRECTION ( 'NONE',  ( 0.000000000000000000, 0.000000000000000000, -1.000000000000000000 ) ) ;
#13214=DIRECTION ( 'NONE',  ( 0.000000000000000000, 0.000000000000000000, 1.000000000000000000 ) ) ;
#13215=ORIENTED_EDGE ( 'NONE', *, *, #5423, .T. ) ;
#13217=ORIENTED_EDGE ( 'NONE', *, *, #25143, .F. ) ;
#13219=DIRECTION ( 'NONE',  ( 0.000000000000000000, 0.000000000000000000, 1.000000000000000000 ) ) ;
#13220=CARTESIAN_POINT ( 'NONE',  ( -3.374631327851540519E-06, 86.60254037844397601, -9.999999999999998224 ) ) ;
#13221=VERTEX_POINT ( 'NONE', #4551 ) ;
#13223=DIRECTION ( 'NONE',  ( 0.000000000000000000, 0.000000000000000000, 1.000000000000000000 ) ) ;
#13224=FACE_OUTER_BOUND ( 'NONE', #17742, .T. ) ;
#13225=VERTEX_POINT ( 'NONE', #21784 ) ;
#13226=AXIS2_PLACEMENT_3D ( 'NONE', #7870, #19305, #30718 ) ;
#13228=EDGE_CURVE ( 'NONE', #31910, #29798, #13635, .T. ) ;
#13229=EDGE_LOOP ( 'NONE', ( #973, #11395, #34813, #27407, #14166, #8616 ) ) ;
#13233=LINE ( 'NONE', #24677, #24535 ) ;
#13234=CARTESIAN_POINT ( 'NONE',  ( 26.99999662536859546, -77.94228634059960825, 17.49999999999999645 ) ) ;
#13235=ORIENTED_EDGE ( 'NONE', *, *, #26768, .T. ) ;
#13236=CARTESIAN_POINT ( 'NONE',  ( 69.99999662536839651, 34.64101615137758472, -5.000000000000000000 ) ) ;
#13237=DIRECTION ( 'NONE',  ( -1.000000000000000000, 0.000000000000000000, 0.000000000000000000 ) ) ;
#13239=ORIENTED_EDGE ( 'NONE', *, *, #12134, .T. ) ;
#13240=DIRECTION ( 'NONE',  ( -1.000000000000000000, 0.000000000000000000, 0.000000000000000000 ) ) ;
#13242=ORIENTED_EDGE ( 'NONE', *, *, #2980, .T. ) ;
#13243=DIRECTION ( 'NONE',  ( 1.000000000000000000, 0.000000000000000000, 0.000000000000000000 ) ) ;
#13246=EDGE_CURVE ( 'NONE', #19401, #3360, #28010, .T. ) ;
#13248=EDGE_LOOP ( 'NONE', ( #8228, #9745, #24483, #2396 ) ) ;
#13249=CARTESIAN_POINT ( 'NONE',  ( 62.97617850287784336, 4.279621169095339184, -49.86561046011506448 ) ) ;
#13251=EDGE_CURVE ( 'NONE', #19079, #28212, #2295, .T. ) ;
#13252=DIRECTION ( 'NONE',  ( 0.000000000000000000, 0.000000000000000000, -1.000000000000000000 ) ) ;
#13253=ORIENTED_EDGE ( 'NONE', *, *, #31625, .F. ) ;
#13255=DIRECTION ( 'NONE',  ( -1.000000000000000000, 0.000000000000000000, 0.000000000000000000 ) ) ;
#13256=CARTESIAN_POINT ( 'NONE',  ( -57.00000337463107059, 60.62177826491078747, 17.49999999999999645 ) ) ;
#13258=DIRECTION ( 'NONE',  ( 1.000000000000000000, 0.000000000000000000, 0.000000000000000000 ) ) ;
#13260=EDGE_LOOP ( 'NONE', ( #18700, #24452 ) ) ;
#13261=CARTESIAN_POINT ( 'NONE',  ( -20.00000337463122690, 86.60254037844397601, -9.999999999999998224 ) ) ;
#13262=DIRECTION ( 'NONE',  ( 0.000000000000000000, 0.000000000000000000, -1.000000000000000000 ) ) ;
#13264=DIRECTION ( 'NONE',  ( 0.000000000000000000, 0.000000000000000000, 1.000000000000000000 ) ) ;
#13266=AXIS2_PLACEMENT_3D ( 'NONE', #32042, #752, #6383 ) ;
#13267=DIRECTION ( 'NONE',  ( 0.000000000000000000, 0.000000000000000000, -1.000000000000000000 ) ) ;
#13269=CARTESIAN_POINT ( 'NONE',  ( 66.99999662536841072, 25.98076211353318854, -9.999999999999998224 ) ) ;
#13270=EDGE_LOOP ( 'NONE', ( #36686, #11799, #15786, #27647 ) ) ;
#13271=DIRECTION ( 'NONE',  ( 0.000000000000000000, 0.000000000000000000, 1.000000000000000000 ) ) ;
#13272=EDGE_LOOP ( 'NONE', ( #23432, #3323 ) ) ;
#13273=DIRECTION ( 'NONE',  ( 1.000000000000000000, 0.000000000000000000, 0.000000000000000000 ) ) ;
#13274=CYLINDRICAL_SURFACE ( 'NONE', #21538, 2.000000000000001776 ) ;
#13278=DIRECTION ( 'NONE',  ( 1.000000000000000000, 0.000000000000000000, 0.000000000000000000 ) ) ;
#13279=CYLINDRICAL_SURFACE ( 'NONE', #11156, 2.000000000000000000 ) ;
#13281=EDGE_LOOP ( 'NONE', ( #35927, #12819 ) ) ;
#13282=EDGE_CURVE ( 'NONE', #24999, #625, #8391, .T. ) ;
#13283=VERTEX_POINT ( 'NONE', #5303 ) ;
#13284=VECTOR ( 'NONE', #17852, 1000.000000000000000 ) ;
#13285=CYLINDRICAL_SURFACE ( 'NONE', #20961, 2.000000000000001776 ) ;
#13286=EDGE_CURVE ( 'NONE', #11018, #13221, #2309, .T. ) ;
#13289=CARTESIAN_POINT ( 'NONE',  ( -65.00000337463104927, -25.98076211353322051, -5.000000000000000000 ) ) ;
#13291=CYLINDRICAL_SURFACE ( 'NONE', #3065, 2.000000000000001776 ) ;
#13293=LINE ( 'NONE', #16137, #8309 ) ;
#13295=EDGE_CURVE ( 'NONE', #1072, #30254, #8313, .T. ) ;
#13296=DIRECTION ( 'NONE',  ( 0.000000000000000000, 0.000000000000000000, 1.000000000000000000 ) ) ;
#13299=ORIENTED_EDGE ( 'NONE', *, *, #16427, .F. ) ;
#13300=ORIENTED_EDGE ( 'NONE', *, *, #27783, .F. ) ;
#13301=DIRECTION ( 'NONE',  ( 0.000000000000000000, 0.000000000000000000, 1.000000000000000000 ) ) ;
#13302=CARTESIAN_POINT ( 'NONE',  ( 62.99999662536839651, 60.62177826491078747, -9.999999999999998224 ) ) ;
#13303=FACE_OUTER_BOUND ( 'NONE', #9794, .T. ) ;
#13304=CARTESIAN_POINT ( 'NONE',  ( 14.99999662536863632, -77.94228634059960825, 12.50000000000000000 ) ) ;
#13305=ORIENTED_EDGE ( 'NONE', *, *, #21943, .F. ) ;
#13307=ADVANCED_FACE ( 'NONE', ( #191 ), #28712, .T. ) ;
#13312=AXIS2_PLACEMENT_3D ( 'NONE', #7525, #13511, #24612 ) ;
#13313=EDGE_CURVE ( 'NONE', #18465, #6603, #28515, .T. ) ;
#13315=ORIENTED_EDGE ( 'NONE', *, *, #23821, .F. ) ;
#13316=DIRECTION ( 'NONE',  ( -1.000000000000000000, 0.000000000000000000, 0.000000000000000000 ) ) ;
#13317=CARTESIAN_POINT ( 'NONE',  ( 52.99999662536844625, 43.30127018922198801, -9.999999999999998224 ) ) ;
#13319=ORIENTED_EDGE ( 'NONE', *, *, #24114, .T. ) ;
#13320=ORIENTED_EDGE ( 'NONE', *, *, #9854, .T. ) ;
#13321=VECTOR ( 'NONE', #34934, 1000.000000000000000 ) ;
#13322=EDGE_CURVE ( 'NONE', #14326, #26888, #34065, .T. ) ;
#13323=VERTEX_POINT ( 'NONE', #31163 ) ;
#13325=DIRECTION ( 'NONE',  ( 1.000000000000000000, 0.000000000000000000, 0.000000000000000000 ) ) ;
#13326=CARTESIAN_POINT ( 'NONE',  ( 71.99999662536839651, -17.32050807568879947, 12.50000000000000000 ) ) ;
#13327=PLANE ( 'NONE',  #22874 ) ;
#13330=DIRECTION ( 'NONE',  ( -1.000000000000000000, 0.000000000000000000, 0.000000000000000000 ) ) ;
#13331=CYLINDRICAL_SURFACE ( 'NONE', #15612, 2.000000000000000000 ) ;
#13332=CYLINDRICAL_SURFACE ( 'NONE', #2037, 2.000000000000001776 ) ;
#13334=AXIS2_PLACEMENT_3D ( 'NONE', #5689, #25774, #28367 ) ;
#13338=ORIENTED_EDGE ( 'NONE', *, *, #20789, .T. ) ;
#13339=ORIENTED_EDGE ( 'NONE', *, *, #18244, .T. ) ;
#13343=ORIENTED_EDGE ( 'NONE', *, *, #27036, .T. ) ;
#13344=VERTEX_POINT ( 'NONE', #5847 ) ;
#13346=ADVANCED_FACE ( 'NONE', ( #25731 ), #29058, .F. ) ;
#13347=DIRECTION ( 'NONE',  ( 1.000000000000000000, 0.000000000000000000, -0.000000000000000000 ) ) ;
#13348=ADVANCED_FACE ( 'NONE', ( #14629 ), #20275, .F. ) ;
#13350=ADVANCED_FACE ( 'NONE', ( #6034 ), #25532, .F. ) ;
#13352=VERTEX_POINT ( 'NONE', #22530 ) ;
#13353=EDGE_LOOP ( 'NONE', ( #25939, #19367, #9808, #13067 ) ) ;
#13354=DIRECTION ( 'NONE',  ( -1.000000000000000000, 0.000000000000000000, 0.000000000000000000 ) ) ;
#13355=AXIS2_PLACEMENT_3D ( 'NONE', #35622, #27359, #1300 ) ;
#13356=DIRECTION ( 'NONE',  ( 0.000000000000000000, 0.000000000000000000, 1.000000000000000000 ) ) ;
#13359=FACE_OUTER_BOUND ( 'NONE', #20006, .T. ) ;
#13360=DIRECTION ( 'NONE',  ( 0.000000000000000000, 0.000000000000000000, 1.000000000000000000 ) ) ;
#13362=CARTESIAN_POINT ( 'NONE',  ( 59.99999662536842493, -51.96152422706639840, -9.999999999999998224 ) ) ;
#13363=ORIENTED_EDGE ( 'NONE', *, *, #32475, .T. ) ;
#13364=CARTESIAN_POINT ( 'NONE',  ( -40.00000337463113453, 69.28203230275516944, 17.49999999999999645 ) ) ;
#13365=FACE_BOUND ( 'NONE', #17699, .T. ) ;
#13366=CARTESIAN_POINT ( 'NONE',  ( 4.999996625368645198, 77.94228634059957983, 17.49999999999999645 ) ) ;
#13368=CARTESIAN_POINT ( 'NONE',  ( -45.00000000000000711, 5.510910596163090344E-15, -10.00000000000000000 ) ) ;
#13369=CARTESIAN_POINT ( 'NONE',  ( 79.99999662536833966, 17.32050807568879236, 17.49999999999999645 ) ) ;
#13370=ADVANCED_FACE ( 'NONE', ( #26076 ), #31862, .F. ) ;
#13371=DIRECTION ( 'NONE',  ( 0.000000000000000000, 0.000000000000000000, 1.000000000000000000 ) ) ;
#13372=AXIS2_PLACEMENT_3D ( 'NONE', #7451, #24144, #10094 ) ;
#13375=ORIENTED_EDGE ( 'NONE', *, *, #25915, .F. ) ;
#13376=CARTESIAN_POINT ( 'NONE',  ( -63.00000337463102085, 43.30127018922198801, 17.49999999999999645 ) ) ;
#13377=CARTESIAN_POINT ( 'NONE',  ( 59.99999662536845335, 34.64101615137759893, 17.49999999999999645 ) ) ;
#13380=EDGE_LOOP ( 'NONE', ( #9290, #8793, #6449, #12538 ) ) ;
#13381=ORIENTED_EDGE ( 'NONE', *, *, #18888, .T. ) ;
#13382=ORIENTED_EDGE ( 'NONE', *, *, #1848, .T. ) ;
#13383=CIRCLE ( 'NONE', #20544, 2.000000000000001776 ) ;
#13384=DIRECTION ( 'NONE',  ( 1.000000000000000000, 0.000000000000000000, 0.000000000000000000 ) ) ;
#13385=DIRECTION ( 'NONE',  ( 1.000000000000000000, 0.000000000000000000, 0.000000000000000000 ) ) ;
#13386=ORIENTED_EDGE ( 'NONE', *, *, #1476, .T. ) ;
#13389=CARTESIAN_POINT ( 'NONE',  ( 24.99999662536857059, 77.94228634059957983, 17.49999999999999645 ) ) ;
#13390=CARTESIAN_POINT ( 'NONE',  ( -73.00000337463097821, 43.30127018922197379, 12.50000000000000000 ) ) ;
#13391=ORIENTED_EDGE ( 'NONE', *, *, #25173, .T. ) ;
#13393=CARTESIAN_POINT ( 'NONE',  ( -25.00000337463120914, 77.94228634059957983, -9.999999999999998224 ) ) ;
#13394=EDGE_LOOP ( 'NONE', ( #555, #17418 ) ) ;
#13395=FACE_BOUND ( 'NONE', #8553, .T. ) ;
#13397=DIRECTION ( 'NONE',  ( 1.000000000000000000, 0.000000000000000000, 0.000000000000000000 ) ) ;
#13398=DIRECTION ( 'NONE',  ( 0.000000000000000000, 0.000000000000000000, 1.000000000000000000 ) ) ;
#13399=DIRECTION ( 'NONE',  ( -1.000000000000000000, 0.000000000000000000, 0.000000000000000000 ) ) ;
#13400=ORIENTED_EDGE ( 'NONE', *, *, #20660, .T. ) ;
#13401=DIRECTION ( 'NONE',  ( 1.000000000000000000, 0.000000000000000000, 0.000000000000000000 ) ) ;
#13402=CIRCLE ( 'NONE', #2653, 2.000000000000000000 ) ;
#13403=CARTESIAN_POINT ( 'NONE',  ( -20.00000337463124112, 69.28203230275516944, -9.999999999999998224 ) ) ;
#13404=DIRECTION ( 'NONE',  ( 0.000000000000000000, 0.000000000000000000, 1.000000000000000000 ) ) ;
#13406=CARTESIAN_POINT ( 'NONE',  ( 39.99999662536853151, 69.28203230275518365, -5.000000000000000000 ) ) ;
#13407=DIRECTION ( 'NONE',  ( 0.000000000000000000, 0.000000000000000000, 1.000000000000000000 ) ) ;
#13409=DIRECTION ( 'NONE',  ( 0.000000000000000000, 0.000000000000000000, -1.000000000000000000 ) ) ;
#13410=DIRECTION ( 'NONE',  ( 1.000000000000000000, 0.000000000000000000, 0.000000000000000000 ) ) ;
#13411=DIRECTION ( 'NONE',  ( 0.000000000000000000, 0.000000000000000000, 1.000000000000000000 ) ) ;
#13412=ADVANCED_FACE ( 'NONE', ( #35078 ), #34895, .F. ) ;
#13413=ORIENTED_EDGE ( 'NONE', *, *, #21563, .T. ) ;
#13414=EDGE_LOOP ( 'NONE', ( #18994, #32798 ) ) ;
#13415=EDGE_CURVE ( 'NONE', #875, #18552, #22676, .T. ) ;
#13417=CARTESIAN_POINT ( 'NONE',  ( -4.279621169095561228, 62.97617850287782915, -4.999999999999997335 ) ) ;
#13418=AXIS2_PLACEMENT_3D ( 'NONE', #32352, #6838, #12464 ) ;
#13419=CARTESIAN_POINT ( 'NONE',  ( -30.00000337463118427, 69.28203230275516944, 12.50000000000000000 ) ) ;
#13421=ORIENTED_EDGE ( 'NONE', *, *, #34300, .F. ) ;
#13422=EDGE_LOOP ( 'NONE', ( #22031, #12142, #26094, #25959 ) ) ;
#13423=DIRECTION ( 'NONE',  ( 0.000000000000000000, 0.000000000000000000, 1.000000000000000000 ) ) ;
#13424=CYLINDRICAL_SURFACE ( 'NONE', #6473, 65.00000000000000000 ) ;
#13425=DIRECTION ( 'NONE',  ( 1.000000000000000000, 0.000000000000000000, 0.000000000000000000 ) ) ;
#13426=DIRECTION ( 'NONE',  ( 0.000000000000000000, 0.000000000000000000, 1.000000000000000000 ) ) ;
#13427=VERTEX_POINT ( 'NONE', #32255 ) ;
#13428=AXIS2_PLACEMENT_3D ( 'NONE', #3555, #29578, #12133 ) ;
#13429=CIRCLE ( 'NONE', #260, 2.000000000000001776 ) ;
#13432=AXIS2_PLACEMENT_3D ( 'NONE', #15932, #27721, #16477 ) ;
#13433=DIRECTION ( 'NONE',  ( -0.000000000000000000, -0.000000000000000000, 1.000000000000000000 ) ) ;
#13434=ORIENTED_EDGE ( 'NONE', *, *, #36596, .F. ) ;
#13435=EDGE_CURVE ( 'NONE', #7613, #14564, #10101, .T. ) ;
#13436=CARTESIAN_POINT ( 'NONE',  ( -19.13981058454750794, 60.93295298010998806, 12.49999999999999822 ) ) ;
#13437=VERTEX_POINT ( 'NONE', #4323 ) ;
#13440=CIRCLE ( 'NONE', #24841, 2.000000000000001776 ) ;
#13441=AXIS2_PLACEMENT_3D ( 'NONE', #12145, #23054, #29237 ) ;
#13442=CYLINDRICAL_SURFACE ( 'NONE', #28445, 2.000000000000001776 ) ;
#13443=EDGE_LOOP ( 'NONE', ( #4267, #27642 ) ) ;
#13445=VECTOR ( 'NONE', #29612, 1000.000000000000000 ) ;
#13446=CARTESIAN_POINT ( 'NONE',  ( 19.99999662536858835, 69.28203230275516944, 17.49999999999999645 ) ) ;
#13447=FACE_OUTER_BOUND ( 'NONE', #9727, .T. ) ;
#13449=ADVANCED_FACE ( 'NONE', ( #35286 ), #12734, .F. ) ;
#13451=CARTESIAN_POINT ( 'NONE',  ( -52.39915983220772233, -35.19434990244957362, 12.49999999999999822 ) ) ;
#13452=DIRECTION ( 'NONE',  ( 0.000000000000000000, 0.000000000000000000, 1.000000000000000000 ) ) ;
#13453=DIRECTION ( 'NONE',  ( 1.000000000000000000, 0.000000000000000000, 0.000000000000000000 ) ) ;
#13454=ORIENTED_EDGE ( 'NONE', *, *, #5438, .F. ) ;
#13455=AXIS2_PLACEMENT_3D ( 'NONE', #17946, #32174, #31796 ) ;
#13457=VECTOR ( 'NONE', #28936, 1000.000000000000000 ) ;
#13458=EDGE_LOOP ( 'NONE', ( #20531, #29676, #24537, #22161, #9235 ) ) ;
#13459=AXIS2_PLACEMENT_3D ( 'NONE', #14730, #484, #7827 ) ;
#13460=ORIENTED_EDGE ( 'NONE', *, *, #238, .F. ) ;
#13461=CARTESIAN_POINT ( 'NONE',  ( 47.99999662536848177, -51.96152422706640550, -9.999999999999998224 ) ) ;
#13463=ORIENTED_EDGE ( 'NONE', *, *, #15761, .F. ) ;
#13464=EDGE_CURVE ( 'NONE', #3339, #14569, #29438, .T. ) ;
#13466=CARTESIAN_POINT ( 'NONE',  ( -10.00000337463128197, 86.60254037844397601, -9.999999999999998224 ) ) ;
#13467=CARTESIAN_POINT ( 'NONE',  ( -45.00000337463111322, -77.94228634059960825, -9.999999999999998224 ) ) ;
#13468=EDGE_CURVE ( 'NONE', #14001, #27785, #34144, .T. ) ;
#13470=DIRECTION ( 'NONE',  ( 0.000000000000000000, 0.000000000000000000, 1.000000000000000000 ) ) ;
#13471=CYLINDRICAL_SURFACE ( 'NONE', #32354, 2.000000000000001776 ) ;
#13472=AXIS2_PLACEMENT_3D ( 'NONE', #7026, #1386, #36265 ) ;
#13473=CARTESIAN_POINT ( 'NONE',  ( 32.99999662536855283, -60.62177826491080168, -9.999999999999998224 ) ) ;
#13474=CYLINDRICAL_SURFACE ( 'NONE', #10660, 2.000000000000001776 ) ;
#13475=AXIS2_PLACEMENT_3D ( 'NONE', #26179, #113, #22826 ) ;
#13477=AXIS2_PLACEMENT_3D ( 'NONE', #2604, #34479, #31653 ) ;
#13479=DIRECTION ( 'NONE',  ( 0.000000000000000000, 0.000000000000000000, -1.000000000000000000 ) ) ;
#13480=DIRECTION ( 'NONE',  ( -0.000000000000000000, -0.000000000000000000, 1.000000000000000000 ) ) ;
#13481=DIRECTION ( 'NONE',  ( 1.000000000000000000, 0.000000000000000000, 0.000000000000000000 ) ) ;
#13482=DIRECTION ( 'NONE',  ( 0.000000000000000000, 0.000000000000000000, -1.000000000000000000 ) ) ;
#13483=EDGE_LOOP ( 'NONE', ( #3153, #22700 ) ) ;
#13484=CIRCLE ( 'NONE', #8117, 2.000000000000001776 ) ;
#13486=CARTESIAN_POINT ( 'NONE',  ( -62.00000337463107769, -34.64101615137762025, -5.000000000000000000 ) ) ;
#13487=EDGE_CURVE ( 'NONE', #23506, #22424, #23886, .T. ) ;
#13488=DIRECTION ( 'NONE',  ( 1.000000000000000000, 0.000000000000000000, 0.000000000000000000 ) ) ;
#13489=VERTEX_POINT ( 'NONE', #18588 ) ;
#13490=DIRECTION ( 'NONE',  ( 1.000000000000000000, 0.000000000000000000, 0.000000000000000000 ) ) ;
#13493=DIRECTION ( 'NONE',  ( 0.000000000000000000, 0.000000000000000000, -1.000000000000000000 ) ) ;
#13497=LINE ( 'NONE', #22148, #29256 ) ;
#13500=AXIS2_PLACEMENT_3D ( 'NONE', #35113, #12396, #222 ) ;
#13501=ORIENTED_EDGE ( 'NONE', *, *, #36200, .F. ) ;
#13502=ADVANCED_FACE ( 'NONE', ( #21188 ), #17825, .F. ) ;
#13503=VECTOR ( 'NONE', #15525, 1000.000000000000000 ) ;
#13504=AXIS2_PLACEMENT_3D ( 'NONE', #30607, #27782, #16190 ) ;
#13505=CIRCLE ( 'NONE', #8752, 2.000000000000001776 ) ;
#13506=AXIS2_PLACEMENT_3D ( 'NONE', #30323, #4843, #15707 ) ;
#13507=ORIENTED_EDGE ( 'NONE', *, *, #26839, .T. ) ;
#13509=DIRECTION ( 'NONE',  ( -0.000000000000000000, -0.000000000000000000, 1.000000000000000000 ) ) ;
#13511=DIRECTION ( 'NONE',  ( 0.000000000000000000, 0.000000000000000000, 1.000000000000000000 ) ) ;
#13512=CYLINDRICAL_SURFACE ( 'NONE', #1564, 2.000000000000001776 ) ;
#13513=VERTEX_POINT ( 'NONE', #29259 ) ;
#13514=CARTESIAN_POINT ( 'NONE',  ( 24.99999662536859546, -77.94228634059960825, 12.50000000000000000 ) ) ;
#13515=AXIS2_PLACEMENT_3D ( 'NONE', #6199, #3046, #25898 ) ;
#13516=CYLINDRICAL_SURFACE ( 'NONE', #26369, 3.499999999999991562 ) ;
#13517=EDGE_CURVE ( 'NONE', #29590, #16919, #7712, .T. ) ;
#13520=CARTESIAN_POINT ( 'NONE',  ( -12.00000337463127842, -69.28203230275519786, -9.999999999999998224 ) ) ;
#13521=CARTESIAN_POINT ( 'NONE',  ( 43.00330684490809574, 60.50675687296563865, 12.50000000000000000 ) ) ;
#13522=ORIENTED_EDGE ( 'NONE', *, *, #28077, .F. ) ;
#13523=AXIS2_PLACEMENT_3D ( 'NONE', #15082, #12441, #11698 ) ;
#13525=DIRECTION ( 'NONE',  ( 0.000000000000000000, 0.000000000000000000, -1.000000000000000000 ) ) ;
#13526=FACE_OUTER_BOUND ( 'NONE', #31379, .T. ) ;
#13528=AXIS2_PLACEMENT_3D ( 'NONE', #12591, #29847, #30404 ) ;
#13529=DIRECTION ( 'NONE',  ( 0.000000000000000000, 0.000000000000000000, 1.000000000000000000 ) ) ;
#13533=VECTOR ( 'NONE', #9522, 1000.000000000000000 ) ;
#13534=AXIS2_PLACEMENT_3D ( 'NONE', #30258, #7400, #9830 ) ;
#13535=CARTESIAN_POINT ( 'NONE',  ( 64.99999662536842493, 43.30127018922200222, 17.49999999999999645 ) ) ;
#13536=CIRCLE ( 'NONE', #14127, 2.000000000000001776 ) ;
#13537=EDGE_CURVE ( 'NONE', #6894, #23662, #21471, .T. ) ;
#13538=ORIENTED_EDGE ( 'NONE', *, *, #34909, .T. ) ;
#13539=EDGE_CURVE ( 'NONE', #23807, #7638, #21550, .T. ) ;
#13540=FACE_BOUND ( 'NONE', #24597, .T. ) ;
#13541=VERTEX_POINT ( 'NONE', #19492 ) ;
#13542=EDGE_LOOP ( 'NONE', ( #18583, #8826, #3583, #1745 ) ) ;
#13543=AXIS2_PLACEMENT_3D ( 'NONE', #24112, #13038, #35559 ) ;
#13544=EDGE_CURVE ( 'NONE', #29981, #20212, #30733, .T. ) ;
#13545=CARTESIAN_POINT ( 'NONE',  ( -62.97617850287781494, -4.279621169095772615, -49.86561046011506448 ) ) ;
#13546=CYLINDRICAL_SURFACE ( 'NONE', #17830, 2.000000000000001776 ) ;
#13548=ORIENTED_EDGE ( 'NONE', *, *, #2508, .T. ) ;
#13549=EDGE_CURVE ( 'NONE', #35451, #20281, #17962, .T. ) ;
#13550=DIRECTION ( 'NONE',  ( 0.000000000000000000, 0.000000000000000000, 1.000000000000000000 ) ) ;
#13552=EDGE_CURVE ( 'NONE', #16108, #25244, #31049, .T. ) ;
#13553=AXIS2_PLACEMENT_3D ( 'NONE', #5128, #10926, #16567 ) ;
#13555=LINE ( 'NONE', #18646, #13681 ) ;
#13557=ORIENTED_EDGE ( 'NONE', *, *, #11671, .F. ) ;
#13558=DIRECTION ( 'NONE',  ( 0.000000000000000000, 0.000000000000000000, 1.000000000000000000 ) ) ;
#13559=CARTESIAN_POINT ( 'NONE',  ( 72.99999662536836809, 43.30127018922198801, 12.50000000000000000 ) ) ;
#13561=DIRECTION ( 'NONE',  ( 1.000000000000000000, 0.000000000000000000, 0.000000000000000000 ) ) ;
#13562=DIRECTION ( 'NONE',  ( -0.000000000000000000, -0.000000000000000000, 1.000000000000000000 ) ) ;
#13563=AXIS2_PLACEMENT_3D ( 'NONE', #10946, #22577, #25044 ) ;
#13564=DIRECTION ( 'NONE',  ( 1.000000000000000000, 0.000000000000000000, 0.000000000000000000 ) ) ;
#13565=ADVANCED_FACE ( 'NONE', ( #5053 ), #10310, .F. ) ;
#13566=CIRCLE ( 'NONE', #21974, 27.00000000000001421 ) ;
#13567=DIRECTION ( 'NONE',  ( 1.000000000000000000, 0.000000000000000000, 0.000000000000000000 ) ) ;
#13569=EDGE_CURVE ( 'NONE', #29323, #22235, #33176, .T. ) ;
#13570=AXIS2_PLACEMENT_3D ( 'NONE', #6869, #18310, #26558 ) ;
#13571=CARTESIAN_POINT ( 'NONE',  ( -2.000003374631327713, 86.60254037844397601, 12.50000000000000000 ) ) ;
#13573=EDGE_CURVE ( 'NONE', #25826, #29785, #5954, .T. ) ;
#13574=DIRECTION ( 'NONE',  ( 0.000000000000000000, 0.000000000000000000, 1.000000000000000000 ) ) ;
#13575=EDGE_LOOP ( 'NONE', ( #9278, #23778 ) ) ;
#13576=DIRECTION ( 'NONE',  ( 0.000000000000000000, 0.000000000000000000, 1.000000000000000000 ) ) ;
#13577=CARTESIAN_POINT ( 'NONE',  ( 24.99999662536859546, -77.94228634059960825, -5.000000000000000000 ) ) ;
#13578=FACE_OUTER_BOUND ( 'NONE', #240, .T. ) ;
#13579=ORIENTED_EDGE ( 'NONE', *, *, #35131, .T. ) ;
#13580=AXIS2_PLACEMENT_3D ( 'NONE', #10362, #23893, #27614 ) ;
#13581=VERTEX_POINT ( 'NONE', #5254 ) ;
#13583=DIRECTION ( 'NONE',  ( 0.000000000000000000, 0.000000000000000000, -1.000000000000000000 ) ) ;
#13584=CYLINDRICAL_SURFACE ( 'NONE', #10675, 2.000000000000001776 ) ;
#13585=ORIENTED_EDGE ( 'NONE', *, *, #15029, .T. ) ;
#13587=DIRECTION ( 'NONE',  ( -1.000000000000000000, 0.000000000000000000, 0.000000000000000000 ) ) ;
#13589=DIRECTION ( 'NONE',  ( 1.000000000000000000, 0.000000000000000000, 0.000000000000000000 ) ) ;
#13590=ORIENTED_EDGE ( 'NONE', *, *, #14301, .F. ) ;
#13593=ORIENTED_EDGE ( 'NONE', *, *, #34850, .T. ) ;
#13594=DIRECTION ( 'NONE',  ( 0.000000000000000000, 0.000000000000000000, 1.000000000000000000 ) ) ;
#13595=AXIS2_PLACEMENT_3D ( 'NONE', #18179, #29608, #3933 ) ;
#13597=CIRCLE ( 'NONE', #4643, 1.999999999999998224 ) ;
#13600=ORIENTED_EDGE ( 'NONE', *, *, #16938, .T. ) ;
#13602=AXIS2_PLACEMENT_3D ( 'NONE', #13809, #22412, #11162 ) ;
#13604=AXIS2_PLACEMENT_3D ( 'NONE', #26280, #28883, #23086 ) ;
#13605=CARTESIAN_POINT ( 'NONE',  ( 29.99999662536857770, -69.28203230275519786, -9.999999999999998224 ) ) ;
#13606=CYLINDRICAL_SURFACE ( 'NONE', #9172, 2.000000000000001776 ) ;
#13607=EDGE_LOOP ( 'NONE', ( #26239, #25579, #6391, #1149 ) ) ;
#13608=CYLINDRICAL_SURFACE ( 'NONE', #26355, 2.000000000000001776 ) ;
#13609=DIRECTION ( 'NONE',  ( 0.000000000000000000, 0.000000000000000000, 1.000000000000000000 ) ) ;
#13610=ORIENTED_EDGE ( 'NONE', *, *, #24087, .T. ) ;
#13613=CARTESIAN_POINT ( 'NONE',  ( 79.99999662536832545, -17.32050807568879591, -5.000000000000000000 ) ) ;
#13615=AXIS2_PLACEMENT_3D ( 'NONE', #14306, #34361, #8662 ) ;
#13616=EDGE_LOOP ( 'NONE', ( #293, #33439, #9571, #27153 ) ) ;
#13617=CIRCLE ( 'NONE', #19592, 2.000000000000001776 ) ;
#13618=EDGE_CURVE ( 'NONE', #10634, #16319, #25103, .T. ) ;
#13619=ORIENTED_EDGE ( 'NONE', *, *, #13569, .T. ) ;
#13620=DIRECTION ( 'NONE',  ( 1.000000000000000000, 0.000000000000000000, 0.000000000000000000 ) ) ;
#13621=DIRECTION ( 'NONE',  ( 1.000000000000000000, 0.000000000000000000, 0.000000000000000000 ) ) ;
#13623=CIRCLE ( 'NONE', #16628, 2.000000000000000000 ) ;
#13624=CARTESIAN_POINT ( 'NONE',  ( -58.00000337463104216, 34.64101615137757051, 12.50000000000000000 ) ) ;
#13625=AXIS2_PLACEMENT_3D ( 'NONE', #31382, #19409, #13795 ) ;
#13626=EDGE_LOOP ( 'NONE', ( #29394, #9488, #18398, #16280 ) ) ;
#13628=CARTESIAN_POINT ( 'NONE',  ( -55.88972745734155012, 34.00000000000049027, -49.22241343995295892 ) ) ;
#13630=CARTESIAN_POINT ( 'NONE',  ( -78.00000337463096400, -34.64101615137762025, 17.49999999999999645 ) ) ;
#13631=CARTESIAN_POINT ( 'NONE',  ( 69.99999662536841072, 51.96152422706640550, 12.50000000000000000 ) ) ;
#13632=VERTEX_POINT ( 'NONE', #36573 ) ;
#13633=ORIENTED_EDGE ( 'NONE', *, *, #4844, .F. ) ;
#13634=CARTESIAN_POINT ( 'NONE',  ( 64.99999662536839651, -43.30127018922199511, -5.000000000000000000 ) ) ;
#13635=CIRCLE ( 'NONE', #18434, 2.000000000000001776 ) ;
#13637=ORIENTED_EDGE ( 'NONE', *, *, #34904, .F. ) ;
#13638=FACE_OUTER_BOUND ( 'NONE', #8199, .T. ) ;
#13639=ORIENTED_EDGE ( 'NONE', *, *, #28441, .F. ) ;
#13640=AXIS2_PLACEMENT_3D ( 'NONE', #34809, #11371, #31412 ) ;
#13641=FACE_BOUND ( 'NONE', #12427, .T. ) ;
#13642=EDGE_CURVE ( 'NONE', #34086, #13708, #27734, .T. ) ;
#13644=CIRCLE ( 'NONE', #34000, 2.000000000000001776 ) ;
#13645=CIRCLE ( 'NONE', #1061, 27.00000000000001066 ) ;
#13646=CARTESIAN_POINT ( 'NONE',  ( -85.00000337463092137, 25.98076211353317433, -5.000000000000000000 ) ) ;
#13648=CARTESIAN_POINT ( 'NONE',  ( -3.374631289687624047E-06, -69.28203230275519786, -5.000000000000000000 ) ) ;
#13649=ORIENTED_EDGE ( 'NONE', *, *, #2544, .T. ) ;
#13651=DIRECTION ( 'NONE',  ( 0.000000000000000000, 0.000000000000000000, 1.000000000000000000 ) ) ;
#13653=EDGE_CURVE ( 'NONE', #36171, #19268, #22307, .T. ) ;
#13654=CYLINDRICAL_SURFACE ( 'NONE', #10785, 2.000000000000000000 ) ;
#13655=DIRECTION ( 'NONE',  ( 0.000000000000000000, 0.000000000000000000, -1.000000000000000000 ) ) ;
#13657=DIRECTION ( 'NONE',  ( 1.000000000000000000, 0.000000000000000000, 0.000000000000000000 ) ) ;
#13658=LINE ( 'NONE', #31442, #17810 ) ;
#13659=AXIS2_PLACEMENT_3D ( 'NONE', #33508, #11353, #14161 ) ;
#13660=CYLINDRICAL_SURFACE ( 'NONE', #22538, 2.000000000000001776 ) ;
#13661=ORIENTED_EDGE ( 'NONE', *, *, #6407, .F. ) ;
#13662=ORIENTED_EDGE ( 'NONE', *, *, #20660, .F. ) ;
#13663=AXIS2_PLACEMENT_3D ( 'NONE', #29076, #14476, #28889 ) ;
#13664=EDGE_CURVE ( 'NONE', #16153, #20325, #25703, .T. ) ;
#13665=FACE_OUTER_BOUND ( 'NONE', #3117, .T. ) ;
#13666=EDGE_LOOP ( 'NONE', ( #1289, #83, #18521, #892 ) ) ;
#13667=CIRCLE ( 'NONE', #34637, 2.000000000000000000 ) ;
#13668=AXIS2_PLACEMENT_3D ( 'NONE', #17804, #20993, #35267 ) ;
#13669=DIRECTION ( 'NONE',  ( 0.000000000000000000, 0.000000000000000000, -1.000000000000000000 ) ) ;
#13671=AXIS2_PLACEMENT_3D ( 'NONE', #14207, #25285, #25663 ) ;
#13672=CARTESIAN_POINT ( 'NONE',  ( -35.19434990244938888, 52.39915983220783602, 12.49999999999999822 ) ) ;
#13673=CIRCLE ( 'NONE', #19067, 2.000000000000001776 ) ;
#13674=DIRECTION ( 'NONE',  ( 0.000000000000000000, 0.000000000000000000, 1.000000000000000000 ) ) ;
#13676=DIRECTION ( 'NONE',  ( -1.000000000000000000, 0.000000000000000000, 0.000000000000000000 ) ) ;
#13677=LINE ( 'NONE', #25476, #27381 ) ;
#13678=CARTESIAN_POINT ( 'NONE',  ( 82.99999662536831124, -25.98076211353319565, -9.999999999999998224 ) ) ;
#13679=ORIENTED_EDGE ( 'NONE', *, *, #16952, .T. ) ;
#13680=VERTEX_POINT ( 'NONE', #27573 ) ;
#13681=VECTOR ( 'NONE', #27996, 1000.000000000000000 ) ;
#13682=DIRECTION ( 'NONE',  ( 0.000000000000000000, 0.000000000000000000, 1.000000000000000000 ) ) ;
#13683=EDGE_CURVE ( 'NONE', #18775, #23924, #14911, .T. ) ;
#13684=DIRECTION ( 'NONE',  ( -0.000000000000000000, -0.000000000000000000, -1.000000000000000000 ) ) ;
#13685=DIRECTION ( 'NONE',  ( 0.000000000000000000, 0.000000000000000000, -1.000000000000000000 ) ) ;
#13686=CARTESIAN_POINT ( 'NONE',  ( 52.39915983220795681, 35.19434990244919703, 12.49999999999999822 ) ) ;
#13689=FACE_OUTER_BOUND ( 'NONE', #9245, .T. ) ;
#13690=CIRCLE ( 'NONE', #34099, 2.000000000000001776 ) ;
#13692=ORIENTED_EDGE ( 'NONE', *, *, #29414, .F. ) ;
#13693=EDGE_CURVE ( 'NONE', #5473, #28380, #18756, .T. ) ;
#13695=CARTESIAN_POINT ( 'NONE',  ( -48.00000337463109190, 51.96152422706637708, -9.999999999999998224 ) ) ;
#13696=ORIENTED_EDGE ( 'NONE', *, *, #28820, .F. ) ;
#13697=CARTESIAN_POINT ( 'NONE',  ( -55.00000337463109901, -60.62177826491083010, -9.999999999999998224 ) ) ;
#13698=FACE_OUTER_BOUND ( 'NONE', #31335, .T. ) ;
#13699=EDGE_CURVE ( 'NONE', #1955, #4119, #4505, .T. ) ;
#13700=CIRCLE ( 'NONE', #35262, 2.000000000000000000 ) ;
#13702=CIRCLE ( 'NONE', #7120, 1.999999999999998224 ) ;
#13703=VERTEX_POINT ( 'NONE', #1698 ) ;
#13704=ORIENTED_EDGE ( 'NONE', *, *, #3656, .T. ) ;
#13705=AXIS2_PLACEMENT_3D ( 'NONE', #36018, #10493, #4706 ) ;
#13706=ORIENTED_EDGE ( 'NONE', *, *, #15550, .F. ) ;
#13707=AXIS2_PLACEMENT_3D ( 'NONE', #31882, #26648, #3224 ) ;
#13708=VERTEX_POINT ( 'NONE', #1878 ) ;
#13711=DIRECTION ( 'NONE',  ( -1.000000000000000000, 0.000000000000000000, -0.000000000000000000 ) ) ;
#13712=DIRECTION ( 'NONE',  ( 1.000000000000000000, 0.000000000000000000, 0.000000000000000000 ) ) ;
#13715=DIRECTION ( 'NONE',  ( 1.000000000000000000, 0.000000000000000000, 0.000000000000000000 ) ) ;
#13716=EDGE_CURVE ( 'NONE', #29194, #10781, #36189, .T. ) ;
#13717=DIRECTION ( 'NONE',  ( 1.000000000000000000, 0.000000000000000000, 0.000000000000000000 ) ) ;
#13719=EDGE_LOOP ( 'NONE', ( #766, #14479 ) ) ;
#13720=CARTESIAN_POINT ( 'NONE',  ( -20.39230267490738768, 84.64139243425341874, 12.50000000000000000 ) ) ;
#13721=AXIS2_PLACEMENT_3D ( 'NONE', #22001, #13550, #27794 ) ;
#13722=LINE ( 'NONE', #27769, #16575 ) ;
#13723=ORIENTED_EDGE ( 'NONE', *, *, #934, .F. ) ;
#13724=ADVANCED_FACE ( 'NONE', ( #19147 ), #36924, .F. ) ;
#13725=ORIENTED_EDGE ( 'NONE', *, *, #31656, .T. ) ;
#13726=DIRECTION ( 'NONE',  ( 0.000000000000000000, 0.000000000000000000, -1.000000000000000000 ) ) ;
#13728=ADVANCED_FACE ( 'NONE', ( #22482 ), #13862, .F. ) ;
#13729=DIRECTION ( 'NONE',  ( 0.000000000000000000, 0.000000000000000000, 1.000000000000000000 ) ) ;
#13730=CARTESIAN_POINT ( 'NONE',  ( -62.00000337463108480, -51.96152422706641971, -5.000000000000000000 ) ) ;
#13733=ORIENTED_EDGE ( 'NONE', *, *, #37075, .T. ) ;
#13734=VECTOR ( 'NONE', #16643, 1000.000000000000000 ) ;
#13735=CARTESIAN_POINT ( 'NONE',  ( -68.00000000000000000, 0.000000000000000000, 12.49999999999999822 ) ) ;
#13736=AXIS2_PLACEMENT_3D ( 'NONE', #6898, #18342, #15539 ) ;
#13738=AXIS2_PLACEMENT_3D ( 'NONE', #24088, #7027, #35717 ) ;
#13739=PLANE ( 'NONE',  #8208 ) ;
#13740=ORIENTED_EDGE ( 'NONE', *, *, #20793, .F. ) ;
#13742=AXIS2_PLACEMENT_3D ( 'NONE', #10156, #9952, #2056 ) ;
#13743=DIRECTION ( 'NONE',  ( 1.000000000000000000, 0.000000000000000000, 0.000000000000000000 ) ) ;
#13744=EDGE_CURVE ( 'NONE', #14529, #26415, #20286, .T. ) ;
#13745=CIRCLE ( 'NONE', #37091, 2.000000000000001776 ) ;
#13746=PLANE ( 'NONE',  #1704 ) ;
#13748=ORIENTED_EDGE ( 'NONE', *, *, #1892, .F. ) ;
#13750=CIRCLE ( 'NONE', #4796, 3.000000000000004885 ) ;
#13751=DIRECTION ( 'NONE',  ( 1.000000000000000000, 0.000000000000000000, 0.000000000000000000 ) ) ;
#13752=LINE ( 'NONE', #4936, #10292 ) ;
#13753=FACE_OUTER_BOUND ( 'NONE', #4093, .T. ) ;
#13754=VERTEX_POINT ( 'NONE', #31821 ) ;
#13757=FACE_BOUND ( 'NONE', #20776, .T. ) ;
#13758=CYLINDRICAL_SURFACE ( 'NONE', #4031, 2.000000000000001776 ) ;
#13759=FACE_OUTER_BOUND ( 'NONE', #19125, .T. ) ;
#13760=DIRECTION ( 'NONE',  ( 1.000000000000000000, 0.000000000000000000, 0.000000000000000000 ) ) ;
#13761=AXIS2_PLACEMENT_3D ( 'NONE', #33839, #31375, #8520 ) ;
#13762=DIRECTION ( 'NONE',  ( 0.000000000000000000, 0.000000000000000000, 1.000000000000000000 ) ) ;
#13765=CARTESIAN_POINT ( 'NONE',  ( -2.000003374631327713, 86.60254037844397601, -9.999999999999998224 ) ) ;
#13767=CARTESIAN_POINT ( 'NONE',  ( 67.99999662536838230, 34.64101615137758472, -9.999999999999998224 ) ) ;
#13768=VERTEX_POINT ( 'NONE', #28470 ) ;
#13770=FACE_OUTER_BOUND ( 'NONE', #10391, .T. ) ;
#13771=CARTESIAN_POINT ( 'NONE',  ( -70.00000337463099243, 17.32050807568877460, -5.000000000000000000 ) ) ;
#13772=AXIS2_PLACEMENT_3D ( 'NONE', #22510, #27592, #7523 ) ;
#13773=DIRECTION ( 'NONE',  ( 1.000000000000000000, 0.000000000000000000, 0.000000000000000000 ) ) ;
#13774=ORIENTED_EDGE ( 'NONE', *, *, #24031, .T. ) ;
#13775=ADVANCED_FACE ( 'NONE', ( #25308 ), #31462, .F. ) ;
#13776=EDGE_LOOP ( 'NONE', ( #29999, #8417 ) ) ;
#13778=AXIS2_PLACEMENT_3D ( 'NONE', #35363, #32129, #29331 ) ;
#13779=DIRECTION ( 'NONE',  ( -1.000000000000000000, 0.000000000000000000, -0.000000000000000000 ) ) ;
#13781=EDGE_CURVE ( 'NONE', #10047, #25550, #29867, .T. ) ;
#13783=VERTEX_POINT ( 'NONE', #28665 ) ;
#13784=ADVANCED_FACE ( 'NONE', ( #3158 ), #28288, .F. ) ;
#13785=DIRECTION ( 'NONE',  ( -1.000000000000000000, 0.000000000000000000, 0.000000000000000000 ) ) ;
#13788=DIRECTION ( 'NONE',  ( 1.000000000000000000, 0.000000000000000000, 0.000000000000000000 ) ) ;
#13789=ORIENTED_EDGE ( 'NONE', *, *, #1519, .T. ) ;
#13790=CARTESIAN_POINT ( 'NONE',  ( -87.83969979969872099, -14.80603122773087499, 12.49999999999999645 ) ) ;
#13791=AXIS2_PLACEMENT_3D ( 'NONE', #30182, #5060, #16697 ) ;
#13792=EDGE_CURVE ( 'NONE', #8784, #29817, #10127, .T. ) ;
#13793=EDGE_CURVE ( 'NONE', #32680, #28932, #8339, .T. ) ;
#13795=DIRECTION ( 'NONE',  ( 1.000000000000000000, 0.000000000000000000, 0.000000000000000000 ) ) ;
#13797=EDGE_CURVE ( 'NONE', #28577, #167, #528, .T. ) ;
#13798=AXIS2_PLACEMENT_3D ( 'NONE', #3380, #2839, #8628 ) ;
#13799=EDGE_CURVE ( 'NONE', #14564, #11272, #32266, .T. ) ;
#13800=VERTEX_POINT ( 'NONE', #11769 ) ;
#13802=AXIS2_PLACEMENT_3D ( 'NONE', #32988, #10123, #15558 ) ;
#13803=DIRECTION ( 'NONE',  ( 0.000000000000000000, 0.000000000000000000, 1.000000000000000000 ) ) ;
#13805=ORIENTED_EDGE ( 'NONE', *, *, #11225, .F. ) ;
#13806=CARTESIAN_POINT ( 'NONE',  ( 49.99999662536848177, -51.96152422706640550, 12.50000000000000000 ) ) ;
#13807=DIRECTION ( 'NONE',  ( 1.000000000000000000, 0.000000000000000000, 0.000000000000000000 ) ) ;
#13808=ORIENTED_EDGE ( 'NONE', *, *, #4159, .F. ) ;
#13809=CARTESIAN_POINT ( 'NONE',  ( -80.00000337463094979, -17.32050807568882078, -5.000000000000000000 ) ) ;
#13810=DIRECTION ( 'NONE',  ( -0.4999999999999979461, 0.8660254037844397068, 0.000000000000000000 ) ) ;
#13811=PLANE ( 'NONE',  #31516 ) ;
#13812=CARTESIAN_POINT ( 'NONE',  ( 79.99999662536833966, 34.64101615137759183, -5.000000000000000000 ) ) ;
#13813=ORIENTED_EDGE ( 'NONE', *, *, #11225, .T. ) ;
#13814=ORIENTED_EDGE ( 'NONE', *, *, #17665, .T. ) ;
#13816=CARTESIAN_POINT ( 'NONE',  ( -66.86787810013036903, 2.778182860042780700, 12.49999999999999645 ) ) ;
#13817=ORIENTED_EDGE ( 'NONE', *, *, #33196, .F. ) ;
#13819=CIRCLE ( 'NONE', #23403, 3.000000000000002665 ) ;
#13820=CARTESIAN_POINT ( 'NONE',  ( 36.99999662536853862, 77.94228634059959404, -9.999999999999998224 ) ) ;
#13821=DIRECTION ( 'NONE',  ( 0.000000000000000000, 0.000000000000000000, 1.000000000000000000 ) ) ;
#13822=DIRECTION ( 'NONE',  ( 0.000000000000000000, 0.000000000000000000, -1.000000000000000000 ) ) ;
#13823=ORIENTED_EDGE ( 'NONE', *, *, #27551, .F. ) ;
#13824=ORIENTED_EDGE ( 'NONE', *, *, #607, .F. ) ;
#13825=FACE_OUTER_BOUND ( 'NONE', #35146, .T. ) ;
#13826=VERTEX_POINT ( 'NONE', #8432 ) ;
#13827=LINE ( 'NONE', #36698, #1772 ) ;
#13828=ORIENTED_EDGE ( 'NONE', *, *, #20870, .F. ) ;
#13829=FACE_BOUND ( 'NONE', #5903, .T. ) ;
#13830=EDGE_CURVE ( 'NONE', #27851, #34166, #334, .T. ) ;
#13831=DIRECTION ( 'NONE',  ( 0.000000000000000000, 0.000000000000000000, 1.000000000000000000 ) ) ;
#13833=EDGE_LOOP ( 'NONE', ( #8270, #13704 ) ) ;
#13835=LINE ( 'NONE', #16655, #878 ) ;
#13836=FACE_OUTER_BOUND ( 'NONE', #10597, .T. ) ;
#13838=AXIS2_PLACEMENT_3D ( 'NONE', #29749, #20756, #24137 ) ;
#13840=DIRECTION ( 'NONE',  ( 1.000000000000000000, 0.000000000000000000, 0.000000000000000000 ) ) ;
#13841=DIRECTION ( 'NONE',  ( 0.000000000000000000, 0.000000000000000000, -1.000000000000000000 ) ) ;
#13843=VERTEX_POINT ( 'NONE', #31657 ) ;
#13845=ORIENTED_EDGE ( 'NONE', *, *, #7980, .F. ) ;
#13846=DIRECTION ( 'NONE',  ( 0.000000000000000000, 0.000000000000000000, -1.000000000000000000 ) ) ;
#13847=CARTESIAN_POINT ( 'NONE',  ( 4.279621169095998212, -62.97617850287780072, 12.49999999999999822 ) ) ;
#13848=EDGE_CURVE ( 'NONE', #21808, #2177, #14324, .T. ) ;
#13849=CARTESIAN_POINT ( 'NONE',  ( 69.99999662536839651, -17.32050807568879947, -5.000000000000000000 ) ) ;
#13850=DIRECTION ( 'NONE',  ( -0.000000000000000000, -0.000000000000000000, 1.000000000000000000 ) ) ;
#13851=FACE_OUTER_BOUND ( 'NONE', #35138, .T. ) ;
#13852=LINE ( 'NONE', #7686, #4829 ) ;
#13853=VECTOR ( 'NONE', #16691, 1000.000000000000000 ) ;
#13856=ORIENTED_EDGE ( 'NONE', *, *, #32785, .T. ) ;
#13858=EDGE_CURVE ( 'NONE', #13783, #28708, #10712, .T. ) ;
#13859=CARTESIAN_POINT ( 'NONE',  ( -65.00000337463102085, 43.30127018922198801, -9.999999999999998224 ) ) ;
#13860=CARTESIAN_POINT ( 'NONE',  ( -33.99999999999945288, 58.88972745734214698, 12.49999999999999822 ) ) ;
#13861=DIRECTION ( 'NONE',  ( 0.000000000000000000, 0.000000000000000000, 1.000000000000000000 ) ) ;
#13862=CYLINDRICAL_SURFACE ( 'NONE', #16711, 2.000000000000001776 ) ;
#13863=ORIENTED_EDGE ( 'NONE', *, *, #11445, .T. ) ;
#13865=ORIENTED_EDGE ( 'NONE', *, *, #28798, .F. ) ;
#13866=EDGE_LOOP ( 'NONE', ( #12092, #17520, #16801, #31332 ) ) ;
#13867=EDGE_CURVE ( 'NONE', #29077, #7029, #21498, .T. ) ;
#13868=CARTESIAN_POINT ( 'NONE',  ( 51.99999662536847467, -69.28203230275519786, -5.000000000000000000 ) ) ;
#13872=DIRECTION ( 'NONE',  ( 1.000000000000000000, 0.000000000000000000, 0.000000000000000000 ) ) ;
#13874=DIRECTION ( 'NONE',  ( 0.000000000000000000, 0.000000000000000000, 1.000000000000000000 ) ) ;
#13877=CIRCLE ( 'NONE', #4307, 2.000000000000001776 ) ;
#13878=VERTEX_POINT ( 'NONE', #32576 ) ;
#13879=ORIENTED_EDGE ( 'NONE', *, *, #20715, .T. ) ;
#13880=ORIENTED_EDGE ( 'NONE', *, *, #5589, .F. ) ;
#13882=EDGE_CURVE ( 'NONE', #13165, #23444, #34092, .T. ) ;
#13883=DIRECTION ( 'NONE',  ( 1.000000000000000000, 0.000000000000000000, 0.000000000000000000 ) ) ;
#13884=DIRECTION ( 'NONE',  ( 1.000000000000000000, 0.000000000000000000, 0.000000000000000000 ) ) ;
#13885=CARTESIAN_POINT ( 'NONE',  ( 4.999996625368645198, 77.94228634059957983, -9.999999999999998224 ) ) ;
#13887=ADVANCED_FACE ( 'NONE', ( #24146 ), #14780, .F. ) ;
#13888=ORIENTED_EDGE ( 'NONE', *, *, #35419, .F. ) ;
#13890=DIRECTION ( 'NONE',  ( 0.000000000000000000, 0.000000000000000000, 1.000000000000000000 ) ) ;
#13891=DIRECTION ( 'NONE',  ( 0.000000000000000000, 0.000000000000000000, 1.000000000000000000 ) ) ;
#13893=CARTESIAN_POINT ( 'NONE',  ( -80.00000337463094979, -17.32050807568882078, -9.999999999999998224 ) ) ;
#13894=ADVANCED_FACE ( 'NONE', ( #6893 ), #26777, .F. ) ;
#13897=EDGE_LOOP ( 'NONE', ( #645, #27989, #14427, #28761 ) ) ;
#13898=ADVANCED_FACE ( 'NONE', ( #29010 ), #35425, .F. ) ;
#13899=FACE_OUTER_BOUND ( 'NONE', #6190, .T. ) ;
#13900=AXIS2_PLACEMENT_3D ( 'NONE', #28357, #8498, #220 ) ;
#13901=DIRECTION ( 'NONE',  ( 0.000000000000000000, 0.000000000000000000, 1.000000000000000000 ) ) ;
#13902=CARTESIAN_POINT ( 'NONE',  ( -40.00000337463113453, 69.28203230275516944, -9.999999999999998224 ) ) ;
#13905=VERTEX_POINT ( 'NONE', #29762 ) ;
#13906=CARTESIAN_POINT ( 'NONE',  ( 17.99999662536861678, -69.28203230275519786, -9.999999999999998224 ) ) ;
#13908=EDGE_CURVE ( 'NONE', #6626, #26576, #4754, .T. ) ;
#13909=DIRECTION ( 'NONE',  ( -1.000000000000000000, 0.000000000000000000, -0.000000000000000000 ) ) ;
#13910=VERTEX_POINT ( 'NONE', #6335 ) ;
#13911=VERTEX_POINT ( 'NONE', #17583 ) ;
#13912=VECTOR ( 'NONE', #35298, 1000.000000000000000 ) ;
#13913=CIRCLE ( 'NONE', #23502, 95.00000000000001421 ) ;
#13915=CARTESIAN_POINT ( 'NONE',  ( -35.00000337463117717, -77.94228634059963667, -9.999999999999998224 ) ) ;
#13916=ORIENTED_EDGE ( 'NONE', *, *, #2064, .T. ) ;
#13918=LINE ( 'NONE', #10921, #8928 ) ;
#13919=DIRECTION ( 'NONE',  ( 1.000000000000000000, 0.000000000000000000, 0.000000000000000000 ) ) ;
#13921=CARTESIAN_POINT ( 'NONE',  ( -2.000003374631327713, 86.60254037844397601, -5.000000000000000000 ) ) ;
#13922=DIRECTION ( 'NONE',  ( 0.000000000000000000, 0.000000000000000000, 1.000000000000000000 ) ) ;
#13923=VERTEX_POINT ( 'NONE', #21331 ) ;
#13924=DIRECTION ( 'NONE',  ( -0.8660254037844449249, -0.4999999999999888978, 0.000000000000000000 ) ) ;
#13925=VECTOR ( 'NONE', #34322, 1000.000000000000000 ) ;
#13927=FACE_BOUND ( 'NONE', #25439, .T. ) ;
#13928=DIRECTION ( 'NONE',  ( 0.000000000000000000, 0.000000000000000000, -1.000000000000000000 ) ) ;
#13930=DIRECTION ( 'NONE',  ( -1.000000000000000000, 0.000000000000000000, 0.000000000000000000 ) ) ;
#13931=DIRECTION ( 'NONE',  ( 0.5000000000000038858, 0.8660254037844362651, 0.000000000000000000 ) ) ;
#13933=FACE_OUTER_BOUND ( 'NONE', #8651, .T. ) ;
#13934=ORIENTED_EDGE ( 'NONE', *, *, #10561, .F. ) ;
#13935=CARTESIAN_POINT ( 'NONE',  ( -32.00000337463118427, 69.28203230275516944, -5.000000000000000000 ) ) ;
#13936=ADVANCED_FACE ( 'NONE', ( #23417 ), #21146, .T. ) ;
#13938=FACE_OUTER_BOUND ( 'NONE', #33099, .T. ) ;
#13939=ORIENTED_EDGE ( 'NONE', *, *, #5109, .F. ) ;
#13940=VECTOR ( 'NONE', #16315, 1000.000000000000000 ) ;
#13941=ORIENTED_EDGE ( 'NONE', *, *, #18751, .T. ) ;
#13942=ORIENTED_EDGE ( 'NONE', *, *, #17790, .F. ) ;
#13943=ADVANCED_FACE ( 'NONE', ( #6539 ), #12121, .F. ) ;
#13945=CARTESIAN_POINT ( 'NONE',  ( 46.99999662536851019, 77.94228634059959404, -9.999999999999998224 ) ) ;
#13948=AXIS2_PLACEMENT_3D ( 'NONE', #1028, #3663, #15093 ) ;
#13949=ORIENTED_EDGE ( 'NONE', *, *, #31388, .T. ) ;
#13952=DIRECTION ( 'NONE',  ( -0.5000000000000101030, -0.8660254037844328234, 0.000000000000000000 ) ) ;
#13953=ORIENTED_EDGE ( 'NONE', *, *, #6102, .T. ) ;
#13954=EDGE_CURVE ( 'NONE', #29027, #4235, #32295, .T. ) ;
#13955=DIRECTION ( 'NONE',  ( -0.000000000000000000, 0.000000000000000000, -1.000000000000000000 ) ) ;
#13956=DIRECTION ( 'NONE',  ( 0.000000000000000000, 0.000000000000000000, 1.000000000000000000 ) ) ;
#13958=LINE ( 'NONE', #5368, #24893 ) ;
#13962=LINE ( 'NONE', #25410, #17688 ) ;
#13964=VERTEX_POINT ( 'NONE', #35784 ) ;
#13965=CARTESIAN_POINT ( 'NONE',  ( -25.00000337463121980, -77.94228634059963667, -9.999999999999998224 ) ) ;
#13966=LINE ( 'NONE', #10248, #14365 ) ;
#13967=EDGE_CURVE ( 'NONE', #27946, #25623, #36499, .T. ) ;
#13970=ADVANCED_FACE ( 'NONE', ( #29962 ), #21703, .F. ) ;
#13973=DIRECTION ( 'NONE',  ( 0.000000000000000000, 0.000000000000000000, -1.000000000000000000 ) ) ;
#13975=ORIENTED_EDGE ( 'NONE', *, *, #20335, .F. ) ;
#13976=CIRCLE ( 'NONE', #23559, 2.000000000000001776 ) ;
#13977=ORIENTED_EDGE ( 'NONE', *, *, #24622, .T. ) ;
#13979=CARTESIAN_POINT ( 'NONE',  ( -10.00000337463128730, 69.28203230275516944, -9.999999999999998224 ) ) ;
#13980=AXIS2_PLACEMENT_3D ( 'NONE', #31599, #34073, #19984 ) ;
#13981=VERTEX_POINT ( 'NONE', #36147 ) ;
#13983=ADVANCED_FACE ( 'NONE', ( #27692 ), #21886, .F. ) ;
#13984=CARTESIAN_POINT ( 'NONE',  ( -65.00000337463102085, 60.62177826491077326, 12.50000000000000000 ) ) ;
#13985=CARTESIAN_POINT ( 'NONE',  ( 54.99999662536846046, -43.30127018922200222, 12.50000000000000000 ) ) ;
#13986=DIRECTION ( 'NONE',  ( 0.000000000000000000, 0.000000000000000000, 1.000000000000000000 ) ) ;
#13987=AXIS2_PLACEMENT_3D ( 'NONE', #990, #6434, #18225 ) ;
#13988=ORIENTED_EDGE ( 'NONE', *, *, #24117, .F. ) ;
#13989=EDGE_LOOP ( 'NONE', ( #3173, #19328 ) ) ;
#13990=AXIS2_PLACEMENT_3D ( 'NONE', #32565, #6881, #1996 ) ;
#13991=DIRECTION ( 'NONE',  ( 0.000000000000000000, 0.000000000000000000, 1.000000000000000000 ) ) ;
#13992=CARTESIAN_POINT ( 'NONE',  ( -87.00000337463093558, 8.660254037844389075, -9.999999999999998224 ) ) ;
#13993=VERTEX_POINT ( 'NONE', #7649 ) ;
#13994=DIRECTION ( 'NONE',  ( 0.000000000000000000, 0.000000000000000000, 1.000000000000000000 ) ) ;
#13996=DIRECTION ( 'NONE',  ( 0.000000000000000000, 0.000000000000000000, 1.000000000000000000 ) ) ;
#13998=LINE ( 'NONE', #8398, #10743 ) ;
#14000=ADVANCED_FACE ( 'NONE', ( #10271 ), #33133, .F. ) ;
#14001=VERTEX_POINT ( 'NONE', #1839 ) ;
#14003=DIRECTION ( 'NONE',  ( -1.000000000000000000, 0.000000000000000000, 0.000000000000000000 ) ) ;
#14005=CARTESIAN_POINT ( 'NONE',  ( -3.499999999999991562, 55.00000000000000000, -5.000000000000000000 ) ) ;
#14006=ORIENTED_EDGE ( 'NONE', *, *, #8278, .F. ) ;
#14007=CARTESIAN_POINT ( 'NONE',  ( 49.99999662536846756, 51.96152422706637708, 12.50000000000000000 ) ) ;
#14008=ADVANCED_FACE ( 'NONE', ( #13638 ), #24897, .F. ) ;
#14010=DIRECTION ( 'NONE',  ( 0.000000000000000000, 0.000000000000000000, 1.000000000000000000 ) ) ;
#14011=ORIENTED_EDGE ( 'NONE', *, *, #30968, .T. ) ;
#14012=CIRCLE ( 'NONE', #34986, 2.000000000000001776 ) ;
#14013=EDGE_LOOP ( 'NONE', ( #18163, #825 ) ) ;
#14014=EDGE_LOOP ( 'NONE', ( #20090, #2731 ) ) ;
#14015=DIRECTION ( 'NONE',  ( 0.000000000000000000, 0.000000000000000000, 1.000000000000000000 ) ) ;
#14016=DIRECTION ( 'NONE',  ( 1.000000000000000000, 0.000000000000000000, 0.000000000000000000 ) ) ;
#14017=EDGE_CURVE ( 'NONE', #4105, #21760, #28715, .T. ) ;
#14018=VECTOR ( 'NONE', #24766, 1000.000000000000000 ) ;
#14019=EDGE_CURVE ( 'NONE', #21235, #12727, #20314, .T. ) ;
#14020=CARTESIAN_POINT ( 'NONE',  ( 71.99999662536839651, 17.32050807568879236, -9.999999999999998224 ) ) ;
#14022=AXIS2_PLACEMENT_3D ( 'NONE', #16896, #36771, #11073 ) ;
#14029=ORIENTED_EDGE ( 'NONE', *, *, #29531, .F. ) ;
#14030=EDGE_LOOP ( 'NONE', ( #9916, #8563, #35704, #21824, #822, #32360 ) ) ;
#14031=CARTESIAN_POINT ( 'NONE',  ( -20.00000337463123756, -86.60254037844400443, 17.49999999999999645 ) ) ;
#14032=CARTESIAN_POINT ( 'NONE',  ( 24.99999662536859546, -77.94228634059960825, -9.999999999999998224 ) ) ;
#14033=DIRECTION ( 'NONE',  ( -0.000000000000000000, -0.000000000000000000, -1.000000000000000000 ) ) ;
#14034=VECTOR ( 'NONE', #913, 1000.000000000000000 ) ;
#14036=VERTEX_POINT ( 'NONE', #8205 ) ;
#14037=AXIS2_PLACEMENT_3D ( 'NONE', #17821, #32437, #29813 ) ;
#14038=CARTESIAN_POINT ( 'NONE',  ( 74.99999662536836809, -8.660254037844401509, 17.49999999999999645 ) ) ;
#14039=ORIENTED_EDGE ( 'NONE', *, *, #30749, .F. ) ;
#14040=ORIENTED_EDGE ( 'NONE', *, *, #35022, .F. ) ;
#14042=VERTEX_POINT ( 'NONE', #31073 ) ;
#14044=EDGE_CURVE ( 'NONE', #34700, #34695, #7156, .T. ) ;
#14045=DIRECTION ( 'NONE',  ( 1.000000000000000000, 0.000000000000000000, 0.000000000000000000 ) ) ;
#14046=AXIS2_PLACEMENT_3D ( 'NONE', #3170, #23799, #32408 ) ;
#14047=CIRCLE ( 'NONE', #15855, 2.000000000000001776 ) ;
#14048=FACE_OUTER_BOUND ( 'NONE', #28303, .T. ) ;
#14049=CIRCLE ( 'NONE', #2685, 3.000000000000002665 ) ;
#14051=VERTEX_POINT ( 'NONE', #14382 ) ;
#14053=ORIENTED_EDGE ( 'NONE', *, *, #29637, .T. ) ;
#14054=ORIENTED_EDGE ( 'NONE', *, *, #10352, .F. ) ;
#14055=ORIENTED_EDGE ( 'NONE', *, *, #35550, .F. ) ;
#14057=CARTESIAN_POINT ( 'NONE',  ( 77.99999662536833966, 34.64101615137759183, 12.50000000000000000 ) ) ;
#14058=CARTESIAN_POINT ( 'NONE',  ( 39.99999662536853151, 69.28203230275518365, -5.000000000000000000 ) ) ;
#14060=DIRECTION ( 'NONE',  ( 1.000000000000000000, 0.000000000000000000, 0.000000000000000000 ) ) ;
#14062=CARTESIAN_POINT ( 'NONE',  ( -63.00000337463102085, 43.30127018922198801, -9.999999999999998224 ) ) ;
#14063=VERTEX_POINT ( 'NONE', #2953 ) ;
#14065=CIRCLE ( 'NONE', #1511, 2.000000000000001776 ) ;
#14066=DIRECTION ( 'NONE',  ( 0.000000000000000000, 0.000000000000000000, 1.000000000000000000 ) ) ;
#14067=ADVANCED_FACE ( 'NONE', ( #11543 ), #19997, .F. ) ;
#14068=DIRECTION ( 'NONE',  ( 0.000000000000000000, 0.000000000000000000, 1.000000000000000000 ) ) ;
#14069=ORIENTED_EDGE ( 'NONE', *, *, #36634, .T. ) ;
#14070=LINE ( 'NONE', #30957, #18474 ) ;
#14071=CARTESIAN_POINT ( 'NONE',  ( 79.99999662536833966, -3.469446951953614189E-15, -9.999999999999998224 ) ) ;
#14073=ORIENTED_EDGE ( 'NONE', *, *, #10709, .F. ) ;
#14074=AXIS2_PLACEMENT_3D ( 'NONE', #9641, #6257, #32321 ) ;
#14075=ORIENTED_EDGE ( 'NONE', *, *, #35614, .F. ) ;
#14078=DIRECTION ( 'NONE',  ( 1.000000000000000000, 0.000000000000000000, 0.000000000000000000 ) ) ;
#14080=ORIENTED_EDGE ( 'NONE', *, *, #10131, .T. ) ;
#14081=ORIENTED_EDGE ( 'NONE', *, *, #28772, .T. ) ;
#14082=CARTESIAN_POINT ( 'NONE',  ( 34.99999662536855283, -60.62177826491080168, -9.999999999999998224 ) ) ;
#14083=AXIS2_PLACEMENT_3D ( 'NONE', #27488, #4622, #33100 ) ;
#14084=ORIENTED_EDGE ( 'NONE', *, *, #35075, .F. ) ;
#14086=DIRECTION ( 'NONE',  ( 1.000000000000000000, 0.000000000000000000, -0.000000000000000000 ) ) ;
#14087=ORIENTED_EDGE ( 'NONE', *, *, #8040, .F. ) ;
#14088=EDGE_CURVE ( 'NONE', #13581, #22989, #17195, .T. ) ;
#14089=AXIS2_PLACEMENT_3D ( 'NONE', #27690, #13433, #16641 ) ;
#14095=FACE_BOUND ( 'NONE', #6627, .T. ) ;
#14096=ORIENTED_EDGE ( 'NONE', *, *, #943, .T. ) ;
#14097=ADVANCED_FACE ( 'NONE', ( #34439 ), #115, .F. ) ;
#14098=EDGE_LOOP ( 'NONE', ( #14839, #7499 ) ) ;
#14099=DIRECTION ( 'NONE',  ( 0.000000000000000000, 0.000000000000000000, -1.000000000000000000 ) ) ;
#14101=AXIS2_PLACEMENT_3D ( 'NONE', #36843, #19246, #19608 ) ;
#14102=CARTESIAN_POINT ( 'NONE',  ( -83.00000337463092137, -8.660254037844422825, 17.49999999999999645 ) ) ;
#14103=AXIS2_PLACEMENT_3D ( 'NONE', #28059, #4832, #35964 ) ;
#14104=CARTESIAN_POINT ( 'NONE',  ( 66.99999662536839651, 60.62177826491078747, -5.000000000000000000 ) ) ;
#14105=ADVANCED_FACE ( 'NONE', ( #33703 ), #22997, .F. ) ;
#14106=ORIENTED_EDGE ( 'NONE', *, *, #17558, .F. ) ;
#14107=FACE_OUTER_BOUND ( 'NONE', #13626, .T. ) ;
#14108=FACE_BOUND ( 'NONE', #4465, .T. ) ;
#14109=DIRECTION ( 'NONE',  ( 0.000000000000000000, 0.000000000000000000, -1.000000000000000000 ) ) ;
#14110=FACE_OUTER_BOUND ( 'NONE', #8109, .T. ) ;
#14113=CARTESIAN_POINT ( 'NONE',  ( -2.000003374631327713, 86.60254037844397601, -9.999999999999998224 ) ) ;
#14115=EDGE_CURVE ( 'NONE', #21277, #11692, #20187, .T. ) ;
#14117=ORIENTED_EDGE ( 'NONE', *, *, #10732, .T. ) ;
#14118=CARTESIAN_POINT ( 'NONE',  ( 74.99999662536835388, -43.30127018922199511, 12.50000000000000000 ) ) ;
#14121=FACE_OUTER_BOUND ( 'NONE', #33653, .T. ) ;
#14122=CIRCLE ( 'NONE', #2756, 2.000000000000000000 ) ;
#14123=AXIS2_PLACEMENT_3D ( 'NONE', #12170, #29263, #26831 ) ;
#14124=ORIENTED_EDGE ( 'NONE', *, *, #8180, .T. ) ;
#14125=CIRCLE ( 'NONE', #29695, 2.000000000000000000 ) ;
#14126=ORIENTED_EDGE ( 'NONE', *, *, #16391, .F. ) ;
#14127=AXIS2_PLACEMENT_3D ( 'NONE', #23208, #12102, #20388 ) ;
#14128=VERTEX_POINT ( 'NONE', #11381 ) ;
#14129=CARTESIAN_POINT ( 'NONE',  ( 70.47608876694671665, 59.13646009116074964, 12.49999999999999822 ) ) ;
#14130=DIRECTION ( 'NONE',  ( 0.000000000000000000, 0.000000000000000000, -1.000000000000000000 ) ) ;
#14131=VERTEX_POINT ( 'NONE', #22828 ) ;
#14132=AXIS2_PLACEMENT_3D ( 'NONE', #25256, #27676, #30851 ) ;
#14133=AXIS2_PLACEMENT_3D ( 'NONE', #9191, #36, #6036 ) ;
#14134=DIRECTION ( 'NONE',  ( 0.000000000000000000, 0.000000000000000000, 1.000000000000000000 ) ) ;
#14135=EDGE_LOOP ( 'NONE', ( #13501, #28157, #542, #34540 ) ) ;
#14136=EDGE_CURVE ( 'NONE', #8997, #29480, #8009, .T. ) ;
#14138=ORIENTED_EDGE ( 'NONE', *, *, #14171, .T. ) ;
#14139=CARTESIAN_POINT ( 'NONE',  ( -85.00000337463092137, -8.660254037844422825, 17.49999999999999645 ) ) ;
#14141=ORIENTED_EDGE ( 'NONE', *, *, #7039, .T. ) ;
#14142=DIRECTION ( 'NONE',  ( 0.000000000000000000, 0.000000000000000000, 1.000000000000000000 ) ) ;
#14145=ADVANCED_FACE ( 'NONE', ( #19448 ), #31613, .F. ) ;
#14146=ORIENTED_EDGE ( 'NONE', *, *, #22910, .F. ) ;
#14148=CYLINDRICAL_SURFACE ( 'NONE', #14672, 2.000000000000001776 ) ;
#14149=VECTOR ( 'NONE', #36824, 1000.000000000000000 ) ;
#14150=CIRCLE ( 'NONE', #16572, 2.000000000000001776 ) ;
#14152=VECTOR ( 'NONE', #35015, 1000.000000000000000 ) ;
#14153=CIRCLE ( 'NONE', #29723, 2.999999999999999556 ) ;
#14154=CARTESIAN_POINT ( 'NONE',  ( 71.99999662536841072, 51.96152422706640550, 12.50000000000000000 ) ) ;
#14155=CARTESIAN_POINT ( 'NONE',  ( -35.00000337463116296, 60.62177826491077326, 12.50000000000000000 ) ) ;
#14156=EDGE_CURVE ( 'NONE', #20671, #32894, #17381, .T. ) ;
#14157=VERTEX_POINT ( 'NONE', #30870 ) ;
#14159=CARTESIAN_POINT ( 'NONE',  ( -83.47442710120355969, 31.09745072740822991, -4.999999999999997335 ) ) ;
#14160=ORIENTED_EDGE ( 'NONE', *, *, #11737, .T. ) ;
#14161=DIRECTION ( 'NONE',  ( 1.000000000000000000, 0.000000000000000000, 0.000000000000000000 ) ) ;
#14162=DIRECTION ( 'NONE',  ( 1.000000000000000000, 0.000000000000000000, 0.000000000000000000 ) ) ;
#14163=DIRECTION ( 'NONE',  ( -1.000000000000000000, 0.000000000000000000, 0.000000000000000000 ) ) ;
#14164=DIRECTION ( 'NONE',  ( 0.000000000000000000, 0.000000000000000000, -1.000000000000000000 ) ) ;
#14165=CIRCLE ( 'NONE', #29149, 2.000000000000001776 ) ;
#14166=ORIENTED_EDGE ( 'NONE', *, *, #29935, .F. ) ;
#14167=EDGE_LOOP ( 'NONE', ( #7741, #15233 ) ) ;
#14169=CARTESIAN_POINT ( 'NONE',  ( -20.00000337463122690, 86.60254037844397601, 12.50000000000000000 ) ) ;
#14171=EDGE_CURVE ( 'NONE', #35934, #33595, #23943, .T. ) ;
#14172=EDGE_LOOP ( 'NONE', ( #28416, #11203, #14270, #20732 ) ) ;
#14173=VERTEX_POINT ( 'NONE', #17002 ) ;
#14174=AXIS2_PLACEMENT_3D ( 'NONE', #19473, #10856, #5427 ) ;
#14176=DIRECTION ( 'NONE',  ( 1.000000000000000000, 0.000000000000000000, 0.000000000000000000 ) ) ;
#14178=FACE_OUTER_BOUND ( 'NONE', #29218, .T. ) ;
#14179=AXIS2_PLACEMENT_3D ( 'NONE', #9874, #4443, #32753 ) ;
#14181=EDGE_CURVE ( 'NONE', #4797, #10781, #13143, .T. ) ;
#14182=ORIENTED_EDGE ( 'NONE', *, *, #16523, .F. ) ;
#14184=AXIS2_PLACEMENT_3D ( 'NONE', #27113, #12856, #17954 ) ;
#14186=ORIENTED_EDGE ( 'NONE', *, *, #19863, .F. ) ;
#14187=EDGE_CURVE ( 'NONE', #5725, #31117, #13827, .T. ) ;
#14188=DIRECTION ( 'NONE',  ( 0.000000000000000000, 0.000000000000000000, 1.000000000000000000 ) ) ;
#14190=FACE_BOUND ( 'NONE', #25283, .T. ) ;
#14191=AXIS2_PLACEMENT_3D ( 'NONE', #4332, #4515, #32447 ) ;
#14192=CARTESIAN_POINT ( 'NONE',  ( -82.00000337463096400, -34.64101615137762025, -5.000000000000000000 ) ) ;
#14194=VECTOR ( 'NONE', #21257, 1000.000000000000000 ) ;
#14195=VERTEX_POINT ( 'NONE', #10996 ) ;
#14198=AXIS2_PLACEMENT_3D ( 'NONE', #10886, #22153, #19165 ) ;
#14199=DIRECTION ( 'NONE',  ( -1.000000000000000000, 0.000000000000000000, 0.000000000000000000 ) ) ;
#14200=EDGE_CURVE ( 'NONE', #15209, #19312, #31671, .T. ) ;
#14201=AXIS2_PLACEMENT_3D ( 'NONE', #13212, #25218, #4786 ) ;
#14202=DIRECTION ( 'NONE',  ( 0.000000000000000000, 0.000000000000000000, -1.000000000000000000 ) ) ;
#14204=VERTEX_POINT ( 'NONE', #29364 ) ;
#14205=CARTESIAN_POINT ( 'NONE',  ( 64.99999662536839651, 60.62177826491078747, 12.50000000000000000 ) ) ;
#14207=CARTESIAN_POINT ( 'NONE',  ( 34.99999662536853862, 77.94228634059959404, -9.999999999999998224 ) ) ;
#14208=DIRECTION ( 'NONE',  ( 1.000000000000000000, 0.000000000000000000, 0.000000000000000000 ) ) ;
#14210=VERTEX_POINT ( 'NONE', #34991 ) ;
#14213=ORIENTED_EDGE ( 'NONE', *, *, #3410, .T. ) ;
#14214=CARTESIAN_POINT ( 'NONE',  ( -63.00000337463102085, 25.98076211353317433, -9.999999999999998224 ) ) ;
#14215=CIRCLE ( 'NONE', #26795, 2.000000000000001776 ) ;
#14216=FACE_OUTER_BOUND ( 'NONE', #24253, .T. ) ;
#14218=AXIS2_PLACEMENT_3D ( 'NONE', #6625, #27219, #12414 ) ;
#14219=CARTESIAN_POINT ( 'NONE',  ( -52.00000337463109190, 51.96152422706637708, -9.999999999999998224 ) ) ;
#14222=EDGE_CURVE ( 'NONE', #35764, #22350, #23381, .T. ) ;
#14226=LINE ( 'NONE', #3152, #35832 ) ;
#14227=ORIENTED_EDGE ( 'NONE', *, *, #20197, .T. ) ;
#14228=AXIS2_PLACEMENT_3D ( 'NONE', #24915, #6600, #27542 ) ;
#14229=EDGE_CURVE ( 'NONE', #22833, #33342, #12537, .T. ) ;
#14230=VERTEX_POINT ( 'NONE', #31955 ) ;
#14231=CYLINDRICAL_SURFACE ( 'NONE', #27850, 2.000000000000001776 ) ;
#14232=AXIS2_PLACEMENT_3D ( 'NONE', #20474, #32653, #35118 ) ;
#14233=CARTESIAN_POINT ( 'NONE',  ( -56.56139351304917540, -61.87160258682602176, -5.000000000000000000 ) ) ;
#14234=CARTESIAN_POINT ( 'NONE',  ( -2.000003374631334818, 69.28203230275516944, -9.999999999999998224 ) ) ;
#14235=CARTESIAN_POINT ( 'NONE',  ( -50.00000337463109190, 51.96152422706637708, -9.999999999999998224 ) ) ;
#14236=EDGE_CURVE ( 'NONE', #24803, #11966, #6557, .T. ) ;
#14238=EDGE_CURVE ( 'NONE', #5952, #26437, #27514, .T. ) ;
#14239=CIRCLE ( 'NONE', #13563, 2.000000000000001776 ) ;
#14240=AXIS2_PLACEMENT_3D ( 'NONE', #24450, #16365, #30614 ) ;
#14241=FACE_BOUND ( 'NONE', #6498, .T. ) ;
#14242=ORIENTED_EDGE ( 'NONE', *, *, #11060, .T. ) ;
#14243=VERTEX_POINT ( 'NONE', #20371 ) ;
#14244=CARTESIAN_POINT ( 'NONE',  ( -63.00000337463106348, -60.62177826491083010, -9.999999999999998224 ) ) ;
#14245=ORIENTED_EDGE ( 'NONE', *, *, #10561, .T. ) ;
#14246=AXIS2_PLACEMENT_3D ( 'NONE', #31768, #23709, #15086 ) ;
#14247=EDGE_CURVE ( 'NONE', #26162, #7932, #15526, .T. ) ;
#14250=EDGE_CURVE ( 'NONE', #35812, #16375, #34115, .T. ) ;
#14252=EDGE_CURVE ( 'NONE', #13826, #36096, #33527, .T. ) ;
#14253=CIRCLE ( 'NONE', #34632, 65.00000000000000000 ) ;
#14255=EDGE_CURVE ( 'NONE', #21994, #12226, #9553, .T. ) ;
#14257=EDGE_CURVE ( 'NONE', #32638, #33663, #20724, .T. ) ;
#14258=ORIENTED_EDGE ( 'NONE', *, *, #6135, .T. ) ;
#14259=AXIS2_PLACEMENT_3D ( 'NONE', #2882, #9043, #32075 ) ;
#14260=EDGE_LOOP ( 'NONE', ( #30052, #24126 ) ) ;
#14261=AXIS2_PLACEMENT_3D ( 'NONE', #20013, #2773, #16847 ) ;
#14262=ORIENTED_EDGE ( 'NONE', *, *, #1951, .F. ) ;
#14264=VERTEX_POINT ( 'NONE', #32362 ) ;
#14265=LINE ( 'NONE', #17602, #19454 ) ;
#14266=DIRECTION ( 'NONE',  ( 0.000000000000000000, 0.000000000000000000, 1.000000000000000000 ) ) ;
#14267=CARTESIAN_POINT ( 'NONE',  ( -20.00000337463122690, 86.60254037844397601, -5.000000000000000000 ) ) ;
#14268=CARTESIAN_POINT ( 'NONE',  ( 56.67878100130369035, -27.78182860042797131, 12.49999999999999822 ) ) ;
#14269=CARTESIAN_POINT ( 'NONE',  ( 69.99999662536838230, -51.96152422706639840, -5.000000000000000000 ) ) ;
#14270=ORIENTED_EDGE ( 'NONE', *, *, #34251, .F. ) ;
#14271=DIRECTION ( 'NONE',  ( 0.000000000000000000, 0.000000000000000000, 1.000000000000000000 ) ) ;
#14272=AXIS2_PLACEMENT_3D ( 'NONE', #33742, #5984, #5596 ) ;
#14274=DIRECTION ( 'NONE',  ( 0.000000000000000000, 0.000000000000000000, 1.000000000000000000 ) ) ;
#14275=ORIENTED_EDGE ( 'NONE', *, *, #26640, .T. ) ;
#14277=DIRECTION ( 'NONE',  ( -0.000000000000000000, -0.000000000000000000, 1.000000000000000000 ) ) ;
#14278=AXIS2_PLACEMENT_3D ( 'NONE', #22655, #2585, #13840 ) ;
#14279=ORIENTED_EDGE ( 'NONE', *, *, #12668, .F. ) ;
#14280=VERTEX_POINT ( 'NONE', #34635 ) ;
#14281=CARTESIAN_POINT ( 'NONE',  ( -85.00000337463092137, 8.660254037844389075, 12.50000000000000000 ) ) ;
#14282=CIRCLE ( 'NONE', #33454, 2.000000000000001776 ) ;
#14283=CARTESIAN_POINT ( 'NONE',  ( -85.00000337463092137, 25.98076211353317433, -5.000000000000000000 ) ) ;
#14286=ORIENTED_EDGE ( 'NONE', *, *, #31089, .F. ) ;
#14287=VERTEX_POINT ( 'NONE', #17545 ) ;
#14288=CIRCLE ( 'NONE', #31616, 2.000000000000001776 ) ;
#14289=AXIS2_PLACEMENT_3D ( 'NONE', #5928, #8912, #11896 ) ;
#14291=DIRECTION ( 'NONE',  ( 0.000000000000000000, 0.000000000000000000, 1.000000000000000000 ) ) ;
#14292=VECTOR ( 'NONE', #35629, 1000.000000000000000 ) ;
#14293=ORIENTED_EDGE ( 'NONE', *, *, #34418, .F. ) ;
#14294=DIRECTION ( 'NONE',  ( 0.000000000000000000, 0.000000000000000000, 1.000000000000000000 ) ) ;
#14295=ORIENTED_EDGE ( 'NONE', *, *, #5015, .T. ) ;
#14296=CARTESIAN_POINT ( 'NONE',  ( 64.99999662536841072, 25.98076211353318854, 17.49999999999999645 ) ) ;
#14297=AXIS2_PLACEMENT_3D ( 'NONE', #22922, #13922, #34550 ) ;
#14298=DIRECTION ( 'NONE',  ( 0.000000000000000000, 0.000000000000000000, 1.000000000000000000 ) ) ;
#14300=CARTESIAN_POINT ( 'NONE',  ( 9.999996625368655856, -86.60254037844400443, -5.000000000000000000 ) ) ;
#14301=EDGE_CURVE ( 'NONE', #20440, #33271, #30521, .T. ) ;
#14302=ORIENTED_EDGE ( 'NONE', *, *, #9133, .T. ) ;
#14303=ORIENTED_EDGE ( 'NONE', *, *, #34183, .T. ) ;
#14304=FACE_OUTER_BOUND ( 'NONE', #21835, .T. ) ;
#14305=DIRECTION ( 'NONE',  ( 0.000000000000000000, 0.000000000000000000, 1.000000000000000000 ) ) ;
#14306=CARTESIAN_POINT ( 'NONE',  ( 54.99999662536844625, 60.62177826491077326, 12.50000000000000000 ) ) ;
#14308=EDGE_LOOP ( 'NONE', ( #2764, #1530 ) ) ;
#14309=LINE ( 'NONE', #25759, #35145 ) ;
#14311=FACE_BOUND ( 'NONE', #12641, .T. ) ;
#14312=AXIS2_PLACEMENT_3D ( 'NONE', #503, #28975, #29369 ) ;
#14314=LINE ( 'NONE', #19927, #26473 ) ;
#14315=CARTESIAN_POINT ( 'NONE',  ( -5.000003374631307729, 77.94228634059957983, 12.50000000000000000 ) ) ;
#14316=DIRECTION ( 'NONE',  ( 0.000000000000000000, 0.000000000000000000, -1.000000000000000000 ) ) ;
#14318=CIRCLE ( 'NONE', #2727, 2.000000000000001776 ) ;
#14320=VERTEX_POINT ( 'NONE', #14735 ) ;
#14321=CARTESIAN_POINT ( 'NONE',  ( -53.00000337463110611, -43.30127018922202353, 12.50000000000000000 ) ) ;
#14324=CIRCLE ( 'NONE', #17908, 33.00000000000001421 ) ;
#14325=ADVANCED_FACE ( 'NONE', ( #12087 ), #9289, .F. ) ;
#14326=VERTEX_POINT ( 'NONE', #32160 ) ;
#14327=ORIENTED_EDGE ( 'NONE', *, *, #32650, .F. ) ;
#14328=AXIS2_PLACEMENT_3D ( 'NONE', #31252, #25828, #14555 ) ;
#14329=ORIENTED_EDGE ( 'NONE', *, *, #21996, .F. ) ;
#14330=CARTESIAN_POINT ( 'NONE',  ( -85.00000337463092137, 25.98076211353317433, 17.49999999999999645 ) ) ;
#14331=CARTESIAN_POINT ( 'NONE',  ( -27.00000337463121625, -77.94228634059963667, 17.49999999999999645 ) ) ;
#14332=CIRCLE ( 'NONE', #22123, 2.000000000000001776 ) ;
#14333=DIRECTION ( 'NONE',  ( 0.000000000000000000, 0.000000000000000000, 1.000000000000000000 ) ) ;
#14334=VERTEX_POINT ( 'NONE', #17933 ) ;
#14335=LINE ( 'NONE', #20486, #20282 ) ;
#14336=AXIS2_PLACEMENT_3D ( 'NONE', #21501, #26938, #1251 ) ;
#14337=ORIENTED_EDGE ( 'NONE', *, *, #3506, .F. ) ;
#14338=CARTESIAN_POINT ( 'NONE',  ( 69.99999662536838230, -51.96152422706639840, 12.50000000000000000 ) ) ;
#14339=ORIENTED_EDGE ( 'NONE', *, *, #329, .T. ) ;
#14341=CARTESIAN_POINT ( 'NONE',  ( 69.99999662536839651, -3.469446951953614189E-15, -9.999999999999998224 ) ) ;
#14342=ORIENTED_EDGE ( 'NONE', *, *, #26290, .F. ) ;
#14343=ORIENTED_EDGE ( 'NONE', *, *, #27737, .F. ) ;
#14344=CYLINDRICAL_SURFACE ( 'NONE', #34561, 27.00000000000001066 ) ;
#14345=CARTESIAN_POINT ( 'NONE',  ( -37.00000337463116296, -60.62177826491080168, 12.50000000000000000 ) ) ;
#14346=CARTESIAN_POINT ( 'NONE',  ( 0.000000000000000000, 0.000000000000000000, 12.49999999999999822 ) ) ;
#14348=ORIENTED_EDGE ( 'NONE', *, *, #1988, .F. ) ;
#14349=CARTESIAN_POINT ( 'NONE',  ( 0.000000000000000000, 0.000000000000000000, 17.49999999999999645 ) ) ;
#14351=AXIS2_PLACEMENT_3D ( 'NONE', #15492, #14939, #6294 ) ;
#14353=CARTESIAN_POINT ( 'NONE',  ( -8.000003374631281972, 86.60254037844397601, -9.999999999999998224 ) ) ;
#14354=AXIS2_PLACEMENT_3D ( 'NONE', #16054, #32930, #30099 ) ;
#14356=DIRECTION ( 'NONE',  ( 0.8660254037844415942, 0.4999999999999949485, 0.000000000000000000 ) ) ;
#14358=ORIENTED_EDGE ( 'NONE', *, *, #33872, .F. ) ;
#14359=CARTESIAN_POINT ( 'NONE',  ( 36.99999662536853862, 77.94228634059959404, -5.000000000000000000 ) ) ;
#14360=CARTESIAN_POINT ( 'NONE',  ( 29.99999662536856349, 69.28203230275518365, 12.50000000000000000 ) ) ;
#14361=AXIS2_PLACEMENT_3D ( 'NONE', #16719, #13509, #13325 ) ;
#14362=DIRECTION ( 'NONE',  ( 0.000000000000000000, 0.000000000000000000, 1.000000000000000000 ) ) ;
#14363=DIRECTION ( 'NONE',  ( 1.000000000000000000, 0.000000000000000000, 0.000000000000000000 ) ) ;
#14364=EDGE_LOOP ( 'NONE', ( #5597, #25420, #852, #34766 ) ) ;
#14365=VECTOR ( 'NONE', #21677, 1000.000000000000000 ) ;
#14366=ADVANCED_FACE ( 'NONE', ( #3679 ), #15108, .F. ) ;
#14368=CIRCLE ( 'NONE', #15543, 27.00000000000001421 ) ;
#14369=DIRECTION ( 'NONE',  ( 0.000000000000000000, 0.000000000000000000, -1.000000000000000000 ) ) ;
#14371=EDGE_CURVE ( 'NONE', #1473, #10472, #12266, .T. ) ;
#14372=ORIENTED_EDGE ( 'NONE', *, *, #13830, .F. ) ;
#14373=ORIENTED_EDGE ( 'NONE', *, *, #8558, .T. ) ;
#14377=CIRCLE ( 'NONE', #28127, 1.999999999999998224 ) ;
#14378=EDGE_LOOP ( 'NONE', ( #35144, #25906 ) ) ;
#14379=EDGE_CURVE ( 'NONE', #9986, #1659, #27477, .T. ) ;
#14380=DIRECTION ( 'NONE',  ( 0.000000000000000000, 0.000000000000000000, 1.000000000000000000 ) ) ;
#14381=ORIENTED_EDGE ( 'NONE', *, *, #30366, .T. ) ;
#14382=CARTESIAN_POINT ( 'NONE',  ( 66.86787810013036903, -2.778182860042780700, -4.999999999999997335 ) ) ;
#14383=ORIENTED_EDGE ( 'NONE', *, *, #24907, .T. ) ;
#14384=PLANE ( 'NONE',  #36314 ) ;
#14386=CARTESIAN_POINT ( 'NONE',  ( 9.999996625368618552, 69.28203230275516944, -9.999999999999998224 ) ) ;
#14387=AXIS2_PLACEMENT_3D ( 'NONE', #23971, #12510, #35418 ) ;
#14388=DIRECTION ( 'NONE',  ( 1.000000000000000000, 0.000000000000000000, 0.000000000000000000 ) ) ;
#14389=EDGE_LOOP ( 'NONE', ( #33959, #26503 ) ) ;
#14391=DIRECTION ( 'NONE',  ( 0.000000000000000000, 0.000000000000000000, -1.000000000000000000 ) ) ;
#14392=EDGE_CURVE ( 'NONE', #20758, #34308, #16179, .T. ) ;
#14393=DIRECTION ( 'NONE',  ( 0.000000000000000000, 0.000000000000000000, 1.000000000000000000 ) ) ;
#14394=CARTESIAN_POINT ( 'NONE',  ( 57.99999662536844625, 34.64101615137759893, -9.999999999999998224 ) ) ;
#14396=CIRCLE ( 'NONE', #4241, 2.000000000000001776 ) ;
#14397=DIRECTION ( 'NONE',  ( 1.000000000000000000, 0.000000000000000000, 0.000000000000000000 ) ) ;
#14398=DIRECTION ( 'NONE',  ( 0.000000000000000000, 0.000000000000000000, -1.000000000000000000 ) ) ;
#14399=DIRECTION ( 'NONE',  ( -1.000000000000000000, 0.000000000000000000, 0.000000000000000000 ) ) ;
#14400=EDGE_CURVE ( 'NONE', #33302, #20878, #25152, .T. ) ;
#14401=ORIENTED_EDGE ( 'NONE', *, *, #11211, .T. ) ;
#14402=ORIENTED_EDGE ( 'NONE', *, *, #22616, .T. ) ;
#14403=EDGE_CURVE ( 'NONE', #807, #24141, #29919, .T. ) ;
#14404=AXIS2_PLACEMENT_3D ( 'NONE', #10130, #21564, #32994 ) ;
#14405=ORIENTED_EDGE ( 'NONE', *, *, #5724, .F. ) ;
#14409=FACE_OUTER_BOUND ( 'NONE', #11229, .T. ) ;
#14411=DIRECTION ( 'NONE',  ( 0.000000000000000000, 0.000000000000000000, 1.000000000000000000 ) ) ;
#14413=ORIENTED_EDGE ( 'NONE', *, *, #36266, .F. ) ;
#14414=VERTEX_POINT ( 'NONE', #7240 ) ;
#14415=DIRECTION ( 'NONE',  ( 0.000000000000000000, 0.000000000000000000, -1.000000000000000000 ) ) ;
#14416=ADVANCED_FACE ( 'NONE', ( #33487 ), #12833, .F. ) ;
#14418=CARTESIAN_POINT ( 'NONE',  ( 14.99999662536863632, -77.94228634059960825, -5.000000000000000000 ) ) ;
#14419=CARTESIAN_POINT ( 'NONE',  ( 69.99999662536839651, -3.469446951953614189E-15, -9.999999999999998224 ) ) ;
#14420=ORIENTED_EDGE ( 'NONE', *, *, #9196, .F. ) ;
#14422=CARTESIAN_POINT ( 'NONE',  ( -90.00000337463090716, -1.040834085586084257E-14, -9.999999999999998224 ) ) ;
#14423=VERTEX_POINT ( 'NONE', #4417 ) ;
#14424=ORIENTED_EDGE ( 'NONE', *, *, #1222, .T. ) ;
#14425=AXIS2_PLACEMENT_3D ( 'NONE', #24574, #32605, #18374 ) ;
#14427=ORIENTED_EDGE ( 'NONE', *, *, #23854, .F. ) ;
#14428=CARTESIAN_POINT ( 'NONE',  ( 69.99999662536839651, -17.32050807568879947, 17.49999999999999645 ) ) ;
#14430=FACE_BOUND ( 'NONE', #31366, .T. ) ;
#14431=ORIENTED_EDGE ( 'NONE', *, *, #33084, .T. ) ;
#14432=EDGE_CURVE ( 'NONE', #31374, #24444, #7050, .T. ) ;
#14434=ORIENTED_EDGE ( 'NONE', *, *, #33989, .F. ) ;
#14435=EDGE_CURVE ( 'NONE', #3388, #5117, #31726, .T. ) ;
#14436=ORIENTED_EDGE ( 'NONE', *, *, #8180, .F. ) ;
#14437=ORIENTED_EDGE ( 'NONE', *, *, #22430, .F. ) ;
#14438=DIRECTION ( 'NONE',  ( 0.000000000000000000, 0.000000000000000000, -1.000000000000000000 ) ) ;
#14439=ADVANCED_FACE ( 'NONE', ( #1239 ), #12656, .F. ) ;
#14440=DIRECTION ( 'NONE',  ( 0.000000000000000000, 0.000000000000000000, 1.000000000000000000 ) ) ;
#14441=EDGE_CURVE ( 'NONE', #25326, #10648, #582, .T. ) ;
#14442=AXIS2_PLACEMENT_3D ( 'NONE', #12928, #1493, #4705 ) ;
#14444=FACE_OUTER_BOUND ( 'NONE', #4211, .T. ) ;
#14445=CARTESIAN_POINT ( 'NONE',  ( 68.17080445151383117, -51.15278694518232072, -5.000000000000000000 ) ) ;
#14446=EDGE_CURVE ( 'NONE', #15915, #34006, #36290, .T. ) ;
#14447=EDGE_LOOP ( 'NONE', ( #3999, #13391 ) ) ;
#14448=DIRECTION ( 'NONE',  ( 1.000000000000000000, 0.000000000000000000, 0.000000000000000000 ) ) ;
#14449=CARTESIAN_POINT ( 'NONE',  ( -44.13139720814380951, 27.50000000000055422, -10.00000000000000000 ) ) ;
#14450=CARTESIAN_POINT ( 'NONE',  ( 49.99999662536846756, 69.28203230275516944, -9.999999999999998224 ) ) ;
#14452=CARTESIAN_POINT ( 'NONE',  ( -40.00000337463113453, -69.28203230275519786, -9.999999999999998224 ) ) ;
#14453=FACE_OUTER_BOUND ( 'NONE', #32127, .T. ) ;
#14454=ADVANCED_FACE ( 'NONE', ( #16236 ), #1966, .F. ) ;
#14457=ORIENTED_EDGE ( 'NONE', *, *, #4042, .T. ) ;
#14458=DIRECTION ( 'NONE',  ( 1.000000000000000000, 0.000000000000000000, 0.000000000000000000 ) ) ;
#14459=ADVANCED_FACE ( 'NONE', ( #28211 ), #8696, .F. ) ;
#14460=CARTESIAN_POINT ( 'NONE',  ( -70.00000337463099243, 17.32050807568877460, -9.999999999999998224 ) ) ;
#14463=CARTESIAN_POINT ( 'NONE',  ( 64.99999662536841072, 25.98076211353318854, -5.000000000000000000 ) ) ;
#14472=VERTEX_POINT ( 'NONE', #2355 ) ;
#14473=VERTEX_POINT ( 'NONE', #36658 ) ;
#14474=DIRECTION ( 'NONE',  ( 1.000000000000000000, 0.000000000000000000, 0.000000000000000000 ) ) ;
#14475=EDGE_CURVE ( 'NONE', #21781, #807, #14377, .T. ) ;
#14476=DIRECTION ( 'NONE',  ( 0.000000000000000000, 0.000000000000000000, 1.000000000000000000 ) ) ;
#14477=ORIENTED_EDGE ( 'NONE', *, *, #29136, .T. ) ;
#14479=ORIENTED_EDGE ( 'NONE', *, *, #5104, .F. ) ;
#14481=CARTESIAN_POINT ( 'NONE',  ( -70.00000337463102085, -51.96152422706641971, -9.999999999999998224 ) ) ;
#14482=DIRECTION ( 'NONE',  ( -1.000000000000000000, 0.000000000000000000, 0.000000000000000000 ) ) ;
#14483=VERTEX_POINT ( 'NONE', #19952 ) ;
#14485=FACE_BOUND ( 'NONE', #7081, .T. ) ;
#14486=ADVANCED_FACE ( 'NONE', ( #17145 ), #16955, .F. ) ;
#14487=CARTESIAN_POINT ( 'NONE',  ( 4.279621169095998212, -62.97617850287780072, 12.49999999999999822 ) ) ;
#14488=CARTESIAN_POINT ( 'NONE',  ( -31.09745072740852123, -83.47442710120344600, -5.000000000000011546 ) ) ;
#14489=DIRECTION ( 'NONE',  ( 0.000000000000000000, 0.000000000000000000, 1.000000000000000000 ) ) ;
#14490=DIRECTION ( 'NONE',  ( 0.000000000000000000, 0.000000000000000000, 1.000000000000000000 ) ) ;
#14492=CIRCLE ( 'NONE', #2533, 2.000000000000000000 ) ;
#14493=DIRECTION ( 'NONE',  ( 1.000000000000000000, 0.000000000000000000, 0.000000000000000000 ) ) ;
#14494=ORIENTED_EDGE ( 'NONE', *, *, #18888, .F. ) ;
#14495=CARTESIAN_POINT ( 'NONE',  ( -47.00000337463111322, -77.94228634059960825, 17.49999999999999645 ) ) ;
#14497=DIRECTION ( 'NONE',  ( 1.000000000000000000, 0.000000000000000000, 0.000000000000000000 ) ) ;
#14498=EDGE_CURVE ( 'NONE', #12006, #16632, #8964, .T. ) ;
#14499=ORIENTED_EDGE ( 'NONE', *, *, #4652, .F. ) ;
#14500=ADVANCED_FACE ( 'NONE', ( #5905 ), #22789, .F. ) ;
#14502=ORIENTED_EDGE ( 'NONE', *, *, #11020, .T. ) ;
#14503=EDGE_CURVE ( 'NONE', #30697, #12872, #24560, .T. ) ;
#14506=DIRECTION ( 'NONE',  ( 1.000000000000000000, 0.000000000000000000, 0.000000000000000000 ) ) ;
#14507=CARTESIAN_POINT ( 'NONE',  ( -87.00000337463093558, 8.660254037844389075, -5.000000000000000000 ) ) ;
#14509=CARTESIAN_POINT ( 'NONE',  ( 35.19434990244975126, -52.39915983220758022, -49.22241343995298024 ) ) ;
#14510=CIRCLE ( 'NONE', #14534, 2.000000000000001776 ) ;
#14511=ORIENTED_EDGE ( 'NONE', *, *, #21585, .T. ) ;
#14513=VERTEX_POINT ( 'NONE', #27827 ) ;
#14514=CARTESIAN_POINT ( 'NONE',  ( -2.374207310413330682E-13, -68.00000000000000000, -49.86348611802629449 ) ) ;
#14516=ORIENTED_EDGE ( 'NONE', *, *, #11837, .T. ) ;
#14517=CARTESIAN_POINT ( 'NONE',  ( -56.52018970185234537, 35.83991598322119643, -49.22241343995295892 ) ) ;
#14519=VECTOR ( 'NONE', #25713, 1000.000000000000000 ) ;
#14520=DIRECTION ( 'NONE',  ( -0.000000000000000000, -0.000000000000000000, 1.000000000000000000 ) ) ;
#14521=ORIENTED_EDGE ( 'NONE', *, *, #33976, .F. ) ;
#14522=DIRECTION ( 'NONE',  ( 0.000000000000000000, 0.000000000000000000, 1.000000000000000000 ) ) ;
#14523=EDGE_CURVE ( 'NONE', #36951, #12099, #20338, .T. ) ;
#14525=FACE_OUTER_BOUND ( 'NONE', #23691, .T. ) ;
#14526=VERTEX_POINT ( 'NONE', #10954 ) ;
#14527=DIRECTION ( 'NONE',  ( 0.000000000000000000, 0.000000000000000000, 1.000000000000000000 ) ) ;
#14528=CARTESIAN_POINT ( 'NONE',  ( -32.50000000000025580, -56.29165124598836201, 12.49999999999999822 ) ) ;
#14529=VERTEX_POINT ( 'NONE', #5360 ) ;
#14530=LINE ( 'NONE', #34611, #21420 ) ;
#14531=DIRECTION ( 'NONE',  ( 0.000000000000000000, 0.000000000000000000, 1.000000000000000000 ) ) ;
#14532=LINE ( 'NONE', #20350, #4017 ) ;
#14534=AXIS2_PLACEMENT_3D ( 'NONE', #3629, #31740, #17874 ) ;
#14535=CARTESIAN_POINT ( 'NONE',  ( -35.00000337463116296, 60.62177826491077326, -9.999999999999998224 ) ) ;
#14536=ORIENTED_EDGE ( 'NONE', *, *, #31220, .F. ) ;
#14537=CYLINDRICAL_SURFACE ( 'NONE', #11733, 2.000000000000001776 ) ;
#14538=DIRECTION ( 'NONE',  ( 1.000000000000000000, 0.000000000000000000, 0.000000000000000000 ) ) ;
#14540=ORIENTED_EDGE ( 'NONE', *, *, #3671, .T. ) ;
#14542=CIRCLE ( 'NONE', #25337, 2.000000000000001776 ) ;
#14543=EDGE_CURVE ( 'NONE', #13993, #21238, #9584, .T. ) ;
#14545=AXIS2_PLACEMENT_3D ( 'NONE', #28559, #8338, #26114 ) ;
#14546=DIRECTION ( 'NONE',  ( 1.000000000000000000, 0.000000000000000000, 0.000000000000000000 ) ) ;
#14551=ORIENTED_EDGE ( 'NONE', *, *, #7392, .T. ) ;
#14552=FACE_BOUND ( 'NONE', #18526, .T. ) ;
#14553=AXIS2_PLACEMENT_3D ( 'NONE', #6790, #32477, #18052 ) ;
#14554=CIRCLE ( 'NONE', #33106, 2.000000000000001776 ) ;
#14555=DIRECTION ( 'NONE',  ( -1.000000000000000000, 0.000000000000000000, 0.000000000000000000 ) ) ;
#14556=DIRECTION ( 'NONE',  ( 0.000000000000000000, 0.000000000000000000, 1.000000000000000000 ) ) ;
#14557=DIRECTION ( 'NONE',  ( 1.000000000000000000, 0.000000000000000000, 0.000000000000000000 ) ) ;
#14560=CARTESIAN_POINT ( 'NONE',  ( -8.000003374631287301, 69.28203230275516944, 17.49999999999999645 ) ) ;
#14561=CIRCLE ( 'NONE', #34355, 2.000000000000001776 ) ;
#14563=LINE ( 'NONE', #17557, #7167 ) ;
#14564=VERTEX_POINT ( 'NONE', #37033 ) ;
#14565=DIRECTION ( 'NONE',  ( -1.000000000000000000, 0.000000000000000000, -0.000000000000000000 ) ) ;
#14567=CARTESIAN_POINT ( 'NONE',  ( -38.00000337463113453, -69.28203230275519786, 17.49999999999999645 ) ) ;
#14568=LINE ( 'NONE', #31802, #27911 ) ;
#14569=VERTEX_POINT ( 'NONE', #34774 ) ;
#14570=EDGE_CURVE ( 'NONE', #34992, #18360, #2394, .T. ) ;
#14571=EDGE_LOOP ( 'NONE', ( #3554, #1197, #36895, #34108 ) ) ;
#14572=VERTEX_POINT ( 'NONE', #20327 ) ;
#14573=AXIS2_PLACEMENT_3D ( 'NONE', #21227, #6987, #30603 ) ;
#14574=AXIS2_PLACEMENT_3D ( 'NONE', #29397, #1091, #23976 ) ;
#14575=CYLINDRICAL_SURFACE ( 'NONE', #22818, 2.000000000000001776 ) ;
#14576=EDGE_CURVE ( 'NONE', #22036, #17723, #7797, .T. ) ;
#14577=DIRECTION ( 'NONE',  ( -1.000000000000000000, 0.000000000000000000, 0.000000000000000000 ) ) ;
#14578=DIRECTION ( 'NONE',  ( 1.000000000000000000, 0.000000000000000000, 0.000000000000000000 ) ) ;
#14579=CARTESIAN_POINT ( 'NONE',  ( 0.000000000000000000, 0.000000000000000000, -10.00000000000000000 ) ) ;
#14580=CARTESIAN_POINT ( 'NONE',  ( 32.16008401677996886, 61.25926521283068382, 12.49999999999999645 ) ) ;
#14581=ORIENTED_EDGE ( 'NONE', *, *, #32367, .F. ) ;
#14582=AXIS2_PLACEMENT_3D ( 'NONE', #34738, #28887, #3409 ) ;
#14585=AXIS2_PLACEMENT_3D ( 'NONE', #2472, #36967, #6023 ) ;
#14586=CARTESIAN_POINT ( 'NONE',  ( -82.00000337463094979, 17.32050807568878525, -9.999999999999998224 ) ) ;
#14587=CARTESIAN_POINT ( 'NONE',  ( -45.00000337463112743, -60.62177826491080168, 12.50000000000000000 ) ) ;
#14589=CIRCLE ( 'NONE', #8602, 27.00000000000001421 ) ;
#14590=ADVANCED_FACE ( 'NONE', ( #23891 ), #29313, .F. ) ;
#14591=FACE_BOUND ( 'NONE', #22829, .T. ) ;
#14592=EDGE_LOOP ( 'NONE', ( #24001, #9910, #22654, #17504 ) ) ;
#14593=VERTEX_POINT ( 'NONE', #20879 ) ;
#14595=CARTESIAN_POINT ( 'NONE',  ( -25.00000337463120914, 77.94228634059957983, 12.50000000000000000 ) ) ;
#14596=EDGE_LOOP ( 'NONE', ( #4338, #34626, #25003 ) ) ;
#14597=EDGE_CURVE ( 'NONE', #5465, #19466, #26337, .T. ) ;
#14598=AXIS2_PLACEMENT_3D ( 'NONE', #26017, #26214, #34469 ) ;
#14599=CARTESIAN_POINT ( 'NONE',  ( -80.00000337463094979, -2.428612866367529932E-14, 12.50000000000000000 ) ) ;
#14600=DIRECTION ( 'NONE',  ( 1.000000000000000000, 0.000000000000000000, -0.000000000000000000 ) ) ;
#14601=ORIENTED_EDGE ( 'NONE', *, *, #6854, .T. ) ;
#14603=EDGE_CURVE ( 'NONE', #3447, #3051, #8387, .T. ) ;
#14604=ORIENTED_EDGE ( 'NONE', *, *, #9391, .T. ) ;
#14605=VECTOR ( 'NONE', #7333, 1000.000000000000000 ) ;
#14606=VERTEX_POINT ( 'NONE', #31912 ) ;
#14607=ADVANCED_FACE ( 'NONE', ( #999 ), #26326, .F. ) ;
#14608=ORIENTED_EDGE ( 'NONE', *, *, #14703, .F. ) ;
#14609=LINE ( 'NONE', #23437, #16453 ) ;
#14611=DIRECTION ( 'NONE',  ( 0.000000000000000000, 0.000000000000000000, 1.000000000000000000 ) ) ;
#14612=DIRECTION ( 'NONE',  ( -0.000000000000000000, -0.000000000000000000, 1.000000000000000000 ) ) ;
#14613=CYLINDRICAL_SURFACE ( 'NONE', #36101, 2.000000000000001776 ) ;
#14614=CARTESIAN_POINT ( 'NONE',  ( -70.00000337463099243, -2.428612866367529932E-14, 12.50000000000000000 ) ) ;
#14615=ORIENTED_EDGE ( 'NONE', *, *, #9099, .T. ) ;
#14617=DIRECTION ( 'NONE',  ( 0.000000000000000000, 0.000000000000000000, -1.000000000000000000 ) ) ;
#14618=PLANE ( 'NONE',  #6239 ) ;
#14619=ORIENTED_EDGE ( 'NONE', *, *, #11287, .F. ) ;
#14620=DIRECTION ( 'NONE',  ( 1.000000000000000000, 0.000000000000000000, 0.000000000000000000 ) ) ;
#14621=DIRECTION ( 'NONE',  ( 1.000000000000000000, 0.000000000000000000, 0.000000000000000000 ) ) ;
#14623=CIRCLE ( 'NONE', #17592, 3.000000000000002665 ) ;
#14624=ORIENTED_EDGE ( 'NONE', *, *, #27065, .T. ) ;
#14625=ADVANCED_FACE ( 'NONE', ( #29118 ), #634, .F. ) ;
#14626=CARTESIAN_POINT ( 'NONE',  ( -4.220252828340121276, -79.78402168683115292, 12.50000000000000000 ) ) ;
#14627=CARTESIAN_POINT ( 'NONE',  ( 0.000000000000000000, 0.000000000000000000, -5.000000000000000000 ) ) ;
#14629=FACE_OUTER_BOUND ( 'NONE', #30597, .T. ) ;
#14630=ORIENTED_EDGE ( 'NONE', *, *, #8054, .T. ) ;
#14631=CIRCLE ( 'NONE', #18857, 2.000000000000001776 ) ;
#14632=CARTESIAN_POINT ( 'NONE',  ( 69.99999662536839651, -3.469446951953614189E-15, -9.999999999999998224 ) ) ;
#14635=VECTOR ( 'NONE', #1658, 1000.000000000000000 ) ;
#14637=CIRCLE ( 'NONE', #31985, 2.000000000000001776 ) ;
#14638=ORIENTED_EDGE ( 'NONE', *, *, #17223, .T. ) ;
#14641=ORIENTED_EDGE ( 'NONE', *, *, #8729, .F. ) ;
#14642=DIRECTION ( 'NONE',  ( -1.000000000000000000, 0.000000000000000000, 0.000000000000000000 ) ) ;
#14643=DIRECTION ( 'NONE',  ( -0.000000000000000000, -0.000000000000000000, 1.000000000000000000 ) ) ;
#14644=CIRCLE ( 'NONE', #2068, 2.000000000000001776 ) ;
#14647=CIRCLE ( 'NONE', #31971, 2.000000000000001776 ) ;
#14648=ORIENTED_EDGE ( 'NONE', *, *, #22469, .T. ) ;
#14649=DIRECTION ( 'NONE',  ( -1.000000000000000000, 0.000000000000000000, 0.000000000000000000 ) ) ;
#14650=DIRECTION ( 'NONE',  ( 1.000000000000000000, 0.000000000000000000, 0.000000000000000000 ) ) ;
#14651=DIRECTION ( 'NONE',  ( 0.000000000000000000, 0.000000000000000000, -1.000000000000000000 ) ) ;
#14652=CIRCLE ( 'NONE', #872, 2.000000000000001776 ) ;
#14653=EDGE_CURVE ( 'NONE', #8095, #6666, #4513, .T. ) ;
#14654=ORIENTED_EDGE ( 'NONE', *, *, #4506, .F. ) ;
#14655=DIRECTION ( 'NONE',  ( 1.000000000000000000, 0.000000000000000000, 0.000000000000000000 ) ) ;
#14656=FACE_BOUND ( 'NONE', #1466, .T. ) ;
#14657=FACE_OUTER_BOUND ( 'NONE', #25871, .T. ) ;
#14658=DIRECTION ( 'NONE',  ( 1.000000000000000000, 0.000000000000000000, 0.000000000000000000 ) ) ;
#14659=CARTESIAN_POINT ( 'NONE',  ( -30.00000337463119848, -69.28203230275522628, -9.999999999999998224 ) ) ;
#14660=DIRECTION ( 'NONE',  ( 1.000000000000000000, 0.000000000000000000, 0.000000000000000000 ) ) ;
#14661=AXIS2_PLACEMENT_3D ( 'NONE', #36349, #10659, #22102 ) ;
#14662=AXIS2_PLACEMENT_3D ( 'NONE', #25792, #86, #5913 ) ;
#14664=EDGE_LOOP ( 'NONE', ( #16407, #26182, #20410, #22311 ) ) ;
#14665=CARTESIAN_POINT ( 'NONE',  ( 74.99999662536835388, -43.30127018922199511, 17.49999999999999645 ) ) ;
#14667=CARTESIAN_POINT ( 'NONE',  ( -10.00000337463128197, 86.60254037844397601, -5.000000000000000000 ) ) ;
#14668=ORIENTED_EDGE ( 'NONE', *, *, #27072, .F. ) ;
#14669=ORIENTED_EDGE ( 'NONE', *, *, #4373, .T. ) ;
#14672=AXIS2_PLACEMENT_3D ( 'NONE', #33849, #8161, #33257 ) ;
#14673=DIRECTION ( 'NONE',  ( -0.000000000000000000, -0.000000000000000000, 1.000000000000000000 ) ) ;
#14674=DIRECTION ( 'NONE',  ( 1.000000000000000000, 0.000000000000000000, 0.000000000000000000 ) ) ;
#14675=EDGE_CURVE ( 'NONE', #18489, #15126, #7208, .T. ) ;
#14676=AXIS2_PLACEMENT_3D ( 'NONE', #30071, #4781, #9823 ) ;
#14678=EDGE_LOOP ( 'NONE', ( #5108, #8187, #13339, #31520, #3077 ) ) ;
#14679=AXIS2_PLACEMENT_3D ( 'NONE', #22995, #11725, #2749 ) ;
#14681=AXIS2_PLACEMENT_3D ( 'NONE', #30000, #10306, #1695 ) ;
#14683=ORIENTED_EDGE ( 'NONE', *, *, #21755, .T. ) ;
#14685=EDGE_LOOP ( 'NONE', ( #31834, #3485, #9339, #15589 ) ) ;
#14686=EDGE_CURVE ( 'NONE', #10648, #25326, #10207, .T. ) ;
#14687=DIRECTION ( 'NONE',  ( -0.000000000000000000, -0.000000000000000000, 1.000000000000000000 ) ) ;
#14688=AXIS2_PLACEMENT_3D ( 'NONE', #29522, #14930, #17541 ) ;
#14690=ADVANCED_FACE ( 'NONE', ( #13139 ), #2255, .F. ) ;
#14691=CIRCLE ( 'NONE', #29049, 2.000000000000000000 ) ;
#14692=ORIENTED_EDGE ( 'NONE', *, *, #36365, .F. ) ;
#14693=VECTOR ( 'NONE', #17626, 1000.000000000000000 ) ;
#14695=CARTESIAN_POINT ( 'NONE',  ( 31.99999662536856704, 69.28203230275518365, 12.50000000000000000 ) ) ;
#14696=CARTESIAN_POINT ( 'NONE',  ( 27.78182860042856461, 56.67878100130339902, 12.49999999999999822 ) ) ;
#14699=ADVANCED_FACE ( 'NONE', ( #13689 ), #33582, .F. ) ;
#14701=ADVANCED_FACE ( 'NONE', ( #4891 ), #24593, .F. ) ;
#14702=CARTESIAN_POINT ( 'NONE',  ( -70.47608876694631874, -59.13646009116124702, -4.999999999999997335 ) ) ;
#14703=EDGE_CURVE ( 'NONE', #23803, #953, #28156, .T. ) ;
#14704=VECTOR ( 'NONE', #24041, 1000.000000000000000 ) ;
#14705=ORIENTED_EDGE ( 'NONE', *, *, #15078, .T. ) ;
#14706=DIRECTION ( 'NONE',  ( 1.000000000000000000, 0.000000000000000000, 0.000000000000000000 ) ) ;
#14707=CARTESIAN_POINT ( 'NONE',  ( 61.99999662536843914, -34.64101615137759893, -9.999999999999998224 ) ) ;
#14708=ADVANCED_FACE ( 'NONE', ( #11043 ), #7504, .F. ) ;
#14711=VECTOR ( 'NONE', #20304, 1000.000000000000000 ) ;
#14712=LINE ( 'NONE', #1022, #14194 ) ;
#14713=CARTESIAN_POINT ( 'NONE',  ( -2.000003374631289521, -69.28203230275519786, -9.999999999999998224 ) ) ;
#14714=CIRCLE ( 'NONE', #6327, 2.000000000000001776 ) ;
#14715=AXIS2_PLACEMENT_3D ( 'NONE', #11290, #6201, #5483 ) ;
#14717=DIRECTION ( 'NONE',  ( 0.000000000000000000, 0.000000000000000000, 1.000000000000000000 ) ) ;
#14718=AXIS2_PLACEMENT_3D ( 'NONE', #28421, #2568, #36695 ) ;
#14719=DIRECTION ( 'NONE',  ( 0.000000000000000000, 0.000000000000000000, -1.000000000000000000 ) ) ;
#14720=VERTEX_POINT ( 'NONE', #2445 ) ;
#14724=ORIENTED_EDGE ( 'NONE', *, *, #8819, .F. ) ;
#14725=AXIS2_PLACEMENT_3D ( 'NONE', #35740, #1797, #4419 ) ;
#14726=ORIENTED_EDGE ( 'NONE', *, *, #3219, .F. ) ;
#14727=ORIENTED_EDGE ( 'NONE', *, *, #28455, .T. ) ;
#14729=DIRECTION ( 'NONE',  ( 1.000000000000000000, 0.000000000000000000, 0.000000000000000000 ) ) ;
#14730=CARTESIAN_POINT ( 'NONE',  ( -40.00000337463113453, 69.28203230275516944, -9.999999999999998224 ) ) ;
#14731=VECTOR ( 'NONE', #24823, 1000.000000000000000 ) ;
#14732=VECTOR ( 'NONE', #24212, 1000.000000000000000 ) ;
#14733=LINE ( 'NONE', #12084, #6896 ) ;
#14735=CARTESIAN_POINT ( 'NONE',  ( -57.00000337463107059, 43.30127018922197379, 12.50000000000000000 ) ) ;
#14736=EDGE_LOOP ( 'NONE', ( #25870, #24314 ) ) ;
#14738=FACE_BOUND ( 'NONE', #29095, .T. ) ;
#14739=VECTOR ( 'NONE', #12862, 1000.000000000000000 ) ;
#14740=AXIS2_PLACEMENT_3D ( 'NONE', #1075, #699, #23405 ) ;
#14742=VECTOR ( 'NONE', #11013, 1000.000000000000000 ) ;
#14743=DIRECTION ( 'NONE',  ( 0.000000000000000000, 0.000000000000000000, 1.000000000000000000 ) ) ;
#14744=DIRECTION ( 'NONE',  ( 0.000000000000000000, 0.000000000000000000, 1.000000000000000000 ) ) ;
#14745=VERTEX_POINT ( 'NONE', #24952 ) ;
#14749=CARTESIAN_POINT ( 'NONE',  ( 58.48108235278871803, 36.97203788308964079, -4.999999999999997335 ) ) ;
#14751=DIRECTION ( 'NONE',  ( -1.000000000000000000, 0.000000000000000000, 0.000000000000000000 ) ) ;
#14752=EDGE_CURVE ( 'NONE', #14801, #2589, #29947, .T. ) ;
#14755=CARTESIAN_POINT ( 'NONE',  ( -65.00000337463102085, 25.98076211353317433, 12.50000000000000000 ) ) ;
#14756=DIRECTION ( 'NONE',  ( 0.000000000000000000, 0.000000000000000000, 1.000000000000000000 ) ) ;
#14757=AXIS2_PLACEMENT_3D ( 'NONE', #13004, #24646, #7019 ) ;
#14758=ORIENTED_EDGE ( 'NONE', *, *, #26266, .T. ) ;
#14759=ORIENTED_EDGE ( 'NONE', *, *, #25869, .T. ) ;
#14760=CIRCLE ( 'NONE', #24351, 33.00000000000001421 ) ;
#14761=ORIENTED_EDGE ( 'NONE', *, *, #3837, .F. ) ;
#14764=AXIS2_PLACEMENT_3D ( 'NONE', #15253, #18071, #29496 ) ;
#14765=CIRCLE ( 'NONE', #11180, 27.00000000000001066 ) ;
#14767=FACE_BOUND ( 'NONE', #18439, .T. ) ;
#14768=VECTOR ( 'NONE', #9697, 1000.000000000000000 ) ;
#14769=DIRECTION ( 'NONE',  ( 1.000000000000000000, 0.000000000000000000, 0.000000000000000000 ) ) ;
#14770=DIRECTION ( 'NONE',  ( -0.000000000000000000, -0.000000000000000000, 1.000000000000000000 ) ) ;
#14771=CYLINDRICAL_SURFACE ( 'NONE', #8252, 45.00000000000000711 ) ;
#14772=ADVANCED_FACE ( 'NONE', ( #22310 ), #33751, .F. ) ;
#14774=EDGE_CURVE ( 'NONE', #26082, #2567, #611, .T. ) ;
#14775=EDGE_LOOP ( 'NONE', ( #28623, #11778, #15447, #29956 ) ) ;
#14776=CIRCLE ( 'NONE', #24372, 2.000000000000001776 ) ;
#14777=ORIENTED_EDGE ( 'NONE', *, *, #13468, .T. ) ;
#14778=CARTESIAN_POINT ( 'NONE',  ( 17.99999662536858125, 86.60254037844397601, -9.999999999999998224 ) ) ;
#14779=CARTESIAN_POINT ( 'NONE',  ( -20.00000337463122690, 86.60254037844397601, -5.000000000000000000 ) ) ;
#14780=CYLINDRICAL_SURFACE ( 'NONE', #27489, 2.000000000000001776 ) ;
#14781=ORIENTED_EDGE ( 'NONE', *, *, #23863, .F. ) ;
#14784=AXIS2_PLACEMENT_3D ( 'NONE', #16853, #28273, #14016 ) ;
#14785=FACE_BOUND ( 'NONE', #27085, .T. ) ;
#14786=ORIENTED_EDGE ( 'NONE', *, *, #28820, .T. ) ;
#14787=ORIENTED_EDGE ( 'NONE', *, *, #12252, .F. ) ;
#14788=CIRCLE ( 'NONE', #33972, 2.000000000000001776 ) ;
#14789=ORIENTED_EDGE ( 'NONE', *, *, #21711, .T. ) ;
#14791=VERTEX_POINT ( 'NONE', #5806 ) ;
#14794=VECTOR ( 'NONE', #8260, 1000.000000000000000 ) ;
#14796=CARTESIAN_POINT ( 'NONE',  ( -20.00000337463123756, -86.60254037844400443, 17.49999999999999645 ) ) ;
#14797=ADVANCED_FACE ( 'NONE', ( #11965 ), #15385, .F. ) ;
#14798=ORIENTED_EDGE ( 'NONE', *, *, #4870, .F. ) ;
#14799=ORIENTED_EDGE ( 'NONE', *, *, #26117, .T. ) ;
#14800=AXIS2_PLACEMENT_3D ( 'NONE', #27669, #1428, #24690 ) ;
#14801=VERTEX_POINT ( 'NONE', #8983 ) ;
#14803=EDGE_LOOP ( 'NONE', ( #15727, #11431, #3873, #18274 ) ) ;
#14805=CARTESIAN_POINT ( 'NONE',  ( -52.39915983220772233, -35.19434990244957362, 12.49999999999999822 ) ) ;
#14806=DIRECTION ( 'NONE',  ( 0.000000000000000000, 0.000000000000000000, 1.000000000000000000 ) ) ;
#14807=ORIENTED_EDGE ( 'NONE', *, *, #7609, .T. ) ;
#14808=DIRECTION ( 'NONE',  ( 0.000000000000000000, 0.000000000000000000, 1.000000000000000000 ) ) ;
#14809=CIRCLE ( 'NONE', #11795, 2.000000000000000000 ) ;
#14811=DIRECTION ( 'NONE',  ( 0.000000000000000000, 0.000000000000000000, 1.000000000000000000 ) ) ;
#14812=ORIENTED_EDGE ( 'NONE', *, *, #13082, .T. ) ;
#14813=DIRECTION ( 'NONE',  ( 0.000000000000000000, 0.000000000000000000, 1.000000000000000000 ) ) ;
#14814=VECTOR ( 'NONE', #13452, 1000.000000000000000 ) ;
#14816=AXIS2_PLACEMENT_3D ( 'NONE', #15221, #29853, #32088 ) ;
#14817=EDGE_CURVE ( 'NONE', #20602, #8231, #2370, .T. ) ;
#14819=ORIENTED_EDGE ( 'NONE', *, *, #19696, .F. ) ;
#14821=CARTESIAN_POINT ( 'NONE',  ( -10.00000337463125000, -86.60254037844400443, -9.999999999999998224 ) ) ;
#14822=ADVANCED_FACE ( 'NONE', ( #22865, #31824, #14241, #22686, #14591, #26032, #5996, #338, #17420, #5445, #2808, #26230, #6155, #23036, #25490, #17246, #17042, #3000, #11772, #28670, #25691, #25861, #31287, #33939, #34301, #17586, #5607, #28474, #11241, #8254, #8604, #20037, #31465, #16871, #151, #29014, #3347, #2612, #36931, #14785, #19688, #28836, #34135, #8436, #20236, #31659, #26584, #714, #20575, #29966, #12125, #7101, #21148, #3722, #20775, #4103, #32000, #32578, #18546, #27138, #4285, #17780, #9715, #32401, #29402, #15716, #1452, #9338, #15149, #9897, #24149, #9540, #6339, #9146, #898, #14982, #23419, #12698, #29217, #12318, #3547, #32212, #34853, #23791, #21336, #6543, #17977, #23590, #26411, #35242, #20973, #6716 ), #35033, .F. ) ;
#14823=VERTEX_POINT ( 'NONE', #18147 ) ;
#14824=CIRCLE ( 'NONE', #7045, 2.000000000000001776 ) ;
#14825=ORIENTED_EDGE ( 'NONE', *, *, #30883, .T. ) ;
#14828=CARTESIAN_POINT ( 'NONE',  ( -50.00000337463110611, -69.28203230275519786, -9.999999999999998224 ) ) ;
#14829=FACE_OUTER_BOUND ( 'NONE', #15877, .T. ) ;
#14831=EDGE_CURVE ( 'NONE', #30141, #10592, #29570, .T. ) ;
#14832=VERTEX_POINT ( 'NONE', #15338 ) ;
#14833=AXIS2_PLACEMENT_3D ( 'NONE', #30840, #13409, #31046 ) ;
#14834=DIRECTION ( 'NONE',  ( 0.000000000000000000, 0.000000000000000000, 1.000000000000000000 ) ) ;
#14836=DIRECTION ( 'NONE',  ( 1.000000000000000000, 0.000000000000000000, 0.000000000000000000 ) ) ;
#14838=CIRCLE ( 'NONE', #10056, 3.499999999999991562 ) ;
#14839=ORIENTED_EDGE ( 'NONE', *, *, #11263, .F. ) ;
#14840=AXIS2_PLACEMENT_3D ( 'NONE', #35185, #35385, #13028 ) ;
#14841=AXIS2_PLACEMENT_3D ( 'NONE', #15603, #18779, #32850 ) ;
#14842=DIRECTION ( 'NONE',  ( -1.000000000000000000, 0.000000000000000000, 0.000000000000000000 ) ) ;
#14843=VERTEX_POINT ( 'NONE', #35427 ) ;
#14844=CARTESIAN_POINT ( 'NONE',  ( -62.97617850287781494, -4.279621169095772615, -4.999999999999997335 ) ) ;
#14845=DIRECTION ( 'NONE',  ( -0.000000000000000000, -0.000000000000000000, 1.000000000000000000 ) ) ;
#14846=AXIS2_PLACEMENT_3D ( 'NONE', #31360, #3074, #5686 ) ;
#14848=ORIENTED_EDGE ( 'NONE', *, *, #15713, .T. ) ;
#14849=ORIENTED_EDGE ( 'NONE', *, *, #5637, .F. ) ;
#14851=DIRECTION ( 'NONE',  ( 0.000000000000000000, 0.000000000000000000, -1.000000000000000000 ) ) ;
#14852=CARTESIAN_POINT ( 'NONE',  ( 84.99999662536831124, -25.98076211353319565, 17.49999999999999645 ) ) ;
#14853=EDGE_CURVE ( 'NONE', #7448, #24238, #34699, .T. ) ;
#14854=VERTEX_POINT ( 'NONE', #26967 ) ;
#14855=CARTESIAN_POINT ( 'NONE',  ( -38.00000337463113453, 69.28203230275516944, -9.999999999999998224 ) ) ;
#14856=FACE_BOUND ( 'NONE', #17088, .T. ) ;
#14857=DIRECTION ( 'NONE',  ( 0.000000000000000000, 0.000000000000000000, 1.000000000000000000 ) ) ;
#14859=CIRCLE ( 'NONE', #3498, 33.00000000000001421 ) ;
#14860=DIRECTION ( 'NONE',  ( 1.000000000000000000, 0.000000000000000000, 0.000000000000000000 ) ) ;
#14861=CARTESIAN_POINT ( 'NONE',  ( -47.00000337463111322, 77.94228634059959404, 17.49999999999999645 ) ) ;
#14862=EDGE_CURVE ( 'NONE', #26322, #31694, #20317, .T. ) ;
#14863=CARTESIAN_POINT ( 'NONE',  ( -30.00000337463119848, -69.28203230275522628, 12.50000000000000000 ) ) ;
#14864=AXIS2_PLACEMENT_3D ( 'NONE', #27056, #7203, #4377 ) ;
#14865=EDGE_CURVE ( 'NONE', #2856, #10704, #16132, .T. ) ;
#14867=ORIENTED_EDGE ( 'NONE', *, *, #32370, .F. ) ;
#14868=CARTESIAN_POINT ( 'NONE',  ( -12.00000337463127842, -69.28203230275519786, -5.000000000000000000 ) ) ;
#14870=CARTESIAN_POINT ( 'NONE',  ( 84.99999662536831124, -8.660254037844397956, 17.49999999999999645 ) ) ;
#14871=DIRECTION ( 'NONE',  ( 0.000000000000000000, 0.000000000000000000, 1.000000000000000000 ) ) ;
#14872=AXIS2_PLACEMENT_3D ( 'NONE', #271, #23161, #34614 ) ;
#14873=EDGE_LOOP ( 'NONE', ( #23555, #32106, #28690, #11243 ) ) ;
#14874=ORIENTED_EDGE ( 'NONE', *, *, #32287, .F. ) ;
#14875=VERTEX_POINT ( 'NONE', #30877 ) ;
#14879=LINE ( 'NONE', #11672, #17228 ) ;
#14880=ORIENTED_EDGE ( 'NONE', *, *, #5467, .T. ) ;
#14882=AXIS2_PLACEMENT_3D ( 'NONE', #13686, #13482, #24945 ) ;
#14883=CIRCLE ( 'NONE', #37058, 2.000000000000001776 ) ;
#14884=DIRECTION ( 'NONE',  ( 1.000000000000000000, 0.000000000000000000, 0.000000000000000000 ) ) ;
#14885=EDGE_CURVE ( 'NONE', #29836, #8231, #27529, .T. ) ;
#14886=ORIENTED_EDGE ( 'NONE', *, *, #36392, .F. ) ;
#14887=CARTESIAN_POINT ( 'NONE',  ( 84.99999662536832545, 25.98076211353319565, 12.50000000000000000 ) ) ;
#14889=CYLINDRICAL_SURFACE ( 'NONE', #11166, 2.000000000000001776 ) ;
#14890=ORIENTED_EDGE ( 'NONE', *, *, #14675, .F. ) ;
#14891=EDGE_LOOP ( 'NONE', ( #31018, #35029 ) ) ;
#14892=CYLINDRICAL_SURFACE ( 'NONE', #20208, 2.000000000000001776 ) ;
#14894=AXIS2_PLACEMENT_3D ( 'NONE', #5617, #13874, #5454 ) ;
#14897=LINE ( 'NONE', #6088, #23277 ) ;
#14898=AXIS2_PLACEMENT_3D ( 'NONE', #12227, #6459, #34405 ) ;
#14900=DIRECTION ( 'NONE',  ( 0.000000000000000000, 0.000000000000000000, 1.000000000000000000 ) ) ;
#14902=EDGE_LOOP ( 'NONE', ( #22785, #22324, #19713, #16900 ) ) ;
#14903=DIRECTION ( 'NONE',  ( 0.000000000000000000, 0.000000000000000000, 1.000000000000000000 ) ) ;
#14904=DIRECTION ( 'NONE',  ( 1.000000000000000000, 0.000000000000000000, 0.000000000000000000 ) ) ;
#14905=VECTOR ( 'NONE', #20323, 1000.000000000000000 ) ;
#14907=EDGE_CURVE ( 'NONE', #10548, #27983, #23320, .T. ) ;
#14909=DIRECTION ( 'NONE',  ( 0.000000000000000000, 0.000000000000000000, 1.000000000000000000 ) ) ;
#14910=CARTESIAN_POINT ( 'NONE',  ( 34.99999662536853862, 77.94228634059959404, -5.000000000000000000 ) ) ;
#14911=CIRCLE ( 'NONE', #1150, 2.000000000000001776 ) ;
#14912=DIRECTION ( 'NONE',  ( 0.000000000000000000, 0.000000000000000000, -1.000000000000000000 ) ) ;
#14914=VECTOR ( 'NONE', #8941, 1000.000000000000000 ) ;
#14915=LINE ( 'NONE', #26351, #32273 ) ;
#14916=CARTESIAN_POINT ( 'NONE',  ( 0.000000000000000000, 0.000000000000000000, -5.000000000000000000 ) ) ;
#14917=EDGE_LOOP ( 'NONE', ( #13110, #10551, #29234, #10272 ) ) ;
#14918=DIRECTION ( 'NONE',  ( 1.000000000000000000, 0.000000000000000000, 0.000000000000000000 ) ) ;
#14919=EDGE_CURVE ( 'NONE', #23244, #33319, #27492, .T. ) ;
#14920=CYLINDRICAL_SURFACE ( 'NONE', #26679, 2.000000000000001776 ) ;
#14921=DIRECTION ( 'NONE',  ( 1.000000000000000000, 0.000000000000000000, 0.000000000000000000 ) ) ;
#14923=ORIENTED_EDGE ( 'NONE', *, *, #36839, .T. ) ;
#14925=ORIENTED_EDGE ( 'NONE', *, *, #3531, .T. ) ;
#14926=AXIS2_PLACEMENT_3D ( 'NONE', #28438, #34455, #9303 ) ;
#14929=AXIS2_PLACEMENT_3D ( 'NONE', #7663, #18909, #33550 ) ;
#14930=DIRECTION ( 'NONE',  ( 0.000000000000000000, 0.000000000000000000, 1.000000000000000000 ) ) ;
#14931=ADVANCED_FACE ( 'NONE', ( #4464 ), #15900, .F. ) ;
#14932=EDGE_CURVE ( 'NONE', #15986, #22847, #24903, .T. ) ;
#14934=LINE ( 'NONE', #23378, #301 ) ;
#14935=ORIENTED_EDGE ( 'NONE', *, *, #3345, .F. ) ;
#14936=EDGE_CURVE ( 'NONE', #23602, #9228, #28105, .T. ) ;
#14937=CIRCLE ( 'NONE', #18527, 33.00000000000001421 ) ;
#14938=EDGE_CURVE ( 'NONE', #7360, #32425, #19706, .T. ) ;
#14939=DIRECTION ( 'NONE',  ( 0.000000000000000000, 0.000000000000000000, -1.000000000000000000 ) ) ;
#14940=ORIENTED_EDGE ( 'NONE', *, *, #17840, .T. ) ;
#14941=FACE_BOUND ( 'NONE', #26413, .T. ) ;
#14942=AXIS2_PLACEMENT_3D ( 'NONE', #24713, #36532, #27134 ) ;
#14943=AXIS2_PLACEMENT_3D ( 'NONE', #16411, #36110, #36295 ) ;
#14945=DIRECTION ( 'NONE',  ( 0.000000000000000000, 0.000000000000000000, 1.000000000000000000 ) ) ;
#14946=CIRCLE ( 'NONE', #35914, 27.00000000000001066 ) ;
#14947=VERTEX_POINT ( 'NONE', #13090 ) ;
#14950=CARTESIAN_POINT ( 'NONE',  ( -93.36492675454779544, -17.14523346298311779, 12.49999999999999822 ) ) ;
#14951=CIRCLE ( 'NONE', #28114, 95.00000000000001421 ) ;
#14952=DIRECTION ( 'NONE',  ( 0.000000000000000000, 0.000000000000000000, 1.000000000000000000 ) ) ;
#14953=DIRECTION ( 'NONE',  ( 1.000000000000000000, 0.000000000000000000, 0.000000000000000000 ) ) ;
#14955=CARTESIAN_POINT ( 'NONE',  ( 19.99999662536861678, -86.60254037844400443, 12.50000000000000000 ) ) ;
#14956=AXIS2_PLACEMENT_3D ( 'NONE', #1062, #23756, #32545 ) ;
#14957=CARTESIAN_POINT ( 'NONE',  ( 47.99999662536846756, 51.96152422706637708, 17.49999999999999645 ) ) ;
#14958=CARTESIAN_POINT ( 'NONE',  ( -38.00000337463113453, 69.28203230275516944, -5.000000000000000000 ) ) ;
#14959=ORIENTED_EDGE ( 'NONE', *, *, #3802, .F. ) ;
#14960=VERTEX_POINT ( 'NONE', #7656 ) ;
#14962=DIRECTION ( 'NONE',  ( 1.000000000000000000, 0.000000000000000000, 0.000000000000000000 ) ) ;
#14963=AXIS2_PLACEMENT_3D ( 'NONE', #14887, #17684, #28929 ) ;
#14964=DIRECTION ( 'NONE',  ( 1.000000000000000000, 0.000000000000000000, 0.000000000000000000 ) ) ;
#14965=AXIS2_PLACEMENT_3D ( 'NONE', #12166, #18016, #15756 ) ;
#14966=DIRECTION ( 'NONE',  ( 0.000000000000000000, 0.000000000000000000, 1.000000000000000000 ) ) ;
#14968=CARTESIAN_POINT ( 'NONE',  ( -8.000003374631281972, 86.60254037844397601, 17.49999999999999645 ) ) ;
#14969=AXIS2_PLACEMENT_3D ( 'NONE', #3774, #29638, #18778 ) ;
#14971=ORIENTED_EDGE ( 'NONE', *, *, #17630, .F. ) ;
#14972=EDGE_CURVE ( 'NONE', #9610, #33654, #26285, .T. ) ;
#14973=ORIENTED_EDGE ( 'NONE', *, *, #7147, .T. ) ;
#14974=DIRECTION ( 'NONE',  ( 0.000000000000000000, 0.000000000000000000, 1.000000000000000000 ) ) ;
#14975=ADVANCED_FACE ( 'NONE', ( #22270 ), #33708, .F. ) ;
#14977=CARTESIAN_POINT ( 'NONE',  ( 59.99999662536843914, -34.64101615137759893, 17.49999999999999645 ) ) ;
#14978=EDGE_CURVE ( 'NONE', #21597, #17068, #6535, .T. ) ;
#14979=DIRECTION ( 'NONE',  ( 0.000000000000000000, 0.000000000000000000, 1.000000000000000000 ) ) ;
#14980=ORIENTED_EDGE ( 'NONE', *, *, #29456, .T. ) ;
#14981=AXIS2_PLACEMENT_3D ( 'NONE', #13406, #36307, #4434 ) ;
#14982=FACE_BOUND ( 'NONE', #29652, .T. ) ;
#14983=ORIENTED_EDGE ( 'NONE', *, *, #24, .T. ) ;
#14984=ORIENTED_EDGE ( 'NONE', *, *, #5939, .T. ) ;
#14985=FACE_OUTER_BOUND ( 'NONE', #14775, .T. ) ;
#14986=VERTEX_POINT ( 'NONE', #18902 ) ;
#14987=AXIS2_PLACEMENT_3D ( 'NONE', #539, #8792, #34685 ) ;
#14989=CARTESIAN_POINT ( 'NONE',  ( -60.00000337463104216, 51.96152422706639129, -5.000000000000000000 ) ) ;
#14990=CARTESIAN_POINT ( 'NONE',  ( -83.00000337463092137, 25.98076211353317433, -9.999999999999998224 ) ) ;
#14992=CIRCLE ( 'NONE', #25185, 2.000000000000001776 ) ;
#14994=ORIENTED_EDGE ( 'NONE', *, *, #30271, .T. ) ;
#14995=AXIS2_PLACEMENT_3D ( 'NONE', #11793, #28496, #2830 ) ;
#14997=EDGE_CURVE ( 'NONE', #18549, #5127, #11327, .T. ) ;
#14998=VERTEX_POINT ( 'NONE', #13269 ) ;
#14999=ORIENTED_EDGE ( 'NONE', *, *, #26266, .F. ) ;
#15001=CARTESIAN_POINT ( 'NONE',  ( -3.374631334790434423E-06, 69.28203230275516944, 12.50000000000000000 ) ) ;
#15003=CARTESIAN_POINT ( 'NONE',  ( -38.00000337463113453, -69.28203230275519786, 12.50000000000000000 ) ) ;
#15006=ORIENTED_EDGE ( 'NONE', *, *, #3108, .F. ) ;
#15007=LINE ( 'NONE', #741, #29007 ) ;
#15008=LINE ( 'NONE', #6371, #13201 ) ;
#15011=DIRECTION ( 'NONE',  ( 1.000000000000000000, 0.000000000000000000, 0.000000000000000000 ) ) ;
#15012=DIRECTION ( 'NONE',  ( 0.000000000000000000, 0.000000000000000000, 1.000000000000000000 ) ) ;
#15013=ORIENTED_EDGE ( 'NONE', *, *, #16130, .T. ) ;
#15014=EDGE_LOOP ( 'NONE', ( #37023, #26033, #30863, #1309, #22704 ) ) ;
#15015=CARTESIAN_POINT ( 'NONE',  ( -20.00000337463123756, -69.28203230275522628, 12.50000000000000000 ) ) ;
#15016=DIRECTION ( 'NONE',  ( -0.000000000000000000, 0.000000000000000000, -1.000000000000000000 ) ) ;
#15017=AXIS2_PLACEMENT_3D ( 'NONE', #33164, #4693, #5038 ) ;
#15018=ADVANCED_FACE ( 'NONE', ( #25995 ), #34643, .F. ) ;
#15019=DIRECTION ( 'NONE',  ( 0.000000000000000000, 0.000000000000000000, 1.000000000000000000 ) ) ;
#15021=ORIENTED_EDGE ( 'NONE', *, *, #27063, .F. ) ;
#15023=DIRECTION ( 'NONE',  ( 0.000000000000000000, 0.000000000000000000, 1.000000000000000000 ) ) ;
#15024=ORIENTED_EDGE ( 'NONE', *, *, #16057, .T. ) ;
#15025=CARTESIAN_POINT ( 'NONE',  ( 1.999996625368665182, 69.28203230275516944, -9.999999999999998224 ) ) ;
#15026=ORIENTED_EDGE ( 'NONE', *, *, #1173, .F. ) ;
#15027=DIRECTION ( 'NONE',  ( 1.000000000000000000, 0.000000000000000000, 0.000000000000000000 ) ) ;
#15028=CARTESIAN_POINT ( 'NONE',  ( -3.374631289687624047E-06, -69.28203230275519786, 17.49999999999999645 ) ) ;
#15029=EDGE_CURVE ( 'NONE', #5584, #2344, #2959, .T. ) ;
#15031=ORIENTED_EDGE ( 'NONE', *, *, #24319, .F. ) ;
#15032=EDGE_LOOP ( 'NONE', ( #20975, #36001, #12621, #11335, #21480, #21624 ) ) ;
#15033=CARTESIAN_POINT ( 'NONE',  ( 71.99999662536839651, -3.469446951953614189E-15, 17.49999999999999645 ) ) ;
#15034=ADVANCED_FACE ( 'NONE', ( #20375 ), #6120, .F. ) ;
#15036=DIRECTION ( 'NONE',  ( 0.000000000000000000, 0.000000000000000000, -1.000000000000000000 ) ) ;
#15037=ORIENTED_EDGE ( 'NONE', *, *, #16072, .T. ) ;
#15039=FACE_BOUND ( 'NONE', #4486, .T. ) ;
#15040=EDGE_CURVE ( 'NONE', #36323, #31133, #13998, .T. ) ;
#15041=LINE ( 'NONE', #34919, #29203 ) ;
#15042=CYLINDRICAL_SURFACE ( 'NONE', #12682, 2.000000000000001776 ) ;
#15043=CARTESIAN_POINT ( 'NONE',  ( 31.83425564451589196, 89.42901512340320380, 12.49999999999999822 ) ) ;
#15044=ORIENTED_EDGE ( 'NONE', *, *, #21655, .T. ) ;
#15045=DIRECTION ( 'NONE',  ( 1.000000000000000000, 0.000000000000000000, 0.000000000000000000 ) ) ;
#15046=FACE_OUTER_BOUND ( 'NONE', #15806, .T. ) ;
#15047=EDGE_CURVE ( 'NONE', #21277, #5475, #11901, .T. ) ;
#15048=ORIENTED_EDGE ( 'NONE', *, *, #28585, .T. ) ;
#15050=FACE_BOUND ( 'NONE', #14013, .T. ) ;
#15051=FACE_OUTER_BOUND ( 'NONE', #2704, .T. ) ;
#15054=ORIENTED_EDGE ( 'NONE', *, *, #20614, .T. ) ;
#15055=DIRECTION ( 'NONE',  ( 1.000000000000000000, 0.000000000000000000, 0.000000000000000000 ) ) ;
#15056=EDGE_CURVE ( 'NONE', #8634, #33684, #37083, .T. ) ;
#15057=CARTESIAN_POINT ( 'NONE',  ( 54.99999662536844625, 60.62177826491077326, -9.999999999999998224 ) ) ;
#15058=CARTESIAN_POINT ( 'NONE',  ( 9.999996625368625658, 86.60254037844397601, 17.49999999999999645 ) ) ;
#15060=CIRCLE ( 'NONE', #24035, 2.000000000000001776 ) ;
#15061=VERTEX_POINT ( 'NONE', #14192 ) ;
#15062=EDGE_LOOP ( 'NONE', ( #32817, #31288 ) ) ;
#15066=ORIENTED_EDGE ( 'NONE', *, *, #9426, .T. ) ;
#15069=ORIENTED_EDGE ( 'NONE', *, *, #34579, .F. ) ;
#15071=CARTESIAN_POINT ( 'NONE',  ( 69.99999662536838230, -51.96152422706639840, 17.49999999999999645 ) ) ;
#15075=ORIENTED_EDGE ( 'NONE', *, *, #28204, .F. ) ;
#15076=ORIENTED_EDGE ( 'NONE', *, *, #9265, .T. ) ;
#15078=EDGE_CURVE ( 'NONE', #31695, #25696, #20912, .T. ) ;
#15079=PLANE ( 'NONE',  #6314 ) ;
#15080=DIRECTION ( 'NONE',  ( 0.000000000000000000, 0.000000000000000000, -1.000000000000000000 ) ) ;
#15081=EDGE_LOOP ( 'NONE', ( #25415, #30657, #15085, #9189 ) ) ;
#15082=CARTESIAN_POINT ( 'NONE',  ( -4.279621169095561228, 62.97617850287782915, 12.49999999999999822 ) ) ;
#15084=AXIS2_PLACEMENT_3D ( 'NONE', #9254, #20691, #4215 ) ;
#15085=ORIENTED_EDGE ( 'NONE', *, *, #32287, .T. ) ;
#15086=DIRECTION ( 'NONE',  ( -1.000000000000000000, 0.000000000000000000, 0.000000000000000000 ) ) ;
#15087=EDGE_CURVE ( 'NONE', #35287, #14947, #25706, .T. ) ;
#15088=DIRECTION ( 'NONE',  ( 0.000000000000000000, 0.000000000000000000, 1.000000000000000000 ) ) ;
#15089=DIRECTION ( 'NONE',  ( 0.000000000000000000, 0.000000000000000000, 1.000000000000000000 ) ) ;
#15090=CARTESIAN_POINT ( 'NONE',  ( -20.00000337463124112, 69.28203230275516944, -5.000000000000000000 ) ) ;
#15091=FACE_OUTER_BOUND ( 'NONE', #33906, .T. ) ;
#15092=EDGE_CURVE ( 'NONE', #32017, #598, #30493, .T. ) ;
#15093=DIRECTION ( 'NONE',  ( 1.000000000000000000, 0.000000000000000000, 0.000000000000000000 ) ) ;
#15094=ORIENTED_EDGE ( 'NONE', *, *, #9161, .T. ) ;
#15098=ORIENTED_EDGE ( 'NONE', *, *, #28842, .T. ) ;
#15099=EDGE_LOOP ( 'NONE', ( #20794, #18093 ) ) ;
#15100=ORIENTED_EDGE ( 'NONE', *, *, #32489, .F. ) ;
#15102=DIRECTION ( 'NONE',  ( 0.000000000000000000, 0.000000000000000000, -1.000000000000000000 ) ) ;
#15103=CARTESIAN_POINT ( 'NONE',  ( -73.00000337463097821, 25.98076211353318854, 12.50000000000000000 ) ) ;
#15105=CIRCLE ( 'NONE', #15700, 2.000000000000000000 ) ;
#15106=DIRECTION ( 'NONE',  ( 1.000000000000000000, 0.000000000000000000, 0.000000000000000000 ) ) ;
#15107=ORIENTED_EDGE ( 'NONE', *, *, #15567, .T. ) ;
#15108=CYLINDRICAL_SURFACE ( 'NONE', #27544, 2.000000000000001776 ) ;
#15109=VERTEX_POINT ( 'NONE', #2577 ) ;
#15110=FACE_BOUND ( 'NONE', #1608, .T. ) ;
#15111=EDGE_CURVE ( 'NONE', #18148, #24065, #28628, .T. ) ;
#15112=DIRECTION ( 'NONE',  ( 0.000000000000000000, 0.000000000000000000, 1.000000000000000000 ) ) ;
#15113=EDGE_CURVE ( 'NONE', #33091, #5840, #23919, .T. ) ;
#15114=DIRECTION ( 'NONE',  ( 0.000000000000000000, 0.000000000000000000, 1.000000000000000000 ) ) ;
#15116=EDGE_LOOP ( 'NONE', ( #29943, #3910, #36281, #31832, #16982 ) ) ;
#15117=DIRECTION ( 'NONE',  ( 0.000000000000000000, 0.000000000000000000, 1.000000000000000000 ) ) ;
#15118=DIRECTION ( 'NONE',  ( 0.000000000000000000, 0.000000000000000000, -1.000000000000000000 ) ) ;
#15119=AXIS2_PLACEMENT_3D ( 'NONE', #24625, #21782, #27419 ) ;
#15120=CARTESIAN_POINT ( 'NONE',  ( -68.00000337463102085, -51.96152422706641971, 17.49999999999999645 ) ) ;
#15121=CARTESIAN_POINT ( 'NONE',  ( -31.00000000000027356, -58.88972745734168512, 12.49999999999999822 ) ) ;
#15122=EDGE_LOOP ( 'NONE', ( #10259, #23034, #2929, #12161 ) ) ;
#15123=CYLINDRICAL_SURFACE ( 'NONE', #10640, 2.000000000000001776 ) ;
#15124=CARTESIAN_POINT ( 'NONE',  ( -37.00000337463116296, 77.94228634059957983, 12.50000000000000000 ) ) ;
#15125=CARTESIAN_POINT ( 'NONE',  ( 7.999996625368656744, -86.60254037844400443, -9.999999999999998224 ) ) ;
#15126=VERTEX_POINT ( 'NONE', #23001 ) ;
#15127=VERTEX_POINT ( 'NONE', #34445 ) ;
#15129=CIRCLE ( 'NONE', #22899, 2.000000000000001776 ) ;
#15130=ORIENTED_EDGE ( 'NONE', *, *, #11736, .F. ) ;
#15132=DIRECTION ( 'NONE',  ( 0.000000000000000000, 0.000000000000000000, 1.000000000000000000 ) ) ;
#15133=DIRECTION ( 'NONE',  ( 0.000000000000000000, 0.000000000000000000, 1.000000000000000000 ) ) ;
#15134=DIRECTION ( 'NONE',  ( -1.000000000000000000, 0.000000000000000000, 0.000000000000000000 ) ) ;
#15135=DIRECTION ( 'NONE',  ( 0.000000000000000000, 0.000000000000000000, -1.000000000000000000 ) ) ;
#15136=CARTESIAN_POINT ( 'NONE',  ( 91.99999662536828282, 0.000000000000000000, -9.999999999999998224 ) ) ;
#15137=FACE_OUTER_BOUND ( 'NONE', #20577, .T. ) ;
#15139=ORIENTED_EDGE ( 'NONE', *, *, #31979, .F. ) ;
#15140=AXIS2_PLACEMENT_3D ( 'NONE', #27002, #6749, #24585 ) ;
#15142=EDGE_CURVE ( 'NONE', #20452, #27221, #16771, .T. ) ;
#15144=ORIENTED_EDGE ( 'NONE', *, *, #21138, .T. ) ;
#15149=FACE_BOUND ( 'NONE', #26947, .T. ) ;
#15150=ORIENTED_EDGE ( 'NONE', *, *, #14222, .T. ) ;
#15151=AXIS2_PLACEMENT_3D ( 'NONE', #19472, #33913, #9270 ) ;
#15152=ORIENTED_EDGE ( 'NONE', *, *, #22780, .T. ) ;
#15153=EDGE_CURVE ( 'NONE', #8725, #25751, #29923, .T. ) ;
#15154=CARTESIAN_POINT ( 'NONE',  ( -65.63757354697304436, -58.72612421542294925, 12.50000000000000000 ) ) ;
#15157=CARTESIAN_POINT ( 'NONE',  ( -53.72397537678465085, -62.16182779291699489, -5.000000000000000000 ) ) ;
#15158=DIRECTION ( 'NONE',  ( 1.000000000000000000, 0.000000000000000000, 0.000000000000000000 ) ) ;
#15162=CIRCLE ( 'NONE', #787, 2.000000000000001776 ) ;
#15164=EDGE_LOOP ( 'NONE', ( #16873, #21633, #19541, #36821 ) ) ;
#15165=EDGE_CURVE ( 'NONE', #8516, #8626, #9683, .T. ) ;
#15166=ORIENTED_EDGE ( 'NONE', *, *, #27848, .F. ) ;
#15167=CIRCLE ( 'NONE', #28917, 2.000000000000001776 ) ;
#15168=VERTEX_POINT ( 'NONE', #32368 ) ;
#15169=ADVANCED_FACE ( 'NONE', ( #15498 ), #9292, .F. ) ;
#15170=DIRECTION ( 'NONE',  ( 1.000000000000000000, 0.000000000000000000, 0.000000000000000000 ) ) ;
#15171=EDGE_CURVE ( 'NONE', #20878, #9729, #32166, .T. ) ;
#15172=DIRECTION ( 'NONE',  ( 0.000000000000000000, 0.000000000000000000, 1.000000000000000000 ) ) ;
#15173=ORIENTED_EDGE ( 'NONE', *, *, #16134, .F. ) ;
#15176=DIRECTION ( 'NONE',  ( 1.000000000000000000, 0.000000000000000000, 0.000000000000000000 ) ) ;
#15177=ORIENTED_EDGE ( 'NONE', *, *, #28307, .F. ) ;
#15178=DIRECTION ( 'NONE',  ( 0.000000000000000000, 0.000000000000000000, 1.000000000000000000 ) ) ;
#15180=CARTESIAN_POINT ( 'NONE',  ( -56.67878100130369035, 27.78182860042797131, -4.999999999999997335 ) ) ;
#15181=VECTOR ( 'NONE', #35668, 1000.000000000000000 ) ;
#15182=CYLINDRICAL_SURFACE ( 'NONE', #18837, 2.000000000000001776 ) ;
#15183=ORIENTED_EDGE ( 'NONE', *, *, #20159, .T. ) ;
#15184=DIRECTION ( 'NONE',  ( 0.000000000000000000, 0.000000000000000000, 1.000000000000000000 ) ) ;
#15185=DIRECTION ( 'NONE',  ( -1.000000000000000000, 0.000000000000000000, 0.000000000000000000 ) ) ;
#15186=AXIS2_PLACEMENT_3D ( 'NONE', #18479, #7033, #15476 ) ;
#15187=EDGE_LOOP ( 'NONE', ( #4956, #7090, #32577, #8043 ) ) ;
#15188=ORIENTED_EDGE ( 'NONE', *, *, #16743, .F. ) ;
#15189=CARTESIAN_POINT ( 'NONE',  ( -20.00000337463123756, -86.60254037844400443, -9.999999999999998224 ) ) ;
#15190=CARTESIAN_POINT ( 'NONE',  ( -83.49774789488644444, 24.66044833507834610, 12.50000000000000000 ) ) ;
#15193=EDGE_LOOP ( 'NONE', ( #19118, #13814, #24917, #1029, #3091 ) ) ;
#15194=ADVANCED_FACE ( 'NONE', ( #32536 ), #6852, .F. ) ;
#15195=CARTESIAN_POINT ( 'NONE',  ( 32.99999662536855283, 60.62177826491078747, 12.50000000000000000 ) ) ;
#15197=VECTOR ( 'NONE', #13423, 1000.000000000000000 ) ;
#15199=DIRECTION ( 'NONE',  ( 1.000000000000000000, 0.000000000000000000, 0.000000000000000000 ) ) ;
#15200=EDGE_LOOP ( 'NONE', ( #21294, #37002, #10197, #13934 ) ) ;
#15201=CARTESIAN_POINT ( 'NONE',  ( -12.00000337463128197, 86.60254037844397601, 17.49999999999999645 ) ) ;
#15202=CIRCLE ( 'NONE', #32570, 2.000000000000001776 ) ;
#15203=CARTESIAN_POINT ( 'NONE',  ( -47.63139720814438505, -27.49999999999955591, -5.000000000000000000 ) ) ;
#15205=CYLINDRICAL_SURFACE ( 'NONE', #32830, 2.000000000000001776 ) ;
#15207=EDGE_LOOP ( 'NONE', ( #25661, #34379 ) ) ;
#15209=VERTEX_POINT ( 'NONE', #23386 ) ;
#15210=CARTESIAN_POINT ( 'NONE',  ( 0.000000000000000000, 0.000000000000000000, 12.49999999999999822 ) ) ;
#15211=EDGE_CURVE ( 'NONE', #18995, #14204, #33534, .T. ) ;
#15213=CYLINDRICAL_SURFACE ( 'NONE', #4689, 2.000000000000001776 ) ;
#15217=LINE ( 'NONE', #17483, #12909 ) ;
#15218=AXIS2_PLACEMENT_3D ( 'NONE', #27088, #13525, #30087 ) ;
#15220=ORIENTED_EDGE ( 'NONE', *, *, #26211, .T. ) ;
#15221=CARTESIAN_POINT ( 'NONE',  ( 70.47608876694671665, 59.13646009116074964, -4.999999999999997335 ) ) ;
#15222=CARTESIAN_POINT ( 'NONE',  ( -72.77422209630324801, -61.06482292022084124, 12.49999999999999822 ) ) ;
#15224=CIRCLE ( 'NONE', #6233, 2.000000000000001776 ) ;
#15225=ORIENTED_EDGE ( 'NONE', *, *, #2827, .F. ) ;
#15226=ORIENTED_EDGE ( 'NONE', *, *, #6750, .F. ) ;
#15227=CIRCLE ( 'NONE', #21198, 27.00000000000001066 ) ;
#15228=DIRECTION ( 'NONE',  ( 1.000000000000000000, 0.000000000000000000, 0.000000000000000000 ) ) ;
#15229=CARTESIAN_POINT ( 'NONE',  ( -57.00000337463109901, -60.62177826491083010, -5.000000000000000000 ) ) ;
#15233=ORIENTED_EDGE ( 'NONE', *, *, #35132, .T. ) ;
#15234=EDGE_CURVE ( 'NONE', #10851, #36497, #31102, .T. ) ;
#15235=ADVANCED_FACE ( 'NONE', ( #18106 ), #34818, .F. ) ;
#15236=DIRECTION ( 'NONE',  ( 0.000000000000000000, 0.000000000000000000, 1.000000000000000000 ) ) ;
#15237=CIRCLE ( 'NONE', #11119, 2.000000000000001776 ) ;
#15239=DIRECTION ( 'NONE',  ( 1.000000000000000000, 0.000000000000000000, 0.000000000000000000 ) ) ;
#15240=CIRCLE ( 'NONE', #20033, 3.000000000000002665 ) ;
#15242=DIRECTION ( 'NONE',  ( 0.000000000000000000, 0.000000000000000000, -1.000000000000000000 ) ) ;
#15243=ORIENTED_EDGE ( 'NONE', *, *, #732, .F. ) ;
#15244=ORIENTED_EDGE ( 'NONE', *, *, #19858, .F. ) ;
#15245=CIRCLE ( 'NONE', #10459, 2.000000000000001776 ) ;
#15246=EDGE_CURVE ( 'NONE', #14320, #26696, #22741, .T. ) ;
#15247=( NAMED_UNIT ( * ) PLANE_ANGLE_UNIT ( ) SI_UNIT ( $, .RADIAN. ) );
#15248=CARTESIAN_POINT ( 'NONE',  ( -75.00000337463097821, -8.660254037844422825, -9.999999999999998224 ) ) ;
#15251=ORIENTED_EDGE ( 'NONE', *, *, #4592, .T. ) ;
#15252=DIRECTION ( 'NONE',  ( 1.000000000000000000, 0.000000000000000000, 0.000000000000000000 ) ) ;
#15253=CARTESIAN_POINT ( 'NONE',  ( -65.00000337463102085, 43.30127018922198801, -5.000000000000000000 ) ) ;
#15256=CARTESIAN_POINT ( 'NONE',  ( 7.999996625368656744, -69.28203230275519786, -9.999999999999998224 ) ) ;
#15257=DIRECTION ( 'NONE',  ( -1.000000000000000000, 0.000000000000000000, 0.000000000000000000 ) ) ;
#15258=CIRCLE ( 'NONE', #20045, 2.000000000000001776 ) ;
#15259=ORIENTED_EDGE ( 'NONE', *, *, #27551, .T. ) ;
#15260=DIRECTION ( 'NONE',  ( 0.000000000000000000, 0.000000000000000000, 1.000000000000000000 ) ) ;
#15261=CARTESIAN_POINT ( 'NONE',  ( 0.000000000000000000, 0.000000000000000000, -5.000000000000000000 ) ) ;
#15262=ORIENTED_EDGE ( 'NONE', *, *, #4007, .T. ) ;
#15264=CARTESIAN_POINT ( 'NONE',  ( 71.99999662536841072, 51.96152422706640550, -5.000000000000000000 ) ) ;
#15265=DIRECTION ( 'NONE',  ( 1.000000000000000000, 0.000000000000000000, 0.000000000000000000 ) ) ;
#15266=DIRECTION ( 'NONE',  ( 1.000000000000000000, 0.000000000000000000, 0.000000000000000000 ) ) ;
#15267=CARTESIAN_POINT ( 'NONE',  ( -15.00000337463125710, -77.94228634059960825, -9.999999999999998224 ) ) ;
#15269=CARTESIAN_POINT ( 'NONE',  ( 70.47608876694671665, 59.13646009116074964, -4.999999999999997335 ) ) ;
#15270=AXIS2_PLACEMENT_3D ( 'NONE', #1055, #3307, #6685 ) ;
#15271=CARTESIAN_POINT ( 'NONE',  ( 34.99999662536855283, -77.94228634059960825, -5.000000000000000000 ) ) ;
#15272=ORIENTED_EDGE ( 'NONE', *, *, #30184, .T. ) ;
#15273=DIRECTION ( 'NONE',  ( 1.000000000000000000, 0.000000000000000000, 0.000000000000000000 ) ) ;
#15274=AXIS2_PLACEMENT_3D ( 'NONE', #2381, #28602, #8177 ) ;
#15275=FACE_OUTER_BOUND ( 'NONE', #1086, .T. ) ;
#15277=CIRCLE ( 'NONE', #33268, 2.000000000000000000 ) ;
#15278=ORIENTED_EDGE ( 'NONE', *, *, #11420, .F. ) ;
#15279=CIRCLE ( 'NONE', #36245, 2.000000000000001776 ) ;
#15280=EDGE_LOOP ( 'NONE', ( #21561, #24811 ) ) ;
#15281=ORIENTED_EDGE ( 'NONE', *, *, #6602, .T. ) ;
#15283=CARTESIAN_POINT ( 'NONE',  ( 0.000000000000000000, 0.000000000000000000, -5.000000000000000000 ) ) ;
#15284=CARTESIAN_POINT ( 'NONE',  ( 49.99999662536846756, 69.28203230275516944, 12.50000000000000000 ) ) ;
#15285=DIRECTION ( 'NONE',  ( 0.000000000000000000, 0.000000000000000000, 1.000000000000000000 ) ) ;
#15286=AXIS2_PLACEMENT_3D ( 'NONE', #10367, #26886, #35892 ) ;
#15287=DIRECTION ( 'NONE',  ( 0.000000000000000000, 0.000000000000000000, 1.000000000000000000 ) ) ;
#15288=CARTESIAN_POINT ( 'NONE',  ( -67.00000337463102085, 25.98076211353317433, 17.49999999999999645 ) ) ;
#15289=ORIENTED_EDGE ( 'NONE', *, *, #18598, .T. ) ;
#15291=EDGE_CURVE ( 'NONE', #27517, #2978, #26375, .T. ) ;
#15292=ORIENTED_EDGE ( 'NONE', *, *, #34193, .F. ) ;
#15293=FACE_BOUND ( 'NONE', #30606, .T. ) ;
#15294=EDGE_CURVE ( 'NONE', #21781, #16030, #31959, .T. ) ;
#15295=CARTESIAN_POINT ( 'NONE',  ( -5.000003374631269537, -77.94228634059960825, -9.999999999999998224 ) ) ;
#15296=CIRCLE ( 'NONE', #20664, 2.000000000000001776 ) ;
#15298=AXIS2_PLACEMENT_3D ( 'NONE', #29090, #3428, #26303 ) ;
#15299=ORIENTED_EDGE ( 'NONE', *, *, #16304, .T. ) ;
#15300=CYLINDRICAL_SURFACE ( 'NONE', #1481, 2.000000000000001776 ) ;
#15301=CIRCLE ( 'NONE', #9921, 1.999999999999998224 ) ;
#15306=ORIENTED_EDGE ( 'NONE', *, *, #30353, .F. ) ;
#15307=DIRECTION ( 'NONE',  ( 1.000000000000000000, 0.000000000000000000, 0.000000000000000000 ) ) ;
#15308=DIRECTION ( 'NONE',  ( 1.000000000000000000, 0.000000000000000000, 0.000000000000000000 ) ) ;
#15309=CARTESIAN_POINT ( 'NONE',  ( 9.999996625368625658, 86.60254037844397601, -9.999999999999998224 ) ) ;
#15311=VERTEX_POINT ( 'NONE', #12839 ) ;
#15312=EDGE_CURVE ( 'NONE', #29261, #35651, #16157, .T. ) ;
#15313=VERTEX_POINT ( 'NONE', #19057 ) ;
#15314=EDGE_LOOP ( 'NONE', ( #2216, #363 ) ) ;
#15315=CARTESIAN_POINT ( 'NONE',  ( -35.00000337463116296, -60.62177826491080168, 12.50000000000000000 ) ) ;
#15316=DIRECTION ( 'NONE',  ( 0.000000000000000000, 0.000000000000000000, 1.000000000000000000 ) ) ;
#15317=ADVANCED_FACE ( 'NONE', ( #27483 ), #16241, .F. ) ;
#15318=CARTESIAN_POINT ( 'NONE',  ( 52.99999662536846046, -43.30127018922200222, -5.000000000000000000 ) ) ;
#15319=AXIS2_PLACEMENT_3D ( 'NONE', #26301, #31890, #32461 ) ;
#15320=EDGE_CURVE ( 'NONE', #10671, #4910, #16745, .T. ) ;
#15321=DIRECTION ( 'NONE',  ( 1.000000000000000000, 0.000000000000000000, 0.000000000000000000 ) ) ;
#15322=CARTESIAN_POINT ( 'NONE',  ( 52.39915983220795681, 35.19434990244919703, 12.49999999999999822 ) ) ;
#15323=AXIS2_PLACEMENT_3D ( 'NONE', #36768, #16345, #2078 ) ;
#15324=AXIS2_PLACEMENT_3D ( 'NONE', #35766, #15316, #18698 ) ;
#15325=FACE_OUTER_BOUND ( 'NONE', #16829, .T. ) ;
#15326=AXIS2_PLACEMENT_3D ( 'NONE', #4710, #3944, #26830 ) ;
#15327=ORIENTED_EDGE ( 'NONE', *, *, #10884, .T. ) ;
#15328=CIRCLE ( 'NONE', #32095, 2.000000000000001776 ) ;
#15329=ORIENTED_EDGE ( 'NONE', *, *, #30448, .F. ) ;
#15330=FACE_OUTER_BOUND ( 'NONE', #5623, .T. ) ;
#15331=CIRCLE ( 'NONE', #34501, 2.000000000000000000 ) ;
#15335=ORIENTED_EDGE ( 'NONE', *, *, #3685, .T. ) ;
#15336=AXIS2_PLACEMENT_3D ( 'NONE', #16450, #10449, #7846 ) ;
#15337=ADVANCED_FACE ( 'NONE', ( #4808 ), #7244, .F. ) ;
#15338=CARTESIAN_POINT ( 'NONE',  ( 77.99999662536833966, 34.64101615137759183, -5.000000000000000000 ) ) ;
#15339=VERTEX_POINT ( 'NONE', #29925 ) ;
#15340=ORIENTED_EDGE ( 'NONE', *, *, #6003, .F. ) ;
#15341=FACE_OUTER_BOUND ( 'NONE', #22336, .T. ) ;
#15342=EDGE_LOOP ( 'NONE', ( #35098, #29837, #10584, #18338, #36926 ) ) ;
#15343=AXIS2_PLACEMENT_3D ( 'NONE', #26895, #33251, #33066 ) ;
#15344=CARTESIAN_POINT ( 'NONE',  ( -67.00000337463102085, 60.62177826491077326, 17.49999999999999645 ) ) ;
#15345=AXIS2_PLACEMENT_3D ( 'NONE', #14269, #28696, #5082 ) ;
#15346=DIRECTION ( 'NONE',  ( 0.000000000000000000, 0.000000000000000000, -1.000000000000000000 ) ) ;
#15347=CARTESIAN_POINT ( 'NONE',  ( 59.99999662536845335, 34.64101615137759893, -5.000000000000000000 ) ) ;
#15349=ORIENTED_EDGE ( 'NONE', *, *, #30503, .T. ) ;
#15350=VERTEX_POINT ( 'NONE', #23695 ) ;
#15351=AXIS2_PLACEMENT_3D ( 'NONE', #31903, #23128, #15228 ) ;
#15352=CIRCLE ( 'NONE', #36330, 95.00000000000001421 ) ;
#15354=AXIS2_PLACEMENT_3D ( 'NONE', #584, #32442, #11627 ) ;
#15357=AXIS2_PLACEMENT_3D ( 'NONE', #6516, #29546, #32551 ) ;
#15364=CYLINDRICAL_SURFACE ( 'NONE', #498, 3.000000000000002665 ) ;
#15365=CARTESIAN_POINT ( 'NONE',  ( 91.99999662536828282, 0.000000000000000000, -9.999999999999998224 ) ) ;
#15366=DIRECTION ( 'NONE',  ( 1.000000000000000000, 0.000000000000000000, 0.000000000000000000 ) ) ;
#15367=EDGE_LOOP ( 'NONE', ( #27349, #18826 ) ) ;
#15369=AXIS2_PLACEMENT_3D ( 'NONE', #14341, #19954, #22396 ) ;
#15370=EDGE_CURVE ( 'NONE', #23192, #28818, #21494, .T. ) ;
#15371=DIRECTION ( 'NONE',  ( 1.000000000000000000, 0.000000000000000000, 0.000000000000000000 ) ) ;
#15372=DIRECTION ( 'NONE',  ( -1.000000000000000000, 0.000000000000000000, 0.000000000000000000 ) ) ;
#15375=EDGE_CURVE ( 'NONE', #11435, #17617, #34729, .T. ) ;
#15378=ORIENTED_EDGE ( 'NONE', *, *, #16584, .F. ) ;
#15379=CIRCLE ( 'NONE', #31528, 33.00000000000001421 ) ;
#15382=CARTESIAN_POINT ( 'NONE',  ( -28.00000337463118427, 69.28203230275516944, -9.999999999999998224 ) ) ;
#15383=CARTESIAN_POINT ( 'NONE',  ( 62.97617850287784336, 4.279621169095339184, -4.999999999999997335 ) ) ;
#15385=CYLINDRICAL_SURFACE ( 'NONE', #4158, 2.000000000000001776 ) ;
#15386=VERTEX_POINT ( 'NONE', #10241 ) ;
#15387=ADVANCED_FACE ( 'NONE', ( #1800 ), #33492, .F. ) ;
#15389=CARTESIAN_POINT ( 'NONE',  ( -78.00000337463094979, -2.428612866367529932E-14, -9.999999999999998224 ) ) ;
#15391=EDGE_CURVE ( 'NONE', #8516, #14843, #10770, .T. ) ;
#15393=CIRCLE ( 'NONE', #36362, 2.000000000000001776 ) ;
#15394=AXIS2_PLACEMENT_3D ( 'NONE', #29507, #656, #12066 ) ;
#15395=EDGE_CURVE ( 'NONE', #28847, #26778, #13233, .T. ) ;
#15396=ORIENTED_EDGE ( 'NONE', *, *, #35294, .F. ) ;
#15398=ADVANCED_FACE ( 'NONE', ( #33288 ), #7800, .F. ) ;
#15399=DIRECTION ( 'NONE',  ( -1.000000000000000000, 0.000000000000000000, -0.000000000000000000 ) ) ;
#15400=ORIENTED_EDGE ( 'NONE', *, *, #21330, .T. ) ;
#15401=CARTESIAN_POINT ( 'NONE',  ( -73.00000337463099243, -25.98076211353322051, -9.999999999999998224 ) ) ;
#15402=AXIS2_PLACEMENT_3D ( 'NONE', #20831, #14294, #5857 ) ;
#15406=ORIENTED_EDGE ( 'NONE', *, *, #31846, .T. ) ;
#15407=AXIS2_PLACEMENT_3D ( 'NONE', #31001, #7571, #2677 ) ;
#15408=CIRCLE ( 'NONE', #1623, 3.000000000000002665 ) ;
#15409=CIRCLE ( 'NONE', #28571, 27.00000000000001421 ) ;
#15412=LINE ( 'NONE', #24208, #5983 ) ;
#15413=CARTESIAN_POINT ( 'NONE',  ( -90.00000337463090716, -1.040834085586084257E-14, -5.000000000000000000 ) ) ;
#15415=FACE_OUTER_BOUND ( 'NONE', #9166, .T. ) ;
#15416=CIRCLE ( 'NONE', #36386, 2.000000000000001776 ) ;
#15417=VERTEX_POINT ( 'NONE', #253 ) ;
#15418=DIRECTION ( 'NONE',  ( 1.000000000000000000, 0.000000000000000000, 0.000000000000000000 ) ) ;
#15420=CIRCLE ( 'NONE', #32184, 2.000000000000001776 ) ;
#15422=FACE_OUTER_BOUND ( 'NONE', #10701, .T. ) ;
#15424=CARTESIAN_POINT ( 'NONE',  ( -55.00000337463107059, 60.62177826491078747, -9.999999999999998224 ) ) ;
#15425=DIRECTION ( 'NONE',  ( 1.000000000000000000, 0.000000000000000000, 0.000000000000000000 ) ) ;
#15426=DIRECTION ( 'NONE',  ( 0.000000000000000000, 0.000000000000000000, -1.000000000000000000 ) ) ;
#15427=VECTOR ( 'NONE', #27498, 1000.000000000000000 ) ;
#15428=VERTEX_POINT ( 'NONE', #5163 ) ;
#15429=ORIENTED_EDGE ( 'NONE', *, *, #27225, .F. ) ;
#15431=DIRECTION ( 'NONE',  ( -0.8660254037844380415, 0.5000000000000009992, 0.000000000000000000 ) ) ;
#15433=CARTESIAN_POINT ( 'NONE',  ( -45.00000337463111322, 77.94228634059959404, -9.999999999999998224 ) ) ;
#15434=VERTEX_POINT ( 'NONE', #16604 ) ;
#15435=ORIENTED_EDGE ( 'NONE', *, *, #18774, .F. ) ;
#15436=CIRCLE ( 'NONE', #32802, 2.000000000000001776 ) ;
#15437=CIRCLE ( 'NONE', #14841, 2.000000000000001776 ) ;
#15438=VERTEX_POINT ( 'NONE', #14345 ) ;
#15439=AXIS2_PLACEMENT_3D ( 'NONE', #402, #14851, #17475 ) ;
#15440=DIRECTION ( 'NONE',  ( 0.000000000000000000, 0.000000000000000000, 1.000000000000000000 ) ) ;
#15442=ORIENTED_EDGE ( 'NONE', *, *, #11222, .F. ) ;
#15443=ADVANCED_FACE ( 'NONE', ( #28769 ), #5365, .F. ) ;
#15444=VERTEX_POINT ( 'NONE', #31215 ) ;
#15445=DIRECTION ( 'NONE',  ( 0.000000000000000000, 0.000000000000000000, -1.000000000000000000 ) ) ;
#15447=ORIENTED_EDGE ( 'NONE', *, *, #1519, .F. ) ;
#15448=AXIS2_PLACEMENT_3D ( 'NONE', #30958, #23025, #36916 ) ;
#15449=CARTESIAN_POINT ( 'NONE',  ( 67.99999662536838230, 34.64101615137758472, -9.999999999999998224 ) ) ;
#15450=LINE ( 'NONE', #19008, #10497 ) ;
#15451=ORIENTED_EDGE ( 'NONE', *, *, #494, .T. ) ;
#15452=EDGE_LOOP ( 'NONE', ( #6080, #1596, #13696, #11168 ) ) ;
#15453=DIRECTION ( 'NONE',  ( 0.000000000000000000, 0.000000000000000000, 1.000000000000000000 ) ) ;
#15454=VECTOR ( 'NONE', #2173, 1000.000000000000000 ) ;
#15455=CARTESIAN_POINT ( 'NONE',  ( -82.00000337463094979, -2.404119930384582903E-14, 17.49999999999999645 ) ) ;
#15456=CARTESIAN_POINT ( 'NONE',  ( 56.99999662536844625, 43.30127018922198801, -9.999999999999998224 ) ) ;
#15458=ORIENTED_EDGE ( 'NONE', *, *, #5572, .T. ) ;
#15459=CARTESIAN_POINT ( 'NONE',  ( 6.999996625368645198, 77.94228634059957983, -9.999999999999998224 ) ) ;
#15460=CARTESIAN_POINT ( 'NONE',  ( -62.00000337463104927, 51.96152422706639129, -9.999999999999998224 ) ) ;
#15461=CIRCLE ( 'NONE', #5883, 3.000000000000002665 ) ;
#15462=ORIENTED_EDGE ( 'NONE', *, *, #2958, .T. ) ;
#15463=CARTESIAN_POINT ( 'NONE',  ( 21.99999662536862033, -86.60254037844400443, -5.000000000000000000 ) ) ;
#15465=CIRCLE ( 'NONE', #12475, 33.00000000000001421 ) ;
#15466=DIRECTION ( 'NONE',  ( 0.000000000000000000, 0.000000000000000000, 1.000000000000000000 ) ) ;
#15467=CARTESIAN_POINT ( 'NONE',  ( -56.67878100130369035, 27.78182860042797131, -49.86348611802629449 ) ) ;
#15469=DIRECTION ( 'NONE',  ( 1.000000000000000000, 0.000000000000000000, 0.000000000000000000 ) ) ;
#15470=DIRECTION ( 'NONE',  ( 0.000000000000000000, 0.000000000000000000, -1.000000000000000000 ) ) ;
#15471=AXIS2_PLACEMENT_3D ( 'NONE', #6374, #26438, #23621 ) ;
#15472=CARTESIAN_POINT ( 'NONE',  ( -18.00000337463123046, 86.60254037844397601, 17.49999999999999645 ) ) ;
#15473=ORIENTED_EDGE ( 'NONE', *, *, #7925, .F. ) ;
#15474=DIRECTION ( 'NONE',  ( 0.000000000000000000, 0.000000000000000000, 1.000000000000000000 ) ) ;
#15475=LINE ( 'NONE', #29701, #15958 ) ;
#15476=DIRECTION ( 'NONE',  ( 1.000000000000000000, 0.000000000000000000, 0.000000000000000000 ) ) ;
#15477=VERTEX_POINT ( 'NONE', #8157 ) ;
#15478=EDGE_CURVE ( 'NONE', #3872, #21416, #36528, .T. ) ;
#15479=AXIS2_PLACEMENT_3D ( 'NONE', #36450, #7936, #10760 ) ;
#15480=VERTEX_POINT ( 'NONE', #11343 ) ;
#15482=DIRECTION ( 'NONE',  ( 0.000000000000000000, 0.000000000000000000, 1.000000000000000000 ) ) ;
#15483=DIRECTION ( 'NONE',  ( -1.000000000000000000, 0.000000000000000000, -0.000000000000000000 ) ) ;
#15484=DIRECTION ( 'NONE',  ( -0.5000000000000094369, -0.8660254037844332675, 0.000000000000000000 ) ) ;
#15485=VECTOR ( 'NONE', #34195, 1000.000000000000000 ) ;
#15487=DIRECTION ( 'NONE',  ( 1.000000000000000000, 0.000000000000000000, 0.000000000000000000 ) ) ;
#15489=CARTESIAN_POINT ( 'NONE',  ( 74.99999662536836809, 43.30127018922198801, 17.49999999999999645 ) ) ;
#15490=ORIENTED_EDGE ( 'NONE', *, *, #14603, .F. ) ;
#15492=CARTESIAN_POINT ( 'NONE',  ( 0.000000000000000000, 55.00000000000000000, -5.000000000000000000 ) ) ;
#15494=VECTOR ( 'NONE', #26692, 1000.000000000000000 ) ;
#15495=FACE_BOUND ( 'NONE', #6029, .T. ) ;
#15496=CARTESIAN_POINT ( 'NONE',  ( 19.99999662536861678, -86.60254037844400443, -5.000000000000000000 ) ) ;
#15498=FACE_OUTER_BOUND ( 'NONE', #26820, .T. ) ;
#15499=DIRECTION ( 'NONE',  ( 0.000000000000000000, 0.000000000000000000, -1.000000000000000000 ) ) ;
#15500=ORIENTED_EDGE ( 'NONE', *, *, #1887, .F. ) ;
#15502=VECTOR ( 'NONE', #33381, 1000.000000000000000 ) ;
#15507=ADVANCED_FACE ( 'NONE', ( #11689 ), #22795, .F. ) ;
#15508=VERTEX_POINT ( 'NONE', #22399 ) ;
#15510=CARTESIAN_POINT ( 'NONE',  ( -15.00000337463125710, -77.94228634059960825, 17.49999999999999645 ) ) ;
#15512=EDGE_CURVE ( 'NONE', #32313, #19796, #25956, .T. ) ;
#15513=ORIENTED_EDGE ( 'NONE', *, *, #23416, .T. ) ;
#15515=AXIS2_PLACEMENT_3D ( 'NONE', #31086, #5414, #24911 ) ;
#15516=ORIENTED_EDGE ( 'NONE', *, *, #10549, .F. ) ;
#15519=DIRECTION ( 'NONE',  ( -1.000000000000000000, 0.000000000000000000, 0.000000000000000000 ) ) ;
#15520=CARTESIAN_POINT ( 'NONE',  ( 64.99999662536841072, 25.98076211353318854, -5.000000000000000000 ) ) ;
#15521=FACE_OUTER_BOUND ( 'NONE', #14685, .T. ) ;
#15522=EDGE_CURVE ( 'NONE', #18158, #8626, #37001, .T. ) ;
#15523=CIRCLE ( 'NONE', #8909, 1.999999999999998224 ) ;
#15524=DIRECTION ( 'NONE',  ( 1.000000000000000000, 0.000000000000000000, 0.000000000000000000 ) ) ;
#15525=DIRECTION ( 'NONE',  ( 0.000000000000000000, 0.000000000000000000, 1.000000000000000000 ) ) ;
#15526=CIRCLE ( 'NONE', #19155, 2.000000000000000000 ) ;
#15527=CARTESIAN_POINT ( 'NONE',  ( -28.00000337463118427, 69.28203230275516944, -5.000000000000000000 ) ) ;
#15528=ORIENTED_EDGE ( 'NONE', *, *, #13653, .T. ) ;
#15529=EDGE_LOOP ( 'NONE', ( #25790, #15607 ) ) ;
#15531=CARTESIAN_POINT ( 'NONE',  ( -71.20512444582767841, -36.23716251175871861, -5.000000000000000000 ) ) ;
#15532=ORIENTED_EDGE ( 'NONE', *, *, #28451, .F. ) ;
#15533=CIRCLE ( 'NONE', #2377, 2.000000000000001776 ) ;
#15534=DIRECTION ( 'NONE',  ( 0.000000000000000000, 0.000000000000000000, -1.000000000000000000 ) ) ;
#15535=ORIENTED_EDGE ( 'NONE', *, *, #34088, .F. ) ;
#15536=DIRECTION ( 'NONE',  ( -0.000000000000000000, -0.000000000000000000, 1.000000000000000000 ) ) ;
#15537=EDGE_CURVE ( 'NONE', #10828, #17104, #15420, .T. ) ;
#15538=AXIS2_PLACEMENT_3D ( 'NONE', #2452, #19695, #30743 ) ;
#15539=DIRECTION ( 'NONE',  ( 1.000000000000000000, 0.000000000000000000, 0.000000000000000000 ) ) ;
#15540=AXIS2_PLACEMENT_3D ( 'NONE', #30300, #33854, #10970 ) ;
#15541=VERTEX_POINT ( 'NONE', #28387 ) ;
#15542=EDGE_LOOP ( 'NONE', ( #14971, #22590, #6816, #3677 ) ) ;
#15543=AXIS2_PLACEMENT_3D ( 'NONE', #2412, #8217, #124 ) ;
#15544=CARTESIAN_POINT ( 'NONE',  ( -82.00000337463094979, -17.32050807568882078, 17.49999999999999645 ) ) ;
#15546=EDGE_CURVE ( 'NONE', #33148, #20492, #20211, .T. ) ;
#15547=DIRECTION ( 'NONE',  ( 0.5000000000000039968, 0.8660254037844363761, 0.000000000000000000 ) ) ;
#15548=DIRECTION ( 'NONE',  ( -0.000000000000000000, -0.000000000000000000, 1.000000000000000000 ) ) ;
#15549=CARTESIAN_POINT ( 'NONE',  ( -27.78182860042817026, -56.67878100130359087, -4.999999999999997335 ) ) ;
#15550=EDGE_CURVE ( 'NONE', #24230, #22827, #28582, .T. ) ;
#15551=ORIENTED_EDGE ( 'NONE', *, *, #13155, .T. ) ;
#15552=AXIS2_PLACEMENT_3D ( 'NONE', #14338, #2908, #2527 ) ;
#15553=ORIENTED_EDGE ( 'NONE', *, *, #30114, .T. ) ;
#15554=ORIENTED_EDGE ( 'NONE', *, *, #18978, .T. ) ;
#15555=ORIENTED_EDGE ( 'NONE', *, *, #7506, .T. ) ;
#15556=CARTESIAN_POINT ( 'NONE',  ( -45.00000337463111322, 77.94228634059959404, -9.999999999999998224 ) ) ;
#15557=CIRCLE ( 'NONE', #4193, 2.000000000000001776 ) ;
#15558=DIRECTION ( 'NONE',  ( 1.000000000000000000, 0.000000000000000000, 0.000000000000000000 ) ) ;
#15559=EDGE_LOOP ( 'NONE', ( #1586, #13091, #1256, #20141 ) ) ;
#15560=CARTESIAN_POINT ( 'NONE',  ( 31.46585318596250502, 86.45172111230321832, -49.86348611802629449 ) ) ;
#15561=PLANE ( 'NONE',  #18753 ) ;
#15563=PLANE ( 'NONE',  #36351 ) ;
#15564=ORIENTED_EDGE ( 'NONE', *, *, #15723, .F. ) ;
#15567=EDGE_CURVE ( 'NONE', #7036, #21808, #35218, .T. ) ;
#15568=VECTOR ( 'NONE', #34963, 1000.000000000000000 ) ;
#15569=FACE_OUTER_BOUND ( 'NONE', #20984, .T. ) ;
#15570=VERTEX_POINT ( 'NONE', #33847 ) ;
#15571=DIRECTION ( 'NONE',  ( -1.000000000000000000, 0.000000000000000000, 0.000000000000000000 ) ) ;
#15572=AXIS2_PLACEMENT_3D ( 'NONE', #24910, #30339, #25111 ) ;
#15573=CARTESIAN_POINT ( 'NONE',  ( 56.67878100130369035, -27.78182860042797131, -49.86348611802629449 ) ) ;
#15574=VERTEX_POINT ( 'NONE', #16961 ) ;
#15575=ORIENTED_EDGE ( 'NONE', *, *, #34118, .F. ) ;
#15576=DIRECTION ( 'NONE',  ( 0.000000000000000000, 0.000000000000000000, 1.000000000000000000 ) ) ;
#15577=LINE ( 'NONE', #27570, #12118 ) ;
#15578=CARTESIAN_POINT ( 'NONE',  ( 59.99999662536843914, -34.64101615137759893, -5.000000000000000000 ) ) ;
#15579=CARTESIAN_POINT ( 'NONE',  ( -50.00000337463109190, 69.28203230275518365, 12.50000000000000000 ) ) ;
#15582=VECTOR ( 'NONE', #4802, 1000.000000000000000 ) ;
#15584=DIRECTION ( 'NONE',  ( -0.000000000000000000, -0.000000000000000000, 1.000000000000000000 ) ) ;
#15585=EDGE_CURVE ( 'NONE', #15870, #698, #28034, .T. ) ;
#15586=ORIENTED_EDGE ( 'NONE', *, *, #4972, .T. ) ;
#15587=EDGE_CURVE ( 'NONE', #32894, #2284, #30406, .T. ) ;
#15588=CARTESIAN_POINT ( 'NONE',  ( 22.99999662536857059, 77.94228634059957983, -9.999999999999998224 ) ) ;
#15589=ORIENTED_EDGE ( 'NONE', *, *, #24044, .F. ) ;
#15591=EDGE_CURVE ( 'NONE', #22677, #18010, #35801, .T. ) ;
#15592=CARTESIAN_POINT ( 'NONE',  ( 71.99999662536838230, -51.96152422706639840, 17.49999999999999645 ) ) ;
#15593=AXIS2_PLACEMENT_3D ( 'NONE', #20399, #17967, #18138 ) ;
#15594=CARTESIAN_POINT ( 'NONE',  ( 6.999996625368676284, -77.94228634059960825, -9.999999999999998224 ) ) ;
#15596=ORIENTED_EDGE ( 'NONE', *, *, #18949, .F. ) ;
#15597=EDGE_LOOP ( 'NONE', ( #26785, #16598, #3994, #8457 ) ) ;
#15599=ORIENTED_EDGE ( 'NONE', *, *, #1203, .T. ) ;
#15601=CYLINDRICAL_SURFACE ( 'NONE', #17361, 2.000000000000001776 ) ;
#15602=CIRCLE ( 'NONE', #17396, 2.000000000000001776 ) ;
#15603=CARTESIAN_POINT ( 'NONE',  ( -60.00000337463107059, -34.64101615137762025, -9.999999999999998224 ) ) ;
#15605=CYLINDRICAL_SURFACE ( 'NONE', #17154, 2.000000000000001776 ) ;
#15606=EDGE_CURVE ( 'NONE', #35441, #31631, #6455, .T. ) ;
#15607=ORIENTED_EDGE ( 'NONE', *, *, #17116, .F. ) ;
#15609=EDGE_CURVE ( 'NONE', #30886, #36051, #4674, .T. ) ;
#15610=CARTESIAN_POINT ( 'NONE',  ( -65.00000337463102085, 25.98076211353317433, 17.49999999999999645 ) ) ;
#15611=ADVANCED_FACE ( 'NONE', ( #12430 ), #21062, .T. ) ;
#15612=AXIS2_PLACEMENT_3D ( 'NONE', #36417, #27598, #22518 ) ;
#15613=DIRECTION ( 'NONE',  ( 1.000000000000000000, 0.000000000000000000, 0.000000000000000000 ) ) ;
#15614=ORIENTED_EDGE ( 'NONE', *, *, #6352, .T. ) ;
#15618=DIRECTION ( 'NONE',  ( 0.000000000000000000, 0.000000000000000000, 1.000000000000000000 ) ) ;
#15620=VERTEX_POINT ( 'NONE', #12222 ) ;
#15621=LINE ( 'NONE', #10534, #1334 ) ;
#15622=CARTESIAN_POINT ( 'NONE',  ( -15.00000337463125710, -77.94228634059960825, -9.999999999999998224 ) ) ;
#15623=DIRECTION ( 'NONE',  ( -1.000000000000000000, 0.000000000000000000, 0.000000000000000000 ) ) ;
#15624=VERTEX_POINT ( 'NONE', #14695 ) ;
#15625=VERTEX_POINT ( 'NONE', #15449 ) ;
#15628=EDGE_CURVE ( 'NONE', #10938, #28829, #448, .T. ) ;
#15629=EDGE_LOOP ( 'NONE', ( #8581, #25505 ) ) ;
#15630=EDGE_CURVE ( 'NONE', #14791, #26021, #12051, .T. ) ;
#15631=ORIENTED_EDGE ( 'NONE', *, *, #16052, .F. ) ;
#15632=DIRECTION ( 'NONE',  ( 0.000000000000000000, 0.000000000000000000, 1.000000000000000000 ) ) ;
#15633=VERTEX_POINT ( 'NONE', #34780 ) ;
#15635=PLANE ( 'NONE',  #14240 ) ;
#15639=ADVANCED_FACE ( 'NONE', ( #32490 ), #26687, .F. ) ;
#15640=DIRECTION ( 'NONE',  ( 0.000000000000000000, 0.000000000000000000, 1.000000000000000000 ) ) ;
#15641=CARTESIAN_POINT ( 'NONE',  ( -80.00000337463094979, 17.32050807568878525, -5.000000000000000000 ) ) ;
#15642=CARTESIAN_POINT ( 'NONE',  ( -33.21453780030408609, 78.84345928898012801, -5.000000000000000000 ) ) ;
#15643=DIRECTION ( 'NONE',  ( 0.000000000000000000, 0.000000000000000000, 1.000000000000000000 ) ) ;
#15644=ORIENTED_EDGE ( 'NONE', *, *, #22942, .T. ) ;
#15645=CARTESIAN_POINT ( 'NONE',  ( 36.99999662536855283, -77.94228634059960825, -9.999999999999998224 ) ) ;
#15646=ORIENTED_EDGE ( 'NONE', *, *, #6463, .T. ) ;
#15648=CARTESIAN_POINT ( 'NONE',  ( -80.00000337463094979, -2.428612866367529932E-14, -9.999999999999998224 ) ) ;
#15649=CARTESIAN_POINT ( 'NONE',  ( -47.63139720814438505, -27.49999999999955591, -10.00000000000000000 ) ) ;
#15650=FACE_OUTER_BOUND ( 'NONE', #14364, .T. ) ;
#15651=ADVANCED_FACE ( 'NONE', ( #20333 ), #9248, .T. ) ;
#15652=DIRECTION ( 'NONE',  ( 1.000000000000000000, 0.000000000000000000, 0.000000000000000000 ) ) ;
#15653=EDGE_CURVE ( 'NONE', #19903, #28212, #18423, .T. ) ;
#15654=DIRECTION ( 'NONE',  ( 0.000000000000000000, 0.000000000000000000, 1.000000000000000000 ) ) ;
#15655=ADVANCED_FACE ( 'NONE', ( #20495, #29320, #31918, #26500, #3644, #814, #23696, #6637, #1006 ), #30053, .F. ) ;
#15656=ADVANCED_FACE ( 'NONE', ( #7004 ), #2107, .F. ) ;
#15657=DIRECTION ( 'NONE',  ( 0.000000000000000000, 0.000000000000000000, 1.000000000000000000 ) ) ;
#15658=ORIENTED_EDGE ( 'NONE', *, *, #30008, .T. ) ;
#15660=AXIS2_PLACEMENT_3D ( 'NONE', #847, #22481, #25687 ) ;
#15661=CYLINDRICAL_SURFACE ( 'NONE', #8753, 2.000000000000001776 ) ;
#15663=ORIENTED_EDGE ( 'NONE', *, *, #487, .F. ) ;
#15664=ORIENTED_EDGE ( 'NONE', *, *, #5273, .F. ) ;
#15665=ORIENTED_EDGE ( 'NONE', *, *, #10591, .T. ) ;
#15667=DIRECTION ( 'NONE',  ( 0.000000000000000000, 0.000000000000000000, -1.000000000000000000 ) ) ;
#15669=VERTEX_POINT ( 'NONE', #29876 ) ;
#15670=DIRECTION ( 'NONE',  ( 1.000000000000000000, 0.000000000000000000, 0.000000000000000000 ) ) ;
#15671=LINE ( 'NONE', #848, #9325 ) ;
#15672=ORIENTED_EDGE ( 'NONE', *, *, #10349, .F. ) ;
#15674=DIRECTION ( 'NONE',  ( 1.000000000000000000, 0.000000000000000000, 0.000000000000000000 ) ) ;
#15675=ORIENTED_EDGE ( 'NONE', *, *, #6707, .F. ) ;
#15676=FACE_BOUND ( 'NONE', #4333, .T. ) ;
#15677=ADVANCED_FACE ( 'NONE', ( #18638 ), #15635, .T. ) ;
#15679=DIRECTION ( 'NONE',  ( 1.000000000000000000, 0.000000000000000000, 0.000000000000000000 ) ) ;
#15680=AXIS2_PLACEMENT_3D ( 'NONE', #259, #23518, #28941 ) ;
#15681=PLANE ( 'NONE',  #24772 ) ;
#15683=CARTESIAN_POINT ( 'NONE',  ( 44.99999662536849598, 60.62177826491077326, -5.000000000000000000 ) ) ;
#15686=DIRECTION ( 'NONE',  ( 0.000000000000000000, 0.000000000000000000, 1.000000000000000000 ) ) ;
#15688=DIRECTION ( 'NONE',  ( 1.000000000000000000, 0.000000000000000000, 0.000000000000000000 ) ) ;
#15689=VERTEX_POINT ( 'NONE', #7558 ) ;
#15691=LINE ( 'NONE', #23957, #22644 ) ;
#15692=DIRECTION ( 'NONE',  ( 1.000000000000000000, 0.000000000000000000, 0.000000000000000000 ) ) ;
#15693=VERTEX_POINT ( 'NONE', #21443 ) ;
#15694=EDGE_CURVE ( 'NONE', #13344, #15444, #6453, .T. ) ;
#15695=ORIENTED_EDGE ( 'NONE', *, *, #32355, .T. ) ;
#15697=DIRECTION ( 'NONE',  ( 1.000000000000000000, 0.000000000000000000, 0.000000000000000000 ) ) ;
#15698=CARTESIAN_POINT ( 'NONE',  ( 57.99999662536844625, 34.64101615137759893, 17.49999999999999645 ) ) ;
#15700=AXIS2_PLACEMENT_3D ( 'NONE', #57, #34204, #11111 ) ;
#15703=CARTESIAN_POINT ( 'NONE',  ( 79.99999662536832545, -17.32050807568879591, -9.999999999999998224 ) ) ;
#15704=CARTESIAN_POINT ( 'NONE',  ( 64.99999662536842493, 43.30127018922200222, -9.999999999999998224 ) ) ;
#15705=ORIENTED_EDGE ( 'NONE', *, *, #19738, .T. ) ;
#15706=ORIENTED_EDGE ( 'NONE', *, *, #36207, .T. ) ;
#15707=DIRECTION ( 'NONE',  ( -1.000000000000000000, 0.000000000000000000, -0.000000000000000000 ) ) ;
#15708=DIRECTION ( 'NONE',  ( 1.000000000000000000, 0.000000000000000000, 0.000000000000000000 ) ) ;
#15709=EDGE_LOOP ( 'NONE', ( #13454, #35473, #27691, #1503 ) ) ;
#15710=DIRECTION ( 'NONE',  ( 0.000000000000000000, 0.000000000000000000, -1.000000000000000000 ) ) ;
#15711=ORIENTED_EDGE ( 'NONE', *, *, #29562, .F. ) ;
#15712=CARTESIAN_POINT ( 'NONE',  ( -59.13646009116099833, 70.47608876694653190, -4.999999999999997335 ) ) ;
#15713=EDGE_CURVE ( 'NONE', #12842, #31614, #23829, .T. ) ;
#15714=AXIS2_PLACEMENT_3D ( 'NONE', #24198, #12745, #33188 ) ;
#15715=CIRCLE ( 'NONE', #3744, 33.00000000000001421 ) ;
#15716=FACE_BOUND ( 'NONE', #4107, .T. ) ;
#15720=PLANE ( 'NONE',  #35616 ) ;
#15721=ORIENTED_EDGE ( 'NONE', *, *, #25735, .T. ) ;
#15722=CARTESIAN_POINT ( 'NONE',  ( 19.99999662536857770, 86.60254037844397601, -9.999999999999998224 ) ) ;
#15723=EDGE_CURVE ( 'NONE', #11450, #12872, #7046, .T. ) ;
#15724=CIRCLE ( 'NONE', #25891, 2.000000000000001776 ) ;
#15725=LINE ( 'NONE', #2213, #20329 ) ;
#15726=DIRECTION ( 'NONE',  ( 0.000000000000000000, -0.000000000000000000, -1.000000000000000000 ) ) ;
#15727=ORIENTED_EDGE ( 'NONE', *, *, #11020, .F. ) ;
#15728=DIRECTION ( 'NONE',  ( -1.000000000000000000, 0.000000000000000000, 0.000000000000000000 ) ) ;
#15729=DIRECTION ( 'NONE',  ( 1.000000000000000000, 0.000000000000000000, 0.000000000000000000 ) ) ;
#15730=VERTEX_POINT ( 'NONE', #1367 ) ;
#15731=ORIENTED_EDGE ( 'NONE', *, *, #32785, .F. ) ;
#15732=ORIENTED_EDGE ( 'NONE', *, *, #31089, .T. ) ;
#15734=EDGE_CURVE ( 'NONE', #27983, #23723, #27790, .T. ) ;
#15736=ORIENTED_EDGE ( 'NONE', *, *, #13954, .T. ) ;
#15737=FACE_OUTER_BOUND ( 'NONE', #24418, .T. ) ;
#15738=DIRECTION ( 'NONE',  ( -1.000000000000000000, 0.000000000000000000, 0.000000000000000000 ) ) ;
#15739=ORIENTED_EDGE ( 'NONE', *, *, #12601, .T. ) ;
#15740=FACE_OUTER_BOUND ( 'NONE', #35438, .T. ) ;
#15741=CIRCLE ( 'NONE', #24123, 2.000000000000001776 ) ;
#15742=CARTESIAN_POINT ( 'NONE',  ( -50.00000337463109190, 69.28203230275518365, -9.999999999999998224 ) ) ;
#15743=CARTESIAN_POINT ( 'NONE',  ( 35.19434990244975126, -52.39915983220758022, 12.49999999999999822 ) ) ;
#15744=CARTESIAN_POINT ( 'NONE',  ( -43.00000337463112743, -60.62177826491080168, -9.999999999999998224 ) ) ;
#15746=CARTESIAN_POINT ( 'NONE',  ( 47.99999662536846756, 51.96152422706637708, 12.50000000000000000 ) ) ;
#15749=ORIENTED_EDGE ( 'NONE', *, *, #12902, .T. ) ;
#15750=CARTESIAN_POINT ( 'NONE',  ( 11.99999662536861855, 69.28203230275516944, -5.000000000000000000 ) ) ;
#15751=CIRCLE ( 'NONE', #36708, 2.000000000000001776 ) ;
#15752=ADVANCED_FACE ( 'NONE', ( #9997 ), #35694, .F. ) ;
#15753=CARTESIAN_POINT ( 'NONE',  ( -52.00000337463110611, -69.28203230275519786, 12.50000000000000000 ) ) ;
#15754=CARTESIAN_POINT ( 'NONE',  ( -62.97617850287781494, -4.279621169095772615, -4.999999999999997335 ) ) ;
#15755=CIRCLE ( 'NONE', #8556, 2.000000000000001776 ) ;
#15756=DIRECTION ( 'NONE',  ( 1.000000000000000000, 0.000000000000000000, 0.000000000000000000 ) ) ;
#15757=ORIENTED_EDGE ( 'NONE', *, *, #7768, .T. ) ;
#15758=LINE ( 'NONE', #35640, #17162 ) ;
#15761=EDGE_CURVE ( 'NONE', #8015, #14529, #7636, .T. ) ;
#15762=CARTESIAN_POINT ( 'NONE',  ( 4.220257619726806020, 79.78402657284750887, -5.000000000000000000 ) ) ;
#15763=AXIS2_PLACEMENT_3D ( 'NONE', #28023, #33479, #7408 ) ;
#15764=EDGE_LOOP ( 'NONE', ( #16141, #399 ) ) ;
#15765=CARTESIAN_POINT ( 'NONE',  ( 64.99999662536842493, 43.30127018922200222, -5.000000000000000000 ) ) ;
#15766=AXIS2_PLACEMENT_3D ( 'NONE', #12312, #27326, #15708 ) ;
#15768=EDGE_CURVE ( 'NONE', #19731, #2354, #16630, .T. ) ;
#15771=ORIENTED_EDGE ( 'NONE', *, *, #5521, .T. ) ;
#15774=FACE_OUTER_BOUND ( 'NONE', #23028, .T. ) ;
#15775=CIRCLE ( 'NONE', #33746, 1.999999999999998224 ) ;
#15776=FACE_BOUND ( 'NONE', #36621, .T. ) ;
#15778=DIRECTION ( 'NONE',  ( 0.000000000000000000, 0.000000000000000000, 1.000000000000000000 ) ) ;
#15779=DIRECTION ( 'NONE',  ( 0.000000000000000000, 0.000000000000000000, 1.000000000000000000 ) ) ;
#15781=DIRECTION ( 'NONE',  ( 1.000000000000000000, 0.000000000000000000, 0.000000000000000000 ) ) ;
#15783=EDGE_CURVE ( 'NONE', #10643, #23885, #12398, .T. ) ;
#15785=CARTESIAN_POINT ( 'NONE',  ( 20.39230124433451152, -84.64139349818795210, 12.50000000000000000 ) ) ;
#15786=ORIENTED_EDGE ( 'NONE', *, *, #10048, .T. ) ;
#15787=DIRECTION ( 'NONE',  ( 0.000000000000000000, 0.000000000000000000, -1.000000000000000000 ) ) ;
#15788=DIRECTION ( 'NONE',  ( -1.000000000000000000, 0.000000000000000000, 0.000000000000000000 ) ) ;
#15789=ORIENTED_EDGE ( 'NONE', *, *, #22199, .F. ) ;
#15790=EDGE_CURVE ( 'NONE', #30459, #12033, #10633, .T. ) ;
#15791=CIRCLE ( 'NONE', #9815, 2.000000000000001776 ) ;
#15792=ORIENTED_EDGE ( 'NONE', *, *, #35156, .F. ) ;
#15793=EDGE_CURVE ( 'NONE', #13489, #210, #7372, .T. ) ;
#15794=PLANE ( 'NONE',  #24097 ) ;
#15795=DIRECTION ( 'NONE',  ( 0.000000000000000000, 0.000000000000000000, -1.000000000000000000 ) ) ;
#15798=EDGE_LOOP ( 'NONE', ( #17019, #9960, #14075, #21557 ) ) ;
#15799=VERTEX_POINT ( 'NONE', #4568 ) ;
#15801=DIRECTION ( 'NONE',  ( 0.000000000000000000, 0.000000000000000000, 1.000000000000000000 ) ) ;
#15804=FACE_BOUND ( 'NONE', #13394, .T. ) ;
#15805=ORIENTED_EDGE ( 'NONE', *, *, #8831, .F. ) ;
#15806=EDGE_LOOP ( 'NONE', ( #17754, #10288, #24876, #25953 ) ) ;
#15807=DIRECTION ( 'NONE',  ( 0.000000000000000000, 0.000000000000000000, -1.000000000000000000 ) ) ;
#15808=ADVANCED_FACE ( 'NONE', ( #16198 ), #27617, .F. ) ;
#15809=LINE ( 'NONE', #10556, #8673 ) ;
#15810=EDGE_LOOP ( 'NONE', ( #31873, #22988, #15378, #11044 ) ) ;
#15811=ORIENTED_EDGE ( 'NONE', *, *, #10394, .F. ) ;
#15812=DIRECTION ( 'NONE',  ( 0.000000000000000000, 0.000000000000000000, 1.000000000000000000 ) ) ;
#15813=DIRECTION ( 'NONE',  ( 0.000000000000000000, 0.000000000000000000, 1.000000000000000000 ) ) ;
#15814=LINE ( 'NONE', #15256, #2510 ) ;
#15815=DIRECTION ( 'NONE',  ( 0.000000000000000000, 0.000000000000000000, 1.000000000000000000 ) ) ;
#15816=AXIS2_PLACEMENT_3D ( 'NONE', #15283, #23933, #18486 ) ;
#15817=VERTEX_POINT ( 'NONE', #7755 ) ;
#15818=FACE_OUTER_BOUND ( 'NONE', #25171, .T. ) ;
#15820=FACE_OUTER_BOUND ( 'NONE', #20331, .T. ) ;
#15821=FACE_OUTER_BOUND ( 'NONE', #4202, .T. ) ;
#15822=DIRECTION ( 'NONE',  ( 1.000000000000000000, 0.000000000000000000, 0.000000000000000000 ) ) ;
#15823=CARTESIAN_POINT ( 'NONE',  ( -72.00000337463102085, -34.64101615137762025, -9.999999999999998224 ) ) ;
#15824=CARTESIAN_POINT ( 'NONE',  ( 89.67878100130370456, -27.78182860042797131, -4.999999999999997335 ) ) ;
#15825=VECTOR ( 'NONE', #10506, 1000.000000000000000 ) ;
#15827=CARTESIAN_POINT ( 'NONE',  ( 72.99999662536836809, 43.30127018922198801, 17.49999999999999645 ) ) ;
#15828=AXIS2_PLACEMENT_3D ( 'NONE', #29248, #20809, #26614 ) ;
#15829=DIRECTION ( 'NONE',  ( -1.000000000000000000, 0.000000000000000000, 0.000000000000000000 ) ) ;
#15830=EDGE_LOOP ( 'NONE', ( #35737, #2476, #34772, #4933, #6409, #18245 ) ) ;
#15831=EDGE_CURVE ( 'NONE', #9610, #19401, #30996, .T. ) ;
#15832=CARTESIAN_POINT ( 'NONE',  ( -65.00000337463102085, 25.98076211353317433, -9.999999999999998224 ) ) ;
#15834=CARTESIAN_POINT ( 'NONE',  ( 86.99999662536831124, -25.98076211353319565, -9.999999999999998224 ) ) ;
#15835=ORIENTED_EDGE ( 'NONE', *, *, #27545, .F. ) ;
#15836=EDGE_CURVE ( 'NONE', #9631, #7182, #13031, .T. ) ;
#15837=VERTEX_POINT ( 'NONE', #25548 ) ;
#15838=ORIENTED_EDGE ( 'NONE', *, *, #21004, .F. ) ;
#15839=DIRECTION ( 'NONE',  ( -0.000000000000000000, -0.000000000000000000, -1.000000000000000000 ) ) ;
#15840=DIRECTION ( 'NONE',  ( 0.000000000000000000, 0.000000000000000000, 1.000000000000000000 ) ) ;
#15841=DIRECTION ( 'NONE',  ( 1.000000000000000000, 0.000000000000000000, 0.000000000000000000 ) ) ;
#15842=CIRCLE ( 'NONE', #36795, 2.000000000000001776 ) ;
#15843=EDGE_CURVE ( 'NONE', #30108, #6520, #17820, .T. ) ;
#15844=ORIENTED_EDGE ( 'NONE', *, *, #24914, .T. ) ;
#15845=EDGE_CURVE ( 'NONE', #20137, #5193, #11239, .T. ) ;
#15846=AXIS2_PLACEMENT_3D ( 'NONE', #9748, #21184, #32616 ) ;
#15847=CARTESIAN_POINT ( 'NONE',  ( -80.00000337463096400, -34.64101615137762025, 12.50000000000000000 ) ) ;
#15848=DIRECTION ( 'NONE',  ( 1.000000000000000000, 0.000000000000000000, 0.000000000000000000 ) ) ;
#15849=ORIENTED_EDGE ( 'NONE', *, *, #22229, .F. ) ;
#15850=CARTESIAN_POINT ( 'NONE',  ( -35.00000337463116296, -60.62177826491080168, -5.000000000000000000 ) ) ;
#15851=ORIENTED_EDGE ( 'NONE', *, *, #35904, .T. ) ;
#15852=CARTESIAN_POINT ( 'NONE',  ( 12.99999662536859901, 77.94228634059957983, -5.000000000000000000 ) ) ;
#15853=EDGE_CURVE ( 'NONE', #13150, #20921, #22747, .T. ) ;
#15854=CIRCLE ( 'NONE', #33213, 1.999999999999998224 ) ;
#15855=AXIS2_PLACEMENT_3D ( 'NONE', #3351, #22869, #20578 ) ;
#15856=EDGE_CURVE ( 'NONE', #17677, #6799, #18451, .T. ) ;
#15857=CARTESIAN_POINT ( 'NONE',  ( 72.99999662536835388, -43.30127018922199511, -9.999999999999998224 ) ) ;
#15858=DIRECTION ( 'NONE',  ( 0.000000000000000000, 0.000000000000000000, 1.000000000000000000 ) ) ;
#15859=ADVANCED_FACE ( 'NONE', ( #28533 ), #34189, .F. ) ;
#15860=VECTOR ( 'NONE', #4313, 1000.000000000000000 ) ;
#15861=EDGE_CURVE ( 'NONE', #15313, #26527, #34624, .T. ) ;
#15862=DIRECTION ( 'NONE',  ( 1.000000000000000000, -0.000000000000000000, 0.000000000000000000 ) ) ;
#15863=EDGE_LOOP ( 'NONE', ( #24438, #18203, #34252, #26980 ) ) ;
#15864=DIRECTION ( 'NONE',  ( 1.000000000000000000, 0.000000000000000000, 0.000000000000000000 ) ) ;
#15866=CARTESIAN_POINT ( 'NONE',  ( 49.99999662536848177, -51.96152422706640550, -9.999999999999998224 ) ) ;
#15867=CIRCLE ( 'NONE', #275, 3.000000000000002665 ) ;
#15868=DIRECTION ( 'NONE',  ( 1.000000000000000000, 0.000000000000000000, -0.000000000000000000 ) ) ;
#15869=DIRECTION ( 'NONE',  ( 0.000000000000000000, 0.000000000000000000, 1.000000000000000000 ) ) ;
#15870=VERTEX_POINT ( 'NONE', #22188 ) ;
#15871=DIRECTION ( 'NONE',  ( 0.000000000000000000, 0.000000000000000000, 1.000000000000000000 ) ) ;
#15872=AXIS2_PLACEMENT_3D ( 'NONE', #32698, #12807, #18471 ) ;
#15874=DIRECTION ( 'NONE',  ( 0.000000000000000000, 0.000000000000000000, 1.000000000000000000 ) ) ;
#15875=AXIS2_PLACEMENT_3D ( 'NONE', #23029, #31992, #29006 ) ;
#15876=ORIENTED_EDGE ( 'NONE', *, *, #17191, .T. ) ;
#15877=EDGE_LOOP ( 'NONE', ( #3099, #17813, #10188, #28890 ) ) ;
#15878=LINE ( 'NONE', #7437, #18958 ) ;
#15879=CARTESIAN_POINT ( 'NONE',  ( -77.00000337463097821, -8.660254037844422825, -9.999999999999998224 ) ) ;
#15881=AXIS2_PLACEMENT_3D ( 'NONE', #14696, #8900, #20334 ) ;
#15882=DIRECTION ( 'NONE',  ( 1.000000000000000000, 0.000000000000000000, 0.000000000000000000 ) ) ;
#15884=DIRECTION ( 'NONE',  ( 0.000000000000000000, 0.000000000000000000, -1.000000000000000000 ) ) ;
#15885=LINE ( 'NONE', #12684, #325 ) ;
#15886=CARTESIAN_POINT ( 'NONE',  ( 71.99999662536841072, 51.96152422706640550, -9.999999999999998224 ) ) ;
#15887=FACE_OUTER_BOUND ( 'NONE', #27535, .T. ) ;
#15888=EDGE_LOOP ( 'NONE', ( #8305, #14245 ) ) ;
#15889=ORIENTED_EDGE ( 'NONE', *, *, #26511, .T. ) ;
#15890=CARTESIAN_POINT ( 'NONE',  ( 47.99999662536846756, 69.28203230275516944, 12.50000000000000000 ) ) ;
#15891=AXIS2_PLACEMENT_3D ( 'NONE', #30069, #4225, #7944 ) ;
#15892=CARTESIAN_POINT ( 'NONE',  ( 64.99999662536841072, -25.98076211353320275, -5.000000000000000000 ) ) ;
#15893=ORIENTED_EDGE ( 'NONE', *, *, #22390, .T. ) ;
#15895=DIRECTION ( 'NONE',  ( -1.000000000000000000, 0.000000000000000000, 0.000000000000000000 ) ) ;
#15896=VERTEX_POINT ( 'NONE', #5659 ) ;
#15897=DIRECTION ( 'NONE',  ( 0.000000000000000000, 0.000000000000000000, 1.000000000000000000 ) ) ;
#15898=CIRCLE ( 'NONE', #327, 2.000000000000001776 ) ;
#15899=AXIS2_PLACEMENT_3D ( 'NONE', #24336, #28069, #16443 ) ;
#15900=CYLINDRICAL_SURFACE ( 'NONE', #1744, 2.000000000000000000 ) ;
#15901=VERTEX_POINT ( 'NONE', #31337 ) ;
#15902=ORIENTED_EDGE ( 'NONE', *, *, #2909, .T. ) ;
#15903=EDGE_CURVE ( 'NONE', #6458, #28343, #11840, .T. ) ;
#15904=CARTESIAN_POINT ( 'NONE',  ( 32.49191361593954497, 89.27079897466093428, -5.000000000000000000 ) ) ;
#15905=VERTEX_POINT ( 'NONE', #5319 ) ;
#15907=CARTESIAN_POINT ( 'NONE',  ( -43.19957991610399972, -47.04203867989563292, 12.49999999999999822 ) ) ;
#15908=DIRECTION ( 'NONE',  ( -1.000000000000000000, 0.000000000000000000, 0.000000000000000000 ) ) ;
#15909=LINE ( 'NONE', #20981, #28671 ) ;
#15910=ORIENTED_EDGE ( 'NONE', *, *, #8345, .F. ) ;
#15911=DIRECTION ( 'NONE',  ( -1.000000000000000000, 0.000000000000000000, 0.000000000000000000 ) ) ;
#15912=DIRECTION ( 'NONE',  ( 0.000000000000000000, 0.000000000000000000, 1.000000000000000000 ) ) ;
#15913=DIRECTION ( 'NONE',  ( 0.000000000000000000, 0.000000000000000000, -1.000000000000000000 ) ) ;
#15914=ORIENTED_EDGE ( 'NONE', *, *, #22353, .T. ) ;
#15915=VERTEX_POINT ( 'NONE', #27986 ) ;
#15919=CARTESIAN_POINT ( 'NONE',  ( 35.19434990244975126, -52.39915983220758022, -49.22241343995298024 ) ) ;
#15920=VERTEX_POINT ( 'NONE', #25197 ) ;
#15921=AXIS2_PLACEMENT_3D ( 'NONE', #28502, #30950, #22716 ) ;
#15922=CARTESIAN_POINT ( 'NONE',  ( 12.99999662536859901, 77.94228634059957983, 12.50000000000000000 ) ) ;
#15924=DIRECTION ( 'NONE',  ( 0.000000000000000000, 0.000000000000000000, 1.000000000000000000 ) ) ;
#15927=AXIS2_PLACEMENT_3D ( 'NONE', #18671, #26537, #32359 ) ;
#15930=AXIS2_PLACEMENT_3D ( 'NONE', #32705, #35722, #1226 ) ;
#15931=CARTESIAN_POINT ( 'NONE',  ( -58.00000337463107059, -34.64101615137762025, -9.999999999999998224 ) ) ;
#15932=CARTESIAN_POINT ( 'NONE',  ( -25.00000337463121980, -77.94228634059963667, 12.50000000000000000 ) ) ;
#15934=DIRECTION ( 'NONE',  ( 0.000000000000000000, 0.000000000000000000, 1.000000000000000000 ) ) ;
#15935=CARTESIAN_POINT ( 'NONE',  ( -78.00000337463094979, 34.64101615137757051, 17.49999999999999645 ) ) ;
#15936=EDGE_LOOP ( 'NONE', ( #36829, #7361, #4873, #12423 ) ) ;
#15937=CIRCLE ( 'NONE', #32677, 33.00000000000002132 ) ;
#15938=VERTEX_POINT ( 'NONE', #25359 ) ;
#15939=EDGE_CURVE ( 'NONE', #1757, #12432, #36792, .T. ) ;
#15940=CYLINDRICAL_SURFACE ( 'NONE', #26620, 2.000000000000001776 ) ;
#15941=LINE ( 'NONE', #16143, #19358 ) ;
#15942=CARTESIAN_POINT ( 'NONE',  ( 51.99999662536847467, 69.28203230275516944, -9.999999999999998224 ) ) ;
#15943=CARTESIAN_POINT ( 'NONE',  ( 77.99999662536833966, -3.224517592124143893E-15, -9.999999999999998224 ) ) ;
#15945=CIRCLE ( 'NONE', #36899, 2.000000000000001776 ) ;
#15946=DIRECTION ( 'NONE',  ( 0.000000000000000000, 0.000000000000000000, 1.000000000000000000 ) ) ;
#15947=DIRECTION ( 'NONE',  ( 0.000000000000000000, 0.000000000000000000, 1.000000000000000000 ) ) ;
#15948=AXIS2_PLACEMENT_3D ( 'NONE', #22514, #36595, #5629 ) ;
#15949=DIRECTION ( 'NONE',  ( 1.000000000000000000, 0.000000000000000000, 0.000000000000000000 ) ) ;
#15950=ORIENTED_EDGE ( 'NONE', *, *, #16749, .T. ) ;
#15951=ADVANCED_FACE ( 'NONE', ( #17100 ), #25748, .T. ) ;
#15952=CARTESIAN_POINT ( 'NONE',  ( 16.99999662536863454, -77.94228634059960825, -9.999999999999998224 ) ) ;
#15953=VERTEX_POINT ( 'NONE', #4316 ) ;
#15954=AXIS2_PLACEMENT_3D ( 'NONE', #31021, #28374, #16588 ) ;
#15956=VECTOR ( 'NONE', #10312, 1000.000000000000000 ) ;
#15957=DIRECTION ( 'NONE',  ( 0.000000000000000000, 0.000000000000000000, -1.000000000000000000 ) ) ;
#15958=VECTOR ( 'NONE', #4787, 1000.000000000000000 ) ;
#15959=CARTESIAN_POINT ( 'NONE',  ( -68.00000337463099243, -2.428612866367529932E-14, 17.49999999999999645 ) ) ;
#15960=AXIS2_PLACEMENT_3D ( 'NONE', #31973, #3320, #34658 ) ;
#15961=CARTESIAN_POINT ( 'NONE',  ( -15.00000337463125710, -77.94228634059960825, -9.999999999999998224 ) ) ;
#15962=VERTEX_POINT ( 'NONE', #27917 ) ;
#15964=VECTOR ( 'NONE', #1748, 1000.000000000000000 ) ;
#15965=ORIENTED_EDGE ( 'NONE', *, *, #23552, .F. ) ;
#15967=EDGE_CURVE ( 'NONE', #16244, #27148, #27433, .T. ) ;
#15969=CARTESIAN_POINT ( 'NONE',  ( 19.99999662536861678, -86.60254037844400443, 12.50000000000000000 ) ) ;
#15970=FACE_OUTER_BOUND ( 'NONE', #6076, .T. ) ;
#15974=DIRECTION ( 'NONE',  ( 0.000000000000000000, 0.000000000000000000, 1.000000000000000000 ) ) ;
#15975=AXIS2_PLACEMENT_3D ( 'NONE', #26101, #20298, #12187 ) ;
#15976=CARTESIAN_POINT ( 'NONE',  ( -68.00000337463100664, -17.32050807568882078, -9.999999999999998224 ) ) ;
#15977=AXIS2_PLACEMENT_3D ( 'NONE', #21918, #35450, #35822 ) ;
#15979=SURFACE_SIDE_STYLE ('',( #16175 ) ) ;
#15980=ORIENTED_EDGE ( 'NONE', *, *, #12567, .T. ) ;
#15981=CARTESIAN_POINT ( 'NONE',  ( 61.53067111003264955, -72.28378166041994746, -4.999999999999997335 ) ) ;
#15982=EDGE_CURVE ( 'NONE', #29268, #25160, #24747, .T. ) ;
#15984=DIRECTION ( 'NONE',  ( 0.000000000000000000, 0.000000000000000000, 1.000000000000000000 ) ) ;
#15986=VERTEX_POINT ( 'NONE', #15746 ) ;
#15989=ADVANCED_FACE ( 'NONE', ( #16482 ), #27368, .F. ) ;
#15990=DIRECTION ( 'NONE',  ( 1.000000000000000000, 0.000000000000000000, 0.000000000000000000 ) ) ;
#15992=DIRECTION ( 'NONE',  ( 0.000000000000000000, 0.000000000000000000, -1.000000000000000000 ) ) ;
#15993=ORIENTED_EDGE ( 'NONE', *, *, #531, .T. ) ;
#15994=ORIENTED_EDGE ( 'NONE', *, *, #20823, .F. ) ;
#15995=ORIENTED_EDGE ( 'NONE', *, *, #3892, .T. ) ;
#15997=FACE_BOUND ( 'NONE', #31915, .T. ) ;
#15998=ORIENTED_EDGE ( 'NONE', *, *, #35796, .F. ) ;
#15999=VECTOR ( 'NONE', #9263, 1000.000000000000000 ) ;
#16001=ORIENTED_EDGE ( 'NONE', *, *, #4319, .F. ) ;
#16002=CIRCLE ( 'NONE', #20772, 2.000000000000001776 ) ;
#16003=AXIS2_PLACEMENT_3D ( 'NONE', #34154, #36590, #31140 ) ;
#16005=ADVANCED_FACE ( 'NONE', ( #33571 ), #36012, .T. ) ;
#16007=CIRCLE ( 'NONE', #32779, 2.000000000000001776 ) ;
#16008=DIRECTION ( 'NONE',  ( 0.000000000000000000, 0.000000000000000000, 1.000000000000000000 ) ) ;
#16010=EDGE_LOOP ( 'NONE', ( #18634, #5159 ) ) ;
#16011=CYLINDRICAL_SURFACE ( 'NONE', #9521, 2.000000000000001776 ) ;
#16013=EDGE_CURVE ( 'NONE', #12099, #36951, #24449, .T. ) ;
#16016=CARTESIAN_POINT ( 'NONE',  ( 42.99999662536850309, 77.94228634059959404, -9.999999999999998224 ) ) ;
#16017=AXIS2_PLACEMENT_3D ( 'NONE', #14910, #29337, #9654 ) ;
#16018=VERTEX_POINT ( 'NONE', #18748 ) ;
#16019=DIRECTION ( 'NONE',  ( 0.000000000000000000, 0.000000000000000000, 1.000000000000000000 ) ) ;
#16020=EDGE_CURVE ( 'NONE', #21899, #1410, #4498, .T. ) ;
#16021=EDGE_LOOP ( 'NONE', ( #19251, #5585 ) ) ;
#16023=DIRECTION ( 'NONE',  ( 1.000000000000000000, 0.000000000000000000, 0.000000000000000000 ) ) ;
#16024=CARTESIAN_POINT ( 'NONE',  ( 0.000000000000000000, 0.000000000000000000, 12.49999999999999822 ) ) ;
#16025=CIRCLE ( 'NONE', #35774, 2.000000000000001776 ) ;
#16026=DIRECTION ( 'NONE',  ( -0.000000000000000000, -0.000000000000000000, -1.000000000000000000 ) ) ;
#16027=LINE ( 'NONE', #24652, #31995 ) ;
#16029=DIRECTION ( 'NONE',  ( 1.000000000000000000, 0.000000000000000000, 0.000000000000000000 ) ) ;
#16030=VERTEX_POINT ( 'NONE', #25135 ) ;
#16032=CIRCLE ( 'NONE', #15407, 2.000000000000001776 ) ;
#16033=DIRECTION ( 'NONE',  ( 1.000000000000000000, 0.000000000000000000, 0.000000000000000000 ) ) ;
#16034=DIRECTION ( 'NONE',  ( 0.000000000000000000, 0.000000000000000000, -1.000000000000000000 ) ) ;
#16035=CIRCLE ( 'NONE', #17236, 2.000000000000001776 ) ;
#16037=VERTEX_POINT ( 'NONE', #15935 ) ;
#16038=VERTEX_POINT ( 'NONE', #7490 ) ;
#16039=ADVANCED_FACE ( 'NONE', ( #13127 ), #13474, .F. ) ;
#16041=CARTESIAN_POINT ( 'NONE',  ( -3.374631303565411855E-06, -86.60254037844400443, -9.999999999999998224 ) ) ;
#16042=CARTESIAN_POINT ( 'NONE',  ( -60.00000337463104216, 51.96152422706639129, -9.999999999999998224 ) ) ;
#16043=EDGE_LOOP ( 'NONE', ( #13916, #20965 ) ) ;
#16044=CIRCLE ( 'NONE', #22004, 2.000000000000001776 ) ;
#16045=AXIS2_PLACEMENT_3D ( 'NONE', #36838, #34401, #5911 ) ;
#16046=DIRECTION ( 'NONE',  ( 0.000000000000000000, 0.000000000000000000, 1.000000000000000000 ) ) ;
#16047=DIRECTION ( 'NONE',  ( 0.000000000000000000, 0.000000000000000000, 1.000000000000000000 ) ) ;
#16048=ORIENTED_EDGE ( 'NONE', *, *, #18685, .T. ) ;
#16049=DIRECTION ( 'NONE',  ( 0.000000000000000000, 0.000000000000000000, 1.000000000000000000 ) ) ;
#16050=VERTEX_POINT ( 'NONE', #36183 ) ;
#16051=CARTESIAN_POINT ( 'NONE',  ( -20.00000337463122690, 86.60254037844397601, -9.999999999999998224 ) ) ;
#16052=EDGE_CURVE ( 'NONE', #6561, #36949, #1694, .T. ) ;
#16053=DIRECTION ( 'NONE',  ( 1.000000000000000000, 0.000000000000000000, 0.000000000000000000 ) ) ;
#16054=CARTESIAN_POINT ( 'NONE',  ( -50.00000337463110611, -69.28203230275519786, -5.000000000000000000 ) ) ;
#16055=CIRCLE ( 'NONE', #20244, 33.00000000000001421 ) ;
#16057=EDGE_CURVE ( 'NONE', #29683, #9216, #21737, .T. ) ;
#16058=ORIENTED_EDGE ( 'NONE', *, *, #15056, .F. ) ;
#16060=AXIS2_PLACEMENT_3D ( 'NONE', #17185, #29163, #14729 ) ;
#16061=AXIS2_PLACEMENT_3D ( 'NONE', #28902, #23305, #3228 ) ;
#16063=CIRCLE ( 'NONE', #1087, 2.000000000000001776 ) ;
#16065=CARTESIAN_POINT ( 'NONE',  ( 76.99999662536835388, -25.98076211353319565, -9.999999999999998224 ) ) ;
#16069=DIRECTION ( 'NONE',  ( 1.000000000000000000, 0.000000000000000000, 0.000000000000000000 ) ) ;
#16071=DIRECTION ( 'NONE',  ( 0.000000000000000000, 0.000000000000000000, 1.000000000000000000 ) ) ;
#16072=EDGE_CURVE ( 'NONE', #24009, #22036, #19140, .T. ) ;
#16074=DIRECTION ( 'NONE',  ( 0.000000000000000000, 0.000000000000000000, -1.000000000000000000 ) ) ;
#16075=EDGE_CURVE ( 'NONE', #13023, #17723, #16310, .T. ) ;
#16076=CIRCLE ( 'NONE', #15448, 33.00000000000001421 ) ;
#16077=VERTEX_POINT ( 'NONE', #24937 ) ;
#16078=ORIENTED_EDGE ( 'NONE', *, *, #10471, .T. ) ;
#16079=FACE_OUTER_BOUND ( 'NONE', #20822, .T. ) ;
#16080=AXIS2_PLACEMENT_3D ( 'NONE', #17844, #21348, #1666 ) ;
#16081=CYLINDRICAL_SURFACE ( 'NONE', #28498, 2.000000000000001776 ) ;
#16082=ADVANCED_FACE ( 'NONE', ( #21373 ), #32816, .F. ) ;
#16083=ADVANCED_FACE ( 'NONE', ( #22473 ), #5246, .F. ) ;
#16084=DIRECTION ( 'NONE',  ( 1.000000000000000000, 0.000000000000000000, 0.000000000000000000 ) ) ;
#16085=ORIENTED_EDGE ( 'NONE', *, *, #18809, .T. ) ;
#16086=EDGE_CURVE ( 'NONE', #18552, #18736, #14226, .T. ) ;
#16087=CIRCLE ( 'NONE', #26268, 33.00000000000001421 ) ;
#16088=FACE_OUTER_BOUND ( 'NONE', #21283, .T. ) ;
#16091=AXIS2_PLACEMENT_3D ( 'NONE', #28309, #2632, #28694 ) ;
#16093=DIRECTION ( 'NONE',  ( 1.000000000000000000, 0.000000000000000000, 0.000000000000000000 ) ) ;
#16094=VERTEX_POINT ( 'NONE', #28111 ) ;
#16097=CARTESIAN_POINT ( 'NONE',  ( -53.00000337463106348, 60.62177826491078747, -9.999999999999998224 ) ) ;
#16099=CARTESIAN_POINT ( 'NONE',  ( -20.00000337463124112, 69.28203230275516944, 12.50000000000000000 ) ) ;
#16100=VERTEX_POINT ( 'NONE', #19677 ) ;
#16101=CARTESIAN_POINT ( 'NONE',  ( -45.00000337463111322, 60.62177826491077326, -9.999999999999998224 ) ) ;
#16102=ORIENTED_EDGE ( 'NONE', *, *, #15783, .T. ) ;
#16106=EDGE_CURVE ( 'NONE', #16140, #8932, #22650, .T. ) ;
#16107=CARTESIAN_POINT ( 'NONE',  ( 90.60231327712337190, 15.97563234535636134, 12.49999999999999822 ) ) ;
#16108=VERTEX_POINT ( 'NONE', #14580 ) ;
#16109=DIRECTION ( 'NONE',  ( 0.000000000000000000, 0.000000000000000000, 1.000000000000000000 ) ) ;
#16110=ORIENTED_EDGE ( 'NONE', *, *, #21202, .F. ) ;
#16112=AXIS2_PLACEMENT_3D ( 'NONE', #15549, #24160, #35611 ) ;
#16113=DIRECTION ( 'NONE',  ( 0.000000000000000000, 0.000000000000000000, 1.000000000000000000 ) ) ;
#16114=PLANE ( 'NONE',  #22718 ) ;
#16115=EDGE_LOOP ( 'NONE', ( #15226, #29129, #14117, #8324 ) ) ;
#16116=CYLINDRICAL_SURFACE ( 'NONE', #17853, 2.000000000000001776 ) ;
#16117=EDGE_CURVE ( 'NONE', #9506, #4700, #2600, .T. ) ;
#16122=EDGE_LOOP ( 'NONE', ( #2044, #16160, #27973, #29475 ) ) ;
#16124=CIRCLE ( 'NONE', #29860, 3.000000000000007994 ) ;
#16125=DIRECTION ( 'NONE',  ( 1.000000000000000000, 0.000000000000000000, 0.000000000000000000 ) ) ;
#16128=DIRECTION ( 'NONE',  ( 0.000000000000000000, 0.000000000000000000, 1.000000000000000000 ) ) ;
#16130=EDGE_CURVE ( 'NONE', #545, #6597, #8242, .T. ) ;
#16131=DIRECTION ( 'NONE',  ( -1.000000000000000000, 0.000000000000000000, 0.000000000000000000 ) ) ;
#16132=CIRCLE ( 'NONE', #25128, 3.000000000000007105 ) ;
#16134=EDGE_CURVE ( 'NONE', #29294, #22278, #25299, .T. ) ;
#16135=DIRECTION ( 'NONE',  ( 0.000000000000000000, 0.000000000000000000, 1.000000000000000000 ) ) ;
#16136=CIRCLE ( 'NONE', #36507, 27.00000000000001421 ) ;
#16137=CARTESIAN_POINT ( 'NONE',  ( 71.99999662536839651, 17.32050807568879236, -9.999999999999998224 ) ) ;
#16140=VERTEX_POINT ( 'NONE', #8781 ) ;
#16141=ORIENTED_EDGE ( 'NONE', *, *, #24241, .T. ) ;
#16142=VECTOR ( 'NONE', #35572, 1000.000000000000000 ) ;
#16143=CARTESIAN_POINT ( 'NONE',  ( -62.00000337463104927, 51.96152422706639129, -9.999999999999998224 ) ) ;
#16144=CYLINDRICAL_SURFACE ( 'NONE', #24657, 2.000000000000001776 ) ;
#16145=CARTESIAN_POINT ( 'NONE',  ( -75.00000337463097821, -8.660254037844422825, 12.50000000000000000 ) ) ;
#16146=EDGE_LOOP ( 'NONE', ( #28383, #28382, #5033, #20186 ) ) ;
#16147=AXIS2_PLACEMENT_3D ( 'NONE', #11304, #10559, #25552 ) ;
#16148=DIRECTION ( 'NONE',  ( 0.000000000000000000, 0.000000000000000000, 1.000000000000000000 ) ) ;
#16149=CARTESIAN_POINT ( 'NONE',  ( -90.00000337463090716, -1.040834085586084257E-14, -9.999999999999998224 ) ) ;
#16151=AXIS2_PLACEMENT_3D ( 'NONE', #20928, #12829, #15670 ) ;
#16153=VERTEX_POINT ( 'NONE', #8592 ) ;
#16155=LINE ( 'NONE', #27583, #10914 ) ;
#16156=DIRECTION ( 'NONE',  ( 0.000000000000000000, 0.000000000000000000, 1.000000000000000000 ) ) ;
#16157=CIRCLE ( 'NONE', #26926, 2.000000000000001776 ) ;
#16158=CARTESIAN_POINT ( 'NONE',  ( -58.88972745734203329, -33.99999999999965894, -4.999999999999997335 ) ) ;
#16159=ORIENTED_EDGE ( 'NONE', *, *, #717, .F. ) ;
#16160=ORIENTED_EDGE ( 'NONE', *, *, #11430, .T. ) ;
#16161=AXIS2_PLACEMENT_3D ( 'NONE', #9164, #14611, #25876 ) ;
#16164=DIRECTION ( 'NONE',  ( -1.000000000000000000, -8.737866397512800437E-15, 0.000000000000000000 ) ) ;
#16165=CIRCLE ( 'NONE', #12522, 2.000000000000001776 ) ;
#16166=CARTESIAN_POINT ( 'NONE',  ( 62.99999662536842493, 43.30127018922200222, 17.49999999999999645 ) ) ;
#16167=CIRCLE ( 'NONE', #17366, 2.000000000000001776 ) ;
#16168=DIRECTION ( 'NONE',  ( -1.000000000000000000, 0.000000000000000000, 0.000000000000000000 ) ) ;
#16170=LINE ( 'NONE', #27200, #14732 ) ;
#16171=ORIENTED_EDGE ( 'NONE', *, *, #10268, .T. ) ;
#16173=FACE_OUTER_BOUND ( 'NONE', #35437, .T. ) ;
#16174=EDGE_CURVE ( 'NONE', #30738, #7932, #16076, .T. ) ;
#16175=SURFACE_STYLE_FILL_AREA ( #4913 ) ;
#16176=ORIENTED_EDGE ( 'NONE', *, *, #16993, .F. ) ;
#16177=CYLINDRICAL_SURFACE ( 'NONE', #2870, 2.000000000000001776 ) ;
#16178=CARTESIAN_POINT ( 'NONE',  ( 9.999996625368625658, 86.60254037844397601, 17.49999999999999645 ) ) ;
#16179=CIRCLE ( 'NONE', #33556, 2.000000000000001776 ) ;
#16181=ORIENTED_EDGE ( 'NONE', *, *, #131, .F. ) ;
#16184=CYLINDRICAL_SURFACE ( 'NONE', #18792, 3.000000000000002665 ) ;
#16187=ORIENTED_EDGE ( 'NONE', *, *, #8723, .F. ) ;
#16188=CIRCLE ( 'NONE', #4814, 2.000000000000001776 ) ;
#16190=DIRECTION ( 'NONE',  ( 1.000000000000000000, 0.000000000000000000, 0.000000000000000000 ) ) ;
#16191=CIRCLE ( 'NONE', #3600, 2.000000000000001776 ) ;
#16192=ORIENTED_EDGE ( 'NONE', *, *, #35928, .T. ) ;
#16193=AXIS2_PLACEMENT_3D ( 'NONE', #13806, #25242, #22236 ) ;
#16194=DIRECTION ( 'NONE',  ( -1.000000000000000000, 0.000000000000000000, 0.000000000000000000 ) ) ;
#16195=ORIENTED_EDGE ( 'NONE', *, *, #9145, .T. ) ;
#16197=ORIENTED_EDGE ( 'NONE', *, *, #19403, .T. ) ;
#16198=FACE_OUTER_BOUND ( 'NONE', #25266, .T. ) ;
#16199=CARTESIAN_POINT ( 'NONE',  ( 19.99999662536861678, -86.60254037844400443, 17.49999999999999645 ) ) ;
#16200=EDGE_LOOP ( 'NONE', ( #21938, #35307, #21006, #33056 ) ) ;
#16201=EDGE_CURVE ( 'NONE', #4892, #32887, #30433, .T. ) ;
#16202=ORIENTED_EDGE ( 'NONE', *, *, #31226, .T. ) ;
#16203=DIRECTION ( 'NONE',  ( 0.000000000000000000, 0.000000000000000000, 1.000000000000000000 ) ) ;
#16204=FACE_OUTER_BOUND ( 'NONE', #10792, .T. ) ;
#16205=CARTESIAN_POINT ( 'NONE',  ( -35.00000337463116296, 77.94228634059957983, -5.000000000000000000 ) ) ;
#16206=LINE ( 'NONE', #5126, #29838 ) ;
#16207=EDGE_CURVE ( 'NONE', #31817, #17794, #7691, .T. ) ;
#16208=ORIENTED_EDGE ( 'NONE', *, *, #34757, .T. ) ;
#16210=AXIS2_PLACEMENT_3D ( 'NONE', #5468, #25174, #36599 ) ;
#16211=FACE_BOUND ( 'NONE', #9725, .T. ) ;
#16212=DIRECTION ( 'NONE',  ( 0.000000000000000000, 0.000000000000000000, 1.000000000000000000 ) ) ;
#16213=CIRCLE ( 'NONE', #32365, 33.00000000000001421 ) ;
#16215=CYLINDRICAL_SURFACE ( 'NONE', #5748, 3.000000000000002665 ) ;
#16216=DIRECTION ( 'NONE',  ( 0.000000000000000000, 0.000000000000000000, 1.000000000000000000 ) ) ;
#16217=DIRECTION ( 'NONE',  ( 1.000000000000000000, 0.000000000000000000, 0.000000000000000000 ) ) ;
#16218=EDGE_CURVE ( 'NONE', #1626, #11213, #7662, .T. ) ;
#16219=DIRECTION ( 'NONE',  ( 1.000000000000000000, 0.000000000000000000, 0.000000000000000000 ) ) ;
#16220=EDGE_LOOP ( 'NONE', ( #18193, #4364, #32530, #11362 ) ) ;
#16221=CARTESIAN_POINT ( 'NONE',  ( 0.000000000000000000, 0.000000000000000000, -5.000000000000000000 ) ) ;
#16223=DIRECTION ( 'NONE',  ( 0.000000000000000000, 0.000000000000000000, 1.000000000000000000 ) ) ;
#16224=VERTEX_POINT ( 'NONE', #20026 ) ;
#16226=ORIENTED_EDGE ( 'NONE', *, *, #26189, .F. ) ;
#16227=CYLINDRICAL_SURFACE ( 'NONE', #35799, 2.000000000000001776 ) ;
#16228=CARTESIAN_POINT ( 'NONE',  ( 37.99999662536853151, 69.28203230275518365, -5.000000000000000000 ) ) ;
#16229=ORIENTED_EDGE ( 'NONE', *, *, #26824, .F. ) ;
#16231=DIRECTION ( 'NONE',  ( 0.4999999999999919509, -0.8660254037844433705, 0.000000000000000000 ) ) ;
#16232=DIRECTION ( 'NONE',  ( 0.000000000000000000, 0.000000000000000000, 1.000000000000000000 ) ) ;
#16234=EDGE_CURVE ( 'NONE', #12760, #6161, #1071, .T. ) ;
#16236=FACE_OUTER_BOUND ( 'NONE', #3112, .T. ) ;
#16237=ORIENTED_EDGE ( 'NONE', *, *, #34193, .T. ) ;
#16238=FACE_BOUND ( 'NONE', #9296, .T. ) ;
#16239=EDGE_CURVE ( 'NONE', #2055, #14243, #31601, .T. ) ;
#16240=CARTESIAN_POINT ( 'NONE',  ( 52.39915983220795681, 35.19434990244919703, 12.49999999999999822 ) ) ;
#16241=CYLINDRICAL_SURFACE ( 'NONE', #14943, 2.000000000000001776 ) ;
#16242=FACE_OUTER_BOUND ( 'NONE', #19456, .T. ) ;
#16243=EDGE_CURVE ( 'NONE', #13116, #27668, #36415, .T. ) ;
#16244=VERTEX_POINT ( 'NONE', #9814 ) ;
#16245=DIRECTION ( 'NONE',  ( 1.000000000000000000, 0.000000000000000000, 0.000000000000000000 ) ) ;
#16247=CARTESIAN_POINT ( 'NONE',  ( 14.99999662536859901, 77.94228634059957983, -5.000000000000000000 ) ) ;
#16248=DIRECTION ( 'NONE',  ( 1.000000000000000000, 0.000000000000000000, 0.000000000000000000 ) ) ;
#16249=EDGE_CURVE ( 'NONE', #17343, #22235, #8885, .T. ) ;
#16250=ORIENTED_EDGE ( 'NONE', *, *, #9771, .T. ) ;
#16251=FACE_BOUND ( 'NONE', #12294, .T. ) ;
#16255=AXIS2_PLACEMENT_3D ( 'NONE', #28117, #5603, #5801 ) ;
#16256=FACE_OUTER_BOUND ( 'NONE', #3225, .T. ) ;
#16257=DIRECTION ( 'NONE',  ( 1.000000000000000000, 0.000000000000000000, 0.000000000000000000 ) ) ;
#16258=ORIENTED_EDGE ( 'NONE', *, *, #26135, .F. ) ;
#16260=CARTESIAN_POINT ( 'NONE',  ( 0.000000000000000000, 0.000000000000000000, -5.000000000000000000 ) ) ;
#16261=CARTESIAN_POINT ( 'NONE',  ( 76.99999662536835388, -25.98076211353319565, -9.999999999999998224 ) ) ;
#16262=DIRECTION ( 'NONE',  ( 0.000000000000000000, 0.000000000000000000, -1.000000000000000000 ) ) ;
#16263=EDGE_CURVE ( 'NONE', #7415, #5822, #1377, .T. ) ;
#16264=ORIENTED_EDGE ( 'NONE', *, *, #155, .T. ) ;
#16265=ORIENTED_EDGE ( 'NONE', *, *, #28962, .T. ) ;
#16266=DIRECTION ( 'NONE',  ( -1.000000000000000000, 0.000000000000000000, -0.000000000000000000 ) ) ;
#16270=ORIENTED_EDGE ( 'NONE', *, *, #7965, .F. ) ;
#16271=EDGE_CURVE ( 'NONE', #6061, #29798, #26510, .T. ) ;
#16272=ORIENTED_EDGE ( 'NONE', *, *, #22483, .F. ) ;
#16274=CIRCLE ( 'NONE', #15680, 65.00000000000000000 ) ;
#16276=ORIENTED_EDGE ( 'NONE', *, *, #30554, .F. ) ;
#16279=EDGE_CURVE ( 'NONE', #33654, #36096, #9077, .T. ) ;
#16280=ORIENTED_EDGE ( 'NONE', *, *, #381, .T. ) ;
#16281=AXIS2_PLACEMENT_3D ( 'NONE', #15383, #23631, #24188 ) ;
#16282=DIRECTION ( 'NONE',  ( 1.000000000000000000, 0.000000000000000000, 0.000000000000000000 ) ) ;
#16284=CARTESIAN_POINT ( 'NONE',  ( -70.00000337463099243, 51.96152422706637708, -9.999999999999998224 ) ) ;
#16285=ORIENTED_EDGE ( 'NONE', *, *, #24751, .T. ) ;
#16287=CARTESIAN_POINT ( 'NONE',  ( -56.74224907228983028, 68.66839587347264739, -4.999999999999997335 ) ) ;
#16288=EDGE_CURVE ( 'NONE', #1500, #12218, #26846, .T. ) ;
#16291=ORIENTED_EDGE ( 'NONE', *, *, #11731, .T. ) ;
#16294=CARTESIAN_POINT ( 'NONE',  ( -22.00000337463122690, 86.60254037844397601, -9.999999999999998224 ) ) ;
#16295=ORIENTED_EDGE ( 'NONE', *, *, #24770, .F. ) ;
#16296=ORIENTED_EDGE ( 'NONE', *, *, #31331, .T. ) ;
#16297=ORIENTED_EDGE ( 'NONE', *, *, #22269, .F. ) ;
#16298=AXIS2_PLACEMENT_3D ( 'NONE', #25762, #11482, #34367 ) ;
#16300=VERTEX_POINT ( 'NONE', #17899 ) ;
#16302=CYLINDRICAL_SURFACE ( 'NONE', #20199, 2.000000000000000000 ) ;
#16303=DIRECTION ( 'NONE',  ( 0.000000000000000000, 0.000000000000000000, 1.000000000000000000 ) ) ;
#16304=EDGE_CURVE ( 'NONE', #15633, #23588, #34068, .T. ) ;
#16305=CARTESIAN_POINT ( 'NONE',  ( -27.78182860042817026, -56.67878100130359087, -49.86348611802629449 ) ) ;
#16306=CARTESIAN_POINT ( 'NONE',  ( -72.00000337463100664, 34.64101615137758472, 17.49999999999999645 ) ) ;
#16308=EDGE_CURVE ( 'NONE', #10426, #18123, #2936, .T. ) ;
#16310=LINE ( 'NONE', #27727, #10073 ) ;
#16313=VERTEX_POINT ( 'NONE', #21069 ) ;
#16315=DIRECTION ( 'NONE',  ( 0.000000000000000000, 0.000000000000000000, 1.000000000000000000 ) ) ;
#16316=DIRECTION ( 'NONE',  ( 0.000000000000000000, 0.000000000000000000, -1.000000000000000000 ) ) ;
#16317=DIRECTION ( 'NONE',  ( 1.000000000000000000, 0.000000000000000000, 0.000000000000000000 ) ) ;
#16318=EDGE_CURVE ( 'NONE', #13911, #32985, #24078, .T. ) ;
#16319=VERTEX_POINT ( 'NONE', #6814 ) ;
#16320=EDGE_CURVE ( 'NONE', #29299, #30786, #21251, .T. ) ;
#16322=CARTESIAN_POINT ( 'NONE',  ( 31.09745072740910388, 83.47442710120324705, -49.86348611802629449 ) ) ;
#16323=ORIENTED_EDGE ( 'NONE', *, *, #4972, .F. ) ;
#16324=AXIS2_PLACEMENT_3D ( 'NONE', #19883, #11, #28310 ) ;
#16326=VERTEX_POINT ( 'NONE', #29681 ) ;
#16329=DIRECTION ( 'NONE',  ( 0.000000000000000000, 0.000000000000000000, -1.000000000000000000 ) ) ;
#16330=EDGE_CURVE ( 'NONE', #34395, #12253, #16206, .T. ) ;
#16331=CARTESIAN_POINT ( 'NONE',  ( -57.00000337463111322, -43.30127018922202353, -9.999999999999998224 ) ) ;
#16332=EDGE_CURVE ( 'NONE', #18228, #34315, #24481, .T. ) ;
#16333=DIRECTION ( 'NONE',  ( 0.000000000000000000, 0.000000000000000000, 1.000000000000000000 ) ) ;
#16334=EDGE_CURVE ( 'NONE', #35831, #34111, #1719, .T. ) ;
#16336=ORIENTED_EDGE ( 'NONE', *, *, #13228, .T. ) ;
#16337=ORIENTED_EDGE ( 'NONE', *, *, #36266, .T. ) ;
#16338=VERTEX_POINT ( 'NONE', #10209 ) ;
#16340=CARTESIAN_POINT ( 'NONE',  ( -86.45172111230354517, 31.46585318596159553, -4.999999999999997335 ) ) ;
#16341=CARTESIAN_POINT ( 'NONE',  ( -17.00000337463126243, 77.94228634059957983, -9.999999999999998224 ) ) ;
#16342=DIRECTION ( 'NONE',  ( 0.000000000000000000, 0.000000000000000000, 1.000000000000000000 ) ) ;
#16344=ORIENTED_EDGE ( 'NONE', *, *, #31674, .T. ) ;
#16345=DIRECTION ( 'NONE',  ( 0.000000000000000000, 0.000000000000000000, 1.000000000000000000 ) ) ;
#16346=DIRECTION ( 'NONE',  ( -1.000000000000000000, 0.000000000000000000, 0.000000000000000000 ) ) ;
#16347=ORIENTED_EDGE ( 'NONE', *, *, #21556, .F. ) ;
#16348=VECTOR ( 'NONE', #16223, 1000.000000000000000 ) ;
#16349=CARTESIAN_POINT ( 'NONE',  ( -35.00000337463116296, 60.62177826491077326, 17.49999999999999645 ) ) ;
#16350=CARTESIAN_POINT ( 'NONE',  ( 32.99999662536855283, 60.62177826491078747, -9.999999999999998224 ) ) ;
#16351=VERTEX_POINT ( 'NONE', #13001 ) ;
#16352=ORIENTED_EDGE ( 'NONE', *, *, #5654, .T. ) ;
#16353=CARTESIAN_POINT ( 'NONE',  ( 77.99999662536832545, -34.64101615137759183, 12.50000000000000000 ) ) ;
#16354=CARTESIAN_POINT ( 'NONE',  ( 11.99999662536861855, 69.28203230275516944, 12.50000000000000000 ) ) ;
#16356=VERTEX_POINT ( 'NONE', #16565 ) ;
#16357=EDGE_LOOP ( 'NONE', ( #36756, #10780, #517, #23155 ) ) ;
#16358=CIRCLE ( 'NONE', #9760, 2.000000000000001776 ) ;
#16359=DIRECTION ( 'NONE',  ( 1.000000000000000000, 0.000000000000000000, 0.000000000000000000 ) ) ;
#16361=EDGE_LOOP ( 'NONE', ( #23977, #3951, #22744, #29015 ) ) ;
#16364=ORIENTED_EDGE ( 'NONE', *, *, #1532, .F. ) ;
#16365=DIRECTION ( 'NONE',  ( 0.000000000000000000, 0.000000000000000000, -1.000000000000000000 ) ) ;
#16367=FACE_OUTER_BOUND ( 'NONE', #36059, .T. ) ;
#16368=EDGE_CURVE ( 'NONE', #3872, #21374, #1935, .T. ) ;
#16369=ORIENTED_EDGE ( 'NONE', *, *, #13088, .T. ) ;
#16374=CARTESIAN_POINT ( 'NONE',  ( 71.99999662536839651, 34.64101615137758472, -9.999999999999998224 ) ) ;
#16375=VERTEX_POINT ( 'NONE', #36075 ) ;
#16378=FACE_BOUND ( 'NONE', #13414, .T. ) ;
#16379=DIRECTION ( 'NONE',  ( 0.000000000000000000, 0.000000000000000000, 1.000000000000000000 ) ) ;
#16381=CARTESIAN_POINT ( 'NONE',  ( -30.00000337463119848, -69.28203230275522628, -9.999999999999998224 ) ) ;
#16382=DIRECTION ( 'NONE',  ( 1.000000000000000000, 0.000000000000000000, 0.000000000000000000 ) ) ;
#16383=CARTESIAN_POINT ( 'NONE',  ( -33.00000337463116296, 77.94228634059957983, 12.50000000000000000 ) ) ;
#16384=AXIS2_PLACEMENT_3D ( 'NONE', #21143, #13080, #23782 ) ;
#16385=FACE_OUTER_BOUND ( 'NONE', #15081, .T. ) ;
#16386=CARTESIAN_POINT ( 'NONE',  ( 79.99999662536832545, -34.64101615137759183, -9.999999999999998224 ) ) ;
#16387=ORIENTED_EDGE ( 'NONE', *, *, #27737, .T. ) ;
#16388=DIRECTION ( 'NONE',  ( -1.000000000000000000, 0.000000000000000000, -0.000000000000000000 ) ) ;
#16389=DIRECTION ( 'NONE',  ( 1.000000000000000000, 0.000000000000000000, 0.000000000000000000 ) ) ;
#16391=EDGE_CURVE ( 'NONE', #22972, #1373, #13555, .T. ) ;
#16392=ADVANCED_FACE ( 'NONE', ( #13197 ), #24820, .F. ) ;
#16393=AXIS2_PLACEMENT_3D ( 'NONE', #36990, #11299, #22916 ) ;
#16396=ORIENTED_EDGE ( 'NONE', *, *, #2668, .F. ) ;
#16398=CARTESIAN_POINT ( 'NONE',  ( 21.99999662536857770, 86.60254037844397601, -9.999999999999998224 ) ) ;
#16400=ORIENTED_EDGE ( 'NONE', *, *, #24311, .F. ) ;
#16401=CIRCLE ( 'NONE', #7410, 2.000000000000001776 ) ;
#16403=EDGE_CURVE ( 'NONE', #17104, #10828, #19681, .T. ) ;
#16404=LINE ( 'NONE', #33485, #26678 ) ;
#16407=ORIENTED_EDGE ( 'NONE', *, *, #25927, .F. ) ;
#16408=DIRECTION ( 'NONE',  ( -1.000000000000000000, 0.000000000000000000, 0.000000000000000000 ) ) ;
#16409=AXIS2_PLACEMENT_3D ( 'NONE', #17573, #8968, #14769 ) ;
#16411=CARTESIAN_POINT ( 'NONE',  ( 29.99999662536857770, -69.28203230275519786, -9.999999999999998224 ) ) ;
#16412=EDGE_CURVE ( 'NONE', #31817, #15730, #30465, .T. ) ;
#16413=ORIENTED_EDGE ( 'NONE', *, *, #15591, .T. ) ;
#16415=CIRCLE ( 'NONE', #36199, 27.00000000000001421 ) ;
#16417=CARTESIAN_POINT ( 'NONE',  ( -12.00000337463128908, 69.28203230275516944, -9.999999999999998224 ) ) ;
#16418=EDGE_LOOP ( 'NONE', ( #12901, #8356, #3012, #31125, #30551 ) ) ;
#16419=AXIS2_PLACEMENT_3D ( 'NONE', #24046, #977, #15613 ) ;
#16420=FACE_BOUND ( 'NONE', #24957, .T. ) ;
#16423=CARTESIAN_POINT ( 'NONE',  ( 64.99999662536839651, -60.62177826491080168, -9.999999999999998224 ) ) ;
#16424=DIRECTION ( 'NONE',  ( 0.000000000000000000, 0.000000000000000000, -1.000000000000000000 ) ) ;
#16425=DIRECTION ( 'NONE',  ( 0.000000000000000000, 0.000000000000000000, 1.000000000000000000 ) ) ;
#16426=ORIENTED_EDGE ( 'NONE', *, *, #11688, .T. ) ;
#16427=EDGE_CURVE ( 'NONE', #19893, #15625, #27466, .T. ) ;
#16428=ORIENTED_EDGE ( 'NONE', *, *, #16466, .T. ) ;
#16430=CARTESIAN_POINT ( 'NONE',  ( 64.99999662536839651, 60.62177826491078747, -9.999999999999998224 ) ) ;
#16431=CARTESIAN_POINT ( 'NONE',  ( 66.99999662536839651, -43.30127018922199511, -9.999999999999998224 ) ) ;
#16433=ORIENTED_EDGE ( 'NONE', *, *, #15047, .F. ) ;
#16434=CARTESIAN_POINT ( 'NONE',  ( -20.00000337463123756, -86.60254037844400443, 12.50000000000000000 ) ) ;
#16435=LINE ( 'NONE', #1829, #26806 ) ;
#16436=ADVANCED_FACE ( 'NONE', ( #30241 ), #19208, .F. ) ;
#16437=DIRECTION ( 'NONE',  ( 1.000000000000000000, 0.000000000000000000, 0.000000000000000000 ) ) ;
#16440=AXIS2_PLACEMENT_3D ( 'NONE', #546, #11782, #23426 ) ;
#16443=DIRECTION ( 'NONE',  ( 1.000000000000000000, 0.000000000000000000, 0.000000000000000000 ) ) ;
#16444=EDGE_CURVE ( 'NONE', #34315, #34831, #11298, .T. ) ;
#16445=VECTOR ( 'NONE', #23065, 1000.000000000000000 ) ;
#16447=ORIENTED_EDGE ( 'NONE', *, *, #5914, .T. ) ;
#16449=ORIENTED_EDGE ( 'NONE', *, *, #10090, .T. ) ;
#16450=CARTESIAN_POINT ( 'NONE',  ( -40.00000337463113453, -69.28203230275519786, -9.999999999999998224 ) ) ;
#16451=DIRECTION ( 'NONE',  ( 1.000000000000000000, 0.000000000000000000, 0.000000000000000000 ) ) ;
#16452=AXIS2_PLACEMENT_3D ( 'NONE', #23616, #29244, #32239 ) ;
#16453=VECTOR ( 'NONE', #5, 1000.000000000000000 ) ;
#16455=ORIENTED_EDGE ( 'NONE', *, *, #24523, .F. ) ;
#16457=DIRECTION ( 'NONE',  ( -1.000000000000000000, 0.000000000000000000, -0.000000000000000000 ) ) ;
#16458=EDGE_CURVE ( 'NONE', #29420, #6561, #509, .T. ) ;
#16459=DIRECTION ( 'NONE',  ( 0.000000000000000000, 0.000000000000000000, -1.000000000000000000 ) ) ;
#16460=DIRECTION ( 'NONE',  ( 1.000000000000000000, 0.000000000000000000, 0.000000000000000000 ) ) ;
#16461=ORIENTED_EDGE ( 'NONE', *, *, #16013, .T. ) ;
#16465=AXIS2_PLACEMENT_3D ( 'NONE', #17392, #28809, #3133 ) ;
#16466=EDGE_CURVE ( 'NONE', #15620, #24169, #35899, .T. ) ;
#16467=CIRCLE ( 'NONE', #18881, 2.000000000000001776 ) ;
#16468=ORIENTED_EDGE ( 'NONE', *, *, #2909, .F. ) ;
#16469=ORIENTED_EDGE ( 'NONE', *, *, #32388, .T. ) ;
#16470=ADVANCED_FACE ( 'NONE', ( #27443 ), #21451, .F. ) ;
#16471=DIRECTION ( 'NONE',  ( -1.000000000000000000, 0.000000000000000000, 0.000000000000000000 ) ) ;
#16472=EDGE_LOOP ( 'NONE', ( #35045, #27522, #22436, #35487 ) ) ;
#16475=DIRECTION ( 'NONE',  ( 0.8660254037844344888, -0.5000000000000071054, 0.000000000000000000 ) ) ;
#16477=DIRECTION ( 'NONE',  ( 1.000000000000000000, 0.000000000000000000, 0.000000000000000000 ) ) ;
#16479=DIRECTION ( 'NONE',  ( 0.000000000000000000, 0.000000000000000000, 1.000000000000000000 ) ) ;
#16482=FACE_OUTER_BOUND ( 'NONE', #21310, .T. ) ;
#16483=AXIS2_PLACEMENT_3D ( 'NONE', #20185, #290, #8562 ) ;
#16484=ORIENTED_EDGE ( 'NONE', *, *, #19233, .F. ) ;
#16485=AXIS2_PLACEMENT_3D ( 'NONE', #708, #9532, #18142 ) ;
#16486=ORIENTED_EDGE ( 'NONE', *, *, #25811, .F. ) ;
#16488=EDGE_CURVE ( 'NONE', #29904, #2589, #7567, .T. ) ;
#16489=CARTESIAN_POINT ( 'NONE',  ( -10.00000337463125000, -86.60254037844400443, -5.000000000000000000 ) ) ;
#16490=CARTESIAN_POINT ( 'NONE',  ( 72.99999662536835388, -25.98076211353319565, 17.49999999999999645 ) ) ;
#16491=DIRECTION ( 'NONE',  ( -1.000000000000000000, 0.000000000000000000, 0.000000000000000000 ) ) ;
#16492=EDGE_LOOP ( 'NONE', ( #31789, #34932, #25704, #29024 ) ) ;
#16493=AXIS2_PLACEMENT_3D ( 'NONE', #3497, #32154, #32356 ) ;
#16495=AXIS2_PLACEMENT_3D ( 'NONE', #18882, #10820, #30311 ) ;
#16496=DIRECTION ( 'NONE',  ( 0.000000000000000000, 0.000000000000000000, 1.000000000000000000 ) ) ;
#16497=ORIENTED_EDGE ( 'NONE', *, *, #28086, .T. ) ;
#16499=DIRECTION ( 'NONE',  ( -0.000000000000000000, -0.000000000000000000, 1.000000000000000000 ) ) ;
#16500=ORIENTED_EDGE ( 'NONE', *, *, #30719, .F. ) ;
#16501=FACE_OUTER_BOUND ( 'NONE', #9097, .T. ) ;
#16502=DIRECTION ( 'NONE',  ( -1.000000000000000000, 0.000000000000000000, -0.000000000000000000 ) ) ;
#16503=EDGE_CURVE ( 'NONE', #21657, #20554, #17274, .T. ) ;
#16504=AXIS2_PLACEMENT_3D ( 'NONE', #3069, #23107, #58 ) ;
#16506=ORIENTED_EDGE ( 'NONE', *, *, #19097, .T. ) ;
#16508=CIRCLE ( 'NONE', #2131, 2.000000000000001776 ) ;
#16509=VERTEX_POINT ( 'NONE', #11477 ) ;
#16510=CIRCLE ( 'NONE', #3334, 2.000000000000001776 ) ;
#16512=EDGE_LOOP ( 'NONE', ( #28506, #19702 ) ) ;
#16513=AXIS2_PLACEMENT_3D ( 'NONE', #30275, #36656, #13589 ) ;
#16514=ADVANCED_FACE ( 'NONE', ( #19564 ), #6051, .F. ) ;
#16515=AXIS2_PLACEMENT_3D ( 'NONE', #29347, #32346, #476 ) ;
#16516=ORIENTED_EDGE ( 'NONE', *, *, #1865, .T. ) ;
#16517=CARTESIAN_POINT ( 'NONE',  ( -20.00000337463123756, -86.60254037844400443, -9.999999999999998224 ) ) ;
#16519=EDGE_CURVE ( 'NONE', #35595, #34395, #34650, .T. ) ;
#16520=CARTESIAN_POINT ( 'NONE',  ( 0.000000000000000000, 0.000000000000000000, 17.49999999999999645 ) ) ;
#16523=EDGE_CURVE ( 'NONE', #16356, #20554, #32846, .T. ) ;
#16524=ORIENTED_EDGE ( 'NONE', *, *, #11577, .F. ) ;
#16525=DIRECTION ( 'NONE',  ( 0.000000000000000000, 0.000000000000000000, -1.000000000000000000 ) ) ;
#16526=CIRCLE ( 'NONE', #14133, 2.000000000000001776 ) ;
#16528=ORIENTED_EDGE ( 'NONE', *, *, #4995, .T. ) ;
#16529=DIRECTION ( 'NONE',  ( 0.000000000000000000, 0.000000000000000000, 1.000000000000000000 ) ) ;
#16530=DIRECTION ( 'NONE',  ( 0.000000000000000000, 0.000000000000000000, -1.000000000000000000 ) ) ;
#16531=EDGE_CURVE ( 'NONE', #2942, #15689, #34198, .T. ) ;
#16537=EDGE_CURVE ( 'NONE', #13513, #3470, #18482, .T. ) ;
#16543=EDGE_CURVE ( 'NONE', #2363, #17289, #31053, .T. ) ;
#16545=VERTEX_POINT ( 'NONE', #37000 ) ;
#16548=AXIS2_PLACEMENT_3D ( 'NONE', #12295, #32188, #35413 ) ;
#16549=VECTOR ( 'NONE', #18841, 1000.000000000000000 ) ;
#16550=FACE_BOUND ( 'NONE', #12545, .T. ) ;
#16551=CIRCLE ( 'NONE', #30905, 1.999999999999998224 ) ;
#16552=ORIENTED_EDGE ( 'NONE', *, *, #9288, .T. ) ;
#16554=ORIENTED_EDGE ( 'NONE', *, *, #34984, .F. ) ;
#16555=VERTEX_POINT ( 'NONE', #31718 ) ;
#16556=AXIS2_PLACEMENT_3D ( 'NONE', #12426, #29483, #3805 ) ;
#16557=DIRECTION ( 'NONE',  ( 0.000000000000000000, 0.000000000000000000, 1.000000000000000000 ) ) ;
#16558=DIRECTION ( 'NONE',  ( 1.000000000000000000, 0.000000000000000000, 0.000000000000000000 ) ) ;
#16560=ORIENTED_EDGE ( 'NONE', *, *, #24863, .T. ) ;
#16562=DIRECTION ( 'NONE',  ( -1.000000000000000000, 0.000000000000000000, 0.000000000000000000 ) ) ;
#16563=AXIS2_PLACEMENT_3D ( 'NONE', #217, #28897, #6410 ) ;
#16564=DIRECTION ( 'NONE',  ( 0.000000000000000000, 0.000000000000000000, 1.000000000000000000 ) ) ;
#16565=CARTESIAN_POINT ( 'NONE',  ( -68.00000337463099243, 51.96152422706637708, 12.50000000000000000 ) ) ;
#16566=ORIENTED_EDGE ( 'NONE', *, *, #3746, .T. ) ;
#16567=DIRECTION ( 'NONE',  ( 1.000000000000000000, 0.000000000000000000, 0.000000000000000000 ) ) ;
#16568=FACE_BOUND ( 'NONE', #30084, .T. ) ;
#16570=DIRECTION ( 'NONE',  ( 0.000000000000000000, 0.000000000000000000, 1.000000000000000000 ) ) ;
#16571=CARTESIAN_POINT ( 'NONE',  ( 77.99999662536833966, 34.64101615137759183, -9.999999999999998224 ) ) ;
#16572=AXIS2_PLACEMENT_3D ( 'NONE', #32889, #15813, #6811 ) ;
#16573=DIRECTION ( 'NONE',  ( 0.000000000000000000, 0.000000000000000000, -1.000000000000000000 ) ) ;
#16574=CARTESIAN_POINT ( 'NONE',  ( -22.00000337463124112, -86.60254037844400443, 17.49999999999999645 ) ) ;
#16575=VECTOR ( 'NONE', #11076, 1000.000000000000000 ) ;
#16576=DIRECTION ( 'NONE',  ( 1.000000000000000000, 0.000000000000000000, 0.000000000000000000 ) ) ;
#16577=LINE ( 'NONE', #28012, #27731 ) ;
#16579=PLANE ( 'NONE',  #29768 ) ;
#16582=ORIENTED_EDGE ( 'NONE', *, *, #21533, .F. ) ;
#16583=CIRCLE ( 'NONE', #20764, 2.000000000000001776 ) ;
#16584=EDGE_CURVE ( 'NONE', #21660, #14230, #14883, .T. ) ;
#16585=ORIENTED_EDGE ( 'NONE', *, *, #7390, .F. ) ;
#16586=ORIENTED_EDGE ( 'NONE', *, *, #3033, .F. ) ;
#16587=EDGE_CURVE ( 'NONE', #27152, #11435, #2322, .T. ) ;
#16588=DIRECTION ( 'NONE',  ( 1.000000000000000000, 0.000000000000000000, 0.000000000000000000 ) ) ;
#16589=FACE_OUTER_BOUND ( 'NONE', #21430, .T. ) ;
#16590=ORIENTED_EDGE ( 'NONE', *, *, #22016, .T. ) ;
#16591=AXIS2_PLACEMENT_3D ( 'NONE', #16517, #28495, #28141 ) ;
#16592=CARTESIAN_POINT ( 'NONE',  ( -30.00000337463118427, 69.28203230275516944, -5.000000000000000000 ) ) ;
#16593=AXIS2_PLACEMENT_3D ( 'NONE', #31684, #3184, #26055 ) ;
#16594=CYLINDRICAL_SURFACE ( 'NONE', #11124, 2.000000000000001776 ) ;
#16595=VERTEX_POINT ( 'NONE', #14104 ) ;
#16598=ORIENTED_EDGE ( 'NONE', *, *, #16201, .F. ) ;
#16599=DIRECTION ( 'NONE',  ( 1.000000000000000000, 0.000000000000000000, 0.000000000000000000 ) ) ;
#16601=AXIS2_PLACEMENT_3D ( 'NONE', #2618, #36941, #11248 ) ;
#16602=VECTOR ( 'NONE', #22371, 1000.000000000000000 ) ;
#16604=CARTESIAN_POINT ( 'NONE',  ( 77.99999662536833966, 34.64101615137759183, -9.999999999999998224 ) ) ;
#16605=ORIENTED_EDGE ( 'NONE', *, *, #21623, .T. ) ;
#16606=DIRECTION ( 'NONE',  ( -1.000000000000000000, 0.000000000000000000, 0.000000000000000000 ) ) ;
#16608=ADVANCED_FACE ( 'NONE', ( #13753 ), #2877, .F. ) ;
#16610=CARTESIAN_POINT ( 'NONE',  ( 10.21421739743242618, 84.61404610869705323, 12.50000000000000000 ) ) ;
#16611=EDGE_LOOP ( 'NONE', ( #22099, #51 ) ) ;
#16612=DIRECTION ( 'NONE',  ( -1.000000000000000000, 0.000000000000000000, 0.000000000000000000 ) ) ;
#16614=EDGE_LOOP ( 'NONE', ( #8565, #37049 ) ) ;
#16615=CARTESIAN_POINT ( 'NONE',  ( -57.00000337463111322, -43.30127018922202353, 12.50000000000000000 ) ) ;
#16616=AXIS2_PLACEMENT_3D ( 'NONE', #11845, #23479, #26299 ) ;
#16617=CARTESIAN_POINT ( 'NONE',  ( -5.000003374631269537, -77.94228634059960825, 12.50000000000000000 ) ) ;
#16618=FACE_OUTER_BOUND ( 'NONE', #15207, .T. ) ;
#16619=DIRECTION ( 'NONE',  ( 0.000000000000000000, 0.000000000000000000, 1.000000000000000000 ) ) ;
#16620=AXIS2_PLACEMENT_3D ( 'NONE', #10286, #768, #7667 ) ;
#16621=ADVANCED_FACE ( 'NONE', ( #25204 ), #36631, .F. ) ;
#16623=CIRCLE ( 'NONE', #438, 2.000000000000001776 ) ;
#16626=CARTESIAN_POINT ( 'NONE',  ( 1.999996625368710257, -69.28203230275519786, -9.999999999999998224 ) ) ;
#16627=MECHANICAL_DESIGN_GEOMETRIC_PRESENTATION_REPRESENTATION('',(#3949),#8749);
#16628=AXIS2_PLACEMENT_3D ( 'NONE', #25298, #8041, #30724 ) ;
#16630=CIRCLE ( 'NONE', #11811, 2.000000000000001776 ) ;
#16631=ORIENTED_EDGE ( 'NONE', *, *, #8225, .T. ) ;
#16632=VERTEX_POINT ( 'NONE', #11644 ) ;
#16634=FACE_OUTER_BOUND ( 'NONE', #36654, .T. ) ;
#16636=CARTESIAN_POINT ( 'NONE',  ( 86.99999662536831124, -8.660254037844397956, -9.999999999999998224 ) ) ;
#16637=VECTOR ( 'NONE', #23355, 1000.000000000000000 ) ;
#16638=EDGE_LOOP ( 'NONE', ( #17383, #23411 ) ) ;
#16639=ORIENTED_EDGE ( 'NONE', *, *, #22546, .T. ) ;
#16640=CARTESIAN_POINT ( 'NONE',  ( 47.63139720814400846, -27.50000000000022737, -10.00000000000000178 ) ) ;
#16641=DIRECTION ( 'NONE',  ( 1.000000000000000000, 0.000000000000000000, 0.000000000000000000 ) ) ;
#16643=DIRECTION ( 'NONE',  ( 0.000000000000000000, 0.000000000000000000, 1.000000000000000000 ) ) ;
#16644=ORIENTED_EDGE ( 'NONE', *, *, #16488, .F. ) ;
#16645=AXIS2_PLACEMENT_3D ( 'NONE', #23733, #29521, #15841 ) ;
#16646=FACE_BOUND ( 'NONE', #22208, .T. ) ;
#16647=AXIS2_PLACEMENT_3D ( 'NONE', #8579, #14398, #11398 ) ;
#16648=VECTOR ( 'NONE', #23873, 1000.000000000000000 ) ;
#16650=EDGE_CURVE ( 'NONE', #21235, #25006, #25757, .T. ) ;
#16652=EDGE_LOOP ( 'NONE', ( #21887, #15335, #16506, #14293 ) ) ;
#16653=ADVANCED_FACE ( 'NONE', ( #36800 ), #12016, .F. ) ;
#16655=CARTESIAN_POINT ( 'NONE',  ( 89.42901512340354486, -31.83425564451495404, -49.86348611802629449 ) ) ;
#16656=VECTOR ( 'NONE', #4698, 1000.000000000000000 ) ;
#16657=DIRECTION ( 'NONE',  ( 1.000000000000000000, 0.000000000000000000, 0.000000000000000000 ) ) ;
#16658=DIRECTION ( 'NONE',  ( 0.000000000000000000, 0.000000000000000000, -1.000000000000000000 ) ) ;
#16659=ORIENTED_EDGE ( 'NONE', *, *, #11063, .F. ) ;
#16660=FACE_OUTER_BOUND ( 'NONE', #7123, .T. ) ;
#16661=EDGE_CURVE ( 'NONE', #8789, #24647, #20289, .T. ) ;
#16662=CARTESIAN_POINT ( 'NONE',  ( 69.99999662536839651, 17.32050807568879236, -5.000000000000000000 ) ) ;
#16663=CIRCLE ( 'NONE', #4108, 33.00000000000002132 ) ;
#16665=ORIENTED_EDGE ( 'NONE', *, *, #1629, .F. ) ;
#16666=EDGE_CURVE ( 'NONE', #5840, #14472, #769, .T. ) ;
#16667=ORIENTED_EDGE ( 'NONE', *, *, #22975, .F. ) ;
#16669=DIRECTION ( 'NONE',  ( 1.000000000000000000, 0.000000000000000000, 0.000000000000000000 ) ) ;
#16671=AXIS2_PLACEMENT_3D ( 'NONE', #15284, #17925, #18668 ) ;
#16672=CIRCLE ( 'NONE', #36434, 2.000000000000001776 ) ;
#16673=DIRECTION ( 'NONE',  ( -1.000000000000000000, 0.000000000000000000, 0.000000000000000000 ) ) ;
#16674=CARTESIAN_POINT ( 'NONE',  ( -72.00000337463102085, -34.64101615137762025, -9.999999999999998224 ) ) ;
#16675=CIRCLE ( 'NONE', #25584, 2.000000000000001776 ) ;
#16676=DIRECTION ( 'NONE',  ( 1.000000000000000000, 0.000000000000000000, 0.000000000000000000 ) ) ;
#16677=AXIS2_PLACEMENT_3D ( 'NONE', #18006, #15184, #370 ) ;
#16678=DIRECTION ( 'NONE',  ( 1.000000000000000000, 0.000000000000000000, 0.000000000000000000 ) ) ;
#16679=EDGE_CURVE ( 'NONE', #23931, #17038, #9602, .T. ) ;
#16680=CARTESIAN_POINT ( 'NONE',  ( -55.00000337463110611, -43.30127018922202353, -9.999999999999998224 ) ) ;
#16681=DIRECTION ( 'NONE',  ( 0.000000000000000000, 0.000000000000000000, 1.000000000000000000 ) ) ;
#16683=DIRECTION ( 'NONE',  ( 0.000000000000000000, 0.000000000000000000, 1.000000000000000000 ) ) ;
#16684=VECTOR ( 'NONE', #24020, 1000.000000000000000 ) ;
#16685=VERTEX_POINT ( 'NONE', #33153 ) ;
#16686=VERTEX_POINT ( 'NONE', #18030 ) ;
#16687=AXIS2_PLACEMENT_3D ( 'NONE', #34959, #31924, #3469 ) ;
#16689=CARTESIAN_POINT ( 'NONE',  ( 64.99999662536841072, 25.98076211353318854, -9.999999999999998224 ) ) ;
#16690=DIRECTION ( 'NONE',  ( 0.000000000000000000, 0.000000000000000000, 1.000000000000000000 ) ) ;
#16691=DIRECTION ( 'NONE',  ( 0.000000000000000000, 0.000000000000000000, 1.000000000000000000 ) ) ;
#16692=DIRECTION ( 'NONE',  ( 1.000000000000000000, 0.000000000000000000, 0.000000000000000000 ) ) ;
#16693=ORIENTED_EDGE ( 'NONE', *, *, #33157, .F. ) ;
#16695=CIRCLE ( 'NONE', #10108, 1.999999999999998224 ) ;
#16696=EDGE_CURVE ( 'NONE', #25889, #7714, #16713, .T. ) ;
#16697=DIRECTION ( 'NONE',  ( 1.000000000000000000, 0.000000000000000000, 0.000000000000000000 ) ) ;
#16699=ORIENTED_EDGE ( 'NONE', *, *, #30542, .F. ) ;
#16700=ORIENTED_EDGE ( 'NONE', *, *, #23918, .F. ) ;
#16701=ADVANCED_FACE ( 'NONE', ( #403 ), #9037, .F. ) ;
#16704=EDGE_LOOP ( 'NONE', ( #29144, #7735, #11979, #4148, #581, #27613 ) ) ;
#16705=DIRECTION ( 'NONE',  ( -1.000000000000000000, 0.000000000000000000, 0.000000000000000000 ) ) ;
#16707=CARTESIAN_POINT ( 'NONE',  ( 47.99999662536848177, -51.96152422706640550, -9.999999999999998224 ) ) ;
#16708=ORIENTED_EDGE ( 'NONE', *, *, #36365, .T. ) ;
#16709=ORIENTED_EDGE ( 'NONE', *, *, #14252, .F. ) ;
#16711=AXIS2_PLACEMENT_3D ( 'NONE', #14419, #28834, #11579 ) ;
#16712=ORIENTED_EDGE ( 'NONE', *, *, #12263, .T. ) ;
#16713=CIRCLE ( 'NONE', #23288, 2.000000000000001776 ) ;
#16714=ORIENTED_EDGE ( 'NONE', *, *, #6698, .F. ) ;
#16715=AXIS2_PLACEMENT_3D ( 'NONE', #35982, #24344, #35790 ) ;
#16717=ORIENTED_EDGE ( 'NONE', *, *, #7145, .F. ) ;
#16718=CARTESIAN_POINT ( 'NONE',  ( -45.00000337463112743, -60.62177826491080168, -9.999999999999998224 ) ) ;
#16719=CARTESIAN_POINT ( 'NONE',  ( 56.67878100130369035, -27.78182860042797131, -49.86348611802629449 ) ) ;
#16720=CARTESIAN_POINT ( 'NONE',  ( 35.19434990244975126, -52.39915983220758022, -4.999999999999997335 ) ) ;
#16725=CARTESIAN_POINT ( 'NONE',  ( -65.00000337463102085, 25.98076211353317433, 17.49999999999999645 ) ) ;
#16726=AXIS2_PLACEMENT_3D ( 'NONE', #21543, #15726, #13101 ) ;
#16727=DIRECTION ( 'NONE',  ( 0.000000000000000000, 0.000000000000000000, -1.000000000000000000 ) ) ;
#16728=ORIENTED_EDGE ( 'NONE', *, *, #27242, .T. ) ;
#16730=CIRCLE ( 'NONE', #14929, 33.00000000000001421 ) ;
#16731=DIRECTION ( 'NONE',  ( 1.000000000000000000, 0.000000000000000000, 0.000000000000000000 ) ) ;
#16734=ADVANCED_FACE ( 'NONE', ( #10287 ), #27347, .F. ) ;
#16735=CARTESIAN_POINT ( 'NONE',  ( 51.99999662536847467, -69.28203230275519786, 12.50000000000000000 ) ) ;
#16736=AXIS2_PLACEMENT_3D ( 'NONE', #3845, #33088, #13032 ) ;
#16740=ORIENTED_EDGE ( 'NONE', *, *, #11014, .T. ) ;
#16742=AXIS2_PLACEMENT_3D ( 'NONE', #17974, #9537, #29400 ) ;
#16743=EDGE_CURVE ( 'NONE', #5023, #14473, #2343, .T. ) ;
#16744=PLANE ( 'NONE',  #12276 ) ;
#16745=CIRCLE ( 'NONE', #20935, 2.000000000000001776 ) ;
#16746=VERTEX_POINT ( 'NONE', #9209 ) ;
#16747=EDGE_CURVE ( 'NONE', #8382, #9458, #28080, .T. ) ;
#16748=AXIS2_PLACEMENT_3D ( 'NONE', #34797, #26521, #29150 ) ;
#16749=EDGE_CURVE ( 'NONE', #17257, #27540, #13105, .T. ) ;
#16750=CARTESIAN_POINT ( 'NONE',  ( -4.279621169095561228, 62.97617850287782915, 12.49999999999999822 ) ) ;
#16752=CARTESIAN_POINT ( 'NONE',  ( -78.00000337463094979, -2.428612866367529932E-14, 17.49999999999999645 ) ) ;
#16754=CIRCLE ( 'NONE', #35922, 2.000000000000001776 ) ;
#16755=CARTESIAN_POINT ( 'NONE',  ( -13.89091430021420237, -62.33939050065180254, 12.49999999999999822 ) ) ;
#16756=ORIENTED_EDGE ( 'NONE', *, *, #24797, .T. ) ;
#16757=ORIENTED_EDGE ( 'NONE', *, *, #27532, .F. ) ;
#16758=CARTESIAN_POINT ( 'NONE',  ( -17.00000337463126243, 77.94228634059957983, 17.49999999999999645 ) ) ;
#16759=DIRECTION ( 'NONE',  ( 0.000000000000000000, 0.000000000000000000, 1.000000000000000000 ) ) ;
#16762=EDGE_CURVE ( 'NONE', #20325, #14036, #2760, .T. ) ;
#16764=DIRECTION ( 'NONE',  ( 0.000000000000000000, 0.000000000000000000, 1.000000000000000000 ) ) ;
#16765=FACE_BOUND ( 'NONE', #15062, .T. ) ;
#16766=DIRECTION ( 'NONE',  ( -1.000000000000000000, 0.000000000000000000, 0.000000000000000000 ) ) ;
#16767=CARTESIAN_POINT ( 'NONE',  ( 19.13981058454793072, -60.93295298010985306, 12.49999999999999822 ) ) ;
#16768=CARTESIAN_POINT ( 'NONE',  ( 69.99999662536838230, -34.64101615137759183, -9.999999999999998224 ) ) ;
#16769=AXIS2_PLACEMENT_3D ( 'NONE', #11506, #25231, #10791 ) ;
#16770=FACE_OUTER_BOUND ( 'NONE', #2436, .T. ) ;
#16771=CIRCLE ( 'NONE', #13146, 33.00000000000001421 ) ;
#16772=DIRECTION ( 'NONE',  ( 1.000000000000000000, 0.000000000000000000, 0.000000000000000000 ) ) ;
#16775=EDGE_LOOP ( 'NONE', ( #34575, #13610, #9221, #17604 ) ) ;
#16776=DIRECTION ( 'NONE',  ( 0.000000000000000000, 0.000000000000000000, -1.000000000000000000 ) ) ;
#16777=DIRECTION ( 'NONE',  ( 0.000000000000000000, 0.000000000000000000, 1.000000000000000000 ) ) ;
#16779=CYLINDRICAL_SURFACE ( 'NONE', #22788, 3.000000000000002665 ) ;
#16781=ORIENTED_EDGE ( 'NONE', *, *, #21087, .T. ) ;
#16782=EDGE_CURVE ( 'NONE', #16375, #35812, #356, .T. ) ;
#16783=EDGE_LOOP ( 'NONE', ( #34691, #10626, #8857, #20576 ) ) ;
#16785=CARTESIAN_POINT ( 'NONE',  ( 0.000000000000000000, 0.000000000000000000, -5.000000000000000000 ) ) ;
#16786=DIRECTION ( 'NONE',  ( 0.000000000000000000, 0.000000000000000000, 1.000000000000000000 ) ) ;
#16787=EDGE_CURVE ( 'NONE', #5093, #3514, #26708, .T. ) ;
#16788=ORIENTED_EDGE ( 'NONE', *, *, #33924, .F. ) ;
#16789=DIRECTION ( 'NONE',  ( 0.000000000000000000, 0.000000000000000000, -1.000000000000000000 ) ) ;
#16791=CIRCLE ( 'NONE', #1234, 27.00000000000001776 ) ;
#16793=ORIENTED_EDGE ( 'NONE', *, *, #20152, .T. ) ;
#16794=EDGE_CURVE ( 'NONE', #12265, #9206, #10547, .T. ) ;
#16795=CYLINDRICAL_SURFACE ( 'NONE', #23132, 1.999999999999998224 ) ;
#16796=AXIS2_PLACEMENT_3D ( 'NONE', #36390, #16496, #27929 ) ;
#16797=VERTEX_POINT ( 'NONE', #6767 ) ;
#16799=DIRECTION ( 'NONE',  ( -0.4999999999999977796, 0.8660254037844398178, 0.000000000000000000 ) ) ;
#16800=CIRCLE ( 'NONE', #28163, 33.00000000000001421 ) ;
#16801=ORIENTED_EDGE ( 'NONE', *, *, #24487, .T. ) ;
#16802=DIRECTION ( 'NONE',  ( 0.000000000000000000, 0.000000000000000000, 1.000000000000000000 ) ) ;
#16803=VECTOR ( 'NONE', #914, 1000.000000000000000 ) ;
#16804=EDGE_CURVE ( 'NONE', #31233, #31147, #9359, .T. ) ;
#16805=CARTESIAN_POINT ( 'NONE',  ( -27.00000337463121625, -77.94228634059963667, -9.999999999999998224 ) ) ;
#16807=FACE_OUTER_BOUND ( 'NONE', #20597, .T. ) ;
#16808=EDGE_CURVE ( 'NONE', #30244, #36248, #8169, .T. ) ;
#16812=EDGE_CURVE ( 'NONE', #36782, #5705, #36898, .T. ) ;
#16813=ORIENTED_EDGE ( 'NONE', *, *, #34196, .F. ) ;
#16814=DIRECTION ( 'NONE',  ( 1.000000000000000000, 0.000000000000000000, 0.000000000000000000 ) ) ;
#16817=CARTESIAN_POINT ( 'NONE',  ( 0.000000000000000000, 0.000000000000000000, -5.000000000000000000 ) ) ;
#16818=ORIENTED_EDGE ( 'NONE', *, *, #18603, .T. ) ;
#16819=ORIENTED_EDGE ( 'NONE', *, *, #24538, .F. ) ;
#16821=DIRECTION ( 'NONE',  ( -1.000000000000000000, 0.000000000000000000, 0.000000000000000000 ) ) ;
#16822=VERTEX_POINT ( 'NONE', #19292 ) ;
#16823=EDGE_LOOP ( 'NONE', ( #4565, #15329, #25873, #28252 ) ) ;
#16824=CIRCLE ( 'NONE', #1851, 3.000000000000002665 ) ;
#16827=DIRECTION ( 'NONE',  ( 0.000000000000000000, 0.000000000000000000, 1.000000000000000000 ) ) ;
#16829=EDGE_LOOP ( 'NONE', ( #19272, #33866, #18328, #994 ) ) ;
#16831=DIRECTION ( 'NONE',  ( 0.000000000000000000, 0.000000000000000000, -1.000000000000000000 ) ) ;
#16832=DIRECTION ( 'NONE',  ( 0.000000000000000000, 0.000000000000000000, 1.000000000000000000 ) ) ;
#16833=ORIENTED_EDGE ( 'NONE', *, *, #24311, .T. ) ;
#16835=ORIENTED_EDGE ( 'NONE', *, *, #36133, .F. ) ;
#16836=FACE_BOUND ( 'NONE', #25350, .T. ) ;
#16838=ORIENTED_EDGE ( 'NONE', *, *, #24022, .T. ) ;
#16840=DIRECTION ( 'NONE',  ( 1.000000000000000000, 0.000000000000000000, 0.000000000000000000 ) ) ;
#16841=CYLINDRICAL_SURFACE ( 'NONE', #19751, 2.000000000000001776 ) ;
#16842=CARTESIAN_POINT ( 'NONE',  ( -43.00000337463111322, 77.94228634059959404, -5.000000000000000000 ) ) ;
#16844=EDGE_CURVE ( 'NONE', #1473, #731, #3367, .T. ) ;
#16845=ORIENTED_EDGE ( 'NONE', *, *, #35016, .T. ) ;
#16846=DIRECTION ( 'NONE',  ( 0.000000000000000000, 0.000000000000000000, 1.000000000000000000 ) ) ;
#16847=DIRECTION ( 'NONE',  ( 1.000000000000000000, 0.000000000000000000, 0.000000000000000000 ) ) ;
#16849=ORIENTED_EDGE ( 'NONE', *, *, #4652, .T. ) ;
#16850=ORIENTED_EDGE ( 'NONE', *, *, #35016, .F. ) ;
#16852=DIRECTION ( 'NONE',  ( 1.000000000000000000, 0.000000000000000000, 0.000000000000000000 ) ) ;
#16853=CARTESIAN_POINT ( 'NONE',  ( 29.99999662536857770, -69.28203230275519786, -9.999999999999998224 ) ) ;
#16854=CARTESIAN_POINT ( 'NONE',  ( -7.000003374631307729, 77.94228634059957983, -5.000000000000000000 ) ) ;
#16856=CARTESIAN_POINT ( 'NONE',  ( 49.99999662536846756, 51.96152422706637708, 17.49999999999999645 ) ) ;
#16859=DIRECTION ( 'NONE',  ( 0.000000000000000000, 0.000000000000000000, 1.000000000000000000 ) ) ;
#16860=EDGE_CURVE ( 'NONE', #16037, #21975, #1577, .T. ) ;
#16865=LINE ( 'NONE', #25484, #7979 ) ;
#16866=CARTESIAN_POINT ( 'NONE',  ( -37.00000337463116296, 60.62177826491077326, -9.999999999999998224 ) ) ;
#16869=ORIENTED_EDGE ( 'NONE', *, *, #23524, .F. ) ;
#16871=FACE_BOUND ( 'NONE', #7259, .T. ) ;
#16873=ORIENTED_EDGE ( 'NONE', *, *, #27653, .F. ) ;
#16876=EDGE_LOOP ( 'NONE', ( #31669, #17957, #6870, #26004 ) ) ;
#16879=VECTOR ( 'NONE', #2498, 1000.000000000000000 ) ;
#16880=CARTESIAN_POINT ( 'NONE',  ( -25.00000337463120914, 77.94228634059957983, -5.000000000000000000 ) ) ;
#16881=EDGE_CURVE ( 'NONE', #28072, #13035, #12310, .T. ) ;
#16883=ORIENTED_EDGE ( 'NONE', *, *, #11358, .T. ) ;
#16886=EDGE_LOOP ( 'NONE', ( #6798, #14867, #36777, #24190, #16700 ) ) ;
#16888=CYLINDRICAL_SURFACE ( 'NONE', #34733, 2.000000000000000000 ) ;
#16889=LINE ( 'NONE', #27951, #5277 ) ;
#16890=CARTESIAN_POINT ( 'NONE',  ( 4.999996625368645198, 77.94228634059957983, 12.50000000000000000 ) ) ;
#16891=CARTESIAN_POINT ( 'NONE',  ( -83.45172111230354517, 31.46585318596159553, 12.49999999999999822 ) ) ;
#16893=CARTESIAN_POINT ( 'NONE',  ( 67.99999662536836809, -34.64101615137759183, -5.000000000000000000 ) ) ;
#16895=ADVANCED_FACE ( 'NONE', ( #2587 ), #13279, .F. ) ;
#16896=CARTESIAN_POINT ( 'NONE',  ( 79.99999662536833966, 34.64101615137759183, 12.50000000000000000 ) ) ;
#16897=ORIENTED_EDGE ( 'NONE', *, *, #25192, .F. ) ;
#16898=DIRECTION ( 'NONE',  ( 1.000000000000000000, 0.000000000000000000, 0.000000000000000000 ) ) ;
#16899=CARTESIAN_POINT ( 'NONE',  ( 57.99999662536842493, -51.96152422706639840, 17.49999999999999645 ) ) ;
#16900=ORIENTED_EDGE ( 'NONE', *, *, #35489, .F. ) ;
#16901=ORIENTED_EDGE ( 'NONE', *, *, #3531, .F. ) ;
#16902=DIRECTION ( 'NONE',  ( 0.000000000000000000, 0.000000000000000000, 1.000000000000000000 ) ) ;
#16903=CIRCLE ( 'NONE', #35471, 2.000000000000000000 ) ;
#16907=EDGE_CURVE ( 'NONE', #32711, #32590, #36550, .T. ) ;
#16909=VERTEX_POINT ( 'NONE', #8025 ) ;
#16910=CARTESIAN_POINT ( 'NONE',  ( 64.99999662536839651, -43.30127018922199511, -9.999999999999998224 ) ) ;
#16911=EDGE_CURVE ( 'NONE', #12612, #22847, #17739, .T. ) ;
#16912=VERTEX_POINT ( 'NONE', #30709 ) ;
#16913=CARTESIAN_POINT ( 'NONE',  ( 0.000000000000000000, 0.000000000000000000, -5.000000000000000000 ) ) ;
#16914=ORIENTED_EDGE ( 'NONE', *, *, #13544, .T. ) ;
#16915=ORIENTED_EDGE ( 'NONE', *, *, #23625, .F. ) ;
#16917=CARTESIAN_POINT ( 'NONE',  ( 31.99999662536856704, 69.28203230275518365, -9.999999999999998224 ) ) ;
#16919=VERTEX_POINT ( 'NONE', #22110 ) ;
#16921=DIRECTION ( 'NONE',  ( 0.000000000000000000, 0.000000000000000000, 1.000000000000000000 ) ) ;
#16922=CYLINDRICAL_SURFACE ( 'NONE', #11151, 2.000000000000001776 ) ;
#16923=CARTESIAN_POINT ( 'NONE',  ( -83.00000337463092137, 8.660254037844389075, -5.000000000000000000 ) ) ;
#16924=DIRECTION ( 'NONE',  ( 0.000000000000000000, 0.000000000000000000, 1.000000000000000000 ) ) ;
#16925=ADVANCED_FACE ( 'NONE', ( #2221 ), #13660, .F. ) ;
#16927=DIRECTION ( 'NONE',  ( 1.000000000000000000, 0.000000000000000000, 0.000000000000000000 ) ) ;
#16928=AXIS2_PLACEMENT_3D ( 'NONE', #11604, #8082, #22712 ) ;
#16929=FACE_BOUND ( 'NONE', #33719, .T. ) ;
#16932=CARTESIAN_POINT ( 'NONE',  ( -73.00000337463097821, 43.30127018922197379, -9.999999999999998224 ) ) ;
#16933=DIRECTION ( 'NONE',  ( 0.000000000000000000, 0.000000000000000000, -1.000000000000000000 ) ) ;
#16934=CARTESIAN_POINT ( 'NONE',  ( 0.000000000000000000, 0.000000000000000000, -5.000000000000000000 ) ) ;
#16935=EDGE_CURVE ( 'NONE', #20017, #10138, #25286, .T. ) ;
#16938=EDGE_CURVE ( 'NONE', #13323, #24795, #17135, .T. ) ;
#16940=VERTEX_POINT ( 'NONE', #5774 ) ;
#16941=CARTESIAN_POINT ( 'NONE',  ( -58.00000337463104216, 34.64101615137757051, 17.49999999999999645 ) ) ;
#16942=CARTESIAN_POINT ( 'NONE',  ( -45.00000337463111322, -77.94228634059960825, -9.999999999999998224 ) ) ;
#16943=DIRECTION ( 'NONE',  ( 0.000000000000000000, 0.000000000000000000, 1.000000000000000000 ) ) ;
#16944=ORIENTED_EDGE ( 'NONE', *, *, #4288, .F. ) ;
#16945=CIRCLE ( 'NONE', #21731, 2.000000000000001776 ) ;
#16946=ORIENTED_EDGE ( 'NONE', *, *, #19640, .F. ) ;
#16949=DIRECTION ( 'NONE',  ( 0.000000000000000000, 0.000000000000000000, 1.000000000000000000 ) ) ;
#16952=EDGE_CURVE ( 'NONE', #3252, #1861, #31483, .T. ) ;
#16953=AXIS2_PLACEMENT_3D ( 'NONE', #36556, #22288, #16852 ) ;
#16954=ORIENTED_EDGE ( 'NONE', *, *, #11490, .F. ) ;
#16955=PLANE ( 'NONE',  #36551 ) ;
#16956=ORIENTED_EDGE ( 'NONE', *, *, #26871, .T. ) ;
#16957=DIRECTION ( 'NONE',  ( 0.000000000000000000, 0.000000000000000000, -1.000000000000000000 ) ) ;
#16959=ORIENTED_EDGE ( 'NONE', *, *, #5405, .F. ) ;
#16960=DIRECTION ( 'NONE',  ( 1.000000000000000000, 0.000000000000000000, 0.000000000000000000 ) ) ;
#16961=CARTESIAN_POINT ( 'NONE',  ( -43.00000337463111322, 60.62177826491077326, 17.49999999999999645 ) ) ;
#16962=VERTEX_POINT ( 'NONE', #31262 ) ;
#16963=CARTESIAN_POINT ( 'NONE',  ( 66.99999662536842493, 43.30127018922200222, -9.999999999999998224 ) ) ;
#16964=AXIS2_PLACEMENT_3D ( 'NONE', #1185, #29473, #7186 ) ;
#16965=DIRECTION ( 'NONE',  ( 0.000000000000000000, 0.000000000000000000, -1.000000000000000000 ) ) ;
#16967=AXIS2_PLACEMENT_3D ( 'NONE', #10691, #33931, #5602 ) ;
#16969=ORIENTED_EDGE ( 'NONE', *, *, #22316, .T. ) ;
#16970=CARTESIAN_POINT ( 'NONE',  ( -30.89873480577614018, 67.49533652152319974, 12.50000000000000000 ) ) ;
#16971=FACE_OUTER_BOUND ( 'NONE', #21787, .T. ) ;
#16972=VERTEX_POINT ( 'NONE', #20206 ) ;
#16973=EDGE_CURVE ( 'NONE', #14843, #8516, #19548, .T. ) ;
#16974=DIRECTION ( 'NONE',  ( 1.000000000000000000, 0.000000000000000000, 0.000000000000000000 ) ) ;
#16975=CARTESIAN_POINT ( 'NONE',  ( 29.99999662536856349, 69.28203230275518365, 17.49999999999999645 ) ) ;
#16976=CARTESIAN_POINT ( 'NONE',  ( 57.99999662536843914, -34.64101615137759893, -9.999999999999998224 ) ) ;
#16977=DIRECTION ( 'NONE',  ( -1.000000000000000000, 0.000000000000000000, -0.000000000000000000 ) ) ;
#16978=AXIS2_PLACEMENT_3D ( 'NONE', #7618, #25239, #21675 ) ;
#16979=EDGE_CURVE ( 'NONE', #5117, #3388, #36909, .T. ) ;
#16980=EDGE_LOOP ( 'NONE', ( #22547, #23983 ) ) ;
#16981=CIRCLE ( 'NONE', #21150, 2.000000000000001776 ) ;
#16982=ORIENTED_EDGE ( 'NONE', *, *, #29260, .F. ) ;
#16983=EDGE_CURVE ( 'NONE', #19499, #1659, #15331, .T. ) ;
#16985=LINE ( 'NONE', #11715, #20551 ) ;
#16986=EDGE_CURVE ( 'NONE', #34280, #35776, #29696, .T. ) ;
#16987=AXIS2_PLACEMENT_3D ( 'NONE', #6281, #279, #8728 ) ;
#16988=ORIENTED_EDGE ( 'NONE', *, *, #35013, .F. ) ;
#16990=DIRECTION ( 'NONE',  ( 1.000000000000000000, 0.000000000000000000, 0.000000000000000000 ) ) ;
#16991=DIRECTION ( 'NONE',  ( 0.5000000000000039968, 0.8660254037844363761, 0.000000000000000000 ) ) ;
#16992=DIRECTION ( 'NONE',  ( 0.000000000000000000, 0.000000000000000000, -1.000000000000000000 ) ) ;
#16993=EDGE_CURVE ( 'NONE', #31042, #15896, #8754, .T. ) ;
#16994=EDGE_LOOP ( 'NONE', ( #11877, #9863, #7580, #34577, #21829, #2458 ) ) ;
#16995=EDGE_CURVE ( 'NONE', #26437, #32411, #9330, .T. ) ;
#16996=ORIENTED_EDGE ( 'NONE', *, *, #28161, .T. ) ;
#16997=DIRECTION ( 'NONE',  ( 0.000000000000000000, 0.000000000000000000, 1.000000000000000000 ) ) ;
#16998=EDGE_CURVE ( 'NONE', #7037, #20745, #13536, .T. ) ;
#16999=FACE_OUTER_BOUND ( 'NONE', #26392, .T. ) ;
#17001=EDGE_CURVE ( 'NONE', #10417, #10952, #17562, .T. ) ;
#17002=CARTESIAN_POINT ( 'NONE',  ( -68.00000337463100664, -17.32050807568882078, -9.999999999999998224 ) ) ;
#17003=EDGE_LOOP ( 'NONE', ( #7052, #27609, #28620, #16959 ) ) ;
#17004=FACE_BOUND ( 'NONE', #16010, .T. ) ;
#17006=DIRECTION ( 'NONE',  ( 1.000000000000000000, 0.000000000000000000, 0.000000000000000000 ) ) ;
#17007=ORIENTED_EDGE ( 'NONE', *, *, #19735, .F. ) ;
#17009=CARTESIAN_POINT ( 'NONE',  ( -52.39915983220772233, -35.19434990244957362, 12.49999999999999822 ) ) ;
#17010=CARTESIAN_POINT ( 'NONE',  ( -63.00000337463102085, 43.30127018922198801, -5.000000000000000000 ) ) ;
#17011=CARTESIAN_POINT ( 'NONE',  ( 17.99999662536858125, 86.60254037844397601, 17.49999999999999645 ) ) ;
#17012=ORIENTED_EDGE ( 'NONE', *, *, #16013, .F. ) ;
#17013=DIRECTION ( 'NONE',  ( 0.000000000000000000, 0.000000000000000000, 1.000000000000000000 ) ) ;
#17014=CARTESIAN_POINT ( 'NONE',  ( -60.00000337463104216, 34.64101615137757051, -9.999999999999998224 ) ) ;
#17015=DIRECTION ( 'NONE',  ( 0.000000000000000000, 0.000000000000000000, -1.000000000000000000 ) ) ;
#17016=ORIENTED_EDGE ( 'NONE', *, *, #31052, .T. ) ;
#17017=CIRCLE ( 'NONE', #33182, 2.000000000000001776 ) ;
#17018=ORIENTED_EDGE ( 'NONE', *, *, #35131, .F. ) ;
#17019=ORIENTED_EDGE ( 'NONE', *, *, #28842, .F. ) ;
#17020=DIRECTION ( 'NONE',  ( -0.4999999999999980016, 0.8660254037844398178, 0.000000000000000000 ) ) ;
#17021=CIRCLE ( 'NONE', #28972, 2.000000000000000000 ) ;
#17024=DIRECTION ( 'NONE',  ( 0.000000000000000000, 0.000000000000000000, 1.000000000000000000 ) ) ;
#17027=CYLINDRICAL_SURFACE ( 'NONE', #5841, 2.000000000000001776 ) ;
#17028=CARTESIAN_POINT ( 'NONE',  ( 71.99999662536841072, 51.96152422706640550, -9.999999999999998224 ) ) ;
#17029=ORIENTED_EDGE ( 'NONE', *, *, #24793, .F. ) ;
#17030=ORIENTED_EDGE ( 'NONE', *, *, #15478, .T. ) ;
#17031=DIRECTION ( 'NONE',  ( 1.000000000000000000, 0.000000000000000000, 0.000000000000000000 ) ) ;
#17032=VECTOR ( 'NONE', #14813, 1000.000000000000000 ) ;
#17033=LINE ( 'NONE', #5051, #13940 ) ;
#17034=ADVANCED_FACE ( 'NONE', ( #26389 ), #37098, .F. ) ;
#17036=CIRCLE ( 'NONE', #9241, 33.00000000000002132 ) ;
#17037=DIRECTION ( 'NONE',  ( 0.000000000000000000, 0.000000000000000000, 1.000000000000000000 ) ) ;
#17038=VERTEX_POINT ( 'NONE', #17215 ) ;
#17039=UNCERTAINTY_MEASURE_WITH_UNIT (LENGTH_MEASURE( 1.000000000000000082E-05 ), #10504, 'distance_accuracy_value', 'NONE');
#17040=CIRCLE ( 'NONE', #36801, 2.000000000000001776 ) ;
#17042=FACE_BOUND ( 'NONE', #1796, .T. ) ;
#17044=ORIENTED_EDGE ( 'NONE', *, *, #13313, .F. ) ;
#17046=DIRECTION ( 'NONE',  ( 0.000000000000000000, 0.000000000000000000, 1.000000000000000000 ) ) ;
#17047=ORIENTED_EDGE ( 'NONE', *, *, #13908, .F. ) ;
#17048=DIRECTION ( 'NONE',  ( 0.000000000000000000, 0.000000000000000000, -1.000000000000000000 ) ) ;
#17049=CIRCLE ( 'NONE', #36810, 27.00000000000001776 ) ;
#17050=CIRCLE ( 'NONE', #22431, 1.999999999999998224 ) ;
#17051=VECTOR ( 'NONE', #11178, 1000.000000000000000 ) ;
#17052=DIRECTION ( 'NONE',  ( 0.000000000000000000, 0.000000000000000000, 1.000000000000000000 ) ) ;
#17053=AXIS2_PLACEMENT_3D ( 'NONE', #136, #11029, #11408 ) ;
#17055=ORIENTED_EDGE ( 'NONE', *, *, #23431, .T. ) ;
#17056=ORIENTED_EDGE ( 'NONE', *, *, #7680, .F. ) ;
#17057=VERTEX_POINT ( 'NONE', #25664 ) ;
#17058=EDGE_CURVE ( 'NONE', #33801, #31156, #5173, .T. ) ;
#17059=VERTEX_POINT ( 'NONE', #26203 ) ;
#17061=VECTOR ( 'NONE', #11930, 1000.000000000000000 ) ;
#17062=DIRECTION ( 'NONE',  ( -1.000000000000000000, 0.000000000000000000, 0.000000000000000000 ) ) ;
#17064=AXIS2_PLACEMENT_3D ( 'NONE', #24828, #7574, #21259 ) ;
#17068=VERTEX_POINT ( 'NONE', #31443 ) ;
#17069=CYLINDRICAL_SURFACE ( 'NONE', #15921, 3.000000000000006217 ) ;
#17071=CARTESIAN_POINT ( 'NONE',  ( 20.39230124433451152, -84.64139349818795210, -5.000000000000000000 ) ) ;
#17072=EDGE_CURVE ( 'NONE', #2028, #27460, #14568, .T. ) ;
#17073=CARTESIAN_POINT ( 'NONE',  ( 59.99999662536842493, 51.96152422706639129, -5.000000000000000000 ) ) ;
#17074=VERTEX_POINT ( 'NONE', #311 ) ;
#17075=FACE_OUTER_BOUND ( 'NONE', #16886, .T. ) ;
#17076=DIRECTION ( 'NONE',  ( 0.000000000000000000, 0.000000000000000000, 1.000000000000000000 ) ) ;
#17077=AXIS2_PLACEMENT_3D ( 'NONE', #123, #9301, #23202 ) ;
#17079=VECTOR ( 'NONE', #7374, 1000.000000000000000 ) ;
#17080=EDGE_LOOP ( 'NONE', ( #16659, #20498 ) ) ;
#17081=DIRECTION ( 'NONE',  ( 1.000000000000000000, 0.000000000000000000, 0.000000000000000000 ) ) ;
#17083=ADVANCED_FACE ( 'NONE', ( #11399 ), #11748, .F. ) ;
#17084=LINE ( 'NONE', #28164, #24162 ) ;
#17087=ORIENTED_EDGE ( 'NONE', *, *, #19421, .F. ) ;
#17088=EDGE_LOOP ( 'NONE', ( #12210, #4447 ) ) ;
#17091=CIRCLE ( 'NONE', #11666, 2.000000000000000000 ) ;
#17094=CARTESIAN_POINT ( 'NONE',  ( 0.000000000000000000, 0.000000000000000000, 12.49999999999999822 ) ) ;
#17095=EDGE_LOOP ( 'NONE', ( #78, #6172, #18232, #19301, #33941 ) ) ;
#17096=AXIS2_PLACEMENT_3D ( 'NONE', #33884, #22435, #30325 ) ;
#17097=DIRECTION ( 'NONE',  ( 0.000000000000000000, 0.000000000000000000, 1.000000000000000000 ) ) ;
#17100=FACE_OUTER_BOUND ( 'NONE', #32871, .T. ) ;
#17101=CIRCLE ( 'NONE', #928, 2.000000000000001776 ) ;
#17102=EDGE_CURVE ( 'NONE', #5705, #18862, #16551, .T. ) ;
#17103=CARTESIAN_POINT ( 'NONE',  ( 59.99999662536845335, 34.64101615137759893, -9.999999999999998224 ) ) ;
#17104=VERTEX_POINT ( 'NONE', #34830 ) ;
#17105=VERTEX_POINT ( 'NONE', #14958 ) ;
#17106=CARTESIAN_POINT ( 'NONE',  ( -33.00000337463116296, 60.62177826491077326, -9.999999999999998224 ) ) ;
#17107=CARTESIAN_POINT ( 'NONE',  ( -7.000003374631269537, -77.94228634059960825, -9.999999999999998224 ) ) ;
#17109=AXIS2_PLACEMENT_3D ( 'NONE', #22060, #2367, #7809 ) ;
#17110=CARTESIAN_POINT ( 'NONE',  ( -77.00000337463097821, 8.660254037844374864, -9.999999999999998224 ) ) ;
#17111=AXIS2_PLACEMENT_3D ( 'NONE', #10432, #13252, #21872 ) ;
#17113=ORIENTED_EDGE ( 'NONE', *, *, #3628, .F. ) ;
#17114=CARTESIAN_POINT ( 'NONE',  ( 51.99999662536848888, -51.96152422706640550, -9.999999999999998224 ) ) ;
#17115=FACE_BOUND ( 'NONE', #35345, .T. ) ;
#17116=EDGE_CURVE ( 'NONE', #9729, #5735, #988, .T. ) ;
#17118=PLANE ( 'NONE',  #30655 ) ;
#17122=EDGE_CURVE ( 'NONE', #20328, #9458, #35408, .T. ) ;
#17123=CIRCLE ( 'NONE', #35082, 2.000000000000001776 ) ;
#17125=ORIENTED_EDGE ( 'NONE', *, *, #26726, .T. ) ;
#17128=DIRECTION ( 'NONE',  ( -1.000000000000000000, 0.000000000000000000, 0.000000000000000000 ) ) ;
#17130=CIRCLE ( 'NONE', #954, 2.000000000000001776 ) ;
#17131=AXIS2_PLACEMENT_3D ( 'NONE', #18189, #27009, #29620 ) ;
#17132=AXIS2_PLACEMENT_3D ( 'NONE', #1237, #23938, #34989 ) ;
#17133=ORIENTED_EDGE ( 'NONE', *, *, #36124, .F. ) ;
#17134=ORIENTED_EDGE ( 'NONE', *, *, #13799, .F. ) ;
#17135=CIRCLE ( 'NONE', #32700, 95.00000000000000000 ) ;
#17136=ORIENTED_EDGE ( 'NONE', *, *, #2, .F. ) ;
#17137=DIRECTION ( 'NONE',  ( 0.000000000000000000, 0.000000000000000000, -1.000000000000000000 ) ) ;
#17139=FACE_OUTER_BOUND ( 'NONE', #25236, .T. ) ;
#17140=EDGE_LOOP ( 'NONE', ( #28596, #26441 ) ) ;
#17141=AXIS2_PLACEMENT_3D ( 'NONE', #28427, #13996, #117 ) ;
#17143=EDGE_CURVE ( 'NONE', #33988, #20247, #34535, .T. ) ;
#17145=FACE_OUTER_BOUND ( 'NONE', #23806, .T. ) ;
#17146=ORIENTED_EDGE ( 'NONE', *, *, #5044, .F. ) ;
#17147=CARTESIAN_POINT ( 'NONE',  ( -67.00000337463102085, 43.30127018922198801, -9.999999999999998224 ) ) ;
#17148=ORIENTED_EDGE ( 'NONE', *, *, #3107, .F. ) ;
#17149=AXIS2_PLACEMENT_3D ( 'NONE', #32501, #20695, #17901 ) ;
#17150=ORIENTED_EDGE ( 'NONE', *, *, #1588, .F. ) ;
#17151=EDGE_CURVE ( 'NONE', #30760, #859, #5788, .T. ) ;
#17154=AXIS2_PLACEMENT_3D ( 'NONE', #12759, #36215, #4534 ) ;
#17158=DIRECTION ( 'NONE',  ( 1.000000000000000000, 0.000000000000000000, 0.000000000000000000 ) ) ;
#17159=AXIS2_PLACEMENT_3D ( 'NONE', #989, #28756, #236 ) ;
#17160=AXIS2_PLACEMENT_3D ( 'NONE', #24642, #10371, #21804 ) ;
#17162=VECTOR ( 'NONE', #18591, 1000.000000000000000 ) ;
#17163=AXIS2_PLACEMENT_3D ( 'NONE', #33780, #2084, #22723 ) ;
#17165=DIRECTION ( 'NONE',  ( 0.000000000000000000, 0.000000000000000000, 1.000000000000000000 ) ) ;
#17166=AXIS2_PLACEMENT_3D ( 'NONE', #28049, #21864, #33310 ) ;
#17167=ORIENTED_EDGE ( 'NONE', *, *, #6046, .F. ) ;
#17169=CARTESIAN_POINT ( 'NONE',  ( -47.63139720814380951, 27.50000000000055422, -10.00000000000000000 ) ) ;
#17171=DIRECTION ( 'NONE',  ( 0.000000000000000000, 0.000000000000000000, 1.000000000000000000 ) ) ;
#17172=FACE_OUTER_BOUND ( 'NONE', #909, .T. ) ;
#17175=CIRCLE ( 'NONE', #3996, 2.000000000000001776 ) ;
#17176=ORIENTED_EDGE ( 'NONE', *, *, #33516, .T. ) ;
#17177=EDGE_CURVE ( 'NONE', #2812, #20017, #33334, .T. ) ;
#17178=ORIENTED_EDGE ( 'NONE', *, *, #6914, .F. ) ;
#17179=DIRECTION ( 'NONE',  ( -1.000000000000000000, 8.994862468027885935E-16, 0.000000000000000000 ) ) ;
#17180=DIRECTION ( 'NONE',  ( 0.8660254037844344888, -0.5000000000000071054, 0.000000000000000000 ) ) ;
#17182=ORIENTED_EDGE ( 'NONE', *, *, #13797, .F. ) ;
#17184=CIRCLE ( 'NONE', #25557, 27.00000000000001066 ) ;
#17185=CARTESIAN_POINT ( 'NONE',  ( -25.00000337463121980, -77.94228634059963667, 17.49999999999999645 ) ) ;
#17188=VECTOR ( 'NONE', #9375, 1000.000000000000000 ) ;
#17190=AXIS2_PLACEMENT_3D ( 'NONE', #26703, #18260, #23712 ) ;
#17191=EDGE_CURVE ( 'NONE', #23997, #10138, #3403, .T. ) ;
#17193=VERTEX_POINT ( 'NONE', #23958 ) ;
#17194=ADVANCED_FACE ( 'NONE', ( #1068 ), #26943, .F. ) ;
#17195=LINE ( 'NONE', #22265, #2365 ) ;
#17196=ORIENTED_EDGE ( 'NONE', *, *, #19474, .T. ) ;
#17197=DIRECTION ( 'NONE',  ( -1.000000000000000000, 0.000000000000000000, 0.000000000000000000 ) ) ;
#17198=AXIS2_PLACEMENT_3D ( 'NONE', #10747, #2307, #5486 ) ;
#17201=CARTESIAN_POINT ( 'NONE',  ( 34.99999662536855283, -77.94228634059960825, 12.50000000000000000 ) ) ;
#17202=EDGE_CURVE ( 'NONE', #12874, #12408, #7257, .T. ) ;
#17203=CIRCLE ( 'NONE', #26194, 2.000000000000001776 ) ;
#17204=ORIENTED_EDGE ( 'NONE', *, *, #23617, .T. ) ;
#17205=EDGE_CURVE ( 'NONE', #8894, #8910, #36337, .T. ) ;
#17207=AXIS2_PLACEMENT_3D ( 'NONE', #3565, #3180, #32019 ) ;
#17208=DIRECTION ( 'NONE',  ( 1.000000000000000000, 0.000000000000000000, 0.000000000000000000 ) ) ;
#17209=AXIS2_PLACEMENT_3D ( 'NONE', #18266, #1392, #35721 ) ;
#17213=DIRECTION ( 'NONE',  ( 1.000000000000000000, 0.000000000000000000, 0.000000000000000000 ) ) ;
#17214=DIRECTION ( 'NONE',  ( -1.000000000000000000, 0.000000000000000000, 0.000000000000000000 ) ) ;
#17215=CARTESIAN_POINT ( 'NONE',  ( 71.99999662536839651, -17.32050807568879947, 17.49999999999999645 ) ) ;
#17216=EDGE_CURVE ( 'NONE', #31694, #18695, #29737, .T. ) ;
#17217=AXIS2_PLACEMENT_3D ( 'NONE', #3643, #28768, #31917 ) ;
#17218=AXIS2_PLACEMENT_3D ( 'NONE', #28279, #13296, #19309 ) ;
#17220=ORIENTED_EDGE ( 'NONE', *, *, #22499, .T. ) ;
#17221=AXIS2_PLACEMENT_3D ( 'NONE', #34597, #6805, #35148 ) ;
#17222=EDGE_LOOP ( 'NONE', ( #30226, #8682 ) ) ;
#17223=EDGE_CURVE ( 'NONE', #30348, #4797, #3989, .T. ) ;
#17224=EDGE_LOOP ( 'NONE', ( #1347, #32037 ) ) ;
#17225=EDGE_CURVE ( 'NONE', #1819, #30350, #26738, .T. ) ;
#17226=AXIS2_PLACEMENT_3D ( 'NONE', #24307, #9695, #12673 ) ;
#17227=DIRECTION ( 'NONE',  ( 1.000000000000000000, 0.000000000000000000, 0.000000000000000000 ) ) ;
#17228=VECTOR ( 'NONE', #9058, 1000.000000000000000 ) ;
#17231=DIRECTION ( 'NONE',  ( 1.000000000000000000, 0.000000000000000000, 0.000000000000000000 ) ) ;
#17233=CIRCLE ( 'NONE', #4062, 27.00000000000001421 ) ;
#17236=AXIS2_PLACEMENT_3D ( 'NONE', #29080, #26291, #36356 ) ;
#17238=DIRECTION ( 'NONE',  ( 0.000000000000000000, 0.000000000000000000, 1.000000000000000000 ) ) ;
#17239=EDGE_CURVE ( 'NONE', #6061, #28630, #24363, .T. ) ;
#17240=CIRCLE ( 'NONE', #14816, 3.000000000000002665 ) ;
#17242=DIRECTION ( 'NONE',  ( 0.000000000000000000, 0.000000000000000000, -1.000000000000000000 ) ) ;
#17243=DIRECTION ( 'NONE',  ( 1.000000000000000000, 0.000000000000000000, 0.000000000000000000 ) ) ;
#17246=FACE_BOUND ( 'NONE', #33313, .T. ) ;
#17249=EDGE_CURVE ( 'NONE', #16094, #15689, #10577, .T. ) ;
#17250=DIRECTION ( 'NONE',  ( 0.000000000000000000, 0.000000000000000000, 1.000000000000000000 ) ) ;
#17251=ORIENTED_EDGE ( 'NONE', *, *, #8934, .F. ) ;
#17254=VECTOR ( 'NONE', #35095, 1000.000000000000000 ) ;
#17255=DIRECTION ( 'NONE',  ( 1.000000000000000000, 0.000000000000000000, 0.000000000000000000 ) ) ;
#17256=VERTEX_POINT ( 'NONE', #3698 ) ;
#17257=VERTEX_POINT ( 'NONE', #15125 ) ;
#17258=AXIS2_PLACEMENT_3D ( 'NONE', #20925, #32353, #6669 ) ;
#17262=EDGE_CURVE ( 'NONE', #18637, #14854, #8201, .T. ) ;
#17263=ORIENTED_EDGE ( 'NONE', *, *, #9736, .T. ) ;
#17264=ORIENTED_EDGE ( 'NONE', *, *, #23944, .T. ) ;
#17265=ADVANCED_FACE ( 'NONE', ( #5380 ), #24515, .F. ) ;
#17266=DIRECTION ( 'NONE',  ( 0.000000000000000000, 0.000000000000000000, 1.000000000000000000 ) ) ;
#17267=ADVANCED_FACE ( 'NONE', ( #16618 ), #36123, .F. ) ;
#17271=DIRECTION ( 'NONE',  ( 0.000000000000000000, 0.000000000000000000, 1.000000000000000000 ) ) ;
#17272=EDGE_LOOP ( 'NONE', ( #27034, #22411, #23313, #29879 ) ) ;
#17273=CARTESIAN_POINT ( 'NONE',  ( 66.99999662536839651, -43.30127018922199511, -9.999999999999998224 ) ) ;
#17274=CIRCLE ( 'NONE', #10689, 33.00000000000002132 ) ;
#17275=CARTESIAN_POINT ( 'NONE',  ( 86.99999662536832545, 25.98076211353319565, -9.999999999999998224 ) ) ;
#17277=EDGE_LOOP ( 'NONE', ( #6340, #18400 ) ) ;
#17278=LINE ( 'NONE', #20068, #26244 ) ;
#17279=CARTESIAN_POINT ( 'NONE',  ( -32.00000337463118427, 69.28203230275516944, 17.49999999999999645 ) ) ;
#17280=CIRCLE ( 'NONE', #33447, 2.000000000000000000 ) ;
#17281=ORIENTED_EDGE ( 'NONE', *, *, #26970, .F. ) ;
#17282=VERTEX_POINT ( 'NONE', #30502 ) ;
#17283=DIRECTION ( 'NONE',  ( 1.000000000000000000, 0.000000000000000000, 0.000000000000000000 ) ) ;
#17284=CIRCLE ( 'NONE', #32221, 2.000000000000001776 ) ;
#17285=CARTESIAN_POINT ( 'NONE',  ( 69.99999662536838230, -51.96152422706639840, -9.999999999999998224 ) ) ;
#17286=DIRECTION ( 'NONE',  ( 1.000000000000000000, 0.000000000000000000, 0.000000000000000000 ) ) ;
#17287=DIRECTION ( 'NONE',  ( 0.000000000000000000, 0.000000000000000000, 1.000000000000000000 ) ) ;
#17288=ORIENTED_EDGE ( 'NONE', *, *, #17534, .T. ) ;
#17289=VERTEX_POINT ( 'NONE', #33112 ) ;
#17290=CIRCLE ( 'NONE', #19091, 27.00000000000001066 ) ;
#17291=ADVANCED_FACE ( 'NONE', ( #7626 ), #28234, .T. ) ;
#17293=CARTESIAN_POINT ( 'NONE',  ( -47.00000337463112743, -60.62177826491080168, -9.999999999999998224 ) ) ;
#17294=DIRECTION ( 'NONE',  ( 0.000000000000000000, 0.000000000000000000, 1.000000000000000000 ) ) ;
#17295=CIRCLE ( 'NONE', #5922, 2.000000000000001776 ) ;
#17296=ORIENTED_EDGE ( 'NONE', *, *, #17832, .F. ) ;
#17297=CARTESIAN_POINT ( 'NONE',  ( -10.00000337463125000, -86.60254037844400443, 12.50000000000000000 ) ) ;
#17298=ORIENTED_EDGE ( 'NONE', *, *, #5790, .F. ) ;
#17300=ORIENTED_EDGE ( 'NONE', *, *, #25973, .F. ) ;
#17303=VERTEX_POINT ( 'NONE', #22414 ) ;
#17304=EDGE_LOOP ( 'NONE', ( #14759, #11212 ) ) ;
#17306=PLANE ( 'NONE',  #25622 ) ;
#17308=ORIENTED_EDGE ( 'NONE', *, *, #33665, .F. ) ;
#17309=FACE_OUTER_BOUND ( 'NONE', #25859, .T. ) ;
#17310=AXIS2_PLACEMENT_3D ( 'NONE', #18728, #19461, #16460 ) ;
#17311=ADVANCED_FACE ( 'NONE', ( #7433 ), #13811, .T. ) ;
#17312=FACE_BOUND ( 'NONE', #35376, .T. ) ;
#17313=CARTESIAN_POINT ( 'NONE',  ( -47.00000337463111322, 60.62177826491077326, -5.000000000000000000 ) ) ;
#17314=CARTESIAN_POINT ( 'NONE',  ( 22.99999662536857059, 77.94228634059957983, 17.49999999999999645 ) ) ;
#17315=DIRECTION ( 'NONE',  ( 0.000000000000000000, 0.000000000000000000, 1.000000000000000000 ) ) ;
#17316=CARTESIAN_POINT ( 'NONE',  ( 44.99999662536849598, 60.62177826491077326, 12.50000000000000000 ) ) ;
#17317=DIRECTION ( 'NONE',  ( 0.000000000000000000, 0.000000000000000000, 1.000000000000000000 ) ) ;
#17318=AXIS2_PLACEMENT_3D ( 'NONE', #33280, #7596, #16231 ) ;
#17320=ORIENTED_EDGE ( 'NONE', *, *, #33462, .F. ) ;
#17324=DIRECTION ( 'NONE',  ( 1.000000000000000000, 0.000000000000000000, 0.000000000000000000 ) ) ;
#17325=VERTEX_POINT ( 'NONE', #21682 ) ;
#17326=ORIENTED_EDGE ( 'NONE', *, *, #16519, .F. ) ;
#17328=ORIENTED_EDGE ( 'NONE', *, *, #1879, .F. ) ;
#17329=DIRECTION ( 'NONE',  ( -1.000000000000000000, 0.000000000000000000, 0.000000000000000000 ) ) ;
#17331=CIRCLE ( 'NONE', #32904, 1.999999999999998224 ) ;
#17333=ORIENTED_EDGE ( 'NONE', *, *, #21242, .F. ) ;
#17334=EDGE_CURVE ( 'NONE', #3043, #33094, #27941, .T. ) ;
#17335=DIRECTION ( 'NONE',  ( 0.000000000000000000, 0.000000000000000000, -1.000000000000000000 ) ) ;
#17336=CIRCLE ( 'NONE', #2225, 2.000000000000001776 ) ;
#17337=VECTOR ( 'NONE', #35003, 1000.000000000000000 ) ;
#17340=VERTEX_POINT ( 'NONE', #4634 ) ;
#17341=CIRCLE ( 'NONE', #19721, 2.000000000000001776 ) ;
#17342=CARTESIAN_POINT ( 'NONE',  ( 77.99999662536832545, -17.32050807568879591, 17.49999999999999645 ) ) ;
#17343=VERTEX_POINT ( 'NONE', #25249 ) ;
#17344=VERTEX_POINT ( 'NONE', #27500 ) ;
#17345=EDGE_CURVE ( 'NONE', #20978, #21059, #29138, .T. ) ;
#17346=LINE ( 'NONE', #14517, #5227 ) ;
#17347=DIRECTION ( 'NONE',  ( 0.000000000000000000, 0.000000000000000000, 1.000000000000000000 ) ) ;
#17349=ORIENTED_EDGE ( 'NONE', *, *, #25467, .T. ) ;
#17350=DIRECTION ( 'NONE',  ( 0.000000000000000000, 0.000000000000000000, 1.000000000000000000 ) ) ;
#17351=DIRECTION ( 'NONE',  ( 1.000000000000000000, 0.000000000000000000, 0.000000000000000000 ) ) ;
#17352=CARTESIAN_POINT ( 'NONE',  ( 11.99999662536862566, 86.60254037844397601, -9.999999999999998224 ) ) ;
#17353=AXIS2_PLACEMENT_3D ( 'NONE', #15295, #26928, #26545 ) ;
#17354=ORIENTED_EDGE ( 'NONE', *, *, #26308, .F. ) ;
#17355=CARTESIAN_POINT ( 'NONE',  ( 59.99999662536842493, 51.96152422706639129, -9.999999999999998224 ) ) ;
#17356=DIRECTION ( 'NONE',  ( 1.000000000000000000, 0.000000000000000000, 0.000000000000000000 ) ) ;
#17357=EDGE_LOOP ( 'NONE', ( #25144, #1020, #14923, #6757 ) ) ;
#17358=EDGE_CURVE ( 'NONE', #12964, #21989, #12972, .T. ) ;
#17359=FACE_OUTER_BOUND ( 'NONE', #35544, .T. ) ;
#17360=FACE_OUTER_BOUND ( 'NONE', #9535, .T. ) ;
#17361=AXIS2_PLACEMENT_3D ( 'NONE', #18034, #12756, #9772 ) ;
#17362=DIRECTION ( 'NONE',  ( 0.000000000000000000, 0.000000000000000000, 1.000000000000000000 ) ) ;
#17364=DIRECTION ( 'NONE',  ( 0.000000000000000000, 0.000000000000000000, 1.000000000000000000 ) ) ;
#17365=ORIENTED_EDGE ( 'NONE', *, *, #31595, .F. ) ;
#17366=AXIS2_PLACEMENT_3D ( 'NONE', #510, #26747, #1250 ) ;
#17368=CARTESIAN_POINT ( 'NONE',  ( 64.99999662536839651, -43.30127018922199511, -5.000000000000000000 ) ) ;
#17369=ORIENTED_EDGE ( 'NONE', *, *, #137, .T. ) ;
#17371=ORIENTED_EDGE ( 'NONE', *, *, #18867, .F. ) ;
#17372=ORIENTED_EDGE ( 'NONE', *, *, #12494, .T. ) ;
#17373=ADVANCED_FACE ( 'NONE', ( #33680 ), #2547, .F. ) ;
#17376=DIRECTION ( 'NONE',  ( 0.000000000000000000, 0.000000000000000000, 1.000000000000000000 ) ) ;
#17377=AXIS2_PLACEMENT_3D ( 'NONE', #21586, #33009, #28763 ) ;
#17378=EDGE_CURVE ( 'NONE', #23671, #24284, #19075, .T. ) ;
#17379=DIRECTION ( 'NONE',  ( -1.000000000000000000, 0.000000000000000000, 0.000000000000000000 ) ) ;
#17381=LINE ( 'NONE', #3126, #31100 ) ;
#17383=ORIENTED_EDGE ( 'NONE', *, *, #24523, .T. ) ;
#17384=FACE_BOUND ( 'NONE', #3376, .T. ) ;
#17385=AXIS2_PLACEMENT_3D ( 'NONE', #8622, #20255, #22709 ) ;
#17386=EDGE_CURVE ( 'NONE', #17794, #12035, #23748, .T. ) ;
#17388=VECTOR ( 'NONE', #2001, 1000.000000000000000 ) ;
#17389=CYLINDRICAL_SURFACE ( 'NONE', #3529, 2.000000000000001776 ) ;
#17390=DIRECTION ( 'NONE',  ( -1.000000000000000000, 0.000000000000000000, 0.000000000000000000 ) ) ;
#17392=CARTESIAN_POINT ( 'NONE',  ( -65.00000337463102085, 25.98076211353317433, -9.999999999999998224 ) ) ;
#17393=CARTESIAN_POINT ( 'NONE',  ( 48.49678893472093932, 67.96280274017779277, 12.50000000000000000 ) ) ;
#17394=CARTESIAN_POINT ( 'NONE',  ( -35.00000337463116296, 77.94228634059957983, 17.49999999999999645 ) ) ;
#17395=ORIENTED_EDGE ( 'NONE', *, *, #21162, .T. ) ;
#17396=AXIS2_PLACEMENT_3D ( 'NONE', #28751, #3076, #14497 ) ;
#17397=DIRECTION ( 'NONE',  ( 1.000000000000000000, 0.000000000000000000, 0.000000000000000000 ) ) ;
#17399=DIRECTION ( 'NONE',  ( 0.000000000000000000, 0.000000000000000000, -1.000000000000000000 ) ) ;
#17400=EDGE_LOOP ( 'NONE', ( #23498, #987 ) ) ;
#17401=EDGE_CURVE ( 'NONE', #8449, #30786, #6985, .T. ) ;
#17405=ORIENTED_EDGE ( 'NONE', *, *, #26768, .F. ) ;
#17406=ADVANCED_FACE ( 'NONE', ( #25077 ), #19255, .F. ) ;
#17407=PLANE ( 'NONE',  #2471 ) ;
#17408=EDGE_CURVE ( 'NONE', #14195, #34040, #31397, .T. ) ;
#17411=DIRECTION ( 'NONE',  ( 3.469446951953612611E-15, 1.000000000000000000, 0.000000000000000000 ) ) ;
#17412=CARTESIAN_POINT ( 'NONE',  ( 64.99999662536841072, -25.98076211353320275, -9.999999999999998224 ) ) ;
#17413=ORIENTED_EDGE ( 'NONE', *, *, #18943, .F. ) ;
#17414=ORIENTED_EDGE ( 'NONE', *, *, #33140, .T. ) ;
#17415=DIRECTION ( 'NONE',  ( 0.000000000000000000, 0.000000000000000000, 1.000000000000000000 ) ) ;
#17416=CARTESIAN_POINT ( 'NONE',  ( 76.99999662536836809, 8.660254037844394404, -9.999999999999998224 ) ) ;
#17417=DIRECTION ( 'NONE',  ( -1.000000000000000000, 0.000000000000000000, 0.000000000000000000 ) ) ;
#17418=ORIENTED_EDGE ( 'NONE', *, *, #26552, .T. ) ;
#17419=ADVANCED_FACE ( 'NONE', ( #6272 ), #100, .F. ) ;
#17420=FACE_BOUND ( 'NONE', #8993, .T. ) ;
#17422=ORIENTED_EDGE ( 'NONE', *, *, #24954, .F. ) ;
#17423=AXIS2_PLACEMENT_3D ( 'NONE', #19475, #25470, #10299 ) ;
#17424=DIRECTION ( 'NONE',  ( 0.000000000000000000, 0.000000000000000000, 1.000000000000000000 ) ) ;
#17425=ORIENTED_EDGE ( 'NONE', *, *, #13246, .T. ) ;
#17426=DIRECTION ( 'NONE',  ( 1.000000000000000000, 0.000000000000000000, 0.000000000000000000 ) ) ;
#17427=CARTESIAN_POINT ( 'NONE',  ( -10.00000337463127842, -69.28203230275519786, 12.50000000000000000 ) ) ;
#17428=EDGE_LOOP ( 'NONE', ( #26243, #32468 ) ) ;
#17430=EDGE_LOOP ( 'NONE', ( #34012, #15658 ) ) ;
#17432=ADVANCED_FACE ( 'NONE', ( #8374 ), #3276, .T. ) ;
#17434=DIRECTION ( 'NONE',  ( 1.000000000000000000, 0.000000000000000000, 0.000000000000000000 ) ) ;
#17436=VECTOR ( 'NONE', #2248, 1000.000000000000000 ) ;
#17437=CARTESIAN_POINT ( 'NONE',  ( 49.99999662536848177, -51.96152422706640550, 17.49999999999999645 ) ) ;
#17440=ORIENTED_EDGE ( 'NONE', *, *, #17249, .F. ) ;
#17441=CARTESIAN_POINT ( 'NONE',  ( 9.999996625368625658, 86.60254037844397601, -9.999999999999998224 ) ) ;
#17444=CARTESIAN_POINT ( 'NONE',  ( 82.99999662536832545, 25.98076211353319565, 12.50000000000000000 ) ) ;
#17445=ORIENTED_EDGE ( 'NONE', *, *, #23159, .T. ) ;
#17446=DIRECTION ( 'NONE',  ( 1.000000000000000000, 0.000000000000000000, 0.000000000000000000 ) ) ;
#17447=EDGE_CURVE ( 'NONE', #17289, #23885, #14532, .T. ) ;
#17448=FACE_OUTER_BOUND ( 'NONE', #32414, .T. ) ;
#17449=ADVANCED_FACE ( 'NONE', ( #22611 ), #19807, .F. ) ;
#17450=EDGE_LOOP ( 'NONE', ( #4260, #22179, #5823, #5842 ) ) ;
#17451=ORIENTED_EDGE ( 'NONE', *, *, #20538, .T. ) ;
#17453=DIRECTION ( 'NONE',  ( 0.000000000000000000, 0.000000000000000000, -1.000000000000000000 ) ) ;
#17454=CARTESIAN_POINT ( 'NONE',  ( 34.99999662536855283, -77.94228634059960825, -9.999999999999998224 ) ) ;
#17456=ORIENTED_EDGE ( 'NONE', *, *, #12812, .F. ) ;
#17457=EDGE_CURVE ( 'NONE', #29052, #5247, #12369, .T. ) ;
#17458=DIRECTION ( 'NONE',  ( -0.000000000000000000, -0.000000000000000000, 1.000000000000000000 ) ) ;
#17459=CARTESIAN_POINT ( 'NONE',  ( 52.99999662536846046, -43.30127018922200222, 12.50000000000000000 ) ) ;
#17460=ADVANCED_FACE ( 'NONE', ( #272 ), #8545, .F. ) ;
#17462=ADVANCED_FACE ( 'NONE', ( #25806 ), #28402, .F. ) ;
#17463=VERTEX_POINT ( 'NONE', #14713 ) ;
#17466=AXIS2_PLACEMENT_3D ( 'NONE', #26270, #1315, #3939 ) ;
#17468=ORIENTED_EDGE ( 'NONE', *, *, #36399, .F. ) ;
#17470=CYLINDRICAL_SURFACE ( 'NONE', #33189, 2.000000000000001776 ) ;
#17473=ORIENTED_EDGE ( 'NONE', *, *, #37031, .F. ) ;
#17474=DIRECTION ( 'NONE',  ( 0.000000000000000000, 0.000000000000000000, 1.000000000000000000 ) ) ;
#17475=DIRECTION ( 'NONE',  ( -1.000000000000000000, 0.000000000000000000, 0.000000000000000000 ) ) ;
#17476=CARTESIAN_POINT ( 'NONE',  ( -20.00000337463123756, -86.60254037844400443, -5.000000000000000000 ) ) ;
#17477=ORIENTED_EDGE ( 'NONE', *, *, #21775, .F. ) ;
#17478=DIRECTION ( 'NONE',  ( 1.000000000000000000, 0.000000000000000000, 0.000000000000000000 ) ) ;
#17479=FACE_BOUND ( 'NONE', #18442, .T. ) ;
#17480=DIRECTION ( 'NONE',  ( -0.4999999999999980016, 0.8660254037844398178, 0.000000000000000000 ) ) ;
#17482=CARTESIAN_POINT ( 'NONE',  ( -10.00000337463125000, -86.60254037844400443, -5.000000000000000000 ) ) ;
#17483=CARTESIAN_POINT ( 'NONE',  ( 72.99999662536835388, -43.30127018922199511, -9.999999999999998224 ) ) ;
#17485=DIRECTION ( 'NONE',  ( -1.000000000000000000, 0.000000000000000000, 0.000000000000000000 ) ) ;
#17486=ORIENTED_EDGE ( 'NONE', *, *, #29385, .F. ) ;
#17488=DIRECTION ( 'NONE',  ( 0.000000000000000000, 0.000000000000000000, 1.000000000000000000 ) ) ;
#17489=FACE_OUTER_BOUND ( 'NONE', #33076, .T. ) ;
#17490=ORIENTED_EDGE ( 'NONE', *, *, #30434, .F. ) ;
#17491=ORIENTED_EDGE ( 'NONE', *, *, #14831, .F. ) ;
#17492=ORIENTED_EDGE ( 'NONE', *, *, #23035, .F. ) ;
#17493=CARTESIAN_POINT ( 'NONE',  ( -53.00000337463109190, -60.62177826491083010, 12.50000000000000000 ) ) ;
#17494=DIRECTION ( 'NONE',  ( 1.000000000000000000, 0.000000000000000000, 0.000000000000000000 ) ) ;
#17495=DIRECTION ( 'NONE',  ( 0.000000000000000000, 0.000000000000000000, 1.000000000000000000 ) ) ;
#17498=AXIS2_PLACEMENT_3D ( 'NONE', #4719, #10706, #27185 ) ;
#17499=FACE_OUTER_BOUND ( 'NONE', #30611, .T. ) ;
#17502=EDGE_CURVE ( 'NONE', #10128, #36402, #25600, .T. ) ;
#17503=DIRECTION ( 'NONE',  ( 0.000000000000000000, 0.000000000000000000, 1.000000000000000000 ) ) ;
#17504=ORIENTED_EDGE ( 'NONE', *, *, #25263, .T. ) ;
#17505=CARTESIAN_POINT ( 'NONE',  ( 56.67878100130369035, -27.78182860042797131, -4.999999999999997335 ) ) ;
#17506=ORIENTED_EDGE ( 'NONE', *, *, #9640, .F. ) ;
#17508=FACE_OUTER_BOUND ( 'NONE', #34806, .T. ) ;
#17513=ORIENTED_EDGE ( 'NONE', *, *, #22726, .F. ) ;
#17514=LINE ( 'NONE', #3815, #25090 ) ;
#17515=FACE_OUTER_BOUND ( 'NONE', #16021, .T. ) ;
#17516=DIRECTION ( 'NONE',  ( -0.4999999999999980016, 0.8660254037844398178, 0.000000000000000000 ) ) ;
#17518=CYLINDRICAL_SURFACE ( 'NONE', #5776, 1.999999999999998224 ) ;
#17519=CARTESIAN_POINT ( 'NONE',  ( -50.00000337463110611, -69.28203230275519786, 12.50000000000000000 ) ) ;
#17520=ORIENTED_EDGE ( 'NONE', *, *, #27375, .F. ) ;
#17522=DIRECTION ( 'NONE',  ( -1.000000000000000000, 0.000000000000000000, 0.000000000000000000 ) ) ;
#17523=DIRECTION ( 'NONE',  ( 1.000000000000000000, 0.000000000000000000, 0.000000000000000000 ) ) ;
#17524=ADVANCED_FACE ( 'NONE', ( #11897 ), #29147, .F. ) ;
#17527=AXIS2_PLACEMENT_3D ( 'NONE', #19490, #27922, #10866 ) ;
#17528=CARTESIAN_POINT ( 'NONE',  ( -42.00000337463114164, 69.28203230275516944, -5.000000000000000000 ) ) ;
#17529=VERTEX_POINT ( 'NONE', #36854 ) ;
#17532=DIRECTION ( 'NONE',  ( -0.4999999999999979461, 0.8660254037844397068, 0.000000000000000000 ) ) ;
#17533=EDGE_LOOP ( 'NONE', ( #21172, #27400 ) ) ;
#17534=EDGE_CURVE ( 'NONE', #10828, #18808, #2726, .T. ) ;
#17535=EDGE_CURVE ( 'NONE', #33756, #32159, #9421, .T. ) ;
#17536=VERTEX_POINT ( 'NONE', #35167 ) ;
#17537=ORIENTED_EDGE ( 'NONE', *, *, #21226, .T. ) ;
#17538=CIRCLE ( 'NONE', #6748, 3.000000000000002665 ) ;
#17539=CARTESIAN_POINT ( 'NONE',  ( 72.99999662536836809, 25.98076211353319565, -9.999999999999998224 ) ) ;
#17540=FACE_OUTER_BOUND ( 'NONE', #32973, .T. ) ;
#17541=DIRECTION ( 'NONE',  ( 1.000000000000000000, 0.000000000000000000, 0.000000000000000000 ) ) ;
#17542=CARTESIAN_POINT ( 'NONE',  ( -70.00000337463099243, 51.96152422706637708, -9.999999999999998224 ) ) ;
#17543=EDGE_LOOP ( 'NONE', ( #8256, #14812 ) ) ;
#17544=ADVANCED_FACE ( 'NONE', ( #12449 ), #1216, .F. ) ;
#17545=CARTESIAN_POINT ( 'NONE',  ( -83.00000337463092137, 8.660254037844389075, -9.999999999999998224 ) ) ;
#17547=FACE_BOUND ( 'NONE', #23298, .T. ) ;
#17548=AXIS2_PLACEMENT_3D ( 'NONE', #28923, #20320, #31555 ) ;
#17549=CIRCLE ( 'NONE', #33736, 2.000000000000001776 ) ;
#17550=DIRECTION ( 'NONE',  ( 0.000000000000000000, 0.000000000000000000, 1.000000000000000000 ) ) ;
#17551=DIRECTION ( 'NONE',  ( 1.000000000000000000, 0.000000000000000000, 0.000000000000000000 ) ) ;
#17552=CARTESIAN_POINT ( 'NONE',  ( 54.99999662536846046, -43.30127018922200222, -9.999999999999998224 ) ) ;
#17554=DIRECTION ( 'NONE',  ( 1.000000000000000000, 0.000000000000000000, 0.000000000000000000 ) ) ;
#17556=DIRECTION ( 'NONE',  ( 0.000000000000000000, 0.000000000000000000, 1.000000000000000000 ) ) ;
#17557=CARTESIAN_POINT ( 'NONE',  ( -73.00000337463097821, 8.660254037844374864, -9.999999999999998224 ) ) ;
#17558=EDGE_CURVE ( 'NONE', #26515, #8511, #28552, .T. ) ;
#17559=EDGE_LOOP ( 'NONE', ( #10095, #5848 ) ) ;
#17560=DIRECTION ( 'NONE',  ( 0.000000000000000000, 0.000000000000000000, 1.000000000000000000 ) ) ;
#17561=DIRECTION ( 'NONE',  ( 0.000000000000000000, 0.000000000000000000, 1.000000000000000000 ) ) ;
#17562=LINE ( 'NONE', #516, #28493 ) ;
#17564=ORIENTED_EDGE ( 'NONE', *, *, #13088, .F. ) ;
#17567=AXIS2_PLACEMENT_3D ( 'NONE', #22176, #7541, #1535 ) ;
#17569=VECTOR ( 'NONE', #31812, 1000.000000000000000 ) ;
#17570=CARTESIAN_POINT ( 'NONE',  ( -65.00000337463106348, -60.62177826491083010, -5.000000000000000000 ) ) ;
#17571=ADVANCED_FACE ( 'NONE', ( #27074 ), #23915, .F. ) ;
#17572=ORIENTED_EDGE ( 'NONE', *, *, #10739, .T. ) ;
#17573=CARTESIAN_POINT ( 'NONE',  ( -90.00000337463090716, -1.040834085586084257E-14, -9.999999999999998224 ) ) ;
#17574=FACE_OUTER_BOUND ( 'NONE', #9637, .T. ) ;
#17575=CARTESIAN_POINT ( 'NONE',  ( 7.999996625368625658, 86.60254037844397601, -9.999999999999998224 ) ) ;
#17576=CYLINDRICAL_SURFACE ( 'NONE', #26961, 2.000000000000000000 ) ;
#17577=ORIENTED_EDGE ( 'NONE', *, *, #14247, .F. ) ;
#17578=CIRCLE ( 'NONE', #16393, 1.999999999999998224 ) ;
#17581=AXIS2_PLACEMENT_3D ( 'NONE', #19528, #36047, #22164 ) ;
#17582=CARTESIAN_POINT ( 'NONE',  ( -63.00000337463104927, -43.30127018922202353, -9.999999999999998224 ) ) ;
#17583=CARTESIAN_POINT ( 'NONE',  ( 26.99999662536856704, 77.94228634059957983, -9.999999999999998224 ) ) ;
#17584=ORIENTED_EDGE ( 'NONE', *, *, #33196, .T. ) ;
#17585=EDGE_CURVE ( 'NONE', #17896, #8583, #11210, .T. ) ;
#17586=FACE_BOUND ( 'NONE', #5810, .T. ) ;
#17589=DIRECTION ( 'NONE',  ( 1.000000000000000000, 0.000000000000000000, 0.000000000000000000 ) ) ;
#17591=ADVANCED_FACE ( 'NONE', ( #20909 ), #12637, .F. ) ;
#17592=AXIS2_PLACEMENT_3D ( 'NONE', #6668, #15667, #5096 ) ;
#17593=DIRECTION ( 'NONE',  ( -1.000000000000000000, 0.000000000000000000, 0.000000000000000000 ) ) ;
#17594=CARTESIAN_POINT ( 'NONE',  ( 19.99999662536861678, -86.60254037844400443, -9.999999999999998224 ) ) ;
#17595=ADVANCED_FACE ( 'NONE', ( #4024 ), #12805, .T. ) ;
#17596=ORIENTED_EDGE ( 'NONE', *, *, #26073, .F. ) ;
#17598=ORIENTED_EDGE ( 'NONE', *, *, #32963, .F. ) ;
#17599=AXIS2_PLACEMENT_3D ( 'NONE', #15203, #21021, #18197 ) ;
#17600=ORIENTED_EDGE ( 'NONE', *, *, #26073, .T. ) ;
#17601=ORIENTED_EDGE ( 'NONE', *, *, #10835, .T. ) ;
#17602=CARTESIAN_POINT ( 'NONE',  ( 67.99999662536839651, 51.96152422706640550, -9.999999999999998224 ) ) ;
#17604=ORIENTED_EDGE ( 'NONE', *, *, #35294, .T. ) ;
#17605=FACE_OUTER_BOUND ( 'NONE', #27788, .T. ) ;
#17607=FACE_OUTER_BOUND ( 'NONE', #24236, .T. ) ;
#17608=VERTEX_POINT ( 'NONE', #32897 ) ;
#17609=CARTESIAN_POINT ( 'NONE',  ( 86.99999662536832545, 25.98076211353319565, -5.000000000000000000 ) ) ;
#17611=EDGE_CURVE ( 'NONE', #5777, #28672, #417, .T. ) ;
#17613=ORIENTED_EDGE ( 'NONE', *, *, #13781, .F. ) ;
#17614=FACE_OUTER_BOUND ( 'NONE', #23211, .T. ) ;
#17617=VERTEX_POINT ( 'NONE', #18083 ) ;
#17620=DIRECTION ( 'NONE',  ( 0.000000000000000000, 0.000000000000000000, 1.000000000000000000 ) ) ;
#17621=DIRECTION ( 'NONE',  ( 1.000000000000000000, 0.000000000000000000, 0.000000000000000000 ) ) ;
#17622=CARTESIAN_POINT ( 'NONE',  ( 79.99999662536832545, -34.64101615137759183, -5.000000000000000000 ) ) ;
#17624=VERTEX_POINT ( 'NONE', #7024 ) ;
#17625=AXIS2_PLACEMENT_3D ( 'NONE', #26237, #17789, #29224 ) ;
#17626=DIRECTION ( 'NONE',  ( 0.000000000000000000, 0.000000000000000000, 1.000000000000000000 ) ) ;
#17628=CIRCLE ( 'NONE', #24855, 27.00000000000001066 ) ;
#17629=CARTESIAN_POINT ( 'NONE',  ( -85.00000337463092137, -8.660254037844422825, -9.999999999999998224 ) ) ;
#17630=EDGE_CURVE ( 'NONE', #20697, #25448, #35160, .T. ) ;
#17631=AXIS2_PLACEMENT_3D ( 'NONE', #22234, #4980, #36668 ) ;
#17634=DIRECTION ( 'NONE',  ( 0.000000000000000000, 0.000000000000000000, -1.000000000000000000 ) ) ;
#17636=CARTESIAN_POINT ( 'NONE',  ( -80.00000337463096400, -34.64101615137762025, -9.999999999999998224 ) ) ;
#17637=EDGE_CURVE ( 'NONE', #25578, #6350, #13002, .T. ) ;
#17638=CARTESIAN_POINT ( 'NONE',  ( -51.67317684408315870, -68.18636331025710717, -5.000000000000000000 ) ) ;
#17639=VECTOR ( 'NONE', #21730, 1000.000000000000000 ) ;
#17641=ORIENTED_EDGE ( 'NONE', *, *, #12109, .F. ) ;
#17642=AXIS2_PLACEMENT_3D ( 'NONE', #15090, #26519, #9476 ) ;
#17644=EDGE_CURVE ( 'NONE', #14287, #22341, #3478, .T. ) ;
#17645=DIRECTION ( 'NONE',  ( 0.000000000000000000, 0.000000000000000000, -1.000000000000000000 ) ) ;
#17647=CARTESIAN_POINT ( 'NONE',  ( -65.00000337463106348, -60.62177826491083010, -9.999999999999998224 ) ) ;
#17649=CIRCLE ( 'NONE', #2671, 27.00000000000001421 ) ;
#17650=ORIENTED_EDGE ( 'NONE', *, *, #25742, .T. ) ;
#17651=CYLINDRICAL_SURFACE ( 'NONE', #15975, 2.000000000000001776 ) ;
#17652=FACE_BOUND ( 'NONE', #30195, .T. ) ;
#17654=DIRECTION ( 'NONE',  ( 1.000000000000000000, 0.000000000000000000, 0.000000000000000000 ) ) ;
#17656=EDGE_CURVE ( 'NONE', #15620, #2172, #8802, .T. ) ;
#17657=DIRECTION ( 'NONE',  ( 1.000000000000000000, 0.000000000000000000, 0.000000000000000000 ) ) ;
#17658=CIRCLE ( 'NONE', #32006, 2.000000000000000000 ) ;
#17659=ADVANCED_FACE ( 'NONE', ( #12241 ), #3826, .F. ) ;
#17660=FACE_OUTER_BOUND ( 'NONE', #33809, .T. ) ;
#17661=ADVANCED_FACE ( 'NONE', ( #10932 ), #21813, .F. ) ;
#17662=EDGE_CURVE ( 'NONE', #15434, #14832, #30452, .T. ) ;
#17663=CARTESIAN_POINT ( 'NONE',  ( -65.00000337463106348, -60.62177826491083010, 17.49999999999999645 ) ) ;
#17665=EDGE_CURVE ( 'NONE', #34583, #3159, #36262, .T. ) ;
#17668=DIRECTION ( 'NONE',  ( 1.000000000000000000, 0.000000000000000000, 0.000000000000000000 ) ) ;
#17669=ORIENTED_EDGE ( 'NONE', *, *, #17386, .F. ) ;
#17670=ORIENTED_EDGE ( 'NONE', *, *, #23863, .T. ) ;
#17671=ORIENTED_EDGE ( 'NONE', *, *, #19293, .T. ) ;
#17673=CARTESIAN_POINT ( 'NONE',  ( -70.00000337463100664, -17.32050807568882078, 12.50000000000000000 ) ) ;
#17675=CIRCLE ( 'NONE', #23676, 2.000000000000001776 ) ;
#17676=DIRECTION ( 'NONE',  ( 1.000000000000000000, 0.000000000000000000, 0.000000000000000000 ) ) ;
#17677=VERTEX_POINT ( 'NONE', #13368 ) ;
#17678=EDGE_LOOP ( 'NONE', ( #102, #34075 ) ) ;
#17679=CIRCLE ( 'NONE', #33267, 2.000000000000001776 ) ;
#17680=AXIS2_PLACEMENT_3D ( 'NONE', #8203, #16832, #8006 ) ;
#17682=CARTESIAN_POINT ( 'NONE',  ( -48.00000337463112032, -51.96152422706641971, 17.49999999999999645 ) ) ;
#17683=EDGE_LOOP ( 'NONE', ( #33019, #4790 ) ) ;
#17684=DIRECTION ( 'NONE',  ( 0.000000000000000000, 0.000000000000000000, 1.000000000000000000 ) ) ;
#17686=CARTESIAN_POINT ( 'NONE',  ( -75.00000337463099243, -25.98076211353322051, -5.000000000000000000 ) ) ;
#17688=VECTOR ( 'NONE', #11154, 1000.000000000000000 ) ;
#17691=DIRECTION ( 'NONE',  ( 1.000000000000000000, 0.000000000000000000, 0.000000000000000000 ) ) ;
#17693=CARTESIAN_POINT ( 'NONE',  ( 27.78182860042856461, 56.67878100130339902, -4.999999999999997335 ) ) ;
#17694=EDGE_LOOP ( 'NONE', ( #29565, #33012, #23379, #6659, #14761 ) ) ;
#17695=DIRECTION ( 'NONE',  ( 1.000000000000000000, 0.000000000000000000, 0.000000000000000000 ) ) ;
#17696=DIRECTION ( 'NONE',  ( -0.000000000000000000, -0.000000000000000000, -1.000000000000000000 ) ) ;
#17698=AXIS2_PLACEMENT_3D ( 'NONE', #17482, #29641, #23481 ) ;
#17699=EDGE_LOOP ( 'NONE', ( #3368, #32634 ) ) ;
#17700=CARTESIAN_POINT ( 'NONE',  ( -80.00000337463096400, -34.64101615137762025, -9.999999999999998224 ) ) ;
#17701=DIRECTION ( 'NONE',  ( 0.000000000000000000, 0.000000000000000000, 1.000000000000000000 ) ) ;
#17703=DIRECTION ( 'NONE',  ( 0.000000000000000000, 0.000000000000000000, 1.000000000000000000 ) ) ;
#17704=AXIS2_PLACEMENT_3D ( 'NONE', #32646, #6970, #35663 ) ;
#17705=CARTESIAN_POINT ( 'NONE',  ( 4.999996625368645198, 77.94228634059957983, -5.000000000000000000 ) ) ;
#17707=AXIS2_PLACEMENT_3D ( 'NONE', #18136, #6704, #27312 ) ;
#17708=AXIS2_PLACEMENT_3D ( 'NONE', #35468, #3759, #1143 ) ;
#17712=ADVANCED_FACE ( 'NONE', ( #33814 ), #4394, .F. ) ;
#17713=DIRECTION ( 'NONE',  ( 0.000000000000000000, 0.000000000000000000, -1.000000000000000000 ) ) ;
#17715=LINE ( 'NONE', #6276, #8573 ) ;
#17718=DIRECTION ( 'NONE',  ( -1.000000000000000000, 0.000000000000000000, 0.000000000000000000 ) ) ;
#17719=CYLINDRICAL_SURFACE ( 'NONE', #16987, 2.000000000000001776 ) ;
#17720=VERTEX_POINT ( 'NONE', #30068 ) ;
#17721=AXIS2_PLACEMENT_3D ( 'NONE', #30133, #15897, #27331 ) ;
#17722=EDGE_LOOP ( 'NONE', ( #24054, #22330, #17133, #27045, #10115 ) ) ;
#17723=VERTEX_POINT ( 'NONE', #24650 ) ;
#17728=AXIS2_PLACEMENT_3D ( 'NONE', #1340, #6968, #18781 ) ;
#17729=CARTESIAN_POINT ( 'NONE',  ( -83.00000337463092137, -8.660254037844422825, 12.50000000000000000 ) ) ;
#17731=CARTESIAN_POINT ( 'NONE',  ( 4.999996625368645198, 77.94228634059957983, 12.50000000000000000 ) ) ;
#17732=ORIENTED_EDGE ( 'NONE', *, *, #35813, .F. ) ;
#17733=FACE_BOUND ( 'NONE', #23158, .T. ) ;
#17734=CIRCLE ( 'NONE', #18956, 3.000000000000001332 ) ;
#17736=AXIS2_PLACEMENT_3D ( 'NONE', #9130, #17958, #31980 ) ;
#17737=EDGE_CURVE ( 'NONE', #9159, #34784, #13597, .T. ) ;
#17738=AXIS2_PLACEMENT_3D ( 'NONE', #29296, #17865, #22937 ) ;
#17739=CIRCLE ( 'NONE', #12944, 2.000000000000001776 ) ;
#17741=CARTESIAN_POINT ( 'NONE',  ( 27.99999662536857414, -69.28203230275519786, -5.000000000000000000 ) ) ;
#17742=EDGE_LOOP ( 'NONE', ( #9082, #33607, #14925, #12400 ) ) ;
#17743=CARTESIAN_POINT ( 'NONE',  ( -43.00000337463111322, -77.94228634059960825, -9.999999999999998224 ) ) ;
#17745=CIRCLE ( 'NONE', #28531, 2.000000000000001776 ) ;
#17746=DIRECTION ( 'NONE',  ( -1.000000000000000000, 0.000000000000000000, 0.000000000000000000 ) ) ;
#17747=LINE ( 'NONE', #34651, #19195 ) ;
#17748=DIRECTION ( 'NONE',  ( -1.000000000000000000, 0.000000000000000000, -0.000000000000000000 ) ) ;
#17749=EDGE_LOOP ( 'NONE', ( #26675, #12979, #9648, #6884, #18331 ) ) ;
#17750=DIRECTION ( 'NONE',  ( 0.000000000000000000, 0.000000000000000000, 1.000000000000000000 ) ) ;
#17751=DIRECTION ( 'NONE',  ( 1.000000000000000000, 0.000000000000000000, 0.000000000000000000 ) ) ;
#17752=CARTESIAN_POINT ( 'NONE',  ( -80.00000337463094979, -17.32050807568882078, -9.999999999999998224 ) ) ;
#17753=VERTEX_POINT ( 'NONE', #1571 ) ;
#17754=ORIENTED_EDGE ( 'NONE', *, *, #32404, .F. ) ;
#17755=CIRCLE ( 'NONE', #2807, 2.000000000000000000 ) ;
#17756=EDGE_CURVE ( 'NONE', #31614, #12842, #29751, .T. ) ;
#17757=ORIENTED_EDGE ( 'NONE', *, *, #8672, .T. ) ;
#17759=DIRECTION ( 'NONE',  ( 0.000000000000000000, 0.000000000000000000, 1.000000000000000000 ) ) ;
#17760=CIRCLE ( 'NONE', #8774, 2.000000000000000000 ) ;
#17761=CIRCLE ( 'NONE', #4013, 2.000000000000001776 ) ;
#17762=CYLINDRICAL_SURFACE ( 'NONE', #7238, 2.000000000000001776 ) ;
#17764=CARTESIAN_POINT ( 'NONE',  ( -80.00000337463094979, -17.32050807568882078, 17.49999999999999645 ) ) ;
#17765=DIRECTION ( 'NONE',  ( 0.000000000000000000, 0.000000000000000000, 1.000000000000000000 ) ) ;
#17766=DIRECTION ( 'NONE',  ( 0.000000000000000000, 0.000000000000000000, 1.000000000000000000 ) ) ;
#17768=EDGE_LOOP ( 'NONE', ( #14848, #29763 ) ) ;
#17772=EDGE_CURVE ( 'NONE', #7403, #35706, #18397, .T. ) ;
#17773=DIRECTION ( 'NONE',  ( -1.000000000000000000, 0.000000000000000000, 0.000000000000000000 ) ) ;
#17775=VERTEX_POINT ( 'NONE', #35907 ) ;
#17777=ADVANCED_FACE ( 'NONE', ( #2330, #24826, #22012, #10216, #27803, #10766, #1770, #4582, #13759 ), #7943, .F. ) ;
#17778=AXIS2_PLACEMENT_3D ( 'NONE', #16718, #2461, #11261 ) ;
#17779=CIRCLE ( 'NONE', #34587, 1.999999999999998224 ) ;
#17780=FACE_BOUND ( 'NONE', #17277, .T. ) ;
#17781=ORIENTED_EDGE ( 'NONE', *, *, #25467, .F. ) ;
#17782=ORIENTED_EDGE ( 'NONE', *, *, #14115, .T. ) ;
#17783=ADVANCED_FACE ( 'NONE', ( #30796 ), #19023, .F. ) ;
#17784=VECTOR ( 'NONE', #35987, 1000.000000000000000 ) ;
#17785=DIRECTION ( 'NONE',  ( 0.000000000000000000, 0.000000000000000000, -1.000000000000000000 ) ) ;
#17788=CIRCLE ( 'NONE', #21387, 2.000000000000001776 ) ;
#17789=DIRECTION ( 'NONE',  ( 0.000000000000000000, 0.000000000000000000, 1.000000000000000000 ) ) ;
#17790=EDGE_CURVE ( 'NONE', #8725, #10442, #21390, .T. ) ;
#17791=FACE_OUTER_BOUND ( 'NONE', #2849, .T. ) ;
#17792=FACE_BOUND ( 'NONE', #33761, .T. ) ;
#17793=EDGE_LOOP ( 'NONE', ( #21347, #3079 ) ) ;
#17794=VERTEX_POINT ( 'NONE', #19216 ) ;
#17795=VECTOR ( 'NONE', #7623, 1000.000000000000000 ) ;
#17796=EDGE_LOOP ( 'NONE', ( #433, #30438, #24623, #32547 ) ) ;
#17797=EDGE_LOOP ( 'NONE', ( #17320, #3686, #33382, #16915 ) ) ;
#17799=DIRECTION ( 'NONE',  ( 0.000000000000000000, 0.000000000000000000, 1.000000000000000000 ) ) ;
#17801=EDGE_CURVE ( 'NONE', #31731, #36755, #32445, .T. ) ;
#17803=VERTEX_POINT ( 'NONE', #16932 ) ;
#17804=CARTESIAN_POINT ( 'NONE',  ( -20.00000337463123756, -69.28203230275522628, -5.000000000000000000 ) ) ;
#17808=VERTEX_POINT ( 'NONE', #17314 ) ;
#17809=CYLINDRICAL_SURFACE ( 'NONE', #16452, 2.000000000000001776 ) ;
#17810=VECTOR ( 'NONE', #19658, 1000.000000000000000 ) ;
#17811=DIRECTION ( 'NONE',  ( -0.000000000000000000, -0.000000000000000000, 1.000000000000000000 ) ) ;
#17812=CYLINDRICAL_SURFACE ( 'NONE', #15828, 2.000000000000001776 ) ;
#17813=ORIENTED_EDGE ( 'NONE', *, *, #34334, .T. ) ;
#17814=LINE ( 'NONE', #6186, #29211 ) ;
#17815=CARTESIAN_POINT ( 'NONE',  ( -10.00000337463128197, 86.60254037844397601, -9.999999999999998224 ) ) ;
#17816=ORIENTED_EDGE ( 'NONE', *, *, #7239, .T. ) ;
#17818=CIRCLE ( 'NONE', #9419, 2.000000000000001776 ) ;
#17819=ORIENTED_EDGE ( 'NONE', *, *, #16679, .F. ) ;
#17820=CIRCLE ( 'NONE', #1662, 2.000000000000001776 ) ;
#17821=CARTESIAN_POINT ( 'NONE',  ( -45.00000337463111322, 60.62177826491077326, 12.50000000000000000 ) ) ;
#17822=ADVANCED_FACE ( 'NONE', ( #25564 ), #36807, .F. ) ;
#17823=CARTESIAN_POINT ( 'NONE',  ( -75.00000337463099243, -25.98076211353322051, 12.50000000000000000 ) ) ;
#17825=CYLINDRICAL_SURFACE ( 'NONE', #11870, 2.000000000000001776 ) ;
#17826=ORIENTED_EDGE ( 'NONE', *, *, #35108, .F. ) ;
#17827=AXIS2_PLACEMENT_3D ( 'NONE', #4022, #9820, #7570 ) ;
#17829=CARTESIAN_POINT ( 'NONE',  ( 24.99999662536857059, 77.94228634059957983, -9.999999999999998224 ) ) ;
#17830=AXIS2_PLACEMENT_3D ( 'NONE', #17103, #31339, #25362 ) ;
#17831=ORIENTED_EDGE ( 'NONE', *, *, #6192, .T. ) ;
#17832=EDGE_CURVE ( 'NONE', #26576, #6626, #9704, .T. ) ;
#17835=DIRECTION ( 'NONE',  ( 1.000000000000000000, 0.000000000000000000, 0.000000000000000000 ) ) ;
#17836=ORIENTED_EDGE ( 'NONE', *, *, #13040, .T. ) ;
#17838=LINE ( 'NONE', #12009, #28467 ) ;
#17840=EDGE_CURVE ( 'NONE', #20086, #13680, #15105, .T. ) ;
#17841=CARTESIAN_POINT ( 'NONE',  ( -20.00000337463123756, -69.28203230275522628, -9.999999999999998224 ) ) ;
#17842=EDGE_LOOP ( 'NONE', ( #33306, #21024, #4914, #33277, #19204 ) ) ;
#17844=CARTESIAN_POINT ( 'NONE',  ( 64.99999662536842493, 43.30127018922200222, -9.999999999999998224 ) ) ;
#17846=DIRECTION ( 'NONE',  ( -0.000000000000000000, -0.000000000000000000, 1.000000000000000000 ) ) ;
#17847=AXIS2_PLACEMENT_3D ( 'NONE', #2241, #21929, #29997 ) ;
#17848=ORIENTED_EDGE ( 'NONE', *, *, #22659, .T. ) ;
#17849=DIRECTION ( 'NONE',  ( 0.000000000000000000, 0.000000000000000000, 1.000000000000000000 ) ) ;
#17850=FACE_BOUND ( 'NONE', #28501, .T. ) ;
#17851=DIRECTION ( 'NONE',  ( 0.000000000000000000, 0.000000000000000000, 1.000000000000000000 ) ) ;
#17852=DIRECTION ( 'NONE',  ( 0.000000000000000000, 0.000000000000000000, 1.000000000000000000 ) ) ;
#17853=AXIS2_PLACEMENT_3D ( 'NONE', #27541, #1853, #19657 ) ;
#17854=DIRECTION ( 'NONE',  ( 0.000000000000000000, 0.000000000000000000, -1.000000000000000000 ) ) ;
#17858=EDGE_CURVE ( 'NONE', #25623, #27946, #7915, .T. ) ;
#17860=CIRCLE ( 'NONE', #7082, 2.000000000000001776 ) ;
#17861=LINE ( 'NONE', #9779, #15181 ) ;
#17862=ORIENTED_EDGE ( 'NONE', *, *, #4264, .F. ) ;
#17863=DIRECTION ( 'NONE',  ( -1.000000000000000000, 0.000000000000000000, 0.000000000000000000 ) ) ;
#17864=CIRCLE ( 'NONE', #23874, 2.000000000000001776 ) ;
#17865=DIRECTION ( 'NONE',  ( 0.000000000000000000, 0.000000000000000000, 1.000000000000000000 ) ) ;
#17866=DIRECTION ( 'NONE',  ( 1.000000000000000000, 0.000000000000000000, 0.000000000000000000 ) ) ;
#17867=VECTOR ( 'NONE', #9474, 1000.000000000000000 ) ;
#17868=ORIENTED_EDGE ( 'NONE', *, *, #12302, .F. ) ;
#17870=VERTEX_POINT ( 'NONE', #28903 ) ;
#17871=VERTEX_POINT ( 'NONE', #14488 ) ;
#17872=AXIS2_PLACEMENT_3D ( 'NONE', #16856, #2237, #19479 ) ;
#17873=EDGE_CURVE ( 'NONE', #32213, #4038, #21074, .T. ) ;
#17874=DIRECTION ( 'NONE',  ( -1.000000000000000000, 0.000000000000000000, 0.000000000000000000 ) ) ;
#17875=CARTESIAN_POINT ( 'NONE',  ( -44.13139720814439215, -27.49999999999955591, -5.000000000000000000 ) ) ;
#17877=CARTESIAN_POINT ( 'NONE',  ( 72.99999662536836809, 25.98076211353319565, -5.000000000000000000 ) ) ;
#17879=ORIENTED_EDGE ( 'NONE', *, *, #11086, .T. ) ;
#17880=ORIENTED_EDGE ( 'NONE', *, *, #9426, .F. ) ;
#17881=AXIS2_PLACEMENT_3D ( 'NONE', #9021, #3042, #22734 ) ;
#17882=AXIS2_PLACEMENT_3D ( 'NONE', #29499, #3818, #15257 ) ;
#17883=DIRECTION ( 'NONE',  ( 0.000000000000000000, 0.000000000000000000, 1.000000000000000000 ) ) ;
#17884=ORIENTED_EDGE ( 'NONE', *, *, #27274, .T. ) ;
#17887=CARTESIAN_POINT ( 'NONE',  ( 74.99999662536836809, -8.660254037844401509, 17.49999999999999645 ) ) ;
#17888=EDGE_LOOP ( 'NONE', ( #29450, #2771, #2961, #9408, #19804, #3185 ) ) ;
#17890=DIRECTION ( 'NONE',  ( 0.000000000000000000, 0.000000000000000000, 1.000000000000000000 ) ) ;
#17891=DIRECTION ( 'NONE',  ( 1.000000000000000000, 0.000000000000000000, 0.000000000000000000 ) ) ;
#17892=ADVANCED_FACE ( 'NONE', ( #14110 ), #17118, .T. ) ;
#17893=CIRCLE ( 'NONE', #11280, 2.000000000000001776 ) ;
#17894=DIRECTION ( 'NONE',  ( 0.000000000000000000, 0.000000000000000000, 1.000000000000000000 ) ) ;
#17896=VERTEX_POINT ( 'NONE', #31002 ) ;
#17898=CARTESIAN_POINT ( 'NONE',  ( 37.99999662536853151, 69.28203230275518365, 17.49999999999999645 ) ) ;
#17899=CARTESIAN_POINT ( 'NONE',  ( 44.13139720814401556, -27.50000000000022737, -5.000000000000000000 ) ) ;
#17901=DIRECTION ( 'NONE',  ( 1.000000000000000000, 0.000000000000000000, 0.000000000000000000 ) ) ;
#17902=DIRECTION ( 'NONE',  ( -1.000000000000000000, 0.000000000000000000, 0.000000000000000000 ) ) ;
#17903=CIRCLE ( 'NONE', #3533, 2.000000000000001776 ) ;
#17904=VERTEX_POINT ( 'NONE', #22763 ) ;
#17905=CARTESIAN_POINT ( 'NONE',  ( -25.00000337463121980, -77.94228634059963667, -9.999999999999998224 ) ) ;
#17906=LINE ( 'NONE', #22978, #17867 ) ;
#17908=AXIS2_PLACEMENT_3D ( 'NONE', #34683, #23230, #1093 ) ;
#17909=DIRECTION ( 'NONE',  ( -0.000000000000000000, -0.000000000000000000, 1.000000000000000000 ) ) ;
#17911=EDGE_CURVE ( 'NONE', #11966, #31223, #14314, .T. ) ;
#17912=CARTESIAN_POINT ( 'NONE',  ( 84.99999662536832545, 25.98076211353319565, -9.999999999999998224 ) ) ;
#17913=DIRECTION ( 'NONE',  ( 0.000000000000000000, 0.000000000000000000, 1.000000000000000000 ) ) ;
#17914=AXIS2_PLACEMENT_3D ( 'NONE', #3662, #6274, #35170 ) ;
#17915=EDGE_LOOP ( 'NONE', ( #31825, #12575 ) ) ;
#17916=ADVANCED_FACE ( 'NONE', ( #5336 ), #2883, .T. ) ;
#17917=DIRECTION ( 'NONE',  ( -0.000000000000000000, -0.000000000000000000, 1.000000000000000000 ) ) ;
#17918=CARTESIAN_POINT ( 'NONE',  ( 61.99999662536842493, 51.96152422706639129, 12.50000000000000000 ) ) ;
#17919=CYLINDRICAL_SURFACE ( 'NONE', #35578, 33.00000000000001421 ) ;
#17920=EDGE_LOOP ( 'NONE', ( #7535, #16728, #28527, #4295 ) ) ;
#17922=VERTEX_POINT ( 'NONE', #28740 ) ;
#17923=AXIS2_PLACEMENT_3D ( 'NONE', #7855, #16658, #27539 ) ;
#17925=DIRECTION ( 'NONE',  ( 0.000000000000000000, 0.000000000000000000, 1.000000000000000000 ) ) ;
#17926=EDGE_CURVE ( 'NONE', #28198, #31907, #33067, .T. ) ;
#17927=VECTOR ( 'NONE', #4112, 1000.000000000000000 ) ;
#17928=CARTESIAN_POINT ( 'NONE',  ( 44.99999662536849598, -77.94228634059960825, -5.000000000000000000 ) ) ;
#17929=DIRECTION ( 'NONE',  ( 1.000000000000000000, 0.000000000000000000, 0.000000000000000000 ) ) ;
#17930=FACE_OUTER_BOUND ( 'NONE', #9819, .T. ) ;
#17931=VERTEX_POINT ( 'NONE', #19570 ) ;
#17932=CIRCLE ( 'NONE', #29291, 2.000000000000001776 ) ;
#17933=CARTESIAN_POINT ( 'NONE',  ( -63.00000337463102085, 60.62177826491077326, 17.49999999999999645 ) ) ;
#17934=ORIENTED_EDGE ( 'NONE', *, *, #18033, .F. ) ;
#17935=FACE_BOUND ( 'NONE', #26690, .T. ) ;
#17936=AXIS2_PLACEMENT_3D ( 'NONE', #36880, #28074, #5951 ) ;
#17938=ADVANCED_FACE ( 'NONE', ( #3068 ), #25923, .F. ) ;
#17939=AXIS2_PLACEMENT_3D ( 'NONE', #20730, #21108, #7057 ) ;
#17940=DIRECTION ( 'NONE',  ( 0.000000000000000000, 0.000000000000000000, 1.000000000000000000 ) ) ;
#17941=EDGE_CURVE ( 'NONE', #22919, #34990, #609, .T. ) ;
#17943=FACE_BOUND ( 'NONE', #24111, .T. ) ;
#17945=LINE ( 'NONE', #26548, #9860 ) ;
#17946=CARTESIAN_POINT ( 'NONE',  ( -20.00000337463123756, -86.60254037844400443, -9.999999999999998224 ) ) ;
#17947=AXIS2_PLACEMENT_3D ( 'NONE', #11393, #8575, #3315 ) ;
#17948=DIRECTION ( 'NONE',  ( 0.000000000000000000, 0.000000000000000000, -1.000000000000000000 ) ) ;
#17950=ORIENTED_EDGE ( 'NONE', *, *, #27648, .F. ) ;
#17951=CARTESIAN_POINT ( 'NONE',  ( 0.000000000000000000, 0.000000000000000000, 12.49999999999999822 ) ) ;
#17953=CARTESIAN_POINT ( 'NONE',  ( -65.00000337463102085, 60.62177826491077326, -9.999999999999998224 ) ) ;
#17954=DIRECTION ( 'NONE',  ( 1.000000000000000000, 0.000000000000000000, 0.000000000000000000 ) ) ;
#17957=ORIENTED_EDGE ( 'NONE', *, *, #18622, .T. ) ;
#17958=DIRECTION ( 'NONE',  ( 0.000000000000000000, 0.000000000000000000, 1.000000000000000000 ) ) ;
#17959=DIRECTION ( 'NONE',  ( 0.000000000000000000, 0.000000000000000000, -1.000000000000000000 ) ) ;
#17960=ADVANCED_FACE ( 'NONE', ( #26300 ), #15042, .F. ) ;
#17961=DIRECTION ( 'NONE',  ( 1.000000000000000000, 0.000000000000000000, 0.000000000000000000 ) ) ;
#17962=CIRCLE ( 'NONE', #3517, 1.999999999999998224 ) ;
#17963=AXIS2_PLACEMENT_3D ( 'NONE', #9778, #30029, #12399 ) ;
#17964=DIRECTION ( 'NONE',  ( -1.000000000000000000, 0.000000000000000000, 0.000000000000000000 ) ) ;
#17966=VECTOR ( 'NONE', #22155, 1000.000000000000000 ) ;
#17967=DIRECTION ( 'NONE',  ( 0.000000000000000000, 0.000000000000000000, -1.000000000000000000 ) ) ;
#17968=EDGE_LOOP ( 'NONE', ( #30584, #12330, #20662, #24994, #26772 ) ) ;
#17970=CYLINDRICAL_SURFACE ( 'NONE', #12886, 2.000000000000000000 ) ;
#17971=CIRCLE ( 'NONE', #19166, 2.000000000000001776 ) ;
#17972=CYLINDRICAL_SURFACE ( 'NONE', #8585, 2.000000000000001776 ) ;
#17974=CARTESIAN_POINT ( 'NONE',  ( 4.999996625368645198, 77.94228634059957983, -5.000000000000000000 ) ) ;
#17977=FACE_BOUND ( 'NONE', #19512, .T. ) ;
#17978=VERTEX_POINT ( 'NONE', #29458 ) ;
#17979=VERTEX_POINT ( 'NONE', #23480 ) ;
#17980=EDGE_CURVE ( 'NONE', #12977, #5893, #19298, .T. ) ;
#17981=AXIS2_PLACEMENT_3D ( 'NONE', #26479, #15426, #27564 ) ;
#17982=DIRECTION ( 'NONE',  ( 0.000000000000000000, 0.000000000000000000, 1.000000000000000000 ) ) ;
#17983=ORIENTED_EDGE ( 'NONE', *, *, #24667, .T. ) ;
#17986=DIRECTION ( 'NONE',  ( 0.000000000000000000, 0.000000000000000000, 1.000000000000000000 ) ) ;
#17987=AXIS2_PLACEMENT_3D ( 'NONE', #366, #23262, #31849 ) ;
#17988=ORIENTED_EDGE ( 'NONE', *, *, #35261, .T. ) ;
#17989=ORIENTED_EDGE ( 'NONE', *, *, #32564, .F. ) ;
#17990=ORIENTED_EDGE ( 'NONE', *, *, #20162, .F. ) ;
#17991=ORIENTED_EDGE ( 'NONE', *, *, #9739, .F. ) ;
#17992=ORIENTED_EDGE ( 'NONE', *, *, #13228, .F. ) ;
#17993=CARTESIAN_POINT ( 'NONE',  ( 4.279621169095998212, -62.97617850287780072, -49.86561046011506448 ) ) ;
#17995=ORIENTED_EDGE ( 'NONE', *, *, #5057, .T. ) ;
#17996=CARTESIAN_POINT ( 'NONE',  ( -27.00000337463120914, 77.94228634059957983, 17.49999999999999645 ) ) ;
#17999=EDGE_CURVE ( 'NONE', #14051, #15920, #32642, .T. ) ;
#18001=CARTESIAN_POINT ( 'NONE',  ( 31.46585318596250502, 86.45172111230321832, -4.999999999999997335 ) ) ;
#18003=CARTESIAN_POINT ( 'NONE',  ( 35.19434990244975126, -52.39915983220758022, -49.22241343995298024 ) ) ;
#18004=CARTESIAN_POINT ( 'NONE',  ( -70.00000337463102085, -51.96152422706641971, 17.49999999999999645 ) ) ;
#18005=ORIENTED_EDGE ( 'NONE', *, *, #18624, .T. ) ;
#18006=CARTESIAN_POINT ( 'NONE',  ( -25.00000337463120914, 77.94228634059957983, -9.999999999999998224 ) ) ;
#18008=DIRECTION ( 'NONE',  ( 0.000000000000000000, 0.000000000000000000, -1.000000000000000000 ) ) ;
#18009=VERTEX_POINT ( 'NONE', #26468 ) ;
#18010=VERTEX_POINT ( 'NONE', #21032 ) ;
#18013=FACE_OUTER_BOUND ( 'NONE', #29332, .T. ) ;
#18014=CIRCLE ( 'NONE', #14425, 2.000000000000001776 ) ;
#18015=CARTESIAN_POINT ( 'NONE',  ( -4.279621169095561228, 62.97617850287782915, -49.86561046011506448 ) ) ;
#18016=DIRECTION ( 'NONE',  ( 0.000000000000000000, 0.000000000000000000, 1.000000000000000000 ) ) ;
#18017=VERTEX_POINT ( 'NONE', #26654 ) ;
#18019=DIRECTION ( 'NONE',  ( 0.000000000000000000, 0.000000000000000000, 1.000000000000000000 ) ) ;
#18020=VERTEX_POINT ( 'NONE', #1168 ) ;
#18022=DIRECTION ( 'NONE',  ( -1.000000000000000000, 0.000000000000000000, 0.000000000000000000 ) ) ;
#18024=LINE ( 'NONE', #29446, #13912 ) ;
#18025=DIRECTION ( 'NONE',  ( -1.000000000000000000, -2.569960705150823820E-15, 0.000000000000000000 ) ) ;
#18026=DIRECTION ( 'NONE',  ( 1.000000000000000000, 0.000000000000000000, 0.000000000000000000 ) ) ;
#18027=EDGE_LOOP ( 'NONE', ( #19649, #25863, #24970, #7181, #31500 ) ) ;
#18028=ORIENTED_EDGE ( 'NONE', *, *, #32366, .F. ) ;
#18029=CARTESIAN_POINT ( 'NONE',  ( -83.00000337463092137, -25.98076211353322051, -9.999999999999998224 ) ) ;
#18030=CARTESIAN_POINT ( 'NONE',  ( -73.00000337463097821, 8.660254037844374864, -9.999999999999998224 ) ) ;
#18032=CARTESIAN_POINT ( 'NONE',  ( 6.999996625368645198, 77.94228634059957983, 12.50000000000000000 ) ) ;
#18033=EDGE_CURVE ( 'NONE', #26254, #30697, #6702, .T. ) ;
#18034=CARTESIAN_POINT ( 'NONE',  ( 39.99999662536853151, 69.28203230275518365, -9.999999999999998224 ) ) ;
#18037=DIRECTION ( 'NONE',  ( -1.000000000000000000, 0.000000000000000000, 0.000000000000000000 ) ) ;
#18039=CARTESIAN_POINT ( 'NONE',  ( -70.00000337463099243, 51.96152422706637708, -9.999999999999998224 ) ) ;
#18041=CYLINDRICAL_SURFACE ( 'NONE', #22386, 3.000000000000002665 ) ;
#18042=ORIENTED_EDGE ( 'NONE', *, *, #22280, .F. ) ;
#18044=EDGE_CURVE ( 'NONE', #5564, #34031, #112, .T. ) ;
#18045=FACE_OUTER_BOUND ( 'NONE', #11382, .T. ) ;
#18046=LINE ( 'NONE', #20861, #27572 ) ;
#18047=ORIENTED_EDGE ( 'NONE', *, *, #7581, .F. ) ;
#18049=EDGE_CURVE ( 'NONE', #11321, #35086, #14492, .T. ) ;
#18050=AXIS2_PLACEMENT_3D ( 'NONE', #13196, #24643, #10372 ) ;
#18052=DIRECTION ( 'NONE',  ( 1.000000000000000000, 0.000000000000000000, 0.000000000000000000 ) ) ;
#18053=CARTESIAN_POINT ( 'NONE',  ( 4.999996625368645198, 77.94228634059957983, 12.50000000000000000 ) ) ;
#18054=ORIENTED_EDGE ( 'NONE', *, *, #19574, .T. ) ;
#18055=CIRCLE ( 'NONE', #1898, 2.000000000000001776 ) ;
#18056=ORIENTED_EDGE ( 'NONE', *, *, #18993, .F. ) ;
#18057=ORIENTED_EDGE ( 'NONE', *, *, #18812, .T. ) ;
#18058=FACE_OUTER_BOUND ( 'NONE', #33704, .T. ) ;
#18059=EDGE_LOOP ( 'NONE', ( #27569, #21691, #9149 ) ) ;
#18061=ORIENTED_EDGE ( 'NONE', *, *, #6656, .F. ) ;
#18062=DIRECTION ( 'NONE',  ( 0.000000000000000000, 0.000000000000000000, 1.000000000000000000 ) ) ;
#18063=ORIENTED_EDGE ( 'NONE', *, *, #2780, .F. ) ;
#18064=EDGE_LOOP ( 'NONE', ( #30949, #32657 ) ) ;
#18065=EDGE_CURVE ( 'NONE', #17340, #36526, #16903, .T. ) ;
#18066=DIRECTION ( 'NONE',  ( 1.000000000000000000, 0.000000000000000000, 0.000000000000000000 ) ) ;
#18068=ORIENTED_EDGE ( 'NONE', *, *, #2164, .F. ) ;
#18069=ORIENTED_EDGE ( 'NONE', *, *, #12735, .F. ) ;
#18070=DIRECTION ( 'NONE',  ( 0.000000000000000000, 0.000000000000000000, 1.000000000000000000 ) ) ;
#18071=DIRECTION ( 'NONE',  ( 0.000000000000000000, 0.000000000000000000, -1.000000000000000000 ) ) ;
#18072=EDGE_CURVE ( 'NONE', #26842, #35523, #722, .T. ) ;
#18076=CARTESIAN_POINT ( 'NONE',  ( -34.00000000000027711, -58.88972745734168512, 12.49999999999999822 ) ) ;
#18077=CARTESIAN_POINT ( 'NONE',  ( 71.99999662536838230, -34.64101615137759183, -9.999999999999998224 ) ) ;
#18078=AXIS2_PLACEMENT_3D ( 'NONE', #16767, #19760, #24211 ) ;
#18079=EDGE_CURVE ( 'NONE', #24231, #27194, #3728, .T. ) ;
#18083=CARTESIAN_POINT ( 'NONE',  ( -52.00000337463110611, -69.28203230275519786, -5.000000000000000000 ) ) ;
#18084=DIRECTION ( 'NONE',  ( -1.000000000000000000, 0.000000000000000000, 0.000000000000000000 ) ) ;
#18085=CARTESIAN_POINT ( 'NONE',  ( -55.88972745734203329, -33.99999999999965894, -49.86561046011506448 ) ) ;
#18088=DIRECTION ( 'NONE',  ( 0.000000000000000000, 0.000000000000000000, -1.000000000000000000 ) ) ;
#18089=CARTESIAN_POINT ( 'NONE',  ( -27.00000337463120914, 77.94228634059957983, -5.000000000000000000 ) ) ;
#18092=EDGE_LOOP ( 'NONE', ( #1520, #16956, #18497, #10238 ) ) ;
#18093=ORIENTED_EDGE ( 'NONE', *, *, #36714, .T. ) ;
#18094=EDGE_CURVE ( 'NONE', #15624, #17979, #20471, .T. ) ;
#18096=CARTESIAN_POINT ( 'NONE',  ( 0.000000000000000000, 0.000000000000000000, -5.000000000000000000 ) ) ;
#18097=DIRECTION ( 'NONE',  ( 0.000000000000000000, 0.000000000000000000, 1.000000000000000000 ) ) ;
#18098=DIRECTION ( 'NONE',  ( -1.000000000000000000, 0.000000000000000000, 0.000000000000000000 ) ) ;
#18099=CIRCLE ( 'NONE', #1938, 3.499999999999987566 ) ;
#18100=CARTESIAN_POINT ( 'NONE',  ( 86.99999662536832545, 25.98076211353319565, -9.999999999999998224 ) ) ;
#18101=VERTEX_POINT ( 'NONE', #5081 ) ;
#18103=ORIENTED_EDGE ( 'NONE', *, *, #19958, .F. ) ;
#18104=FACE_BOUND ( 'NONE', #18433, .T. ) ;
#18105=EDGE_CURVE ( 'NONE', #30085, #13632, #4330, .T. ) ;
#18106=FACE_OUTER_BOUND ( 'NONE', #4917, .T. ) ;
#18107=DIRECTION ( 'NONE',  ( -1.000000000000000000, 0.000000000000000000, -0.000000000000000000 ) ) ;
#18109=ORIENTED_EDGE ( 'NONE', *, *, #1746, .F. ) ;
#18110=DIRECTION ( 'NONE',  ( 1.000000000000000000, 0.000000000000000000, 0.000000000000000000 ) ) ;
#18114=AXIS2_PLACEMENT_3D ( 'NONE', #20481, #6433, #8881 ) ;
#18115=CARTESIAN_POINT ( 'NONE',  ( 36.99999662536855283, -60.62177826491080168, -5.000000000000000000 ) ) ;
#18116=DIRECTION ( 'NONE',  ( 0.000000000000000000, 0.000000000000000000, 1.000000000000000000 ) ) ;
#18117=ORIENTED_EDGE ( 'NONE', *, *, #10347, .T. ) ;
#18118=DIRECTION ( 'NONE',  ( 0.000000000000000000, 0.000000000000000000, 1.000000000000000000 ) ) ;
#18119=EDGE_CURVE ( 'NONE', #2201, #8255, #29464, .T. ) ;
#18120=DIRECTION ( 'NONE',  ( 0.000000000000000000, 0.000000000000000000, 1.000000000000000000 ) ) ;
#18122=EDGE_CURVE ( 'NONE', #8851, #30126, #7902, .T. ) ;
#18123=VERTEX_POINT ( 'NONE', #33407 ) ;
#18127=CIRCLE ( 'NONE', #28900, 33.00000000000001421 ) ;
#18128=CARTESIAN_POINT ( 'NONE',  ( -45.00000337463111322, 60.62177826491077326, 12.50000000000000000 ) ) ;
#18130=ADVANCED_FACE ( 'NONE', ( #33599 ), #13327, .T. ) ;
#18131=EDGE_CURVE ( 'NONE', #30229, #25550, #9103, .T. ) ;
#18134=ADVANCED_FACE ( 'NONE', ( #15970 ), #30758, .F. ) ;
#18135=CARTESIAN_POINT ( 'NONE',  ( 84.99999662536832545, 8.660254037844394404, -5.000000000000000000 ) ) ;
#18136=CARTESIAN_POINT ( 'NONE',  ( 52.39915983220795681, 35.19434990244919703, -4.999999999999997335 ) ) ;
#18137=EDGE_CURVE ( 'NONE', #6640, #2842, #32466, .T. ) ;
#18138=DIRECTION ( 'NONE',  ( -1.000000000000000000, 0.000000000000000000, 0.000000000000000000 ) ) ;
#18139=ORIENTED_EDGE ( 'NONE', *, *, #12131, .T. ) ;
#18141=AXIS2_PLACEMENT_3D ( 'NONE', #25892, #34523, #21576 ) ;
#18142=DIRECTION ( 'NONE',  ( 1.000000000000000000, 0.000000000000000000, 0.000000000000000000 ) ) ;
#18143=DIRECTION ( 'NONE',  ( 0.000000000000000000, 0.000000000000000000, 1.000000000000000000 ) ) ;
#18144=EDGE_LOOP ( 'NONE', ( #874, #29384, #16264, #9098 ) ) ;
#18145=CARTESIAN_POINT ( 'NONE',  ( 64.99999662536839651, -60.62177826491080168, -5.000000000000000000 ) ) ;
#18146=ORIENTED_EDGE ( 'NONE', *, *, #21568, .T. ) ;
#18147=CARTESIAN_POINT ( 'NONE',  ( -66.86787810013036903, 2.778182860042780700, -4.999999999999997335 ) ) ;
#18148=VERTEX_POINT ( 'NONE', #27405 ) ;
#18149=CIRCLE ( 'NONE', #32491, 3.000000000000002665 ) ;
#18150=ORIENTED_EDGE ( 'NONE', *, *, #3904, .T. ) ;
#18155=CARTESIAN_POINT ( 'NONE',  ( 66.99999662536839651, -60.62177826491080168, 17.49999999999999645 ) ) ;
#18157=ORIENTED_EDGE ( 'NONE', *, *, #2954, .F. ) ;
#18158=VERTEX_POINT ( 'NONE', #36214 ) ;
#18159=CIRCLE ( 'NONE', #9157, 2.000000000000001776 ) ;
#18160=ORIENTED_EDGE ( 'NONE', *, *, #10813, .F. ) ;
#18161=ORIENTED_EDGE ( 'NONE', *, *, #25158, .F. ) ;
#18163=ORIENTED_EDGE ( 'NONE', *, *, #18094, .T. ) ;
#18166=EDGE_LOOP ( 'NONE', ( #4362, #7315 ) ) ;
#18170=ORIENTED_EDGE ( 'NONE', *, *, #27137, .F. ) ;
#18171=CARTESIAN_POINT ( 'NONE',  ( -83.10591231744739105, 8.018055418181152305, -5.000000000000000000 ) ) ;
#18172=CIRCLE ( 'NONE', #2012, 2.000000000000001776 ) ;
#18173=CARTESIAN_POINT ( 'NONE',  ( 56.74224907229030634, -68.66839587347224949, -4.999999999999997335 ) ) ;
#18174=CIRCLE ( 'NONE', #180, 2.000000000000001776 ) ;
#18175=EDGE_CURVE ( 'NONE', #18010, #22677, #29489, .T. ) ;
#18176=FACE_OUTER_BOUND ( 'NONE', #21930, .T. ) ;
#18177=ORIENTED_EDGE ( 'NONE', *, *, #18949, .T. ) ;
#18178=DIRECTION ( 'NONE',  ( 1.000000000000000000, 0.000000000000000000, 0.000000000000000000 ) ) ;
#18179=CARTESIAN_POINT ( 'NONE',  ( 24.99999662536859546, -77.94228634059960825, 12.50000000000000000 ) ) ;
#18180=AXIS2_PLACEMENT_3D ( 'NONE', #17368, #11907, #23369 ) ;
#18181=ORIENTED_EDGE ( 'NONE', *, *, #4190, .F. ) ;
#18182=VERTEX_POINT ( 'NONE', #7171 ) ;
#18183=CARTESIAN_POINT ( 'NONE',  ( 65.00000000000000000, 7.960204194457797252E-15, 17.49999999999999645 ) ) ;
#18184=DIRECTION ( 'NONE',  ( 0.000000000000000000, 0.000000000000000000, 1.000000000000000000 ) ) ;
#18185=CARTESIAN_POINT ( 'NONE',  ( -68.00000337463100664, -17.32050807568882078, -5.000000000000000000 ) ) ;
#18189=CARTESIAN_POINT ( 'NONE',  ( -75.00000337463097821, 8.660254037844374864, -9.999999999999998224 ) ) ;
#18190=CIRCLE ( 'NONE', #22994, 2.000000000000000000 ) ;
#18192=DIRECTION ( 'NONE',  ( 0.000000000000000000, 0.000000000000000000, -1.000000000000000000 ) ) ;
#18193=ORIENTED_EDGE ( 'NONE', *, *, #3879, .F. ) ;
#18194=EDGE_CURVE ( 'NONE', #13427, #17922, #12955, .T. ) ;
#18195=CARTESIAN_POINT ( 'NONE',  ( 0.000000000000000000, 0.000000000000000000, 12.49999999999999822 ) ) ;
#18197=DIRECTION ( 'NONE',  ( -1.000000000000000000, 0.000000000000000000, 0.000000000000000000 ) ) ;
#18200=ORIENTED_EDGE ( 'NONE', *, *, #30380, .F. ) ;
#18202=DIRECTION ( 'NONE',  ( 1.000000000000000000, 0.000000000000000000, 0.000000000000000000 ) ) ;
#18203=ORIENTED_EDGE ( 'NONE', *, *, #22250, .F. ) ;
#18204=CARTESIAN_POINT ( 'NONE',  ( 9.999996625368655856, -86.60254037844400443, -9.999999999999998224 ) ) ;
#18205=FACE_BOUND ( 'NONE', #16043, .T. ) ;
#18206=DIRECTION ( 'NONE',  ( 0.000000000000000000, 0.000000000000000000, -1.000000000000000000 ) ) ;
#18207=CARTESIAN_POINT ( 'NONE',  ( -70.00000337463102085, -51.96152422706641971, -9.999999999999998224 ) ) ;
#18208=LINE ( 'NONE', #23862, #8130 ) ;
#18209=EDGE_LOOP ( 'NONE', ( #26686, #32554 ) ) ;
#18212=CARTESIAN_POINT ( 'NONE',  ( -3.499999999999987566, -55.00000000000000000, -10.00000000000000178 ) ) ;
#18213=EDGE_CURVE ( 'NONE', #23401, #21975, #30400, .T. ) ;
#18216=CARTESIAN_POINT ( 'NONE',  ( 86.99999662536831124, -25.98076211353319565, -9.999999999999998224 ) ) ;
#18218=DIRECTION ( 'NONE',  ( 1.000000000000000000, 0.000000000000000000, 0.000000000000000000 ) ) ;
#18221=VECTOR ( 'NONE', #31292, 1000.000000000000000 ) ;
#18222=VERTEX_POINT ( 'NONE', #27199 ) ;
#18223=AXIS2_PLACEMENT_3D ( 'NONE', #34329, #14068, #31494 ) ;
#18224=DIRECTION ( 'NONE',  ( 0.000000000000000000, 0.000000000000000000, 1.000000000000000000 ) ) ;
#18225=DIRECTION ( 'NONE',  ( 1.000000000000000000, 0.000000000000000000, 0.000000000000000000 ) ) ;
#18226=DIRECTION ( 'NONE',  ( 1.000000000000000000, 0.000000000000000000, 0.000000000000000000 ) ) ;
#18227=ORIENTED_EDGE ( 'NONE', *, *, #1295, .T. ) ;
#18228=VERTEX_POINT ( 'NONE', #24416 ) ;
#18229=ORIENTED_EDGE ( 'NONE', *, *, #11475, .T. ) ;
#18232=ORIENTED_EDGE ( 'NONE', *, *, #31674, .F. ) ;
#18234=AXIS2_PLACEMENT_3D ( 'NONE', #28852, #20427, #31838 ) ;
#18235=ORIENTED_EDGE ( 'NONE', *, *, #24026, .T. ) ;
#18236=LINE ( 'NONE', #4000, #5821 ) ;
#18237=VERTEX_POINT ( 'NONE', #19711 ) ;
#18238=EDGE_CURVE ( 'NONE', #8351, #26162, #24724, .T. ) ;
#18240=AXIS2_PLACEMENT_3D ( 'NONE', #34172, #16902, #31501 ) ;
#18241=CARTESIAN_POINT ( 'NONE',  ( -18.00000337463123756, -69.28203230275522628, -9.999999999999998224 ) ) ;
#18242=CYLINDRICAL_SURFACE ( 'NONE', #27240, 2.000000000000001776 ) ;
#18243=ORIENTED_EDGE ( 'NONE', *, *, #16762, .T. ) ;
#18244=EDGE_CURVE ( 'NONE', #33756, #14593, #31683, .T. ) ;
#18245=ORIENTED_EDGE ( 'NONE', *, *, #31331, .F. ) ;
#18246=FACE_OUTER_BOUND ( 'NONE', #15597, .T. ) ;
#18248=CIRCLE ( 'NONE', #13455, 2.000000000000001776 ) ;
#18249=CARTESIAN_POINT ( 'NONE',  ( 1.999996625368696490, -86.60254037844400443, 17.49999999999999645 ) ) ;
#18250=CIRCLE ( 'NONE', #23043, 95.00000000000001421 ) ;
#18251=DIRECTION ( 'NONE',  ( 0.000000000000000000, 0.000000000000000000, 1.000000000000000000 ) ) ;
#18252=VECTOR ( 'NONE', #13986, 1000.000000000000000 ) ;
#18253=EDGE_CURVE ( 'NONE', #13437, #13179, #2560, .T. ) ;
#18254=ORIENTED_EDGE ( 'NONE', *, *, #19242, .F. ) ;
#18255=CARTESIAN_POINT ( 'NONE',  ( -47.63139720814438505, -27.49999999999955591, -5.000000000000000000 ) ) ;
#18256=FACE_OUTER_BOUND ( 'NONE', #10032, .T. ) ;
#18258=DIRECTION ( 'NONE',  ( 0.000000000000000000, 0.000000000000000000, 1.000000000000000000 ) ) ;
#18259=CARTESIAN_POINT ( 'NONE',  ( 58.88972745734226066, 33.99999999999924682, -49.86561046011506448 ) ) ;
#18260=DIRECTION ( 'NONE',  ( 0.000000000000000000, 0.000000000000000000, 1.000000000000000000 ) ) ;
#18261=CARTESIAN_POINT ( 'NONE',  ( -72.00000337463100664, 17.32050807568877460, -9.999999999999998224 ) ) ;
#18262=DIRECTION ( 'NONE',  ( 1.000000000000000000, 0.000000000000000000, 0.000000000000000000 ) ) ;
#18263=CIRCLE ( 'NONE', #23030, 3.000000000000002665 ) ;
#18265=ORIENTED_EDGE ( 'NONE', *, *, #2455, .F. ) ;
#18266=CARTESIAN_POINT ( 'NONE',  ( -25.00000337463120914, 77.94228634059957983, -5.000000000000000000 ) ) ;
#18267=AXIS2_PLACEMENT_3D ( 'NONE', #6824, #12242, #6100 ) ;
#18269=LINE ( 'NONE', #6833, #21718 ) ;
#18270=CIRCLE ( 'NONE', #9299, 2.000000000000001776 ) ;
#18271=ORIENTED_EDGE ( 'NONE', *, *, #44, .F. ) ;
#18274=ORIENTED_EDGE ( 'NONE', *, *, #9881, .T. ) ;
#18276=CARTESIAN_POINT ( 'NONE',  ( 34.46585318596250858, 86.45172111230321832, -4.999999999999997335 ) ) ;
#18277=PLANE ( 'NONE',  #5276 ) ;
#18278=CARTESIAN_POINT ( 'NONE',  ( 56.74224907229030634, -68.66839587347224949, 12.49999999999999645 ) ) ;
#18280=AXIS2_PLACEMENT_3D ( 'NONE', #25238, #8364, #33850 ) ;
#18281=ADVANCED_FACE ( 'NONE', ( #14444 ), #22328, .F. ) ;
#18282=CIRCLE ( 'NONE', #2116, 27.00000000000001421 ) ;
#18283=FACE_OUTER_BOUND ( 'NONE', #23592, .T. ) ;
#18284=FACE_OUTER_BOUND ( 'NONE', #16783, .T. ) ;
#18285=ORIENTED_EDGE ( 'NONE', *, *, #15967, .F. ) ;
#18286=ADVANCED_FACE ( 'NONE', ( #25878 ), #36959, .F. ) ;
#18288=DIRECTION ( 'NONE',  ( 1.000000000000000000, 0.000000000000000000, 0.000000000000000000 ) ) ;
#18289=ORIENTED_EDGE ( 'NONE', *, *, #29591, .T. ) ;
#18290=FACE_BOUND ( 'NONE', #2543, .T. ) ;
#18291=DIRECTION ( 'NONE',  ( 0.000000000000000000, 0.000000000000000000, 1.000000000000000000 ) ) ;
#18293=AXIS2_PLACEMENT_3D ( 'NONE', #19964, #36841, #34051 ) ;
#18295=AXIS2_PLACEMENT_3D ( 'NONE', #17316, #7945, #20111 ) ;
#18296=EDGE_LOOP ( 'NONE', ( #25665, #27867, #35977, #22804 ) ) ;
#18298=CIRCLE ( 'NONE', #12911, 3.000000000000002665 ) ;
#18299=AXIS2_PLACEMENT_3D ( 'NONE', #20084, #25900, #5651 ) ;
#18301=AXIS2_PLACEMENT_3D ( 'NONE', #9842, #23738, #7048 ) ;
#18302=CIRCLE ( 'NONE', #33270, 2.000000000000001776 ) ;
#18305=DIRECTION ( 'NONE',  ( 0.000000000000000000, 0.000000000000000000, 1.000000000000000000 ) ) ;
#18307=EDGE_LOOP ( 'NONE', ( #15272, #16208, #37025 ) ) ;
#18310=DIRECTION ( 'NONE',  ( 0.000000000000000000, 0.000000000000000000, 1.000000000000000000 ) ) ;
#18311=CIRCLE ( 'NONE', #3346, 95.00000000000000000 ) ;
#18312=EDGE_LOOP ( 'NONE', ( #6679, #7020 ) ) ;
#18313=ORIENTED_EDGE ( 'NONE', *, *, #29941, .F. ) ;
#18314=ORIENTED_EDGE ( 'NONE', *, *, #29752, .T. ) ;
#18315=CARTESIAN_POINT ( 'NONE',  ( -72.00000337463100664, -17.32050807568882078, -9.999999999999998224 ) ) ;
#18316=CARTESIAN_POINT ( 'NONE',  ( 17.99999662536858125, 86.60254037844397601, -9.999999999999998224 ) ) ;
#18317=AXIS2_PLACEMENT_3D ( 'NONE', #22604, #19418, #31043 ) ;
#18318=DIRECTION ( 'NONE',  ( 0.000000000000000000, 0.000000000000000000, 1.000000000000000000 ) ) ;
#18319=EDGE_CURVE ( 'NONE', #20996, #35319, #18726, .T. ) ;
#18320=CIRCLE ( 'NONE', #10533, 27.00000000000001421 ) ;
#18321=CARTESIAN_POINT ( 'NONE',  ( 0.000000000000000000, 55.00000000000000000, -10.00000000000000000 ) ) ;
#18322=CARTESIAN_POINT ( 'NONE',  ( -40.00000337463113453, 69.28203230275516944, 12.50000000000000000 ) ) ;
#18323=EDGE_CURVE ( 'NONE', #14606, #35117, #133, .T. ) ;
#18325=CIRCLE ( 'NONE', #2161, 2.000000000000001776 ) ;
#18328=ORIENTED_EDGE ( 'NONE', *, *, #12498, .F. ) ;
#18329=ADVANCED_FACE ( 'NONE', ( #25169 ), #20257, .F. ) ;
#18330=CIRCLE ( 'NONE', #30903, 2.000000000000001776 ) ;
#18331=ORIENTED_EDGE ( 'NONE', *, *, #3671, .F. ) ;
#18332=FACE_OUTER_BOUND ( 'NONE', #5997, .T. ) ;
#18333=CARTESIAN_POINT ( 'NONE',  ( -2.374207310413330682E-13, -68.00000000000000000, -4.999999999999997335 ) ) ;
#18334=ORIENTED_EDGE ( 'NONE', *, *, #28412, .T. ) ;
#18335=EDGE_CURVE ( 'NONE', #792, #35451, #11440, .T. ) ;
#18336=DIRECTION ( 'NONE',  ( 0.000000000000000000, 0.000000000000000000, 1.000000000000000000 ) ) ;
#18338=ORIENTED_EDGE ( 'NONE', *, *, #12176, .T. ) ;
#18339=FACE_OUTER_BOUND ( 'NONE', #791, .T. ) ;
#18341=AXIS2_PLACEMENT_3D ( 'NONE', #34726, #2859, #20445 ) ;
#18342=DIRECTION ( 'NONE',  ( 0.000000000000000000, 0.000000000000000000, 1.000000000000000000 ) ) ;
#18343=VERTEX_POINT ( 'NONE', #25330 ) ;
#18344=EDGE_LOOP ( 'NONE', ( #26486, #20439 ) ) ;
#18346=ORIENTED_EDGE ( 'NONE', *, *, #419, .T. ) ;
#18347=EDGE_CURVE ( 'NONE', #26170, #7831, #11067, .T. ) ;
#18349=AXIS2_PLACEMENT_3D ( 'NONE', #22198, #36633, #33635 ) ;
#18350=EDGE_CURVE ( 'NONE', #2100, #25853, #35491, .T. ) ;
#18354=DIRECTION ( 'NONE',  ( 0.000000000000000000, 0.000000000000000000, 1.000000000000000000 ) ) ;
#18355=CARTESIAN_POINT ( 'NONE',  ( -25.00000337463120914, 77.94228634059957983, 17.49999999999999645 ) ) ;
#18356=ORIENTED_EDGE ( 'NONE', *, *, #34788, .T. ) ;
#18357=ORIENTED_EDGE ( 'NONE', *, *, #33232, .T. ) ;
#18360=VERTEX_POINT ( 'NONE', #28695 ) ;
#18361=VECTOR ( 'NONE', #33117, 1000.000000000000000 ) ;
#18362=AXIS2_PLACEMENT_3D ( 'NONE', #9223, #20656, #20311 ) ;
#18363=ORIENTED_EDGE ( 'NONE', *, *, #20778, .T. ) ;
#18364=ORIENTED_EDGE ( 'NONE', *, *, #8629, .T. ) ;
#18365=CARTESIAN_POINT ( 'NONE',  ( -58.00000337463104216, 51.96152422706639129, -9.999999999999998224 ) ) ;
#18367=EDGE_LOOP ( 'NONE', ( #560, #1240 ) ) ;
#18368=CARTESIAN_POINT ( 'NONE',  ( -22.00000337463124112, -69.28203230275522628, -5.000000000000000000 ) ) ;
#18369=LINE ( 'NONE', #15365, #3144 ) ;
#18370=CYLINDRICAL_SURFACE ( 'NONE', #26756, 2.000000000000001776 ) ;
#18371=ORIENTED_EDGE ( 'NONE', *, *, #8860, .T. ) ;
#18372=CARTESIAN_POINT ( 'NONE',  ( -33.99999999999945288, 58.88972745734214698, -4.999999999999997335 ) ) ;
#18373=AXIS2_PLACEMENT_3D ( 'NONE', #17505, #31751, #12046 ) ;
#18374=DIRECTION ( 'NONE',  ( 1.000000000000000000, 0.000000000000000000, 0.000000000000000000 ) ) ;
#18377=ORIENTED_EDGE ( 'NONE', *, *, #24172, .T. ) ;
#18378=DIRECTION ( 'NONE',  ( 0.000000000000000000, 0.000000000000000000, -1.000000000000000000 ) ) ;
#18379=EDGE_CURVE ( 'NONE', #3118, #25301, #29423, .T. ) ;
#18380=DIRECTION ( 'NONE',  ( 1.000000000000000000, 0.000000000000000000, 0.000000000000000000 ) ) ;
#18381=ORIENTED_EDGE ( 'NONE', *, *, #34354, .F. ) ;
#18382=CIRCLE ( 'NONE', #32746, 33.00000000000001421 ) ;
#18384=LINE ( 'NONE', #18183, #13445 ) ;
#18385=AXIS2_PLACEMENT_3D ( 'NONE', #1301, #10477, #21171 ) ;
#18387=CARTESIAN_POINT ( 'NONE',  ( -61.53067111003215217, 72.28378166042038799, -49.22241343995295892 ) ) ;
#18388=DIRECTION ( 'NONE',  ( 1.000000000000000000, 0.000000000000000000, 0.000000000000000000 ) ) ;
#18389=DIRECTION ( 'NONE',  ( -1.000000000000000000, 0.000000000000000000, 0.000000000000000000 ) ) ;
#18390=EDGE_CURVE ( 'NONE', #35025, #1395, #31859, .T. ) ;
#18391=ORIENTED_EDGE ( 'NONE', *, *, #10566, .F. ) ;
#18392=ORIENTED_EDGE ( 'NONE', *, *, #31869, .F. ) ;
#18394=AXIS2_PLACEMENT_3D ( 'NONE', #21, #11449, #22894 ) ;
#18396=AXIS2_PLACEMENT_3D ( 'NONE', #5451, #33948, #28297 ) ;
#18397=CIRCLE ( 'NONE', #2226, 2.000000000000000000 ) ;
#18398=ORIENTED_EDGE ( 'NONE', *, *, #5215, .T. ) ;
#18399=CARTESIAN_POINT ( 'NONE',  ( -67.00000337463104927, -43.30127018922202353, -5.000000000000000000 ) ) ;
#18400=ORIENTED_EDGE ( 'NONE', *, *, #31062, .T. ) ;
#18401=EDGE_CURVE ( 'NONE', #6597, #22278, #15129, .T. ) ;
#18402=CARTESIAN_POINT ( 'NONE',  ( 41.99999662536853151, -69.28203230275519786, -9.999999999999998224 ) ) ;
#18405=LINE ( 'NONE', #29833, #9225 ) ;
#18407=DIRECTION ( 'NONE',  ( 0.000000000000000000, 0.000000000000000000, -1.000000000000000000 ) ) ;
#18408=EDGE_CURVE ( 'NONE', #7069, #6161, #18369, .T. ) ;
#18409=VERTEX_POINT ( 'NONE', #26809 ) ;
#18410=ORIENTED_EDGE ( 'NONE', *, *, #3690, .F. ) ;
#18411=AXIS2_PLACEMENT_3D ( 'NONE', #18259, #29691, #15265 ) ;
#18412=AXIS2_PLACEMENT_3D ( 'NONE', #27894, #19463, #17214 ) ;
#18413=VECTOR ( 'NONE', #12642, 1000.000000000000000 ) ;
#18414=ORIENTED_EDGE ( 'NONE', *, *, #246, .F. ) ;
#18415=CARTESIAN_POINT ( 'NONE',  ( 76.99999662536836809, 43.30127018922198801, -9.999999999999998224 ) ) ;
#18416=FACE_OUTER_BOUND ( 'NONE', #2487, .T. ) ;
#18417=DIRECTION ( 'NONE',  ( 1.000000000000000000, 0.000000000000000000, 0.000000000000000000 ) ) ;
#18420=EDGE_LOOP ( 'NONE', ( #4546, #27620 ) ) ;
#18421=CYLINDRICAL_SURFACE ( 'NONE', #12301, 2.000000000000001776 ) ;
#18422=CIRCLE ( 'NONE', #29191, 2.000000000000001776 ) ;
#18423=CIRCLE ( 'NONE', #24420, 2.000000000000001776 ) ;
#18426=EDGE_LOOP ( 'NONE', ( #8552, #14295, #12106, #3348, #342 ) ) ;
#18427=CARTESIAN_POINT ( 'NONE',  ( 35.19434990244975126, -52.39915983220758022, -4.999999999999997335 ) ) ;
#18428=FACE_BOUND ( 'NONE', #10670, .T. ) ;
#18429=LINE ( 'NONE', #32472, #7825 ) ;
#18431=ADVANCED_FACE ( 'NONE', ( #9365 ), #14613, .F. ) ;
#18432=ORIENTED_EDGE ( 'NONE', *, *, #26539, .F. ) ;
#18433=EDGE_LOOP ( 'NONE', ( #8147, #3349 ) ) ;
#18434=AXIS2_PLACEMENT_3D ( 'NONE', #7918, #15992, #36056 ) ;
#18435=DIRECTION ( 'NONE',  ( 1.000000000000000000, 0.000000000000000000, 0.000000000000000000 ) ) ;
#18436=CARTESIAN_POINT ( 'NONE',  ( -50.00000337463109190, 69.28203230275518365, -9.999999999999998224 ) ) ;
#18437=DIRECTION ( 'NONE',  ( 0.000000000000000000, 0.000000000000000000, 1.000000000000000000 ) ) ;
#18438=ORIENTED_EDGE ( 'NONE', *, *, #6465, .F. ) ;
#18439=EDGE_LOOP ( 'NONE', ( #27234, #18802 ) ) ;
#18440=CIRCLE ( 'NONE', #2267, 2.000000000000001776 ) ;
#18441=AXIS2_PLACEMENT_3D ( 'NONE', #33406, #10519, #30589 ) ;
#18442=EDGE_LOOP ( 'NONE', ( #25114, #20061 ) ) ;
#18443=CIRCLE ( 'NONE', #1682, 2.000000000000000000 ) ;
#18444=CARTESIAN_POINT ( 'NONE',  ( -75.00000337463097821, 25.98076211353318854, -9.999999999999998224 ) ) ;
#18445=CIRCLE ( 'NONE', #26815, 3.000000000000002665 ) ;
#18447=ORIENTED_EDGE ( 'NONE', *, *, #329, .F. ) ;
#18448=DIRECTION ( 'NONE',  ( 0.000000000000000000, 0.000000000000000000, 1.000000000000000000 ) ) ;
#18449=ORIENTED_EDGE ( 'NONE', *, *, #14017, .F. ) ;
#18450=ORIENTED_EDGE ( 'NONE', *, *, #18379, .F. ) ;
#18451=CIRCLE ( 'NONE', #2905, 45.00000000000000711 ) ;
#18452=DIRECTION ( 'NONE',  ( 1.000000000000000000, 0.000000000000000000, -0.000000000000000000 ) ) ;
#18455=ORIENTED_EDGE ( 'NONE', *, *, #7657, .T. ) ;
#18457=CARTESIAN_POINT ( 'NONE',  ( -78.00000337463094979, 34.64101615137757051, -5.000000000000000000 ) ) ;
#18458=AXIS2_PLACEMENT_3D ( 'NONE', #25115, #31260, #34276 ) ;
#18459=CARTESIAN_POINT ( 'NONE',  ( 56.99999662536846046, -43.30127018922200222, -9.999999999999998224 ) ) ;
#18461=CARTESIAN_POINT ( 'NONE',  ( 34.99999662536855283, -77.94228634059960825, -5.000000000000000000 ) ) ;
#18462=VERTEX_POINT ( 'NONE', #20430 ) ;
#18463=FACE_OUTER_BOUND ( 'NONE', #28933, .T. ) ;
#18465=VERTEX_POINT ( 'NONE', #1474 ) ;
#18466=CYLINDRICAL_SURFACE ( 'NONE', #22151, 2.000000000000000000 ) ;
#18467=CIRCLE ( 'NONE', #30423, 2.000000000000001776 ) ;
#18468=VECTOR ( 'NONE', #24779, 1000.000000000000000 ) ;
#18471=DIRECTION ( 'NONE',  ( 1.000000000000000000, 0.000000000000000000, 0.000000000000000000 ) ) ;
#18472=CIRCLE ( 'NONE', #22059, 2.000000000000001776 ) ;
#18473=DIRECTION ( 'NONE',  ( -1.051347561198064495E-14, -1.000000000000000000, 0.000000000000000000 ) ) ;
#18474=VECTOR ( 'NONE', #36603, 1000.000000000000000 ) ;
#18477=CARTESIAN_POINT ( 'NONE',  ( 34.99999662536853862, 77.94228634059959404, -9.999999999999998224 ) ) ;
#18478=CARTESIAN_POINT ( 'NONE',  ( -80.00000337463094979, -2.428612866367529932E-14, 17.49999999999999645 ) ) ;
#18479=CARTESIAN_POINT ( 'NONE',  ( -45.00000337463111322, 60.62177826491077326, -9.999999999999998224 ) ) ;
#18480=EDGE_CURVE ( 'NONE', #7831, #13768, #18099, .T. ) ;
#18482=CIRCLE ( 'NONE', #32241, 33.00000000000001421 ) ;
#18483=VERTEX_POINT ( 'NONE', #18923 ) ;
#18484=ORIENTED_EDGE ( 'NONE', *, *, #27040, .F. ) ;
#18485=DIRECTION ( 'NONE',  ( -1.000000000000000000, 0.000000000000000000, 0.000000000000000000 ) ) ;
#18486=DIRECTION ( 'NONE',  ( -1.000000000000000000, 0.000000000000000000, -0.000000000000000000 ) ) ;
#18487=DIRECTION ( 'NONE',  ( -1.000000000000000000, 0.000000000000000000, 0.000000000000000000 ) ) ;
#18488=EDGE_CURVE ( 'NONE', #5388, #12428, #15724, .T. ) ;
#18489=VERTEX_POINT ( 'NONE', #21728 ) ;
#18490=CIRCLE ( 'NONE', #13064, 2.000000000000001776 ) ;
#18492=CARTESIAN_POINT ( 'NONE',  ( -10.00000337463128730, 69.28203230275516944, -9.999999999999998224 ) ) ;
#18493=EDGE_CURVE ( 'NONE', #2053, #29771, #9722, .T. ) ;
#18495=ORIENTED_EDGE ( 'NONE', *, *, #29786, .T. ) ;
#18496=CARTESIAN_POINT ( 'NONE',  ( 44.13139720814420031, 27.49999999999988987, -10.00000000000000000 ) ) ;
#18497=ORIENTED_EDGE ( 'NONE', *, *, #3650, .F. ) ;
#18498=CIRCLE ( 'NONE', #6521, 2.000000000000001776 ) ;
#18499=CARTESIAN_POINT ( 'NONE',  ( 76.99999662536836809, 43.30127018922198801, 17.49999999999999645 ) ) ;
#18500=CARTESIAN_POINT ( 'NONE',  ( -33.00000337463116296, -60.62177826491080168, -9.999999999999998224 ) ) ;
#18501=AXIS2_PLACEMENT_3D ( 'NONE', #12299, #9134, #14577 ) ;
#18503=AXIS2_PLACEMENT_3D ( 'NONE', #30045, #15440, #35881 ) ;
#18504=DIRECTION ( 'NONE',  ( 0.000000000000000000, 0.000000000000000000, 1.000000000000000000 ) ) ;
#18506=ORIENTED_EDGE ( 'NONE', *, *, #36596, .T. ) ;
#18507=LINE ( 'NONE', #24861, #29653 ) ;
#18508=AXIS2_PLACEMENT_3D ( 'NONE', #14587, #34297, #20233 ) ;
#18509=DIRECTION ( 'NONE',  ( 0.000000000000000000, 0.000000000000000000, -1.000000000000000000 ) ) ;
#18510=VECTOR ( 'NONE', #29279, 1000.000000000000000 ) ;
#18511=CARTESIAN_POINT ( 'NONE',  ( 0.000000000000000000, 0.000000000000000000, 12.49999999999999822 ) ) ;
#18512=CYLINDRICAL_SURFACE ( 'NONE', #31113, 2.000000000000001776 ) ;
#18513=ORIENTED_EDGE ( 'NONE', *, *, #11690, .T. ) ;
#18514=CARTESIAN_POINT ( 'NONE',  ( 84.99999662536832545, 8.660254037844394404, -9.999999999999998224 ) ) ;
#18519=CIRCLE ( 'NONE', #14926, 2.000000000000000000 ) ;
#18521=ORIENTED_EDGE ( 'NONE', *, *, #32773, .F. ) ;
#18522=AXIS2_PLACEMENT_3D ( 'NONE', #12531, #28537, #2874 ) ;
#18524=CARTESIAN_POINT ( 'NONE',  ( -77.00000337463097821, 43.30127018922197379, -5.000000000000000000 ) ) ;
#18525=FACE_OUTER_BOUND ( 'NONE', #4923, .T. ) ;
#18526=EDGE_LOOP ( 'NONE', ( #6537, #36552 ) ) ;
#18527=AXIS2_PLACEMENT_3D ( 'NONE', #4606, #12262, #18098 ) ;
#18528=DIRECTION ( 'NONE',  ( -0.000000000000000000, -0.000000000000000000, 1.000000000000000000 ) ) ;
#18531=EDGE_CURVE ( 'NONE', #10265, #6948, #30091, .T. ) ;
#18532=AXIS2_PLACEMENT_3D ( 'NONE', #29567, #15534, #29213 ) ;
#18533=CARTESIAN_POINT ( 'NONE',  ( 0.000000000000000000, 55.00000000000000000, -5.000000000000000000 ) ) ;
#18534=ORIENTED_EDGE ( 'NONE', *, *, #1848, .F. ) ;
#18535=VERTEX_POINT ( 'NONE', #36173 ) ;
#18536=CYLINDRICAL_SURFACE ( 'NONE', #21299, 1.999999999999998224 ) ;
#18537=AXIS2_PLACEMENT_3D ( 'NONE', #2206, #19452, #7458 ) ;
#18538=ADVANCED_FACE ( 'NONE', ( #15737 ), #15561, .T. ) ;
#18539=DIRECTION ( 'NONE',  ( 0.000000000000000000, 0.000000000000000000, 1.000000000000000000 ) ) ;
#18540=ORIENTED_EDGE ( 'NONE', *, *, #20513, .F. ) ;
#18541=VECTOR ( 'NONE', #11021, 1000.000000000000000 ) ;
#18544=DIRECTION ( 'NONE',  ( 0.000000000000000000, 0.000000000000000000, 1.000000000000000000 ) ) ;
#18545=CIRCLE ( 'NONE', #29907, 2.000000000000001776 ) ;
#18546=FACE_BOUND ( 'NONE', #32480, .T. ) ;
#18548=ORIENTED_EDGE ( 'NONE', *, *, #18683, .F. ) ;
#18549=VERTEX_POINT ( 'NONE', #15922 ) ;
#18550=AXIS2_PLACEMENT_3D ( 'NONE', #25659, #11008, #22652 ) ;
#18552=VERTEX_POINT ( 'NONE', #7124 ) ;
#18557=CARTESIAN_POINT ( 'NONE',  ( -75.00000337463097821, 25.98076211353318854, 17.49999999999999645 ) ) ;
#18558=ORIENTED_EDGE ( 'NONE', *, *, #21476, .F. ) ;
#18559=CARTESIAN_POINT ( 'NONE',  ( -18.00000337463123756, -86.60254037844400443, -9.999999999999998224 ) ) ;
#18561=EDGE_CURVE ( 'NONE', #15127, #24605, #153, .T. ) ;
#18564=ORIENTED_EDGE ( 'NONE', *, *, #10268, .F. ) ;
#18565=DIRECTION ( 'NONE',  ( 0.000000000000000000, 0.000000000000000000, 1.000000000000000000 ) ) ;
#18566=EDGE_CURVE ( 'NONE', #16909, #36669, #15751, .T. ) ;
#18568=DIRECTION ( 'NONE',  ( 1.000000000000000000, 0.000000000000000000, 0.000000000000000000 ) ) ;
#18569=ORIENTED_EDGE ( 'NONE', *, *, #3957, .T. ) ;
#18572=CARTESIAN_POINT ( 'NONE',  ( 74.99999662536836809, 25.98076211353319565, -9.999999999999998224 ) ) ;
#18573=EDGE_LOOP ( 'NONE', ( #30671, #11726, #30684, #35161 ) ) ;
#18574=CARTESIAN_POINT ( 'NONE',  ( 86.99999662536832545, 8.660254037844394404, -9.999999999999998224 ) ) ;
#18576=AXIS2_PLACEMENT_3D ( 'NONE', #5925, #17701, #17356 ) ;
#18577=DIRECTION ( 'NONE',  ( 1.000000000000000000, 0.000000000000000000, 0.000000000000000000 ) ) ;
#18578=CARTESIAN_POINT ( 'NONE',  ( 73.90204319670436917, -6.988578749851891203, -5.000000000000000000 ) ) ;
#18579=AXIS2_PLACEMENT_3D ( 'NONE', #20738, #17948, #29375 ) ;
#18580=CARTESIAN_POINT ( 'NONE',  ( 57.99999662536842493, -51.96152422706639840, -9.999999999999998224 ) ) ;
#18583=ORIENTED_EDGE ( 'NONE', *, *, #3572, .T. ) ;
#18584=DIRECTION ( 'NONE',  ( 0.000000000000000000, 0.000000000000000000, 1.000000000000000000 ) ) ;
#18585=EDGE_CURVE ( 'NONE', #20117, #32307, #29988, .T. ) ;
#18586=DIRECTION ( 'NONE',  ( 0.000000000000000000, 0.000000000000000000, 1.000000000000000000 ) ) ;
#18587=CARTESIAN_POINT ( 'NONE',  ( 32.50000000000065370, 56.29165124598813463, 12.49999999999999822 ) ) ;
#18588=CARTESIAN_POINT ( 'NONE',  ( -63.00000337463102085, 60.62177826491077326, -9.999999999999998224 ) ) ;
#18591=DIRECTION ( 'NONE',  ( 0.000000000000000000, 0.000000000000000000, 1.000000000000000000 ) ) ;
#18592=FACE_OUTER_BOUND ( 'NONE', #21580, .T. ) ;
#18593=ORIENTED_EDGE ( 'NONE', *, *, #37103, .T. ) ;
#18594=DIRECTION ( 'NONE',  ( 0.000000000000000000, 0.000000000000000000, 1.000000000000000000 ) ) ;
#18595=ORIENTED_EDGE ( 'NONE', *, *, #34645, .T. ) ;
#18596=LINE ( 'NONE', #24599, #4166 ) ;
#18597=DIRECTION ( 'NONE',  ( 0.000000000000000000, 0.000000000000000000, 1.000000000000000000 ) ) ;
#18598=EDGE_CURVE ( 'NONE', #8789, #29589, #17538, .T. ) ;
#18603=EDGE_CURVE ( 'NONE', #24524, #31695, #20523, .T. ) ;
#18604=ORIENTED_EDGE ( 'NONE', *, *, #19176, .F. ) ;
#18606=DIRECTION ( 'NONE',  ( 1.000000000000000000, 0.000000000000000000, 0.000000000000000000 ) ) ;
#18607=ADVANCED_FACE ( 'NONE', ( #11903 ), #8031, .T. ) ;
#18608=CARTESIAN_POINT ( 'NONE',  ( 72.99999662536835388, -25.98076211353319565, -9.999999999999998224 ) ) ;
#18609=CARTESIAN_POINT ( 'NONE',  ( 42.99999662536848888, 60.62177826491077326, -9.999999999999998224 ) ) ;
#18610=LINE ( 'NONE', #13160, #9945 ) ;
#18611=EDGE_CURVE ( 'NONE', #36868, #148, #660, .T. ) ;
#18612=ORIENTED_EDGE ( 'NONE', *, *, #35205, .T. ) ;
#18613=CARTESIAN_POINT ( 'NONE',  ( 76.71706219562632612, -9.685771384082254798, 12.50000000000000000 ) ) ;
#18614=LINE ( 'NONE', #32649, #7185 ) ;
#18615=CIRCLE ( 'NONE', #32978, 2.000000000000001776 ) ;
#18618=DIRECTION ( 'NONE',  ( 1.000000000000000000, 0.000000000000000000, 0.000000000000000000 ) ) ;
#18619=DIRECTION ( 'NONE',  ( 1.000000000000000000, 0.000000000000000000, 0.000000000000000000 ) ) ;
#18620=EDGE_CURVE ( 'NONE', #4001, #29187, #18149, .T. ) ;
#18621=EDGE_LOOP ( 'NONE', ( #27379, #36542 ) ) ;
#18622=EDGE_CURVE ( 'NONE', #550, #35128, #28101, .T. ) ;
#18624=EDGE_CURVE ( 'NONE', #7482, #32676, #17715, .T. ) ;
#18625=ADVANCED_FACE ( 'NONE', ( #5586 ), #25124, .F. ) ;
#18626=CARTESIAN_POINT ( 'NONE',  ( -35.00000337463116296, 77.94228634059957983, -9.999999999999998224 ) ) ;
#18627=DIRECTION ( 'NONE',  ( 1.000000000000000000, 0.000000000000000000, 0.000000000000000000 ) ) ;
#18628=FACE_OUTER_BOUND ( 'NONE', #2141, .T. ) ;
#18629=ORIENTED_EDGE ( 'NONE', *, *, #1561, .F. ) ;
#18631=EDGE_LOOP ( 'NONE', ( #14213, #5742 ) ) ;
#18632=DIRECTION ( 'NONE',  ( 0.000000000000000000, 0.000000000000000000, 1.000000000000000000 ) ) ;
#18634=ORIENTED_EDGE ( 'NONE', *, *, #28682, .F. ) ;
#18635=FACE_BOUND ( 'NONE', #27531, .T. ) ;
#18636=ORIENTED_EDGE ( 'NONE', *, *, #36830, .F. ) ;
#18637=VERTEX_POINT ( 'NONE', #11214 ) ;
#18638=FACE_OUTER_BOUND ( 'NONE', #24090, .T. ) ;
#18640=AXIS2_PLACEMENT_3D ( 'NONE', #26951, #12865, #12298 ) ;
#18641=ORIENTED_EDGE ( 'NONE', *, *, #578, .F. ) ;
#18643=DIRECTION ( 'NONE',  ( 0.000000000000000000, 0.000000000000000000, 1.000000000000000000 ) ) ;
#18644=DIRECTION ( 'NONE',  ( 1.000000000000000000, 0.000000000000000000, 0.000000000000000000 ) ) ;
#18645=DIRECTION ( 'NONE',  ( 0.000000000000000000, 0.000000000000000000, 1.000000000000000000 ) ) ;
#18646=CARTESIAN_POINT ( 'NONE',  ( -67.00000337463102085, 60.62177826491077326, -9.999999999999998224 ) ) ;
#18647=ORIENTED_EDGE ( 'NONE', *, *, #26331, .F. ) ;
#18648=DIRECTION ( 'NONE',  ( -1.000000000000000000, 0.000000000000000000, 0.000000000000000000 ) ) ;
#18649=ORIENTED_EDGE ( 'NONE', *, *, #16804, .F. ) ;
#18650=CARTESIAN_POINT ( 'NONE',  ( -50.00000337463112032, -51.96152422706641971, -9.999999999999998224 ) ) ;
#18652=DIRECTION ( 'NONE',  ( -0.000000000000000000, -0.000000000000000000, 1.000000000000000000 ) ) ;
#18653=DIRECTION ( 'NONE',  ( 0.000000000000000000, 0.000000000000000000, 1.000000000000000000 ) ) ;
#18654=CYLINDRICAL_SURFACE ( 'NONE', #18895, 1.999999999999998224 ) ;
#18655=CARTESIAN_POINT ( 'NONE',  ( 27.78182860042856461, 56.67878100130339902, 12.49999999999999822 ) ) ;
#18656=DIRECTION ( 'NONE',  ( 0.000000000000000000, 0.000000000000000000, 1.000000000000000000 ) ) ;
#18657=ORIENTED_EDGE ( 'NONE', *, *, #14885, .T. ) ;
#18658=CARTESIAN_POINT ( 'NONE',  ( 26.99999662536859546, -77.94228634059960825, -9.999999999999998224 ) ) ;
#18659=AXIS2_PLACEMENT_3D ( 'NONE', #14418, #8599, #5440 ) ;
#18660=CARTESIAN_POINT ( 'NONE',  ( -82.00000337463094979, 17.32050807568878525, -5.000000000000000000 ) ) ;
#18661=CARTESIAN_POINT ( 'NONE',  ( 69.99999662536838230, -51.96152422706639840, -9.999999999999998224 ) ) ;
#18662=ORIENTED_EDGE ( 'NONE', *, *, #34858, .F. ) ;
#18663=EDGE_LOOP ( 'NONE', ( #19428, #11917, #13076, #19248 ) ) ;
#18665=EDGE_CURVE ( 'NONE', #21723, #29824, #7962, .T. ) ;
#18666=LINE ( 'NONE', #16398, #6452 ) ;
#18667=CARTESIAN_POINT ( 'NONE',  ( 54.99999662536844625, 43.30127018922198801, -5.000000000000000000 ) ) ;
#18668=DIRECTION ( 'NONE',  ( 1.000000000000000000, 0.000000000000000000, 0.000000000000000000 ) ) ;
#18669=ORIENTED_EDGE ( 'NONE', *, *, #20113, .F. ) ;
#18670=DIRECTION ( 'NONE',  ( 0.000000000000000000, 0.000000000000000000, 1.000000000000000000 ) ) ;
#18671=CARTESIAN_POINT ( 'NONE',  ( 0.000000000000000000, 0.000000000000000000, 12.49999999999999822 ) ) ;
#18672=ORIENTED_EDGE ( 'NONE', *, *, #30354, .T. ) ;
#18673=DIRECTION ( 'NONE',  ( 0.000000000000000000, 0.000000000000000000, 1.000000000000000000 ) ) ;
#18675=FACE_BOUND ( 'NONE', #26541, .T. ) ;
#18678=VECTOR ( 'NONE', #3817, 1000.000000000000000 ) ;
#18679=CARTESIAN_POINT ( 'NONE',  ( 71.20511420343271425, 36.23716514913449060, -5.000000000000000000 ) ) ;
#18680=VERTEX_POINT ( 'NONE', #34973 ) ;
#18681=CARTESIAN_POINT ( 'NONE',  ( -15.97563234535668109, 90.60231327712331506, -49.86561046011506448 ) ) ;
#18683=EDGE_CURVE ( 'NONE', #13179, #8353, #28898, .T. ) ;
#18685=EDGE_CURVE ( 'NONE', #13703, #16037, #10855, .T. ) ;
#18689=DIRECTION ( 'NONE',  ( 0.000000000000000000, -0.000000000000000000, -1.000000000000000000 ) ) ;
#18690=ORIENTED_EDGE ( 'NONE', *, *, #17216, .T. ) ;
#18691=FACE_OUTER_BOUND ( 'NONE', #32580, .T. ) ;
#18693=CARTESIAN_POINT ( 'NONE',  ( -35.00000337463116296, 77.94228634059957983, -9.999999999999998224 ) ) ;
#18694=ADVANCED_FACE ( 'NONE', ( #36903 ), #31098, .F. ) ;
#18695=VERTEX_POINT ( 'NONE', #25670 ) ;
#18696=ORIENTED_EDGE ( 'NONE', *, *, #23416, .F. ) ;
#18697=DIRECTION ( 'NONE',  ( 0.000000000000000000, 0.000000000000000000, 1.000000000000000000 ) ) ;
#18698=DIRECTION ( 'NONE',  ( 1.000000000000000000, 0.000000000000000000, 0.000000000000000000 ) ) ;
#18699=DIRECTION ( 'NONE',  ( 3.469446951953612611E-15, 1.000000000000000000, 0.000000000000000000 ) ) ;
#18700=ORIENTED_EDGE ( 'NONE', *, *, #20381, .F. ) ;
#18702=EDGE_CURVE ( 'NONE', #27052, #27413, #3163, .T. ) ;
#18703=CARTESIAN_POINT ( 'NONE',  ( -3.499999999999987566, 55.00000000000000000, -10.00000000000000178 ) ) ;
#18705=DIRECTION ( 'NONE',  ( 0.000000000000000000, 0.000000000000000000, 1.000000000000000000 ) ) ;
#18706=DIRECTION ( 'NONE',  ( -1.000000000000000000, 0.000000000000000000, 0.000000000000000000 ) ) ;
#18708=ORIENTED_EDGE ( 'NONE', *, *, #13415, .T. ) ;
#18711=EDGE_LOOP ( 'NONE', ( #30616, #3898 ) ) ;
#18713=EDGE_LOOP ( 'NONE', ( #36920, #33623, #17992, #26360, #6400 ) ) ;
#18714=CARTESIAN_POINT ( 'NONE',  ( -50.00000337463110611, -69.28203230275519786, 17.49999999999999645 ) ) ;
#18715=AXIS2_PLACEMENT_3D ( 'NONE', #17636, #6594, #12175 ) ;
#18716=AXIS2_PLACEMENT_3D ( 'NONE', #17673, #28922, #21047 ) ;
#18718=ORIENTED_EDGE ( 'NONE', *, *, #33713, .F. ) ;
#18721=CARTESIAN_POINT ( 'NONE',  ( -38.00000337463113453, -69.28203230275519786, -5.000000000000000000 ) ) ;
#18722=ORIENTED_EDGE ( 'NONE', *, *, #11430, .F. ) ;
#18723=EDGE_CURVE ( 'NONE', #725, #21874, #27701, .T. ) ;
#18725=DIRECTION ( 'NONE',  ( 1.000000000000000000, 0.000000000000000000, 0.000000000000000000 ) ) ;
#18726=CIRCLE ( 'NONE', #6722, 2.000000000000001776 ) ;
#18727=DIRECTION ( 'NONE',  ( 0.000000000000000000, 0.000000000000000000, 1.000000000000000000 ) ) ;
#18728=CARTESIAN_POINT ( 'NONE',  ( 89.99999662536828282, 0.000000000000000000, -9.999999999999998224 ) ) ;
#18729=VERTEX_POINT ( 'NONE', #14214 ) ;
#18730=CYLINDRICAL_SURFACE ( 'NONE', #25082, 2.000000000000001776 ) ;
#18731=EDGE_CURVE ( 'NONE', #26888, #14326, #4376, .T. ) ;
#18732=DIRECTION ( 'NONE',  ( -0.000000000000000000, -0.000000000000000000, 1.000000000000000000 ) ) ;
#18733=ORIENTED_EDGE ( 'NONE', *, *, #7822, .F. ) ;
#18734=ORIENTED_EDGE ( 'NONE', *, *, #29385, .T. ) ;
#18735=EDGE_CURVE ( 'NONE', #5564, #25160, #12127, .T. ) ;
#18736=VERTEX_POINT ( 'NONE', #472 ) ;
#18737=CARTESIAN_POINT ( 'NONE',  ( 81.99999662536833966, 34.64101615137759183, -9.999999999999998224 ) ) ;
#18738=FACE_OUTER_BOUND ( 'NONE', #27902, .T. ) ;
#18739=ORIENTED_EDGE ( 'NONE', *, *, #30271, .F. ) ;
#18740=CARTESIAN_POINT ( 'NONE',  ( 0.000000000000000000, 0.000000000000000000, -5.000000000000000000 ) ) ;
#18741=DIRECTION ( 'NONE',  ( 1.000000000000000000, 0.000000000000000000, 0.000000000000000000 ) ) ;
#18742=VERTEX_POINT ( 'NONE', #8232 ) ;
#18743=DIRECTION ( 'NONE',  ( -0.000000000000000000, -0.000000000000000000, 1.000000000000000000 ) ) ;
#18747=LINE ( 'NONE', #30168, #5228 ) ;
#18748=CARTESIAN_POINT ( 'NONE',  ( -43.00000337463112743, -60.62177826491080168, 17.49999999999999645 ) ) ;
#18749=VERTEX_POINT ( 'NONE', #29698 ) ;
#18750=ORIENTED_EDGE ( 'NONE', *, *, #3690, .T. ) ;
#18751=EDGE_CURVE ( 'NONE', #4621, #8789, #772, .T. ) ;
#18752=DIRECTION ( 'NONE',  ( 0.000000000000000000, 0.000000000000000000, 1.000000000000000000 ) ) ;
#18753=AXIS2_PLACEMENT_3D ( 'NONE', #18740, #32804, #24368 ) ;
#18754=CARTESIAN_POINT ( 'NONE',  ( -53.00000337463110611, -43.30127018922202353, -9.999999999999998224 ) ) ;
#18755=PLANE ( 'NONE',  #11464 ) ;
#18756=LINE ( 'NONE', #10143, #19132 ) ;
#18757=ORIENTED_EDGE ( 'NONE', *, *, #17585, .T. ) ;
#18758=EDGE_CURVE ( 'NONE', #30786, #17343, #9749, .T. ) ;
#18759=DIRECTION ( 'NONE',  ( 0.000000000000000000, 0.000000000000000000, 1.000000000000000000 ) ) ;
#18764=CYLINDRICAL_SURFACE ( 'NONE', #427, 2.000000000000000000 ) ;
#18765=VECTOR ( 'NONE', #4194, 1000.000000000000000 ) ;
#18766=ORIENTED_EDGE ( 'NONE', *, *, #8439, .T. ) ;
#18768=DIRECTION ( 'NONE',  ( 1.000000000000000000, 0.000000000000000000, 0.000000000000000000 ) ) ;
#18769=AXIS2_PLACEMENT_3D ( 'NONE', #28116, #13480, #2438 ) ;
#18770=CARTESIAN_POINT ( 'NONE',  ( -68.00000337463099243, 17.32050807568877460, -9.999999999999998224 ) ) ;
#18771=CARTESIAN_POINT ( 'NONE',  ( -8.000003374631287301, 69.28203230275516944, -5.000000000000000000 ) ) ;
#18772=EDGE_LOOP ( 'NONE', ( #7211, #443, #24150, #21548 ) ) ;
#18773=ORIENTED_EDGE ( 'NONE', *, *, #27711, .F. ) ;
#18774=EDGE_CURVE ( 'NONE', #29875, #23027, #21741, .T. ) ;
#18775=VERTEX_POINT ( 'NONE', #30076 ) ;
#18777=AXIS2_PLACEMENT_3D ( 'NONE', #19221, #36642, #36271 ) ;
#18778=DIRECTION ( 'NONE',  ( 1.000000000000000000, 0.000000000000000000, 0.000000000000000000 ) ) ;
#18779=DIRECTION ( 'NONE',  ( 0.000000000000000000, 0.000000000000000000, 1.000000000000000000 ) ) ;
#18781=DIRECTION ( 'NONE',  ( 1.000000000000000000, 0.000000000000000000, 0.000000000000000000 ) ) ;
#18782=VERTEX_POINT ( 'NONE', #13016 ) ;
#18783=CIRCLE ( 'NONE', #2016, 1.999999999999998224 ) ;
#18784=CARTESIAN_POINT ( 'NONE',  ( 31.46585318596250502, 86.45172111230321832, -4.999999999999997335 ) ) ;
#18787=CARTESIAN_POINT ( 'NONE',  ( 2.999996625368645198, 77.94228634059957983, -9.999999999999998224 ) ) ;
#18788=EDGE_LOOP ( 'NONE', ( #8823, #14096, #33224, #20827 ) ) ;
#18790=CARTESIAN_POINT ( 'NONE',  ( -80.00000337463094979, -17.32050807568882078, -5.000000000000000000 ) ) ;
#18791=CYLINDRICAL_SURFACE ( 'NONE', #25539, 2.000000000000001776 ) ;
#18792=AXIS2_PLACEMENT_3D ( 'NONE', #33786, #10354, #27775 ) ;
#18793=VERTEX_POINT ( 'NONE', #4399 ) ;
#18794=CIRCLE ( 'NONE', #36168, 2.000000000000001776 ) ;
#18796=EDGE_CURVE ( 'NONE', #9227, #7555, #14542, .T. ) ;
#18797=DIRECTION ( 'NONE',  ( 1.000000000000000000, 0.000000000000000000, 0.000000000000000000 ) ) ;
#18798=DIRECTION ( 'NONE',  ( 0.000000000000000000, 0.000000000000000000, 1.000000000000000000 ) ) ;
#18801=ORIENTED_EDGE ( 'NONE', *, *, #12613, .F. ) ;
#18802=ORIENTED_EDGE ( 'NONE', *, *, #32137, .T. ) ;
#18803=VERTEX_POINT ( 'NONE', #29342 ) ;
#18804=AXIS2_PLACEMENT_3D ( 'NONE', #31336, #11469, #19743 ) ;
#18805=EDGE_CURVE ( 'NONE', #24065, #2400, #35513, .T. ) ;
#18806=DIRECTION ( 'NONE',  ( 0.000000000000000000, 0.000000000000000000, 1.000000000000000000 ) ) ;
#18807=ORIENTED_EDGE ( 'NONE', *, *, #16239, .F. ) ;
#18808=VERTEX_POINT ( 'NONE', #12813 ) ;
#18809=EDGE_CURVE ( 'NONE', #29585, #16050, #3773, .T. ) ;
#18810=CARTESIAN_POINT ( 'NONE',  ( 0.000000000000000000, -55.00000000000000000, -5.000000000000000000 ) ) ;
#18811=ORIENTED_EDGE ( 'NONE', *, *, #14570, .F. ) ;
#18812=EDGE_CURVE ( 'NONE', #8370, #21726, #5576, .T. ) ;
#18814=CARTESIAN_POINT ( 'NONE',  ( -63.00000337463102085, 60.62177826491077326, -9.999999999999998224 ) ) ;
#18815=CARTESIAN_POINT ( 'NONE',  ( 57.99999662536842493, -51.96152422706639840, -9.999999999999998224 ) ) ;
#18816=ORIENTED_EDGE ( 'NONE', *, *, #21897, .F. ) ;
#18817=EDGE_LOOP ( 'NONE', ( #11824, #27660 ) ) ;
#18818=LINE ( 'NONE', #6810, #26273 ) ;
#18821=CARTESIAN_POINT ( 'NONE',  ( 71.99999662536839651, -3.469446951953614189E-15, -5.000000000000000000 ) ) ;
#18824=CIRCLE ( 'NONE', #2644, 3.000000000000006217 ) ;
#18825=ADVANCED_FACE ( 'NONE', ( #20914 ), #7028, .F. ) ;
#18826=ORIENTED_EDGE ( 'NONE', *, *, #26122, .F. ) ;
#18827=DIRECTION ( 'NONE',  ( 1.000000000000000000, 0.000000000000000000, 0.000000000000000000 ) ) ;
#18828=VERTEX_POINT ( 'NONE', #6658 ) ;
#18829=CYLINDRICAL_SURFACE ( 'NONE', #4680, 2.000000000000001776 ) ;
#18832=DIRECTION ( 'NONE',  ( 0.000000000000000000, 0.000000000000000000, 1.000000000000000000 ) ) ;
#18833=CARTESIAN_POINT ( 'NONE',  ( 69.99999662536839651, -3.469446951953614189E-15, 17.49999999999999645 ) ) ;
#18836=DIRECTION ( 'NONE',  ( 0.000000000000000000, 0.000000000000000000, 1.000000000000000000 ) ) ;
#18837=AXIS2_PLACEMENT_3D ( 'NONE', #26436, #6372, #24008 ) ;
#18838=DIRECTION ( 'NONE',  ( 0.000000000000000000, 0.000000000000000000, 1.000000000000000000 ) ) ;
#18839=ORIENTED_EDGE ( 'NONE', *, *, #9501, .T. ) ;
#18841=DIRECTION ( 'NONE',  ( 0.000000000000000000, 0.000000000000000000, 1.000000000000000000 ) ) ;
#18842=DIRECTION ( 'NONE',  ( 1.000000000000000000, 0.000000000000000000, 0.000000000000000000 ) ) ;
#18844=ORIENTED_EDGE ( 'NONE', *, *, #26397, .T. ) ;
#18845=ORIENTED_EDGE ( 'NONE', *, *, #34655, .T. ) ;
#18846=DIRECTION ( 'NONE',  ( 1.000000000000000000, 0.000000000000000000, 0.000000000000000000 ) ) ;
#18847=DIRECTION ( 'NONE',  ( 0.000000000000000000, 0.000000000000000000, 1.000000000000000000 ) ) ;
#18848=AXIS2_PLACEMENT_3D ( 'NONE', #35264, #9914, #9558 ) ;
#18851=CARTESIAN_POINT ( 'NONE',  ( -68.00000337463100664, -17.32050807568882078, -9.999999999999998224 ) ) ;
#18852=FACE_OUTER_BOUND ( 'NONE', #34886, .T. ) ;
#18855=ORIENTED_EDGE ( 'NONE', *, *, #4326, .F. ) ;
#18856=FACE_BOUND ( 'NONE', #20227, .T. ) ;
#18857=AXIS2_PLACEMENT_3D ( 'NONE', #21902, #27339, #35433 ) ;
#18858=AXIS2_PLACEMENT_3D ( 'NONE', #718, #20413, #6160 ) ;
#18859=CARTESIAN_POINT ( 'NONE',  ( -87.00000337463093558, 8.660254037844389075, -9.999999999999998224 ) ) ;
#18860=DIRECTION ( 'NONE',  ( 0.000000000000000000, 0.000000000000000000, 1.000000000000000000 ) ) ;
#18861=VECTOR ( 'NONE', #13850, 1000.000000000000000 ) ;
#18862=VERTEX_POINT ( 'NONE', #15472 ) ;
#18864=DIRECTION ( 'NONE',  ( -0.000000000000000000, -0.000000000000000000, 1.000000000000000000 ) ) ;
#18865=EDGE_CURVE ( 'NONE', #12353, #5148, #26906, .T. ) ;
#18866=DIRECTION ( 'NONE',  ( 1.000000000000000000, 0.000000000000000000, 0.000000000000000000 ) ) ;
#18867=EDGE_CURVE ( 'NONE', #30363, #6764, #30632, .T. ) ;
#18868=PLANE ( 'NONE',  #6599 ) ;
#18869=CARTESIAN_POINT ( 'NONE',  ( 18.03952607653389961, -86.20686977408767859, 12.50000000000000000 ) ) ;
#18870=ADVANCED_FACE ( 'NONE', ( #13933 ), #19383, .F. ) ;
#18871=ORIENTED_EDGE ( 'NONE', *, *, #3985, .T. ) ;
#18872=LINE ( 'NONE', #30499, #15427 ) ;
#18874=CARTESIAN_POINT ( 'NONE',  ( 22.99999662536857059, 77.94228634059957983, -9.999999999999998224 ) ) ;
#18876=ORIENTED_EDGE ( 'NONE', *, *, #6849, .T. ) ;
#18877=ORIENTED_EDGE ( 'NONE', *, *, #36750, .T. ) ;
#18878=FACE_OUTER_BOUND ( 'NONE', #29370, .T. ) ;
#18880=AXIS2_PLACEMENT_3D ( 'NONE', #33549, #37089, #14199 ) ;
#18881=AXIS2_PLACEMENT_3D ( 'NONE', #10657, #30535, #10840 ) ;
#18882=CARTESIAN_POINT ( 'NONE',  ( 39.99999662536853151, -69.28203230275519786, -9.999999999999998224 ) ) ;
#18883=ORIENTED_EDGE ( 'NONE', *, *, #879, .F. ) ;
#18884=CARTESIAN_POINT ( 'NONE',  ( -88.00000337463090716, -1.040834085586084257E-14, 12.50000000000000000 ) ) ;
#18885=DIRECTION ( 'NONE',  ( 0.000000000000000000, 0.000000000000000000, -1.000000000000000000 ) ) ;
#18886=CARTESIAN_POINT ( 'NONE',  ( -50.00000337463112032, -51.96152422706641971, 12.50000000000000000 ) ) ;
#18887=LINE ( 'NONE', #10439, #17388 ) ;
#18888=EDGE_CURVE ( 'NONE', #23793, #11572, #12155, .T. ) ;
#18889=EDGE_LOOP ( 'NONE', ( #3752, #8030, #18117, #16176 ) ) ;
#18891=CYLINDRICAL_SURFACE ( 'NONE', #36280, 2.000000000000000000 ) ;
#18892=CIRCLE ( 'NONE', #15891, 2.000000000000001776 ) ;
#18893=DIRECTION ( 'NONE',  ( 1.000000000000000000, 0.000000000000000000, 0.000000000000000000 ) ) ;
#18895=AXIS2_PLACEMENT_3D ( 'NONE', #22015, #13208, #13567 ) ;
#18896=CARTESIAN_POINT ( 'NONE',  ( 62.33939050065184517, -13.89091430021398565, 12.49999999999999822 ) ) ;
#18897=ORIENTED_EDGE ( 'NONE', *, *, #5743, .T. ) ;
#18899=AXIS2_PLACEMENT_3D ( 'NONE', #24894, #36338, #18893 ) ;
#18900=AXIS2_PLACEMENT_3D ( 'NONE', #1032, #23169, #17718 ) ;
#18901=CIRCLE ( 'NONE', #12281, 2.000000000000001776 ) ;
#18902=CARTESIAN_POINT ( 'NONE',  ( -17.00000337463125533, -77.94228634059960825, 17.49999999999999645 ) ) ;
#18903=ORIENTED_EDGE ( 'NONE', *, *, #20734, .F. ) ;
#18904=DIRECTION ( 'NONE',  ( 1.000000000000000000, 0.000000000000000000, 0.000000000000000000 ) ) ;
#18905=VERTEX_POINT ( 'NONE', #22207 ) ;
#18906=VECTOR ( 'NONE', #1249, 1000.000000000000000 ) ;
#18908=CARTESIAN_POINT ( 'NONE',  ( 77.99999662536833966, -3.224517592124143893E-15, 12.50000000000000000 ) ) ;
#18909=DIRECTION ( 'NONE',  ( 0.000000000000000000, 0.000000000000000000, -1.000000000000000000 ) ) ;
#18910=LINE ( 'NONE', #10283, #28087 ) ;
#18911=EDGE_CURVE ( 'NONE', #21307, #12339, #16577, .T. ) ;
#18912=EDGE_LOOP ( 'NONE', ( #9978, #21496 ) ) ;
#18913=FACE_OUTER_BOUND ( 'NONE', #12580, .T. ) ;
#18915=DIRECTION ( 'NONE',  ( -1.000000000000000000, 0.000000000000000000, 0.000000000000000000 ) ) ;
#18916=EDGE_LOOP ( 'NONE', ( #9452, #18346, #8314, #36962 ) ) ;
#18918=ORIENTED_EDGE ( 'NONE', *, *, #33002, .T. ) ;
#18919=AXIS2_PLACEMENT_3D ( 'NONE', #3426, #21033, #20468 ) ;
#18920=CARTESIAN_POINT ( 'NONE',  ( 34.99999662536855283, -60.62177826491080168, 17.49999999999999645 ) ) ;
#18921=ORIENTED_EDGE ( 'NONE', *, *, #35261, .F. ) ;
#18923=CARTESIAN_POINT ( 'NONE',  ( 34.46585318596250858, 86.45172111230321832, 12.49999999999999822 ) ) ;
#18924=DIRECTION ( 'NONE',  ( 1.000000000000000000, 0.000000000000000000, 0.000000000000000000 ) ) ;
#18925=AXIS2_PLACEMENT_3D ( 'NONE', #12933, #4711, #10148 ) ;
#18926=AXIS2_PLACEMENT_3D ( 'NONE', #13377, #26909, #10387 ) ;
#18927=FACE_OUTER_BOUND ( 'NONE', #6754, .T. ) ;
#18928=AXIS2_PLACEMENT_3D ( 'NONE', #602, #15036, #23474 ) ;
#18929=EDGE_CURVE ( 'NONE', #16545, #20202, #30730, .T. ) ;
#18930=DIRECTION ( 'NONE',  ( 0.000000000000000000, 0.000000000000000000, 1.000000000000000000 ) ) ;
#18931=CARTESIAN_POINT ( 'NONE',  ( 32.99999662536855283, -77.94228634059960825, -5.000000000000000000 ) ) ;
#18932=DIRECTION ( 'NONE',  ( 0.000000000000000000, 0.000000000000000000, 1.000000000000000000 ) ) ;
#18933=CIRCLE ( 'NONE', #2763, 33.00000000000001421 ) ;
#18934=ADVANCED_FACE ( 'NONE', ( #2336 ), #7776, .F. ) ;
#18935=DIRECTION ( 'NONE',  ( 1.000000000000000000, 0.000000000000000000, 0.000000000000000000 ) ) ;
#18936=VERTEX_POINT ( 'NONE', #33646 ) ;
#18937=AXIS2_PLACEMENT_3D ( 'NONE', #4462, #4284, #10100 ) ;
#18938=EDGE_LOOP ( 'NONE', ( #8342, #29317 ) ) ;
#18940=CARTESIAN_POINT ( 'NONE',  ( 39.99999662536853151, -69.28203230275519786, 17.49999999999999645 ) ) ;
#18941=CARTESIAN_POINT ( 'NONE',  ( -10.00000337463128197, 86.60254037844397601, 12.50000000000000000 ) ) ;
#18943=EDGE_CURVE ( 'NONE', #31490, #14801, #2127, .T. ) ;
#18944=ORIENTED_EDGE ( 'NONE', *, *, #8934, .T. ) ;
#18946=AXIS2_PLACEMENT_3D ( 'NONE', #22805, #25611, #19611 ) ;
#18947=CARTESIAN_POINT ( 'NONE',  ( -70.00000337463100664, -17.32050807568882078, -9.999999999999998224 ) ) ;
#18948=DIRECTION ( 'NONE',  ( -0.000000000000000000, -0.000000000000000000, 1.000000000000000000 ) ) ;
#18949=EDGE_CURVE ( 'NONE', #16912, #17074, #34942, .T. ) ;
#18950=AXIS2_PLACEMENT_3D ( 'NONE', #34160, #2634, #3023 ) ;
#18952=EDGE_LOOP ( 'NONE', ( #17513, #25401, #1101, #25217 ) ) ;
#18955=EDGE_LOOP ( 'NONE', ( #1134, #1954 ) ) ;
#18956=AXIS2_PLACEMENT_3D ( 'NONE', #14129, #17137, #36652 ) ;
#18958=VECTOR ( 'NONE', #1822, 1000.000000000000000 ) ;
#18959=CARTESIAN_POINT ( 'NONE',  ( 87.83969979969883468, 14.80603122773026037, 12.49999999999999645 ) ) ;
#18960=AXIS2_PLACEMENT_3D ( 'NONE', #36774, #16530, #5638 ) ;
#18961=CARTESIAN_POINT ( 'NONE',  ( 69.99999662536839651, 34.64101615137758472, 12.50000000000000000 ) ) ;
#18962=AXIS2_PLACEMENT_3D ( 'NONE', #9087, #11525, #28783 ) ;
#18965=ORIENTED_EDGE ( 'NONE', *, *, #9805, .F. ) ;
#18966=VERTEX_POINT ( 'NONE', #24833 ) ;
#18967=CARTESIAN_POINT ( 'NONE',  ( -52.00000337463112032, -51.96152422706641971, -9.999999999999998224 ) ) ;
#18968=CIRCLE ( 'NONE', #16556, 2.000000000000001776 ) ;
#18969=ORIENTED_EDGE ( 'NONE', *, *, #34824, .F. ) ;
#18970=DIRECTION ( 'NONE',  ( 1.000000000000000000, 0.000000000000000000, 0.000000000000000000 ) ) ;
#18971=CARTESIAN_POINT ( 'NONE',  ( 79.99999662536833966, 34.64101615137759183, -9.999999999999998224 ) ) ;
#18972=CARTESIAN_POINT ( 'NONE',  ( -73.00000337463097821, -8.660254037844422825, 12.50000000000000000 ) ) ;
#18973=DIRECTION ( 'NONE',  ( -1.000000000000000000, 0.000000000000000000, -0.000000000000000000 ) ) ;
#18974=CYLINDRICAL_SURFACE ( 'NONE', #34522, 3.499999999999989342 ) ;
#18975=EDGE_LOOP ( 'NONE', ( #36423, #1859 ) ) ;
#18976=FACE_OUTER_BOUND ( 'NONE', #17968, .T. ) ;
#18977=AXIS2_PLACEMENT_3D ( 'NONE', #31348, #4939, #30998 ) ;
#18978=EDGE_CURVE ( 'NONE', #10304, #24755, #4784, .T. ) ;
#18979=DIRECTION ( 'NONE',  ( 0.000000000000000000, 0.000000000000000000, 1.000000000000000000 ) ) ;
#18982=ORIENTED_EDGE ( 'NONE', *, *, #31619, .T. ) ;
#18983=CARTESIAN_POINT ( 'NONE',  ( -80.00000337463094979, -2.428612866367529932E-14, -9.999999999999998224 ) ) ;
#18984=DIRECTION ( 'NONE',  ( 0.000000000000000000, 0.000000000000000000, 1.000000000000000000 ) ) ;
#18985=DIRECTION ( 'NONE',  ( 0.000000000000000000, 0.000000000000000000, 1.000000000000000000 ) ) ;
#18986=ORIENTED_EDGE ( 'NONE', *, *, #5453, .T. ) ;
#18987=EDGE_CURVE ( 'NONE', #12004, #17325, #6183, .T. ) ;
#18989=ORIENTED_EDGE ( 'NONE', *, *, #2094, .F. ) ;
#18991=CYLINDRICAL_SURFACE ( 'NONE', #35560, 2.000000000000001776 ) ;
#18993=EDGE_CURVE ( 'NONE', #26245, #26119, #33139, .T. ) ;
#18994=ORIENTED_EDGE ( 'NONE', *, *, #27203, .T. ) ;
#18995=VERTEX_POINT ( 'NONE', #33466 ) ;
#18996=ORIENTED_EDGE ( 'NONE', *, *, #24767, .F. ) ;
#18997=VECTOR ( 'NONE', #30010, 1000.000000000000000 ) ;
#18998=DIRECTION ( 'NONE',  ( 0.000000000000000000, 0.000000000000000000, 1.000000000000000000 ) ) ;
#18999=EDGE_CURVE ( 'NONE', #29382, #6775, #22356, .T. ) ;
#19000=EDGE_LOOP ( 'NONE', ( #3820, #18069 ) ) ;
#19001=AXIS2_PLACEMENT_3D ( 'NONE', #16975, #28233, #14162 ) ;
#19002=DIRECTION ( 'NONE',  ( 0.000000000000000000, 0.000000000000000000, -1.000000000000000000 ) ) ;
#19003=ORIENTED_EDGE ( 'NONE', *, *, #22172, .T. ) ;
#19005=VERTEX_POINT ( 'NONE', #31008 ) ;
#19006=CARTESIAN_POINT ( 'NONE',  ( -4.279621169095561228, 62.97617850287782915, -49.86561046011506448 ) ) ;
#19007=VECTOR ( 'NONE', #6483, 1000.000000000000000 ) ;
#19008=CARTESIAN_POINT ( 'NONE',  ( -43.00000337463111322, 77.94228634059959404, -9.999999999999998224 ) ) ;
#19010=ORIENTED_EDGE ( 'NONE', *, *, #26390, .T. ) ;
#19011=DIRECTION ( 'NONE',  ( -1.000000000000000000, 0.000000000000000000, 0.000000000000000000 ) ) ;
#19012=DIRECTION ( 'NONE',  ( 0.000000000000000000, 0.000000000000000000, 1.000000000000000000 ) ) ;
#19013=CARTESIAN_POINT ( 'NONE',  ( -70.00000337463099243, -2.428612866367529932E-14, -9.999999999999998224 ) ) ;
#19014=AXIS2_PLACEMENT_3D ( 'NONE', #19793, #5532, #16960 ) ;
#19015=CIRCLE ( 'NONE', #30375, 27.00000000000001421 ) ;
#19016=LINE ( 'NONE', #1761, #8477 ) ;
#19017=DIRECTION ( 'NONE',  ( 0.000000000000000000, 0.000000000000000000, 1.000000000000000000 ) ) ;
#19019=EDGE_LOOP ( 'NONE', ( #32982, #20515 ) ) ;
#19020=DIRECTION ( 'NONE',  ( 0.000000000000000000, 0.000000000000000000, 1.000000000000000000 ) ) ;
#19021=FACE_BOUND ( 'NONE', #1453, .T. ) ;
#19022=DIRECTION ( 'NONE',  ( 0.000000000000000000, 0.000000000000000000, 1.000000000000000000 ) ) ;
#19023=CYLINDRICAL_SURFACE ( 'NONE', #5231, 2.000000000000001776 ) ;
#19024=CIRCLE ( 'NONE', #30976, 27.00000000000001421 ) ;
#19025=CARTESIAN_POINT ( 'NONE',  ( 4.999996625368676284, -77.94228634059960825, -9.999999999999998224 ) ) ;
#19026=CYLINDRICAL_SURFACE ( 'NONE', #27845, 2.000000000000001776 ) ;
#19028=DIRECTION ( 'NONE',  ( -1.000000000000000000, 0.000000000000000000, 0.000000000000000000 ) ) ;
#19029=AXIS2_PLACEMENT_3D ( 'NONE', #30124, #30319, #1642 ) ;
#19030=EDGE_CURVE ( 'NONE', #7462, #9506, #29540, .T. ) ;
#19031=DIRECTION ( 'NONE',  ( 0.000000000000000000, 0.000000000000000000, 1.000000000000000000 ) ) ;
#19032=ORIENTED_EDGE ( 'NONE', *, *, #32885, .T. ) ;
#19034=EDGE_CURVE ( 'NONE', #357, #36483, #13383, .T. ) ;
#19035=CIRCLE ( 'NONE', #10060, 2.000000000000001776 ) ;
#19038=DIRECTION ( 'NONE',  ( 0.000000000000000000, 0.000000000000000000, 1.000000000000000000 ) ) ;
#19041=ORIENTED_EDGE ( 'NONE', *, *, #22493, .F. ) ;
#19042=ORIENTED_EDGE ( 'NONE', *, *, #34294, .T. ) ;
#19043=ORIENTED_EDGE ( 'NONE', *, *, #35816, .T. ) ;
#19044=AXIS2_PLACEMENT_3D ( 'NONE', #15424, #35320, #11854 ) ;
#19045=CARTESIAN_POINT ( 'NONE',  ( -67.00000337463106348, -60.62177826491083010, -9.999999999999998224 ) ) ;
#19046=FACE_OUTER_BOUND ( 'NONE', #35461, .T. ) ;
#19047=VERTEX_POINT ( 'NONE', #31358 ) ;
#19048=DIRECTION ( 'NONE',  ( -1.000000000000000000, 0.000000000000000000, 0.000000000000000000 ) ) ;
#19050=CARTESIAN_POINT ( 'NONE',  ( 80.69570903995992239, -15.44541228182033699, -5.000000000000000000 ) ) ;
#19051=VERTEX_POINT ( 'NONE', #3072 ) ;
#19053=EDGE_LOOP ( 'NONE', ( #12523, #13142, #5399, #14935 ) ) ;
#19054=FACE_BOUND ( 'NONE', #19589, .T. ) ;
#19056=CARTESIAN_POINT ( 'NONE',  ( -73.00000337463097821, -8.660254037844422825, 17.49999999999999645 ) ) ;
#19057=CARTESIAN_POINT ( 'NONE',  ( -43.00000337463111322, 60.62177826491077326, -9.999999999999998224 ) ) ;
#19058=AXIS2_PLACEMENT_3D ( 'NONE', #961, #35301, #20096 ) ;
#19060=ORIENTED_EDGE ( 'NONE', *, *, #26399, .T. ) ;
#19061=CARTESIAN_POINT ( 'NONE',  ( 17.99999662536861678, -69.28203230275519786, -9.999999999999998224 ) ) ;
#19062=CIRCLE ( 'NONE', #4088, 2.000000000000001776 ) ;
#19063=VECTOR ( 'NONE', #2586, 1000.000000000000000 ) ;
#19067=AXIS2_PLACEMENT_3D ( 'NONE', #26616, #9013, #26818 ) ;
#19068=ORIENTED_EDGE ( 'NONE', *, *, #13848, .T. ) ;
#19069=FACE_BOUND ( 'NONE', #28112, .T. ) ;
#19070=LINE ( 'NONE', #24688, #2384 ) ;
#19071=ORIENTED_EDGE ( 'NONE', *, *, #3960, .F. ) ;
#19072=EDGE_CURVE ( 'NONE', #5817, #5072, #13976, .T. ) ;
#19073=CYLINDRICAL_SURFACE ( 'NONE', #20790, 2.000000000000001776 ) ;
#19074=DIRECTION ( 'NONE',  ( 1.000000000000000000, 0.000000000000000000, 0.000000000000000000 ) ) ;
#19075=LINE ( 'NONE', #1985, #23153 ) ;
#19076=EDGE_CURVE ( 'NONE', #9332, #34006, #7406, .T. ) ;
#19077=AXIS2_PLACEMENT_3D ( 'NONE', #28656, #2796, #28828 ) ;
#19078=ORIENTED_EDGE ( 'NONE', *, *, #14576, .T. ) ;
#19079=VERTEX_POINT ( 'NONE', #26109 ) ;
#19080=EDGE_CURVE ( 'NONE', #27157, #31151, #18174, .T. ) ;
#19081=DIRECTION ( 'NONE',  ( 1.000000000000000000, 0.000000000000000000, 0.000000000000000000 ) ) ;
#19082=CIRCLE ( 'NONE', #34045, 2.000000000000001776 ) ;
#19083=CARTESIAN_POINT ( 'NONE',  ( -62.97617850287781494, -4.279621169095772615, -4.999999999999997335 ) ) ;
#19085=DIRECTION ( 'NONE',  ( 0.000000000000000000, 0.000000000000000000, 1.000000000000000000 ) ) ;
#19087=VERTEX_POINT ( 'NONE', #19771 ) ;
#19088=AXIS2_PLACEMENT_3D ( 'NONE', #9348, #26042, #14600 ) ;
#19089=CARTESIAN_POINT ( 'NONE',  ( 0.000000000000000000, 0.000000000000000000, -5.000000000000000000 ) ) ;
#19090=CARTESIAN_POINT ( 'NONE',  ( -67.00000337463104927, -25.98076211353322051, 12.50000000000000000 ) ) ;
#19091=AXIS2_PLACEMENT_3D ( 'NONE', #19882, #14612, #11983 ) ;
#19092=CARTESIAN_POINT ( 'NONE',  ( 67.99999662536838230, 17.32050807568879236, 17.49999999999999645 ) ) ;
#19094=EDGE_CURVE ( 'NONE', #33342, #22833, #16981, .T. ) ;
#19095=ORIENTED_EDGE ( 'NONE', *, *, #28255, .T. ) ;
#19097=EDGE_CURVE ( 'NONE', #19686, #21619, #3800, .T. ) ;
#19100=CIRCLE ( 'NONE', #28650, 2.000000000000001776 ) ;
#19101=EDGE_CURVE ( 'NONE', #21726, #8370, #7990, .T. ) ;
#19102=DIRECTION ( 'NONE',  ( -1.000000000000000000, 0.000000000000000000, 0.000000000000000000 ) ) ;
#19103=ORIENTED_EDGE ( 'NONE', *, *, #18238, .F. ) ;
#19107=LINE ( 'NONE', #19277, #12317 ) ;
#19110=DIRECTION ( 'NONE',  ( -1.000000000000000000, 0.000000000000000000, 0.000000000000000000 ) ) ;
#19111=DIRECTION ( 'NONE',  ( 0.000000000000000000, 0.000000000000000000, 1.000000000000000000 ) ) ;
#19112=ORIENTED_EDGE ( 'NONE', *, *, #12739, .F. ) ;
#19115=CIRCLE ( 'NONE', #16726, 3.000000000000004885 ) ;
#19116=DIRECTION ( 'NONE',  ( 1.000000000000000000, 0.000000000000000000, 0.000000000000000000 ) ) ;
#19117=DIRECTION ( 'NONE',  ( 0.000000000000000000, 0.000000000000000000, 1.000000000000000000 ) ) ;
#19118=ORIENTED_EDGE ( 'NONE', *, *, #21138, .F. ) ;
#19119=CARTESIAN_POINT ( 'NONE',  ( 0.000000000000000000, 0.000000000000000000, -5.000000000000000000 ) ) ;
#19120=AXIS2_PLACEMENT_3D ( 'NONE', #31431, #34996, #17551 ) ;
#19121=DIRECTION ( 'NONE',  ( 1.000000000000000000, 0.000000000000000000, 0.000000000000000000 ) ) ;
#19123=ORIENTED_EDGE ( 'NONE', *, *, #9576, .F. ) ;
#19124=EDGE_CURVE ( 'NONE', #13703, #23401, #14561, .T. ) ;
#19125=EDGE_LOOP ( 'NONE', ( #4861, #13024, #25977, #3738, #1378, #8699, #11498, #6913, #5297, #10714, #10305, #19071, #13845, #14984 ) ) ;
#19127=VECTOR ( 'NONE', #30817, 1000.000000000000000 ) ;
#19128=DIRECTION ( 'NONE',  ( 1.000000000000000000, 0.000000000000000000, 0.000000000000000000 ) ) ;
#19130=DIRECTION ( 'NONE',  ( -0.000000000000000000, -0.000000000000000000, -1.000000000000000000 ) ) ;
#19131=CARTESIAN_POINT ( 'NONE',  ( 47.99999662536846756, -69.28203230275519786, -9.999999999999998224 ) ) ;
#19132=VECTOR ( 'NONE', #33005, 1000.000000000000000 ) ;
#19133=CYLINDRICAL_SURFACE ( 'NONE', #35989, 1.999999999999998224 ) ;
#19134=VECTOR ( 'NONE', #2761, 1000.000000000000000 ) ;
#19140=LINE ( 'NONE', #30564, #26229 ) ;
#19141=ORIENTED_EDGE ( 'NONE', *, *, #3341, .F. ) ;
#19142=ORIENTED_EDGE ( 'NONE', *, *, #28274, .F. ) ;
#19143=CIRCLE ( 'NONE', #7756, 2.000000000000001776 ) ;
#19144=CARTESIAN_POINT ( 'NONE',  ( 52.39915983220795681, 35.19434990244919703, 12.49999999999999822 ) ) ;
#19145=EDGE_CURVE ( 'NONE', #20765, #12599, #803, .T. ) ;
#19146=DIRECTION ( 'NONE',  ( -1.000000000000000000, 0.000000000000000000, 0.000000000000000000 ) ) ;
#19147=FACE_OUTER_BOUND ( 'NONE', #9305, .T. ) ;
#19148=ORIENTED_EDGE ( 'NONE', *, *, #17858, .T. ) ;
#19150=DIRECTION ( 'NONE',  ( 0.000000000000000000, 0.000000000000000000, 1.000000000000000000 ) ) ;
#19153=CARTESIAN_POINT ( 'NONE',  ( -85.00000337463092137, -25.98076211353322051, -9.999999999999998224 ) ) ;
#19154=EDGE_LOOP ( 'NONE', ( #25897, #14683 ) ) ;
#19155=AXIS2_PLACEMENT_3D ( 'NONE', #17731, #35192, #23940 ) ;
#19156=DIRECTION ( 'NONE',  ( 1.000000000000000000, 0.000000000000000000, 0.000000000000000000 ) ) ;
#19158=CARTESIAN_POINT ( 'NONE',  ( 44.99999662536851019, 77.94228634059959404, -9.999999999999998224 ) ) ;
#19161=CIRCLE ( 'NONE', #10777, 2.000000000000001776 ) ;
#19163=ADVANCED_FACE ( 'NONE', ( #6227 ), #25769, .F. ) ;
#19164=ORIENTED_EDGE ( 'NONE', *, *, #9881, .F. ) ;
#19165=DIRECTION ( 'NONE',  ( 1.000000000000000000, 0.000000000000000000, 0.000000000000000000 ) ) ;
#19166=AXIS2_PLACEMENT_3D ( 'NONE', #21859, #4984, #36308 ) ;
#19167=CARTESIAN_POINT ( 'NONE',  ( 9.999996625368655856, -69.28203230275519786, -9.999999999999998224 ) ) ;
#19169=AXIS2_PLACEMENT_3D ( 'NONE', #21904, #4858, #36709 ) ;
#19170=CYLINDRICAL_SURFACE ( 'NONE', #13049, 2.000000000000000000 ) ;
#19171=DIRECTION ( 'NONE',  ( -1.000000000000000000, 0.000000000000000000, 0.000000000000000000 ) ) ;
#19172=CARTESIAN_POINT ( 'NONE',  ( 19.99999662536861678, -86.60254037844400443, 12.50000000000000000 ) ) ;
#19174=CARTESIAN_POINT ( 'NONE',  ( -43.00000337463111322, 77.94228634059959404, -9.999999999999998224 ) ) ;
#19175=DIRECTION ( 'NONE',  ( 1.000000000000000000, 0.000000000000000000, 0.000000000000000000 ) ) ;
#19176=EDGE_CURVE ( 'NONE', #17536, #18182, #36738, .T. ) ;
#19178=ORIENTED_EDGE ( 'NONE', *, *, #34671, .T. ) ;
#19179=DIRECTION ( 'NONE',  ( 1.000000000000000000, 0.000000000000000000, 0.000000000000000000 ) ) ;
#19181=AXIS2_PLACEMENT_3D ( 'NONE', #13393, #24110, #24851 ) ;
#19182=EDGE_LOOP ( 'NONE', ( #9872, #23941, #23226, #30892, #18377, #13215, #23783, #7887, #13319, #9793 ) ) ;
#19185=AXIS2_PLACEMENT_3D ( 'NONE', #14863, #20114, #3071 ) ;
#19186=EDGE_CURVE ( 'NONE', #29302, #3947, #17861, .T. ) ;
#19188=CARTESIAN_POINT ( 'NONE',  ( -75.00000337463097821, 8.660254037844374864, 12.50000000000000000 ) ) ;
#19189=ORIENTED_EDGE ( 'NONE', *, *, #29549, .F. ) ;
#19190=ORIENTED_EDGE ( 'NONE', *, *, #36558, .T. ) ;
#19192=CARTESIAN_POINT ( 'NONE',  ( 71.99999662536838230, -51.96152422706639840, -9.999999999999998224 ) ) ;
#19193=AXIS2_PLACEMENT_3D ( 'NONE', #23579, #32199, #26219 ) ;
#19194=ORIENTED_EDGE ( 'NONE', *, *, #6849, .F. ) ;
#19195=VECTOR ( 'NONE', #23952, 1000.000000000000000 ) ;
#19196=CARTESIAN_POINT ( 'NONE',  ( -22.00000337463124112, 69.28203230275516944, 12.50000000000000000 ) ) ;
#19199=CARTESIAN_POINT ( 'NONE',  ( -75.00000337463097821, 8.660254037844374864, -5.000000000000000000 ) ) ;
#19201=DIRECTION ( 'NONE',  ( 0.000000000000000000, 0.000000000000000000, 1.000000000000000000 ) ) ;
#19202=EDGE_LOOP ( 'NONE', ( #13661, #26207, #6318, #34933 ) ) ;
#19204=ORIENTED_EDGE ( 'NONE', *, *, #3904, .F. ) ;
#19205=CARTESIAN_POINT ( 'NONE',  ( -62.33939050065184517, 13.89091430021398565, 12.49999999999999822 ) ) ;
#19206=DIRECTION ( 'NONE',  ( 0.000000000000000000, 0.000000000000000000, 1.000000000000000000 ) ) ;
#19207=LINE ( 'NONE', #28180, #16879 ) ;
#19208=CYLINDRICAL_SURFACE ( 'NONE', #12489, 2.000000000000000000 ) ;
#19209=ORIENTED_EDGE ( 'NONE', *, *, #14247, .T. ) ;
#19210=CYLINDRICAL_SURFACE ( 'NONE', #27926, 2.000000000000001776 ) ;
#19212=FACE_BOUND ( 'NONE', #14167, .T. ) ;
#19213=EDGE_CURVE ( 'NONE', #18148, #33445, #36152, .T. ) ;
#19214=CARTESIAN_POINT ( 'NONE',  ( 66.99999662536841072, -25.98076211353320275, -9.999999999999998224 ) ) ;
#19215=CIRCLE ( 'NONE', #3544, 2.000000000000001776 ) ;
#19216=CARTESIAN_POINT ( 'NONE',  ( -10.21421600225141724, -84.61404523131187716, 12.50000000000000000 ) ) ;
#19217=DIRECTION ( 'NONE',  ( 0.000000000000000000, 0.000000000000000000, 1.000000000000000000 ) ) ;
#19218=DIRECTION ( 'NONE',  ( 0.000000000000000000, 0.000000000000000000, 1.000000000000000000 ) ) ;
#19220=ADVANCED_FACE ( 'NONE', ( #15422 ), #32290, .F. ) ;
#19221=CARTESIAN_POINT ( 'NONE',  ( 19.99999662536857770, 86.60254037844397601, 17.49999999999999645 ) ) ;
#19222=EDGE_LOOP ( 'NONE', ( #20838, #2523, #22520, #1211 ) ) ;
#19225=CARTESIAN_POINT ( 'NONE',  ( -37.00000337463117717, -77.94228634059963667, -9.999999999999998224 ) ) ;
#19227=VERTEX_POINT ( 'NONE', #26860 ) ;
#19228=ORIENTED_EDGE ( 'NONE', *, *, #23638, .T. ) ;
#19230=FACE_OUTER_BOUND ( 'NONE', #8871, .T. ) ;
#19231=ORIENTED_EDGE ( 'NONE', *, *, #4124, .T. ) ;
#19233=EDGE_CURVE ( 'NONE', #29485, #12226, #34924, .T. ) ;
#19234=DIRECTION ( 'NONE',  ( 1.000000000000000000, 0.000000000000000000, 0.000000000000000000 ) ) ;
#19235=ORIENTED_EDGE ( 'NONE', *, *, #28610, .T. ) ;
#19236=CARTESIAN_POINT ( 'NONE',  ( -23.00000337463121980, -77.94228634059963667, -9.999999999999998224 ) ) ;
#19237=ORIENTED_EDGE ( 'NONE', *, *, #6102, .F. ) ;
#19238=DIRECTION ( 'NONE',  ( 0.000000000000000000, 0.000000000000000000, 1.000000000000000000 ) ) ;
#19239=EDGE_CURVE ( 'NONE', #19877, #17193, #15775, .T. ) ;
#19241=CARTESIAN_POINT ( 'NONE',  ( 14.99999662536859901, 77.94228634059957983, -9.999999999999998224 ) ) ;
#19242=EDGE_CURVE ( 'NONE', #3733, #24428, #1176, .T. ) ;
#19243=EDGE_LOOP ( 'NONE', ( #21965, #8197 ) ) ;
#19246=DIRECTION ( 'NONE',  ( 0.000000000000000000, 0.000000000000000000, 1.000000000000000000 ) ) ;
#19247=CARTESIAN_POINT ( 'NONE',  ( 95.00000000000000000, 1.163414459189985643E-14, 17.49999999999999645 ) ) ;
#19248=ORIENTED_EDGE ( 'NONE', *, *, #18347, .F. ) ;
#19249=FACE_BOUND ( 'NONE', #32350, .T. ) ;
#19250=CARTESIAN_POINT ( 'NONE',  ( -14.80603122773057478, 87.83969979969877784, -4.999999999999997335 ) ) ;
#19251=ORIENTED_EDGE ( 'NONE', *, *, #14597, .T. ) ;
#19252=FACE_OUTER_BOUND ( 'NONE', #10193, .T. ) ;
#19253=CIRCLE ( 'NONE', #22242, 2.000000000000001776 ) ;
#19254=CARTESIAN_POINT ( 'NONE',  ( -31.83425564451526668, -89.42901512340343118, 12.49999999999999822 ) ) ;
#19255=CYLINDRICAL_SURFACE ( 'NONE', #21357, 2.000000000000001776 ) ;
#19256=ORIENTED_EDGE ( 'NONE', *, *, #25844, .F. ) ;
#19257=ADVANCED_FACE ( 'NONE', ( #32858 ), #12196, .F. ) ;
#19258=ORIENTED_EDGE ( 'NONE', *, *, #22238, .T. ) ;
#19259=CARTESIAN_POINT ( 'NONE',  ( -56.67878100130369035, 27.78182860042797131, -4.999999999999997335 ) ) ;
#19260=DIRECTION ( 'NONE',  ( 0.000000000000000000, 0.000000000000000000, 1.000000000000000000 ) ) ;
#19261=CARTESIAN_POINT ( 'NONE',  ( 51.13139720814417899, 27.49999999999988987, -10.00000000000000000 ) ) ;
#19262=ORIENTED_EDGE ( 'NONE', *, *, #15609, .F. ) ;
#19263=EDGE_LOOP ( 'NONE', ( #16295, #27704 ) ) ;
#19264=DIRECTION ( 'NONE',  ( 0.000000000000000000, 0.000000000000000000, 1.000000000000000000 ) ) ;
#19268=VERTEX_POINT ( 'NONE', #21215 ) ;
#19269=ORIENTED_EDGE ( 'NONE', *, *, #15628, .T. ) ;
#19270=EDGE_CURVE ( 'NONE', #14483, #34280, #9798, .T. ) ;
#19271=FACE_OUTER_BOUND ( 'NONE', #25316, .T. ) ;
#19272=ORIENTED_EDGE ( 'NONE', *, *, #4492, .F. ) ;
#19275=ORIENTED_EDGE ( 'NONE', *, *, #19742, .T. ) ;
#19277=CARTESIAN_POINT ( 'NONE',  ( 52.99999662536844625, 43.30127018922198801, -9.999999999999998224 ) ) ;
#19279=ADVANCED_FACE ( 'NONE', ( #1346 ), #18041, .T. ) ;
#19280=DIRECTION ( 'NONE',  ( -1.000000000000000000, 0.000000000000000000, 0.000000000000000000 ) ) ;
#19283=ORIENTED_EDGE ( 'NONE', *, *, #32427, .F. ) ;
#19286=DIRECTION ( 'NONE',  ( 1.000000000000000000, 0.000000000000000000, 0.000000000000000000 ) ) ;
#19287=DIRECTION ( 'NONE',  ( 0.000000000000000000, 0.000000000000000000, -1.000000000000000000 ) ) ;
#19288=DIRECTION ( 'NONE',  ( -1.000000000000000000, 0.000000000000000000, -0.000000000000000000 ) ) ;
#19289=ORIENTED_EDGE ( 'NONE', *, *, #28453, .F. ) ;
#19290=CARTESIAN_POINT ( 'NONE',  ( -58.00000337463107059, -34.64101615137762025, 17.49999999999999645 ) ) ;
#19291=CARTESIAN_POINT ( 'NONE',  ( 32.16008401677996886, 61.25926521283067672, -49.22241343995293761 ) ) ;
#19292=CARTESIAN_POINT ( 'NONE',  ( -52.00000337463110611, -69.28203230275519786, -9.999999999999998224 ) ) ;
#19293=EDGE_CURVE ( 'NONE', #25751, #12329, #21791, .T. ) ;
#19295=ORIENTED_EDGE ( 'NONE', *, *, #17177, .F. ) ;
#19296=ORIENTED_EDGE ( 'NONE', *, *, #6106, .T. ) ;
#19297=EDGE_CURVE ( 'NONE', #27785, #15953, #11002, .T. ) ;
#19298=CIRCLE ( 'NONE', #10902, 2.000000000000001776 ) ;
#19299=EDGE_CURVE ( 'NONE', #8413, #28397, #31938, .T. ) ;
#19301=ORIENTED_EDGE ( 'NONE', *, *, #36062, .T. ) ;
#19303=CARTESIAN_POINT ( 'NONE',  ( -86.45172111230354517, 31.46585318596159553, -4.999999999999997335 ) ) ;
#19304=DIRECTION ( 'NONE',  ( 1.000000000000000000, 0.000000000000000000, 0.000000000000000000 ) ) ;
#19305=DIRECTION ( 'NONE',  ( 0.000000000000000000, -0.000000000000000000, -1.000000000000000000 ) ) ;
#19306=LINE ( 'NONE', #5040, #15860 ) ;
#19307=DIRECTION ( 'NONE',  ( 1.000000000000000000, 0.000000000000000000, 0.000000000000000000 ) ) ;
#19309=DIRECTION ( 'NONE',  ( 1.000000000000000000, 0.000000000000000000, 0.000000000000000000 ) ) ;
#19311=ORIENTED_EDGE ( 'NONE', *, *, #10307, .T. ) ;
#19312=VERTEX_POINT ( 'NONE', #8088 ) ;
#19313=AXIS2_PLACEMENT_3D ( 'NONE', #18626, #10184, #18435 ) ;
#19314=DIRECTION ( 'NONE',  ( -1.000000000000000000, 0.000000000000000000, 0.000000000000000000 ) ) ;
#19315=CARTESIAN_POINT ( 'NONE',  ( 89.42901512340354486, -31.83425564451495404, 12.49999999999999822 ) ) ;
#19316=CARTESIAN_POINT ( 'NONE',  ( -80.00000337463094979, 34.64101615137757051, -9.999999999999998224 ) ) ;
#19317=CARTESIAN_POINT ( 'NONE',  ( 79.99999662536833966, -3.469446951953614189E-15, 17.49999999999999645 ) ) ;
#19318=ORIENTED_EDGE ( 'NONE', *, *, #36424, .F. ) ;
#19320=ORIENTED_EDGE ( 'NONE', *, *, #28610, .F. ) ;
#19322=CARTESIAN_POINT ( 'NONE',  ( -3.374631334790434423E-06, 69.28203230275516944, -9.999999999999998224 ) ) ;
#19323=EDGE_LOOP ( 'NONE', ( #32394, #10896, #20768, #27010 ) ) ;
#19325=CARTESIAN_POINT ( 'NONE',  ( -31.00000000000027356, -58.88972745734168512, -49.22241343995298024 ) ) ;
#19327=DIRECTION ( 'NONE',  ( -0.5000000000000112133, -0.8660254037844322683, 0.000000000000000000 ) ) ;
#19328=ORIENTED_EDGE ( 'NONE', *, *, #30434, .T. ) ;
#19329=ORIENTED_EDGE ( 'NONE', *, *, #734, .T. ) ;
#19331=AXIS2_PLACEMENT_3D ( 'NONE', #1876, #30001, #4503 ) ;
#19332=ORIENTED_EDGE ( 'NONE', *, *, #15768, .T. ) ;
#19333=LINE ( 'NONE', #25512, #32147 ) ;
#19334=EDGE_CURVE ( 'NONE', #34734, #4235, #30596, .T. ) ;
#19335=CARTESIAN_POINT ( 'NONE',  ( 79.99999662536832545, -17.32050807568879591, -5.000000000000000000 ) ) ;
#19336=DIRECTION ( 'NONE',  ( 0.000000000000000000, 0.000000000000000000, -1.000000000000000000 ) ) ;
#19338=CARTESIAN_POINT ( 'NONE',  ( -67.00000337463102085, 25.98076211353317433, -5.000000000000000000 ) ) ;
#19339=ORIENTED_EDGE ( 'NONE', *, *, #1588, .T. ) ;
#19341=DIRECTION ( 'NONE',  ( 0.000000000000000000, 0.000000000000000000, -1.000000000000000000 ) ) ;
#19343=PRESENTATION_STYLE_ASSIGNMENT (( #1730 ) ) ;
#19344=EDGE_LOOP ( 'NONE', ( #20173, #2903, #24204, #24815 ) ) ;
#19346=CARTESIAN_POINT ( 'NONE',  ( -58.00000337463108480, -51.96152422706641971, -9.999999999999998224 ) ) ;
#19349=CARTESIAN_POINT ( 'NONE',  ( 44.99999662536851019, 77.94228634059959404, -5.000000000000000000 ) ) ;
#19350=CARTESIAN_POINT ( 'NONE',  ( -93.36492675454779544, -17.14523346298311779, -49.86561046011506448 ) ) ;
#19354=ORIENTED_EDGE ( 'NONE', *, *, #18665, .T. ) ;
#19355=AXIS2_PLACEMENT_3D ( 'NONE', #11867, #11501, #2696 ) ;
#19356=ADVANCED_FACE ( 'NONE', ( #27765 ), #13332, .F. ) ;
#19357=FACE_BOUND ( 'NONE', #26894, .T. ) ;
#19358=VECTOR ( 'NONE', #27374, 1000.000000000000000 ) ;
#19359=EDGE_LOOP ( 'NONE', ( #6708, #35256 ) ) ;
#19360=LINE ( 'NONE', #11091, #8808 ) ;
#19361=ORIENTED_EDGE ( 'NONE', *, *, #32563, .T. ) ;
#19362=VERTEX_POINT ( 'NONE', #15785 ) ;
#19363=DIRECTION ( 'NONE',  ( -1.000000000000000000, 0.000000000000000000, 0.000000000000000000 ) ) ;
#19365=CARTESIAN_POINT ( 'NONE',  ( 49.99999662536846756, 69.28203230275516944, 17.49999999999999645 ) ) ;
#19366=EDGE_LOOP ( 'NONE', ( #12560, #34820, #33731, #28153 ) ) ;
#19367=ORIENTED_EDGE ( 'NONE', *, *, #33285, .T. ) ;
#19369=CARTESIAN_POINT ( 'NONE',  ( 44.99999662536851019, -60.62177826491080168, -9.999999999999998224 ) ) ;
#19371=DIRECTION ( 'NONE',  ( 0.000000000000000000, 0.000000000000000000, 1.000000000000000000 ) ) ;
#19373=CYLINDRICAL_SURFACE ( 'NONE', #1592, 2.000000000000001776 ) ;
#19374=ADVANCED_FACE ( 'NONE', ( #13164 ), #5087, .F. ) ;
#19375=FACE_BOUND ( 'NONE', #36076, .T. ) ;
#19376=DIRECTION ( 'NONE',  ( -1.000000000000000000, 0.000000000000000000, 0.000000000000000000 ) ) ;
#19377=AXIS2_PLACEMENT_3D ( 'NONE', #7358, #18798, #7917 ) ;
#19378=DIRECTION ( 'NONE',  ( 0.000000000000000000, 0.000000000000000000, 1.000000000000000000 ) ) ;
#19379=DIRECTION ( 'NONE',  ( 0.000000000000000000, 0.000000000000000000, 1.000000000000000000 ) ) ;
#19380=DIRECTION ( 'NONE',  ( 1.000000000000000000, 0.000000000000000000, 0.000000000000000000 ) ) ;
#19381=AXIS2_PLACEMENT_3D ( 'NONE', #19144, #4886, #31114 ) ;
#19382=DIRECTION ( 'NONE',  ( 0.000000000000000000, 0.000000000000000000, -1.000000000000000000 ) ) ;
#19383=CYLINDRICAL_SURFACE ( 'NONE', #31909, 2.000000000000001776 ) ;
#19384=ORIENTED_EDGE ( 'NONE', *, *, #12536, .F. ) ;
#19386=CARTESIAN_POINT ( 'NONE',  ( 26.99999662536856704, 77.94228634059957983, -5.000000000000000000 ) ) ;
#19387=DIRECTION ( 'NONE',  ( 1.000000000000000000, 0.000000000000000000, 0.000000000000000000 ) ) ;
#19388=MANIFOLD_SOLID_BREP ( 'M6 Clearance Hole1', #9999 ) ;
#19389=CIRCLE ( 'NONE', #4428, 2.000000000000001776 ) ;
#19390=ORIENTED_EDGE ( 'NONE', *, *, #21775, .T. ) ;
#19391=ORIENTED_EDGE ( 'NONE', *, *, #9193, .T. ) ;
#19392=EDGE_LOOP ( 'NONE', ( #23404, #35046, #21273, #30936 ) ) ;
#19393=CIRCLE ( 'NONE', #24178, 2.000000000000001776 ) ;
#19396=DIRECTION ( 'NONE',  ( 1.000000000000000000, 0.000000000000000000, 0.000000000000000000 ) ) ;
#19397=ORIENTED_EDGE ( 'NONE', *, *, #14255, .T. ) ;
#19398=ADVANCED_FACE ( 'NONE', ( #36601 ), #30207, .F. ) ;
#19400=DIRECTION ( 'NONE',  ( 0.000000000000000000, 0.000000000000000000, 1.000000000000000000 ) ) ;
#19401=VERTEX_POINT ( 'NONE', #28152 ) ;
#19403=EDGE_CURVE ( 'NONE', #4724, #15428, #33165, .T. ) ;
#19404=ORIENTED_EDGE ( 'NONE', *, *, #27768, .T. ) ;
#19405=CARTESIAN_POINT ( 'NONE',  ( -52.00000337463110611, -69.28203230275519786, 17.49999999999999645 ) ) ;
#19406=AXIS2_PLACEMENT_3D ( 'NONE', #21317, #15884, #7084 ) ;
#19408=DIRECTION ( 'NONE',  ( 1.000000000000000000, 0.000000000000000000, 0.000000000000000000 ) ) ;
#19409=DIRECTION ( 'NONE',  ( 0.000000000000000000, 0.000000000000000000, 1.000000000000000000 ) ) ;
#19413=CIRCLE ( 'NONE', #20000, 2.000000000000001776 ) ;
#19414=CARTESIAN_POINT ( 'NONE',  ( 62.99999662536841072, 25.98076211353318854, 12.50000000000000000 ) ) ;
#19415=DIRECTION ( 'NONE',  ( 0.000000000000000000, 0.000000000000000000, 1.000000000000000000 ) ) ;
#19416=EDGE_LOOP ( 'NONE', ( #5146, #20265, #665, #30726 ) ) ;
#19417=CIRCLE ( 'NONE', #18223, 2.000000000000001776 ) ;
#19418=DIRECTION ( 'NONE',  ( 0.000000000000000000, -0.000000000000000000, -1.000000000000000000 ) ) ;
#19419=DIRECTION ( 'NONE',  ( 0.000000000000000000, 0.000000000000000000, 1.000000000000000000 ) ) ;
#19420=EDGE_LOOP ( 'NONE', ( #26547, #23242 ) ) ;
#19421=EDGE_CURVE ( 'NONE', #28397, #8413, #5625, .T. ) ;
#19423=CARTESIAN_POINT ( 'NONE',  ( -60.00000337463104216, 34.64101615137757051, -9.999999999999998224 ) ) ;
#19424=CARTESIAN_POINT ( 'NONE',  ( 49.99999662536846756, 51.96152422706637708, -5.000000000000000000 ) ) ;
#19425=DIRECTION ( 'NONE',  ( 0.000000000000000000, 0.000000000000000000, 1.000000000000000000 ) ) ;
#19426=EDGE_CURVE ( 'NONE', #30126, #1094, #31367, .T. ) ;
#19427=ORIENTED_EDGE ( 'NONE', *, *, #6750, .T. ) ;
#19428=ORIENTED_EDGE ( 'NONE', *, *, #2468, .F. ) ;
#19431=FACE_OUTER_BOUND ( 'NONE', #33041, .T. ) ;
#19432=EDGE_CURVE ( 'NONE', #5777, #5185, #8287, .T. ) ;
#19433=CARTESIAN_POINT ( 'NONE',  ( 0.000000000000000000, 0.000000000000000000, 12.49999999999999822 ) ) ;
#19434=ORIENTED_EDGE ( 'NONE', *, *, #18401, .T. ) ;
#19436=ADVANCED_FACE ( 'NONE', ( #11610 ), #25720, .F. ) ;
#19437=DIRECTION ( 'NONE',  ( -1.000000000000000000, 0.000000000000000000, 0.000000000000000000 ) ) ;
#19439=LINE ( 'NONE', #16636, #24856 ) ;
#19440=ORIENTED_EDGE ( 'NONE', *, *, #24604, .T. ) ;
#19442=CIRCLE ( 'NONE', #32592, 2.000000000000001776 ) ;
#19443=ORIENTED_EDGE ( 'NONE', *, *, #2019, .F. ) ;
#19444=DIRECTION ( 'NONE',  ( -0.8660254037844379305, 0.5000000000000012212, 0.000000000000000000 ) ) ;
#19448=FACE_OUTER_BOUND ( 'NONE', #29865, .T. ) ;
#19449=VERTEX_POINT ( 'NONE', #19889 ) ;
#19450=FACE_BOUND ( 'NONE', #29667, .T. ) ;
#19451=EDGE_CURVE ( 'NONE', #8273, #21059, #22519, .T. ) ;
#19452=DIRECTION ( 'NONE',  ( 0.000000000000000000, 0.000000000000000000, 1.000000000000000000 ) ) ;
#19454=VECTOR ( 'NONE', #31485, 1000.000000000000000 ) ;
#19456=EDGE_LOOP ( 'NONE', ( #9063, #31035, #36026, #10326 ) ) ;
#19458=AXIS2_PLACEMENT_3D ( 'NONE', #21575, #30367, #21377 ) ;
#19460=CARTESIAN_POINT ( 'NONE',  ( 61.99999662536845335, 34.64101615137759893, -9.999999999999998224 ) ) ;
#19461=DIRECTION ( 'NONE',  ( 0.000000000000000000, 0.000000000000000000, 1.000000000000000000 ) ) ;
#19462=ORIENTED_EDGE ( 'NONE', *, *, #2218, .F. ) ;
#19463=DIRECTION ( 'NONE',  ( 0.000000000000000000, 0.000000000000000000, -1.000000000000000000 ) ) ;
#19464=CARTESIAN_POINT ( 'NONE',  ( 54.99999662536844625, 43.30127018922198801, 12.50000000000000000 ) ) ;
#19466=VERTEX_POINT ( 'NONE', #17444 ) ;
#19467=EDGE_CURVE ( 'NONE', #15920, #25343, #5017, .T. ) ;
#19468=ORIENTED_EDGE ( 'NONE', *, *, #29505, .F. ) ;
#19469=FACE_OUTER_BOUND ( 'NONE', #12238, .T. ) ;
#19470=EDGE_CURVE ( 'NONE', #11022, #4612, #35570, .T. ) ;
#19471=ORIENTED_EDGE ( 'NONE', *, *, #32604, .F. ) ;
#19472=CARTESIAN_POINT ( 'NONE',  ( 39.99999662536853151, -69.28203230275519786, -9.999999999999998224 ) ) ;
#19473=CARTESIAN_POINT ( 'NONE',  ( 4.999996625368645198, 77.94228634059957983, -9.999999999999998224 ) ) ;
#19474=EDGE_CURVE ( 'NONE', #31658, #12512, #19393, .T. ) ;
#19475=CARTESIAN_POINT ( 'NONE',  ( 54.99999662536844625, 60.62177826491077326, 17.49999999999999645 ) ) ;
#19476=CIRCLE ( 'NONE', #23083, 2.000000000000000000 ) ;
#19479=DIRECTION ( 'NONE',  ( 1.000000000000000000, 0.000000000000000000, 0.000000000000000000 ) ) ;
#19482=EDGE_CURVE ( 'NONE', #6351, #30934, #20594, .T. ) ;
#19484=CIRCLE ( 'NONE', #5731, 2.000000000000001776 ) ;
#19485=CARTESIAN_POINT ( 'NONE',  ( 0.000000000000000000, 0.000000000000000000, -5.000000000000000000 ) ) ;
#19487=VECTOR ( 'NONE', #6150, 1000.000000000000000 ) ;
#19488=ORIENTED_EDGE ( 'NONE', *, *, #6209, .F. ) ;
#19490=CARTESIAN_POINT ( 'NONE',  ( 68.00000000000000000, 0.000000000000000000, -4.999999999999997335 ) ) ;
#19492=CARTESIAN_POINT ( 'NONE',  ( -35.83991598322101879, -56.52018970185248037, 12.49999999999999645 ) ) ;
#19493=VERTEX_POINT ( 'NONE', #11446 ) ;
#19495=AXIS2_PLACEMENT_3D ( 'NONE', #35401, #15686, #24684 ) ;
#19496=CIRCLE ( 'NONE', #7529, 33.00000000000001421 ) ;
#19497=EDGE_CURVE ( 'NONE', #553, #2942, #19417, .T. ) ;
#19498=CARTESIAN_POINT ( 'NONE',  ( -45.00000337463111322, 60.62177826491077326, -9.999999999999998224 ) ) ;
#19499=VERTEX_POINT ( 'NONE', #34512 ) ;
#19500=VERTEX_POINT ( 'NONE', #31315 ) ;
#19502=ORIENTED_EDGE ( 'NONE', *, *, #6002, .F. ) ;
#19504=CARTESIAN_POINT ( 'NONE',  ( -22.00000337463124112, -86.60254037844400443, 12.50000000000000000 ) ) ;
#19506=AXIS2_PLACEMENT_3D ( 'NONE', #11848, #34921, #14860 ) ;
#19507=CARTESIAN_POINT ( 'NONE',  ( -55.00000337463107059, 60.62177826491078747, -5.000000000000000000 ) ) ;
#19510=CIRCLE ( 'NONE', #28487, 2.000000000000001776 ) ;
#19511=AXIS2_PLACEMENT_3D ( 'NONE', #13735, #2098, #10546 ) ;
#19512=EDGE_LOOP ( 'NONE', ( #34799, #22888 ) ) ;
#19513=AXIS2_PLACEMENT_3D ( 'NONE', #3676, #7236, #21282 ) ;
#19515=ORIENTED_EDGE ( 'NONE', *, *, #32370, .T. ) ;
#19516=EDGE_CURVE ( 'NONE', #28397, #23804, #8460, .T. ) ;
#19517=ORIENTED_EDGE ( 'NONE', *, *, #5772, .T. ) ;
#19518=CARTESIAN_POINT ( 'NONE',  ( 51.99999662536847467, 69.28203230275516944, 12.50000000000000000 ) ) ;
#19519=CARTESIAN_POINT ( 'NONE',  ( 62.99999662536839651, -43.30127018922199511, -9.999999999999998224 ) ) ;
#19521=DIRECTION ( 'NONE',  ( -1.000000000000000000, 0.000000000000000000, 0.000000000000000000 ) ) ;
#19522=DIRECTION ( 'NONE',  ( 0.000000000000000000, 0.000000000000000000, 1.000000000000000000 ) ) ;
#19523=CARTESIAN_POINT ( 'NONE',  ( 66.99999662536842493, 43.30127018922200222, -9.999999999999998224 ) ) ;
#19524=ORIENTED_EDGE ( 'NONE', *, *, #9519, .F. ) ;
#19525=DIRECTION ( 'NONE',  ( 1.000000000000000000, 0.000000000000000000, 0.000000000000000000 ) ) ;
#19528=CARTESIAN_POINT ( 'NONE',  ( -15.97563234535668109, 90.60231327712331506, -4.999999999999997335 ) ) ;
#19530=DIRECTION ( 'NONE',  ( 0.000000000000000000, 0.000000000000000000, 1.000000000000000000 ) ) ;
#19531=ADVANCED_FACE ( 'NONE', ( #20264 ), #14618, .F. ) ;
#19534=AXIS2_PLACEMENT_3D ( 'NONE', #33453, #1937, #10569 ) ;
#19538=CARTESIAN_POINT ( 'NONE',  ( -45.00000337463112743, -60.62177826491080168, -9.999999999999998224 ) ) ;
#19540=ORIENTED_EDGE ( 'NONE', *, *, #3390, .T. ) ;
#19541=ORIENTED_EDGE ( 'NONE', *, *, #25324, .T. ) ;
#19542=CIRCLE ( 'NONE', #8162, 95.00000000000000000 ) ;
#19543=CIRCLE ( 'NONE', #14123, 33.00000000000001421 ) ;
#19544=EDGE_CURVE ( 'NONE', #16100, #25705, #32596, .T. ) ;
#19545=CIRCLE ( 'NONE', #9356, 2.000000000000001776 ) ;
#19546=ADVANCED_FACE ( 'NONE', ( #26816 ), #744, .F. ) ;
#19547=DIRECTION ( 'NONE',  ( 0.000000000000000000, 0.000000000000000000, -1.000000000000000000 ) ) ;
#19548=CIRCLE ( 'NONE', #15960, 2.000000000000001776 ) ;
#19549=EDGE_CURVE ( 'NONE', #36258, #7482, #27188, .T. ) ;
#19550=EDGE_LOOP ( 'NONE', ( #19524, #7766 ) ) ;
#19551=EDGE_CURVE ( 'NONE', #15061, #13344, #25996, .T. ) ;
#19552=CARTESIAN_POINT ( 'NONE',  ( 64.99999662536839651, -43.30127018922199511, -9.999999999999998224 ) ) ;
#19553=ORIENTED_EDGE ( 'NONE', *, *, #3685, .F. ) ;
#19555=AXIS2_PLACEMENT_3D ( 'NONE', #8355, #19790, #31377 ) ;
#19556=CARTESIAN_POINT ( 'NONE',  ( 0.000000000000000000, 0.000000000000000000, -10.00000000000000000 ) ) ;
#19557=CYLINDRICAL_SURFACE ( 'NONE', #35225, 2.000000000000001776 ) ;
#19558=ORIENTED_EDGE ( 'NONE', *, *, #12053, .T. ) ;
#19560=DIRECTION ( 'NONE',  ( -0.8660254037844449249, -0.4999999999999888978, 0.000000000000000000 ) ) ;
#19561=FACE_OUTER_BOUND ( 'NONE', #18092, .T. ) ;
#19562=CIRCLE ( 'NONE', #32111, 2.000000000000001776 ) ;
#19563=DIRECTION ( 'NONE',  ( 0.000000000000000000, 0.000000000000000000, 1.000000000000000000 ) ) ;
#19564=FACE_OUTER_BOUND ( 'NONE', #6140, .T. ) ;
#19565=ORIENTED_EDGE ( 'NONE', *, *, #20634, .T. ) ;
#19566=CYLINDRICAL_SURFACE ( 'NONE', #18977, 2.000000000000001776 ) ;
#19567=FACE_BOUND ( 'NONE', #36117, .T. ) ;
#19569=CARTESIAN_POINT ( 'NONE',  ( 66.99999662536839651, 60.62177826491078747, -9.999999999999998224 ) ) ;
#19570=CARTESIAN_POINT ( 'NONE',  ( -27.00000337463120914, 77.94228634059957983, -9.999999999999998224 ) ) ;
#19571=CIRCLE ( 'NONE', #24959, 2.000000000000001776 ) ;
#19572=DIRECTION ( 'NONE',  ( 0.000000000000000000, 0.000000000000000000, 1.000000000000000000 ) ) ;
#19573=AXIS2_PLACEMENT_3D ( 'NONE', #13249, #10256, #21511 ) ;
#19574=EDGE_CURVE ( 'NONE', #36626, #19903, #6184, .T. ) ;
#19575=CARTESIAN_POINT ( 'NONE',  ( 0.000000000000000000, 0.000000000000000000, -5.000000000000000000 ) ) ;
#19577=DIRECTION ( 'NONE',  ( 1.000000000000000000, 0.000000000000000000, 0.000000000000000000 ) ) ;
#19578=DIRECTION ( 'NONE',  ( 3.469446951953612217E-15, 1.000000000000000000, 0.000000000000000000 ) ) ;
#19579=ORIENTED_EDGE ( 'NONE', *, *, #3584, .F. ) ;
#19580=CARTESIAN_POINT ( 'NONE',  ( 81.99999662536832545, -34.64101615137759183, -9.999999999999998224 ) ) ;
#19581=CARTESIAN_POINT ( 'NONE',  ( 90.60231327712337190, 15.97563234535636134, -4.999999999999997335 ) ) ;
#19582=CARTESIAN_POINT ( 'NONE',  ( 56.67878100130369035, -27.78182860042797131, 12.49999999999999822 ) ) ;
#19583=ORIENTED_EDGE ( 'NONE', *, *, #2508, .F. ) ;
#19584=AXIS2_PLACEMENT_3D ( 'NONE', #32264, #39, #11465 ) ;
#19585=ORIENTED_EDGE ( 'NONE', *, *, #12463, .F. ) ;
#19586=VERTEX_POINT ( 'NONE', #29044 ) ;
#19587=CARTESIAN_POINT ( 'NONE',  ( 19.99999662536858835, 69.28203230275516944, -5.000000000000000000 ) ) ;
#19588=DIRECTION ( 'NONE',  ( 1.000000000000000000, 0.000000000000000000, 0.000000000000000000 ) ) ;
#19589=EDGE_LOOP ( 'NONE', ( #27424, #9287 ) ) ;
#19590=CIRCLE ( 'NONE', #4035, 2.000000000000001776 ) ;
#19592=AXIS2_PLACEMENT_3D ( 'NONE', #29700, #32704, #3833 ) ;
#19593=VERTEX_POINT ( 'NONE', #9929 ) ;
#19596=DIRECTION ( 'NONE',  ( 1.000000000000000000, 0.000000000000000000, 0.000000000000000000 ) ) ;
#19597=EDGE_LOOP ( 'NONE', ( #15664, #6991, #29034, #33955, #8072, #21411 ) ) ;
#19598=LINE ( 'NONE', #17147, #34541 ) ;
#19599=ORIENTED_EDGE ( 'NONE', *, *, #16106, .T. ) ;
#19600=AXIS2_PLACEMENT_3D ( 'NONE', #3750, #21180, #12355 ) ;
#19601=AXIS2_PLACEMENT_3D ( 'NONE', #29892, #829, #26902 ) ;
#19604=ORIENTED_EDGE ( 'NONE', *, *, #3213, .F. ) ;
#19605=DIRECTION ( 'NONE',  ( -0.000000000000000000, -0.000000000000000000, 1.000000000000000000 ) ) ;
#19606=VECTOR ( 'NONE', #11938, 1000.000000000000000 ) ;
#19607=VECTOR ( 'NONE', #24760, 1000.000000000000000 ) ;
#19608=DIRECTION ( 'NONE',  ( 1.000000000000000000, 0.000000000000000000, 0.000000000000000000 ) ) ;
#19609=DIRECTION ( 'NONE',  ( 0.000000000000000000, 0.000000000000000000, -1.000000000000000000 ) ) ;
#19611=DIRECTION ( 'NONE',  ( 1.000000000000000000, 0.000000000000000000, 0.000000000000000000 ) ) ;
#19612=DIRECTION ( 'NONE',  ( 1.000000000000000000, 0.000000000000000000, 0.000000000000000000 ) ) ;
#19614=DIRECTION ( 'NONE',  ( 0.000000000000000000, 0.000000000000000000, 1.000000000000000000 ) ) ;
#19616=CARTESIAN_POINT ( 'NONE',  ( 81.99999662536833966, 17.32050807568879236, -9.999999999999998224 ) ) ;
#19619=CARTESIAN_POINT ( 'NONE',  ( -80.00000337463094979, 17.32050807568878525, -9.999999999999998224 ) ) ;
#19620=CIRCLE ( 'NONE', #14228, 2.000000000000001776 ) ;
#19621=ORIENTED_EDGE ( 'NONE', *, *, #7972, .T. ) ;
#19622=AXIS2_PLACEMENT_3D ( 'NONE', #9781, #12030, #29295 ) ;
#19623=ORIENTED_EDGE ( 'NONE', *, *, #24459, .T. ) ;
#19628=AXIS2_PLACEMENT_3D ( 'NONE', #19199, #15807, #4762 ) ;
#19630=VERTEX_POINT ( 'NONE', #21000 ) ;
#19631=ORIENTED_EDGE ( 'NONE', *, *, #7456, .F. ) ;
#19632=DIRECTION ( 'NONE',  ( 1.000000000000000000, 0.000000000000000000, 0.000000000000000000 ) ) ;
#19634=DIRECTION ( 'NONE',  ( 1.000000000000000000, 0.000000000000000000, 0.000000000000000000 ) ) ;
#19635=AXIS2_PLACEMENT_3D ( 'NONE', #20698, #29335, #35165 ) ;
#19637=ORIENTED_EDGE ( 'NONE', *, *, #12798, .F. ) ;
#19638=DIRECTION ( 'NONE',  ( 0.000000000000000000, 0.000000000000000000, 1.000000000000000000 ) ) ;
#19639=ORIENTED_EDGE ( 'NONE', *, *, #1913, .T. ) ;
#19640=EDGE_CURVE ( 'NONE', #30820, #7069, #34410, .T. ) ;
#19642=VERTEX_POINT ( 'NONE', #929 ) ;
#19645=FACE_BOUND ( 'NONE', #3239, .T. ) ;
#19649=ORIENTED_EDGE ( 'NONE', *, *, #35281, .F. ) ;
#19651=LINE ( 'NONE', #31083, #8092 ) ;
#19652=AXIS2_PLACEMENT_3D ( 'NONE', #8485, #2660, #13743 ) ;
#19653=DIRECTION ( 'NONE',  ( 1.000000000000000000, 0.000000000000000000, 0.000000000000000000 ) ) ;
#19655=EDGE_CURVE ( 'NONE', #17775, #10369, #31960, .T. ) ;
#19656=ORIENTED_EDGE ( 'NONE', *, *, #30205, .F. ) ;
#19657=DIRECTION ( 'NONE',  ( 1.000000000000000000, 0.000000000000000000, 0.000000000000000000 ) ) ;
#19658=DIRECTION ( 'NONE',  ( 0.000000000000000000, 0.000000000000000000, 1.000000000000000000 ) ) ;
#19661=ORIENTED_EDGE ( 'NONE', *, *, #347, .T. ) ;
#19662=ORIENTED_EDGE ( 'NONE', *, *, #25251, .T. ) ;
#19663=AXIS2_PLACEMENT_3D ( 'NONE', #16755, #22917, #34004 ) ;
#19664=EDGE_LOOP ( 'NONE', ( #33848, #18042 ) ) ;
#19665=ADVANCED_FACE ( 'NONE', ( #18176 ), #15182, .F. ) ;
#19667=CARTESIAN_POINT ( 'NONE',  ( -78.00000337463094979, 34.64101615137757051, -9.999999999999998224 ) ) ;
#19669=AXIS2_PLACEMENT_3D ( 'NONE', #36676, #22809, #8544 ) ;
#19671=ADVANCED_FACE ( 'NONE', ( #15569 ), #17812, .F. ) ;
#19672=VECTOR ( 'NONE', #31496, 1000.000000000000000 ) ;
#19673=FACE_OUTER_BOUND ( 'NONE', #31340, .T. ) ;
#19675=DIRECTION ( 'NONE',  ( 0.000000000000000000, 0.000000000000000000, -1.000000000000000000 ) ) ;
#19676=CARTESIAN_POINT ( 'NONE',  ( -72.00000337463100664, 34.64101615137758472, -9.999999999999998224 ) ) ;
#19677=CARTESIAN_POINT ( 'NONE',  ( -32.00000337463118427, 69.28203230275516944, 12.50000000000000000 ) ) ;
#19678=AXIS2_PLACEMENT_3D ( 'NONE', #26827, #3940, #32043 ) ;
#19679=ORIENTED_EDGE ( 'NONE', *, *, #5711, .F. ) ;
#19680=VERTEX_POINT ( 'NONE', #21177 ) ;
#19681=CIRCLE ( 'NONE', #23261, 2.000000000000001776 ) ;
#19682=DIRECTION ( 'NONE',  ( 1.000000000000000000, 0.000000000000000000, 0.000000000000000000 ) ) ;
#19683=DIRECTION ( 'NONE',  ( 0.000000000000000000, 0.000000000000000000, 1.000000000000000000 ) ) ;
#19684=DIRECTION ( 'NONE',  ( 0.000000000000000000, 0.000000000000000000, 1.000000000000000000 ) ) ;
#19685=DIRECTION ( 'NONE',  ( 1.000000000000000000, 0.000000000000000000, 0.000000000000000000 ) ) ;
#19686=VERTEX_POINT ( 'NONE', #32243 ) ;
#19688=FACE_BOUND ( 'NONE', #10814, .T. ) ;
#19689=AXIS2_PLACEMENT_3D ( 'NONE', #8264, #19698, #27942 ) ;
#19690=EDGE_LOOP ( 'NONE', ( #20322, #849, #4960, #31603 ) ) ;
#19691=ORIENTED_EDGE ( 'NONE', *, *, #31702, .F. ) ;
#19692=AXIS2_PLACEMENT_3D ( 'NONE', #13194, #10370, #21066 ) ;
#19693=CYLINDRICAL_SURFACE ( 'NONE', #9255, 2.000000000000000000 ) ;
#19695=DIRECTION ( 'NONE',  ( 0.000000000000000000, 0.000000000000000000, 1.000000000000000000 ) ) ;
#19696=EDGE_CURVE ( 'NONE', #26711, #25432, #36786, .T. ) ;
#19698=DIRECTION ( 'NONE',  ( -0.000000000000000000, -0.000000000000000000, 1.000000000000000000 ) ) ;
#19701=VERTEX_POINT ( 'NONE', #4493 ) ;
#19702=ORIENTED_EDGE ( 'NONE', *, *, #14686, .T. ) ;
#19705=ORIENTED_EDGE ( 'NONE', *, *, #25066, .T. ) ;
#19706=CIRCLE ( 'NONE', #33501, 2.000000000000001776 ) ;
#19707=ORIENTED_EDGE ( 'NONE', *, *, #29573, .T. ) ;
#19710=LINE ( 'NONE', #16341, #36405 ) ;
#19711=CARTESIAN_POINT ( 'NONE',  ( -48.49679504533954599, -67.96280346788670101, -5.000000000000000000 ) ) ;
#19713=ORIENTED_EDGE ( 'NONE', *, *, #7365, .T. ) ;
#19715=DIRECTION ( 'NONE',  ( -0.4999999999999980571, 0.8660254037844399289, 0.000000000000000000 ) ) ;
#19716=EDGE_CURVE ( 'NONE', #19466, #21436, #27913, .T. ) ;
#19717=VECTOR ( 'NONE', #35803, 1000.000000000000000 ) ;
#19718=DIRECTION ( 'NONE',  ( -1.000000000000000000, 0.000000000000000000, 0.000000000000000000 ) ) ;
#19719=ORIENTED_EDGE ( 'NONE', *, *, #5056, .F. ) ;
#19720=DIRECTION ( 'NONE',  ( 0.000000000000000000, 0.000000000000000000, 1.000000000000000000 ) ) ;
#19721=AXIS2_PLACEMENT_3D ( 'NONE', #547, #32222, #29226 ) ;
#19722=CYLINDRICAL_SURFACE ( 'NONE', #35126, 2.000000000000001776 ) ;
#19723=EDGE_LOOP ( 'NONE', ( #3316, #13375 ) ) ;
#19724=ORIENTED_EDGE ( 'NONE', *, *, #22971, .F. ) ;
#19725=DIRECTION ( 'NONE',  ( 0.000000000000000000, 0.000000000000000000, -1.000000000000000000 ) ) ;
#19726=CIRCLE ( 'NONE', #8359, 2.000000000000001776 ) ;
#19727=DIRECTION ( 'NONE',  ( -0.000000000000000000, -0.000000000000000000, 1.000000000000000000 ) ) ;
#19728=DIRECTION ( 'NONE',  ( -0.000000000000000000, -0.000000000000000000, 1.000000000000000000 ) ) ;
#19730=ORIENTED_EDGE ( 'NONE', *, *, #9624, .T. ) ;
#19731=VERTEX_POINT ( 'NONE', #32812 ) ;
#19732=AXIS2_PLACEMENT_3D ( 'NONE', #5751, #6497, #18288 ) ;
#19735=EDGE_CURVE ( 'NONE', #16685, #33148, #24933, .T. ) ;
#19736=EDGE_LOOP ( 'NONE', ( #10830, #9700, #14242, #36306, #31977, #17029 ) ) ;
#19737=AXIS2_PLACEMENT_3D ( 'NONE', #2125, #4947, #22767 ) ;
#19738=EDGE_CURVE ( 'NONE', #20714, #2553, #10480, .T. ) ;
#19739=CARTESIAN_POINT ( 'NONE',  ( 61.99999662536843914, -34.64101615137759893, -9.999999999999998224 ) ) ;
#19740=ORIENTED_EDGE ( 'NONE', *, *, #28412, .F. ) ;
#19742=EDGE_CURVE ( 'NONE', #16632, #19630, #29593, .T. ) ;
#19743=DIRECTION ( 'NONE',  ( 1.000000000000000000, 0.000000000000000000, 0.000000000000000000 ) ) ;
#19744=DIRECTION ( 'NONE',  ( 0.000000000000000000, 0.000000000000000000, 1.000000000000000000 ) ) ;
#19745=AXIS2_PLACEMENT_3D ( 'NONE', #3693, #32377, #4435 ) ;
#19746=CARTESIAN_POINT ( 'NONE',  ( -47.00000337463111322, 60.62177826491077326, -9.999999999999998224 ) ) ;
#19747=ORIENTED_EDGE ( 'NONE', *, *, #31094, .T. ) ;
#19748=ORIENTED_EDGE ( 'NONE', *, *, #21690, .T. ) ;
#19749=ADVANCED_FACE ( 'NONE', ( #7132 ), #4878, .T. ) ;
#19750=DIRECTION ( 'NONE',  ( 0.000000000000000000, 0.000000000000000000, 1.000000000000000000 ) ) ;
#19751=AXIS2_PLACEMENT_3D ( 'NONE', #25281, #14393, #31629 ) ;
#19752=CARTESIAN_POINT ( 'NONE',  ( -60.00000337463108480, -51.96152422706641971, -5.000000000000000000 ) ) ;
#19753=EDGE_CURVE ( 'NONE', #32313, #27517, #235, .T. ) ;
#19754=CARTESIAN_POINT ( 'NONE',  ( -90.00000337463090716, -1.040834085586084257E-14, -9.999999999999998224 ) ) ;
#19756=ORIENTED_EDGE ( 'NONE', *, *, #15171, .T. ) ;
#19758=FACE_BOUND ( 'NONE', #5972, .T. ) ;
#19760=DIRECTION ( 'NONE',  ( 0.000000000000000000, 0.000000000000000000, -1.000000000000000000 ) ) ;
#19763=EDGE_CURVE ( 'NONE', #21017, #35319, #15227, .T. ) ;
#19764=DIRECTION ( 'NONE',  ( -1.000000000000000000, 0.000000000000000000, -0.000000000000000000 ) ) ;
#19765=ADVANCED_FACE ( 'NONE', ( #21924 ), #33368, .F. ) ;
#19768=EDGE_CURVE ( 'NONE', #31156, #33801, #12206, .T. ) ;
#19771=CARTESIAN_POINT ( 'NONE',  ( 81.99999662536833966, 34.64101615137759183, 17.49999999999999645 ) ) ;
#19774=CARTESIAN_POINT ( 'NONE',  ( -78.00000337463094979, -17.32050807568882078, -9.999999999999998224 ) ) ;
#19775=CIRCLE ( 'NONE', #1806, 2.000000000000001776 ) ;
#19776=CARTESIAN_POINT ( 'NONE',  ( 1.999996625368665182, 69.28203230275516944, -5.000000000000000000 ) ) ;
#19779=ORIENTED_EDGE ( 'NONE', *, *, #13464, .F. ) ;
#19780=AXIS2_PLACEMENT_3D ( 'NONE', #17169, #22606, #28595 ) ;
#19781=FACE_OUTER_BOUND ( 'NONE', #9737, .T. ) ;
#19782=DIRECTION ( 'NONE',  ( 1.000000000000000000, 0.000000000000000000, 0.000000000000000000 ) ) ;
#19783=AXIS2_PLACEMENT_3D ( 'NONE', #3519, #14952, #12097 ) ;
#19784=ORIENTED_EDGE ( 'NONE', *, *, #22906, .F. ) ;
#19785=DIRECTION ( 'NONE',  ( 1.000000000000000000, 0.000000000000000000, 0.000000000000000000 ) ) ;
#19786=VERTEX_POINT ( 'NONE', #33567 ) ;
#19787=AXIS2_PLACEMENT_3D ( 'NONE', #31107, #16681, #5243 ) ;
#19789=VERTEX_POINT ( 'NONE', #25129 ) ;
#19790=DIRECTION ( 'NONE',  ( -0.000000000000000000, -0.000000000000000000, 1.000000000000000000 ) ) ;
#19791=VECTOR ( 'NONE', #10699, 1000.000000000000000 ) ;
#19793=CARTESIAN_POINT ( 'NONE',  ( 4.999996625368645198, 77.94228634059957983, -9.999999999999998224 ) ) ;
#19795=CIRCLE ( 'NONE', #29, 2.000000000000001776 ) ;
#19796=VERTEX_POINT ( 'NONE', #4695 ) ;
#19797=DIRECTION ( 'NONE',  ( 0.000000000000000000, 0.000000000000000000, 1.000000000000000000 ) ) ;
#19799=CARTESIAN_POINT ( 'NONE',  ( 93.55673653616000252, 16.49657687835711073, -5.000000000000000000 ) ) ;
#19800=CARTESIAN_POINT ( 'NONE',  ( -3.374631289687624047E-06, -69.28203230275519786, -5.000000000000000000 ) ) ;
#19801=ORIENTED_EDGE ( 'NONE', *, *, #23769, .F. ) ;
#19802=DIRECTION ( 'NONE',  ( 0.000000000000000000, 0.000000000000000000, 1.000000000000000000 ) ) ;
#19803=CARTESIAN_POINT ( 'NONE',  ( 61.99999662536843914, -34.64101615137759893, 12.50000000000000000 ) ) ;
#19804=ORIENTED_EDGE ( 'NONE', *, *, #12961, .F. ) ;
#19805=CARTESIAN_POINT ( 'NONE',  ( -75.00000337463097821, -8.660254037844422825, 17.49999999999999645 ) ) ;
#19807=CYLINDRICAL_SURFACE ( 'NONE', #32759, 2.000000000000001776 ) ;
#19808=CYLINDRICAL_SURFACE ( 'NONE', #26617, 2.000000000000001776 ) ;
#19810=EDGE_CURVE ( 'NONE', #18552, #875, #857, .T. ) ;
#19813=CARTESIAN_POINT ( 'NONE',  ( 19.13981058454793072, -60.93295298010985306, 12.49999999999999822 ) ) ;
#19814=ORIENTED_EDGE ( 'NONE', *, *, #34041, .T. ) ;
#19815=ORIENTED_EDGE ( 'NONE', *, *, #10808, .F. ) ;
#19819=CARTESIAN_POINT ( 'NONE',  ( -87.83969979969870678, -14.80603122773086966, -4.999999999999997335 ) ) ;
#19820=CARTESIAN_POINT ( 'NONE',  ( 27.78182860042856461, 56.67878100130339902, -4.999999999999997335 ) ) ;
#19821=EDGE_LOOP ( 'NONE', ( #10212, #31122 ) ) ;
#19822=EDGE_LOOP ( 'NONE', ( #30466, #25412, #4405, #2265 ) ) ;
#19824=CARTESIAN_POINT ( 'NONE',  ( -35.19434990244938888, 52.39915983220783602, -4.999999999999997335 ) ) ;
#19825=EDGE_LOOP ( 'NONE', ( #4918, #25551, #4629, #14494, #6518, #18438, #33583, #32692, #6915, #8582, #18177, #22742, #24883 ) ) ;
#19826=CARTESIAN_POINT ( 'NONE',  ( 79.99999662536832545, -34.64101615137759183, 12.50000000000000000 ) ) ;
#19828=FACE_BOUND ( 'NONE', #32317, .T. ) ;
#19830=EDGE_CURVE ( 'NONE', #22507, #23780, #31390, .T. ) ;
#19831=CARTESIAN_POINT ( 'NONE',  ( 19.99999662536857770, 86.60254037844397601, -9.999999999999998224 ) ) ;
#19832=ORIENTED_EDGE ( 'NONE', *, *, #11710, .F. ) ;
#19834=DIRECTION ( 'NONE',  ( 0.000000000000000000, 0.000000000000000000, 1.000000000000000000 ) ) ;
#19836=CARTESIAN_POINT ( 'NONE',  ( 44.99999662536851019, -60.62177826491080168, -9.999999999999998224 ) ) ;
#19837=FACE_OUTER_BOUND ( 'NONE', #34170, .T. ) ;
#19838=ORIENTED_EDGE ( 'NONE', *, *, #28077, .T. ) ;
#19839=CARTESIAN_POINT ( 'NONE',  ( -85.00000337463092137, -8.660254037844422825, 12.50000000000000000 ) ) ;
#19840=FACE_OUTER_BOUND ( 'NONE', #3850, .T. ) ;
#19844=EDGE_CURVE ( 'NONE', #27194, #24231, #24832, .T. ) ;
#19845=EDGE_LOOP ( 'NONE', ( #7002, #12511, #15736, #22030 ) ) ;
#19846=DIRECTION ( 'NONE',  ( -1.000000000000000000, 0.000000000000000000, 0.000000000000000000 ) ) ;
#19847=CARTESIAN_POINT ( 'NONE',  ( -18.00000337463123046, 86.60254037844397601, -9.999999999999998224 ) ) ;
#19848=CARTESIAN_POINT ( 'NONE',  ( -31.46585318596190106, -86.45172111230344569, 12.49999999999999822 ) ) ;
#19850=CYLINDRICAL_SURFACE ( 'NONE', #25674, 2.000000000000001776 ) ;
#19853=DIRECTION ( 'NONE',  ( 0.000000000000000000, 0.000000000000000000, 1.000000000000000000 ) ) ;
#19855=ORIENTED_EDGE ( 'NONE', *, *, #20570, .T. ) ;
#19857=CYLINDRICAL_SURFACE ( 'NONE', #13477, 2.000000000000001776 ) ;
#19858=EDGE_CURVE ( 'NONE', #1373, #210, #23019, .T. ) ;
#19859=DIRECTION ( 'NONE',  ( 1.000000000000000000, 0.000000000000000000, 0.000000000000000000 ) ) ;
#19860=CARTESIAN_POINT ( 'NONE',  ( 0.000000000000000000, -55.00000000000000000, -10.00000000000000178 ) ) ;
#19863=EDGE_CURVE ( 'NONE', #33445, #2400, #19306, .T. ) ;
#19864=DIRECTION ( 'NONE',  ( 1.000000000000000000, 0.000000000000000000, 0.000000000000000000 ) ) ;
#19865=ORIENTED_EDGE ( 'NONE', *, *, #15585, .T. ) ;
#19868=LINE ( 'NONE', #14244, #18221 ) ;
#19869=ORIENTED_EDGE ( 'NONE', *, *, #29017, .T. ) ;
#19870=CARTESIAN_POINT ( 'NONE',  ( 34.99999662536855283, 60.62177826491078747, 17.49999999999999645 ) ) ;
#19873=AXIS2_PLACEMENT_3D ( 'NONE', #16205, #10759, #22195 ) ;
#19876=ORIENTED_EDGE ( 'NONE', *, *, #18122, .F. ) ;
#19877=VERTEX_POINT ( 'NONE', #33738 ) ;
#19878=ORIENTED_EDGE ( 'NONE', *, *, #15320, .F. ) ;
#19882=CARTESIAN_POINT ( 'NONE',  ( -56.67878100130369035, 27.78182860042797131, -4.999999999999997335 ) ) ;
#19883=CARTESIAN_POINT ( 'NONE',  ( 89.99999662536828282, 0.000000000000000000, -9.999999999999998224 ) ) ;
#19885=EDGE_LOOP ( 'NONE', ( #8952, #7398, #27699, #36620 ) ) ;
#19886=CARTESIAN_POINT ( 'NONE',  ( 49.99999662536846756, -69.28203230275519786, -9.999999999999998224 ) ) ;
#19887=EDGE_CURVE ( 'NONE', #8683, #27052, #28651, .T. ) ;
#19888=DIRECTION ( 'NONE',  ( 0.000000000000000000, 0.000000000000000000, -1.000000000000000000 ) ) ;
#19889=CARTESIAN_POINT ( 'NONE',  ( 72.99999662536836809, 8.660254037844394404, -5.000000000000000000 ) ) ;
#19890=EDGE_LOOP ( 'NONE', ( #6899, #13633 ) ) ;
#19893=VERTEX_POINT ( 'NONE', #2792 ) ;
#19894=EDGE_CURVE ( 'NONE', #6948, #31042, #8421, .T. ) ;
#19895=ORIENTED_EDGE ( 'NONE', *, *, #28079, .T. ) ;
#19899=LINE ( 'NONE', #28513, #31848 ) ;
#19902=EDGE_LOOP ( 'NONE', ( #10531, #21057, #16048, #35543 ) ) ;
#19903=VERTEX_POINT ( 'NONE', #8037 ) ;
#19904=CARTESIAN_POINT ( 'NONE',  ( 82.99999662536831124, -8.660254037844397956, -9.999999999999998224 ) ) ;
#19905=CARTESIAN_POINT ( 'NONE',  ( 81.99999662536832545, -34.64101615137759183, -5.000000000000000000 ) ) ;
#19909=CARTESIAN_POINT ( 'NONE',  ( -80.00000337463094979, 17.32050807568878525, 12.50000000000000000 ) ) ;
#19913=ADVANCED_FACE ( 'NONE', ( #19673 ), #33920, .F. ) ;
#19914=CARTESIAN_POINT ( 'NONE',  ( 74.99999662536836809, 43.30127018922198801, -9.999999999999998224 ) ) ;
#19915=EDGE_LOOP ( 'NONE', ( #2279, #26691, #36872, #1352 ) ) ;
#19916=ORIENTED_EDGE ( 'NONE', *, *, #23921, .T. ) ;
#19917=DIRECTION ( 'NONE',  ( 1.000000000000000000, -0.000000000000000000, 0.000000000000000000 ) ) ;
#19918=LINE ( 'NONE', #22920, #4615 ) ;
#19919=CARTESIAN_POINT ( 'NONE',  ( -80.00000337463096400, -34.64101615137762025, 17.49999999999999645 ) ) ;
#19920=DIRECTION ( 'NONE',  ( 1.000000000000000000, 0.000000000000000000, 0.000000000000000000 ) ) ;
#19921=ORIENTED_EDGE ( 'NONE', *, *, #29791, .F. ) ;
#19922=CARTESIAN_POINT ( 'NONE',  ( 31.27962116909601420, -62.97617850287780072, 12.49999999999999822 ) ) ;
#19924=FACE_BOUND ( 'NONE', #10925, .T. ) ;
#19925=AXIS2_PLACEMENT_3D ( 'NONE', #2894, #22570, #34217 ) ;
#19926=LINE ( 'NONE', #26103, #10061 ) ;
#19927=CARTESIAN_POINT ( 'NONE',  ( -3.499999999999991562, 55.00000000000000000, -10.00000000000000000 ) ) ;
#19929=CARTESIAN_POINT ( 'NONE',  ( -65.00000337463102085, 25.98076211353317433, -9.999999999999998224 ) ) ;
#19930=EDGE_CURVE ( 'NONE', #10704, #24005, #7402, .T. ) ;
#19931=DIRECTION ( 'NONE',  ( 0.000000000000000000, 0.000000000000000000, 1.000000000000000000 ) ) ;
#19932=CARTESIAN_POINT ( 'NONE',  ( -60.00000337463108480, -51.96152422706641971, -9.999999999999998224 ) ) ;
#19933=ORIENTED_EDGE ( 'NONE', *, *, #28206, .F. ) ;
#19935=LINE ( 'NONE', #2514, #4066 ) ;
#19936=CARTESIAN_POINT ( 'NONE',  ( 35.19434990244975126, -52.39915983220758022, 12.49999999999999822 ) ) ;
#19939=EDGE_CURVE ( 'NONE', #4318, #10468, #9852, .T. ) ;
#19940=AXIS2_PLACEMENT_3D ( 'NONE', #9018, #577, #23074 ) ;
#19941=VERTEX_POINT ( 'NONE', #11221 ) ;
#19942=EDGE_LOOP ( 'NONE', ( #28136, #23052, #3647, #11447, #667 ) ) ;
#19943=DIRECTION ( 'NONE',  ( 1.000000000000000000, 0.000000000000000000, 0.000000000000000000 ) ) ;
#19946=CARTESIAN_POINT ( 'NONE',  ( -3.000003374631269981, -77.94228634059960825, -9.999999999999998224 ) ) ;
#19947=ORIENTED_EDGE ( 'NONE', *, *, #28390, .T. ) ;
#19948=EDGE_CURVE ( 'NONE', #22555, #21363, #5069, .T. ) ;
#19949=DIRECTION ( 'NONE',  ( 1.000000000000000000, 0.000000000000000000, 0.000000000000000000 ) ) ;
#19950=VECTOR ( 'NONE', #10579, 1000.000000000000000 ) ;
#19951=ORIENTED_EDGE ( 'NONE', *, *, #13061, .F. ) ;
#19952=CARTESIAN_POINT ( 'NONE',  ( -3.108944973436880588, -78.59336093177338967, -5.000000000000000000 ) ) ;
#19953=ORIENTED_EDGE ( 'NONE', *, *, #30397, .F. ) ;
#19954=DIRECTION ( 'NONE',  ( 0.000000000000000000, 0.000000000000000000, 1.000000000000000000 ) ) ;
#19955=EDGE_LOOP ( 'NONE', ( #30633, #17848 ) ) ;
#19957=VERTEX_POINT ( 'NONE', #31270 ) ;
#19958=EDGE_CURVE ( 'NONE', #14414, #34086, #4404, .T. ) ;
#19959=FACE_OUTER_BOUND ( 'NONE', #36681, .T. ) ;
#19960=DIRECTION ( 'NONE',  ( 0.000000000000000000, 0.000000000000000000, -1.000000000000000000 ) ) ;
#19962=EDGE_CURVE ( 'NONE', #34330, #28343, #20542, .T. ) ;
#19963=EDGE_LOOP ( 'NONE', ( #36099, #10516, #9557, #30918 ) ) ;
#19964=CARTESIAN_POINT ( 'NONE',  ( -85.00000337463092137, 8.660254037844389075, -9.999999999999998224 ) ) ;
#19967=DIRECTION ( 'NONE',  ( 1.000000000000000000, 0.000000000000000000, 0.000000000000000000 ) ) ;
#19968=DIRECTION ( 'NONE',  ( 1.000000000000000000, 0.000000000000000000, 0.000000000000000000 ) ) ;
#19969=VECTOR ( 'NONE', #23585, 1000.000000000000000 ) ;
#19970=ORIENTED_EDGE ( 'NONE', *, *, #30968, .F. ) ;
#19971=FACE_OUTER_BOUND ( 'NONE', #24098, .T. ) ;
#19973=ORIENTED_EDGE ( 'NONE', *, *, #3508, .T. ) ;
#19974=CARTESIAN_POINT ( 'NONE',  ( -8.000003374631249997, -86.60254037844400443, 12.50000000000000000 ) ) ;
#19977=CARTESIAN_POINT ( 'NONE',  ( -70.00000337463102085, -51.96152422706641971, -9.999999999999998224 ) ) ;
#19978=AXIS2_PLACEMENT_3D ( 'NONE', #3056, #27659, #31175 ) ;
#19979=EDGE_CURVE ( 'NONE', #17608, #24795, #7978, .T. ) ;
#19980=ORIENTED_EDGE ( 'NONE', *, *, #826, .F. ) ;
#19981=AXIS2_PLACEMENT_3D ( 'NONE', #21039, #26662, #23486 ) ;
#19983=CARTESIAN_POINT ( 'NONE',  ( -30.00000337463118427, 69.28203230275516944, 12.50000000000000000 ) ) ;
#19984=DIRECTION ( 'NONE',  ( 1.000000000000000000, 0.000000000000000000, 0.000000000000000000 ) ) ;
#19985=AXIS2_PLACEMENT_3D ( 'NONE', #13979, #35962, #4831 ) ;
#19986=ORIENTED_EDGE ( 'NONE', *, *, #1353, .T. ) ;
#19987=ORIENTED_EDGE ( 'NONE', *, *, #21330, .F. ) ;
#19988=LINE ( 'NONE', #25088, #15197 ) ;
#19989=DIRECTION ( 'NONE',  ( 0.000000000000000000, 0.000000000000000000, 1.000000000000000000 ) ) ;
#19991=CARTESIAN_POINT ( 'NONE',  ( 42.99999662536850309, 77.94228634059959404, -9.999999999999998224 ) ) ;
#19992=EDGE_LOOP ( 'NONE', ( #35361, #25223, #36577, #8395 ) ) ;
#19993=ORIENTED_EDGE ( 'NONE', *, *, #28855, .F. ) ;
#19994=CIRCLE ( 'NONE', #33156, 33.00000000000001421 ) ;
#19995=DIRECTION ( 'NONE',  ( 0.000000000000000000, 0.000000000000000000, 1.000000000000000000 ) ) ;
#19996=EDGE_LOOP ( 'NONE', ( #19621, #5456 ) ) ;
#19997=PLANE ( 'NONE',  #32899 ) ;
#19998=ORIENTED_EDGE ( 'NONE', *, *, #8744, .T. ) ;
#19999=FACE_BOUND ( 'NONE', #3419, .T. ) ;
#20000=AXIS2_PLACEMENT_3D ( 'NONE', #14428, #30746, #34143 ) ;
#20001=ADVANCED_FACE ( 'NONE', ( #24506 ), #7426, .F. ) ;
#20004=EDGE_CURVE ( 'NONE', #13186, #12570, #25358, .T. ) ;
#20005=DIRECTION ( 'NONE',  ( 0.000000000000000000, 0.000000000000000000, 1.000000000000000000 ) ) ;
#20006=EDGE_LOOP ( 'NONE', ( #31597, #11969, #3549, #14758, #21663, #18877, #31685, #33049, #19639, #22416, #6969, #30997, #12985, #7329, #18989, #23742 ) ) ;
#20009=DIRECTION ( 'NONE',  ( 0.000000000000000000, 0.000000000000000000, 1.000000000000000000 ) ) ;
#20010=LINE ( 'NONE', #11744, #1165 ) ;
#20011=EDGE_LOOP ( 'NONE', ( #4970, #7593, #20641, #23811 ) ) ;
#20012=DIRECTION ( 'NONE',  ( -0.000000000000000000, 0.000000000000000000, -1.000000000000000000 ) ) ;
#20013=CARTESIAN_POINT ( 'NONE',  ( -3.374631303565411855E-06, -86.60254037844400443, -9.999999999999998224 ) ) ;
#20014=DIRECTION ( 'NONE',  ( -1.000000000000000000, 0.000000000000000000, 0.000000000000000000 ) ) ;
#20016=AXIS2_PLACEMENT_3D ( 'NONE', #20924, #12256, #28963 ) ;
#20017=VERTEX_POINT ( 'NONE', #33673 ) ;
#20018=ORIENTED_EDGE ( 'NONE', *, *, #33017, .F. ) ;
#20019=ADVANCED_FACE ( 'NONE', ( #33105 ), #4625, .F. ) ;
#20020=CARTESIAN_POINT ( 'NONE',  ( -75.00000337463100664, -43.30127018922202353, -9.999999999999998224 ) ) ;
#20021=VECTOR ( 'NONE', #1482, 1000.000000000000000 ) ;
#20023=DIRECTION ( 'NONE',  ( 1.000000000000000000, 0.000000000000000000, 0.000000000000000000 ) ) ;
#20024=PLANE ( 'NONE',  #23088 ) ;
#20025=DIRECTION ( 'NONE',  ( -0.000000000000000000, -0.000000000000000000, 1.000000000000000000 ) ) ;
#20026=CARTESIAN_POINT ( 'NONE',  ( 7.999996625368625658, 86.60254037844397601, -5.000000000000000000 ) ) ;
#20028=ORIENTED_EDGE ( 'NONE', *, *, #25645, .T. ) ;
#20029=CYLINDRICAL_SURFACE ( 'NONE', #15875, 2.000000000000001776 ) ;
#20030=AXIS2_PLACEMENT_3D ( 'NONE', #4735, #15974, #15418 ) ;
#20031=CARTESIAN_POINT ( 'NONE',  ( 14.99999662536863632, -77.94228634059960825, -9.999999999999998224 ) ) ;
#20032=LINE ( 'NONE', #30916, #32400 ) ;
#20033=AXIS2_PLACEMENT_3D ( 'NONE', #11526, #13973, #28235 ) ;
#20034=DIRECTION ( 'NONE',  ( 0.000000000000000000, 0.000000000000000000, 1.000000000000000000 ) ) ;
#20035=ORIENTED_EDGE ( 'NONE', *, *, #9866, .T. ) ;
#20036=AXIS2_PLACEMENT_3D ( 'NONE', #36186, #1875, #24384 ) ;
#20037=FACE_BOUND ( 'NONE', #21701, .T. ) ;
#20038=ORIENTED_EDGE ( 'NONE', *, *, #20069, .T. ) ;
#20040=EDGE_CURVE ( 'NONE', #7675, #7436, #12840, .T. ) ;
#20041=CARTESIAN_POINT ( 'NONE',  ( -63.00000337463106348, -60.62177826491083010, 12.50000000000000000 ) ) ;
#20042=EDGE_LOOP ( 'NONE', ( #7491, #21163 ) ) ;
#20043=AXIS2_PLACEMENT_3D ( 'NONE', #5616, #17052, #28482 ) ;
#20044=VECTOR ( 'NONE', #23039, 1000.000000000000000 ) ;
#20045=AXIS2_PLACEMENT_3D ( 'NONE', #24104, #29165, #1235 ) ;
#20046=DIRECTION ( 'NONE',  ( 0.000000000000000000, 0.000000000000000000, 1.000000000000000000 ) ) ;
#20047=DIRECTION ( 'NONE',  ( -1.000000000000000000, 0.000000000000000000, 0.000000000000000000 ) ) ;
#20048=ORIENTED_EDGE ( 'NONE', *, *, #5687, .T. ) ;
#20051=ORIENTED_EDGE ( 'NONE', *, *, #5221, .F. ) ;
#20052=ORIENTED_EDGE ( 'NONE', *, *, #34444, .T. ) ;
#20054=CARTESIAN_POINT ( 'NONE',  ( 76.99999662536836809, 43.30127018922198801, 12.50000000000000000 ) ) ;
#20056=CIRCLE ( 'NONE', #2697, 2.000000000000001776 ) ;
#20057=CARTESIAN_POINT ( 'NONE',  ( 42.99999662536850309, 77.94228634059959404, 17.49999999999999645 ) ) ;
#20058=CARTESIAN_POINT ( 'NONE',  ( 59.99999662536842493, -51.96152422706639840, 12.50000000000000000 ) ) ;
#20060=EDGE_CURVE ( 'NONE', #719, #24333, #14637, .T. ) ;
#20061=ORIENTED_EDGE ( 'NONE', *, *, #24091, .T. ) ;
#20062=AXIS2_PLACEMENT_3D ( 'NONE', #16099, #27521, #5009 ) ;
#20066=DIRECTION ( 'NONE',  ( 0.000000000000000000, 0.000000000000000000, 1.000000000000000000 ) ) ;
#20068=CARTESIAN_POINT ( 'NONE',  ( -53.00000337463110611, -43.30127018922202353, -9.999999999999998224 ) ) ;
#20069=EDGE_CURVE ( 'NONE', #2324, #15669, #1977, .T. ) ;
#20071=CIRCLE ( 'NONE', #3903, 2.000000000000001776 ) ;
#20073=VECTOR ( 'NONE', #6456, 1000.000000000000000 ) ;
#20074=ORIENTED_EDGE ( 'NONE', *, *, #1869, .F. ) ;
#20075=ADVANCED_FACE ( 'NONE', ( #5172 ), #13606, .F. ) ;
#20076=CARTESIAN_POINT ( 'NONE',  ( -45.00000337463111322, -77.94228634059960825, 12.50000000000000000 ) ) ;
#20077=CYLINDRICAL_SURFACE ( 'NONE', #1978, 2.000000000000001776 ) ;
#20078=DIRECTION ( 'NONE',  ( 0.000000000000000000, 0.000000000000000000, 1.000000000000000000 ) ) ;
#20080=ORIENTED_EDGE ( 'NONE', *, *, #10600, .T. ) ;
#20082=LINE ( 'NONE', #23079, #32070 ) ;
#20084=CARTESIAN_POINT ( 'NONE',  ( 74.99999662536835388, -25.98076211353319565, -5.000000000000000000 ) ) ;
#20086=VERTEX_POINT ( 'NONE', #16610 ) ;
#20087=EDGE_CURVE ( 'NONE', #12699, #5447, #36304, .T. ) ;
#20089=CARTESIAN_POINT ( 'NONE',  ( -70.00000337463099243, 34.64101615137758472, -9.999999999999998224 ) ) ;
#20090=ORIENTED_EDGE ( 'NONE', *, *, #23154, .T. ) ;
#20091=CIRCLE ( 'NONE', #19511, 3.000000000000002665 ) ;
#20092=AXIS2_PLACEMENT_3D ( 'NONE', #24849, #36102, #10401 ) ;
#20093=ORIENTED_EDGE ( 'NONE', *, *, #1611, .T. ) ;
#20094=CIRCLE ( 'NONE', #23683, 2.000000000000001776 ) ;
#20096=DIRECTION ( 'NONE',  ( 1.000000000000000000, 0.000000000000000000, 0.000000000000000000 ) ) ;
#20097=ORIENTED_EDGE ( 'NONE', *, *, #6441, .F. ) ;
#20098=ORIENTED_EDGE ( 'NONE', *, *, #12812, .T. ) ;
#20099=CARTESIAN_POINT ( 'NONE',  ( -73.00000337463097821, 8.660254037844374864, -9.999999999999998224 ) ) ;
#20101=CARTESIAN_POINT ( 'NONE',  ( 0.000000000000000000, 0.000000000000000000, -5.000000000000000000 ) ) ;
#20104=ORIENTED_EDGE ( 'NONE', *, *, #22497, .T. ) ;
#20107=FACE_BOUND ( 'NONE', #18367, .T. ) ;
#20108=CARTESIAN_POINT ( 'NONE',  ( -52.00000337463109190, 69.28203230275518365, -5.000000000000000000 ) ) ;
#20110=DIRECTION ( 'NONE',  ( 0.000000000000000000, 0.000000000000000000, 1.000000000000000000 ) ) ;
#20111=DIRECTION ( 'NONE',  ( 1.000000000000000000, 0.000000000000000000, 0.000000000000000000 ) ) ;
#20112=CIRCLE ( 'NONE', #18317, 3.000000000000006661 ) ;
#20113=EDGE_CURVE ( 'NONE', #34280, #15339, #33820, .T. ) ;
#20114=DIRECTION ( 'NONE',  ( 0.000000000000000000, 0.000000000000000000, 1.000000000000000000 ) ) ;
#20115=AXIS2_PLACEMENT_3D ( 'NONE', #6223, #778, #23307 ) ;
#20116=DIRECTION ( 'NONE',  ( 1.000000000000000000, 0.000000000000000000, 0.000000000000000000 ) ) ;
#20117=VERTEX_POINT ( 'NONE', #10966 ) ;
#20118=CARTESIAN_POINT ( 'NONE',  ( -67.00000337463102085, 25.98076211353317433, -9.999999999999998224 ) ) ;
#20121=DIRECTION ( 'NONE',  ( 0.000000000000000000, 0.000000000000000000, -1.000000000000000000 ) ) ;
#20122=CIRCLE ( 'NONE', #12913, 2.000000000000001776 ) ;
#20123=CIRCLE ( 'NONE', #14740, 3.499999999999987566 ) ;
#20125=ORIENTED_EDGE ( 'NONE', *, *, #9681, .F. ) ;
#20127=ORIENTED_EDGE ( 'NONE', *, *, #21186, .F. ) ;
#20128=EDGE_CURVE ( 'NONE', #29187, #12874, #14049, .T. ) ;
#20129=CARTESIAN_POINT ( 'NONE',  ( -22.00000337463124112, -86.60254037844400443, -9.999999999999998224 ) ) ;
#20130=CARTESIAN_POINT ( 'NONE',  ( 14.99999662536863632, -77.94228634059960825, 12.50000000000000000 ) ) ;
#20131=DIRECTION ( 'NONE',  ( 1.000000000000000000, 0.000000000000000000, 0.000000000000000000 ) ) ;
#20132=ORIENTED_EDGE ( 'NONE', *, *, #6914, .T. ) ;
#20133=CIRCLE ( 'NONE', #26717, 1.999999999999998224 ) ;
#20134=FACE_OUTER_BOUND ( 'NONE', #4601, .T. ) ;
#20135=EDGE_LOOP ( 'NONE', ( #13590, #30475 ) ) ;
#20137=VERTEX_POINT ( 'NONE', #8536 ) ;
#20138=CARTESIAN_POINT ( 'NONE',  ( 44.99999662536849598, 60.62177826491077326, -5.000000000000000000 ) ) ;
#20139=ORIENTED_EDGE ( 'NONE', *, *, #6531, .F. ) ;
#20140=AXIS2_PLACEMENT_3D ( 'NONE', #18255, #29684, #18648 ) ;
#20141=ORIENTED_EDGE ( 'NONE', *, *, #26252, .F. ) ;
#20144=CIRCLE ( 'NONE', #8158, 2.000000000000001776 ) ;
#20148=LINE ( 'NONE', #20892, #27479 ) ;
#20149=AXIS2_PLACEMENT_3D ( 'NONE', #16785, #34384, #13779 ) ;
#20152=EDGE_CURVE ( 'NONE', #19630, #31778, #1471, .T. ) ;
#20154=CARTESIAN_POINT ( 'NONE',  ( -87.00000337463093558, -25.98076211353322051, 17.49999999999999645 ) ) ;
#20155=AXIS2_PLACEMENT_3D ( 'NONE', #21306, #32745, #7072 ) ;
#20156=EDGE_LOOP ( 'NONE', ( #27058, #14668, #18750, #21679 ) ) ;
#20157=DIRECTION ( 'NONE',  ( 1.000000000000000000, 0.000000000000000000, 0.000000000000000000 ) ) ;
#20159=EDGE_CURVE ( 'NONE', #7729, #12225, #6266, .T. ) ;
#20160=VERTEX_POINT ( 'NONE', #33851 ) ;
#20162=EDGE_CURVE ( 'NONE', #3839, #36232, #23641, .T. ) ;
#20163=CARTESIAN_POINT ( 'NONE',  ( 61.99999662536842493, -51.96152422706639840, 17.49999999999999645 ) ) ;
#20164=CARTESIAN_POINT ( 'NONE',  ( 79.99999662536832545, -17.32050807568879591, -9.999999999999998224 ) ) ;
#20165=DIRECTION ( 'NONE',  ( 0.000000000000000000, 0.000000000000000000, -1.000000000000000000 ) ) ;
#20166=DIRECTION ( 'NONE',  ( 0.000000000000000000, 0.000000000000000000, 1.000000000000000000 ) ) ;
#20167=VERTEX_POINT ( 'NONE', #11695 ) ;
#20169=CARTESIAN_POINT ( 'NONE',  ( 76.99999662536836809, 25.98076211353319565, -9.999999999999998224 ) ) ;
#20170=CIRCLE ( 'NONE', #373, 2.000000000000001776 ) ;
#20172=ORIENTED_EDGE ( 'NONE', *, *, #14503, .F. ) ;
#20173=ORIENTED_EDGE ( 'NONE', *, *, #36350, .F. ) ;
#20174=EDGE_CURVE ( 'NONE', #3735, #36464, #4484, .T. ) ;
#20175=AXIS2_PLACEMENT_3D ( 'NONE', #4309, #1123, #7679 ) ;
#20177=DIRECTION ( 'NONE',  ( 0.000000000000000000, 0.000000000000000000, -1.000000000000000000 ) ) ;
#20178=ADVANCED_BREP_SHAPE_REPRESENTATION ( '', ( #19388, #21385 ), #23118 ) ;
#20179=CARTESIAN_POINT ( 'NONE',  ( 0.000000000000000000, 0.000000000000000000, -5.000000000000000000 ) ) ;
#20180=CARTESIAN_POINT ( 'NONE',  ( -4.279621169095561228, 62.97617850287782915, -4.999999999999997335 ) ) ;
#20182=VECTOR ( 'NONE', #34888, 1000.000000000000000 ) ;
#20183=CIRCLE ( 'NONE', #4016, 3.499999999999989342 ) ;
#20185=CARTESIAN_POINT ( 'NONE',  ( 9.999996625368655856, -69.28203230275519786, -5.000000000000000000 ) ) ;
#20186=ORIENTED_EDGE ( 'NONE', *, *, #14371, .F. ) ;
#20187=LINE ( 'NONE', #37079, #29894 ) ;
#20189=FACE_BOUND ( 'NONE', #35004, .T. ) ;
#20192=DIRECTION ( 'NONE',  ( 0.000000000000000000, 0.000000000000000000, 1.000000000000000000 ) ) ;
#20193=FACE_OUTER_BOUND ( 'NONE', #21717, .T. ) ;
#20194=EDGE_CURVE ( 'NONE', #14287, #20625, #28422, .T. ) ;
#20196=AXIS2_PLACEMENT_3D ( 'NONE', #9769, #27401, #16164 ) ;
#20197=EDGE_CURVE ( 'NONE', #28343, #26021, #9258, .T. ) ;
#20198=FACE_OUTER_BOUND ( 'NONE', #16146, .T. ) ;
#20199=AXIS2_PLACEMENT_3D ( 'NONE', #13466, #1225, #14918 ) ;
#20200=FACE_OUTER_BOUND ( 'NONE', #9138, .T. ) ;
#20201=PLANE ( 'NONE',  #23932 ) ;
#20202=VERTEX_POINT ( 'NONE', #25609 ) ;
#20203=DIRECTION ( 'NONE',  ( 0.000000000000000000, 0.000000000000000000, 1.000000000000000000 ) ) ;
#20204=EDGE_CURVE ( 'NONE', #25880, #9332, #28590, .T. ) ;
#20206=CARTESIAN_POINT ( 'NONE',  ( -30.99999999999944933, 58.88972745734214698, 12.49999999999999822 ) ) ;
#20208=AXIS2_PLACEMENT_3D ( 'NONE', #447, #34400, #26332 ) ;
#20209=VECTOR ( 'NONE', #27725, 1000.000000000000000 ) ;
#20210=EDGE_LOOP ( 'NONE', ( #28755, #20360, #27042, #10229, #24012, #19540, #3526, #16297, #28792, #26998, #28667, #14777, #31300, #14638, #34687, #3602, #35410, #13148, #6834, #14383, #15144, #28036, #20400, #25508, #7076, #19068, #796, #9912, #14124, #2799, #18314, #3578, #19329, #6559, #11466, #18146, #25085, #16639, #28777, #27945, #13942, #36361, #17671, #15646, #2518, #1145, #36439, #34341, #30893, #33572, #32571, #14994, #4300, #16497, #6934, #16336, #5858, #33134, #13413, #9698, #35844, #4955, #28264, #14339, #19235, #11106, #6440, #29484, #8494, #7452, #21649, #32626, #30341, #9108, #15289, #19427, #16171, #2077, #9804, #36140, #3884, #12088, #12778, #9546, #6990, #34043, #15551, #26427, #9257, #12622, #36228, #20547, #13941, #25865, #22957, #20661, #24163, #8743, #29114, #2151, #2230, #35915, #21053, #36847, #23013, #34974, #28302, #35581, #291, #35605, #35920, #35439, #5550, #13953, #31469, #15914, #4176, #37037, #8526, #12779, #16291, #10210, #25230, #1720, #13320, #4761, #36425, #10003, #27984, #28720, #1547, #32002, #6621, #23954, #36589, #13507, #10797, #20478, #4242, #31266, #31743, #9022, #17451, #9170, #35304, #28747, #2015, #28536, #8335, #36606, #9583, #18944, #35565, #7659, #4507, #28028, #15451, #12771, #22191, #30497, #21216, #14160, #11599, #29117, #24346, #30678, #14424, #26154, #20686, #27227, #8690, #27160, #29433, #18982, #25259, #36444, #32108, #185, #30365, #12386, #3145, #23708, #10364, #33967, #33618, #24429, #9059, #14980, #13343, #10190, #9554, #15555, #17354, #25911, #9442, #31402, #22660, #17030, #28138 ) ) ;
#20211=CIRCLE ( 'NONE', #8828, 3.000000000000002220 ) ;
#20212=VERTEX_POINT ( 'NONE', #20154 ) ;
#20213=ORIENTED_EDGE ( 'NONE', *, *, #23168, .F. ) ;
#20215=ADVANCED_FACE ( 'NONE', ( #16807 ), #31580, .F. ) ;
#20216=EDGE_CURVE ( 'NONE', #13186, #10841, #2538, .T. ) ;
#20217=FACE_BOUND ( 'NONE', #22843, .T. ) ;
#20218=EDGE_CURVE ( 'NONE', #23471, #10338, #19389, .T. ) ;
#20219=CIRCLE ( 'NONE', #19029, 33.00000000000001421 ) ;
#20221=CARTESIAN_POINT ( 'NONE',  ( 9.999996625368655856, -86.60254037844400443, 17.49999999999999645 ) ) ;
#20223=CARTESIAN_POINT ( 'NONE',  ( 0.000000000000000000, 0.000000000000000000, 17.49999999999999645 ) ) ;
#20224=AXIS2_PLACEMENT_3D ( 'NONE', #8735, #31949, #37069 ) ;
#20226=CARTESIAN_POINT ( 'NONE',  ( 67.99999662536839651, 51.96152422706640550, -9.999999999999998224 ) ) ;
#20227=EDGE_LOOP ( 'NONE', ( #32615, #5311 ) ) ;
#20228=AXIS2_PLACEMENT_3D ( 'NONE', #4679, #4863, #7471 ) ;
#20231=CIRCLE ( 'NONE', #21435, 3.000000000000004885 ) ;
#20232=DIRECTION ( 'NONE',  ( 1.000000000000000000, 0.000000000000000000, 0.000000000000000000 ) ) ;
#20233=DIRECTION ( 'NONE',  ( 1.000000000000000000, 0.000000000000000000, 0.000000000000000000 ) ) ;
#20234=ORIENTED_EDGE ( 'NONE', *, *, #35330, .F. ) ;
#20236=FACE_BOUND ( 'NONE', #18955, .T. ) ;
#20237=VERTEX_POINT ( 'NONE', #14353 ) ;
#20239=DIRECTION ( 'NONE',  ( 0.000000000000000000, 0.000000000000000000, 1.000000000000000000 ) ) ;
#20240=ORIENTED_EDGE ( 'NONE', *, *, #23623, .F. ) ;
#20241=AXIS2_PLACEMENT_3D ( 'NONE', #19805, #31228, #16974 ) ;
#20244=AXIS2_PLACEMENT_3D ( 'NONE', #596, #23648, #5865 ) ;
#20245=CARTESIAN_POINT ( 'NONE',  ( 0.000000000000000000, 0.000000000000000000, 12.49999999999999822 ) ) ;
#20247=VERTEX_POINT ( 'NONE', #17352 ) ;
#20248=CIRCLE ( 'NONE', #16091, 95.00000000000000000 ) ;
#20249=ORIENTED_EDGE ( 'NONE', *, *, #3237, .F. ) ;
#20250=AXIS2_PLACEMENT_3D ( 'NONE', #17014, #5773, #8411 ) ;
#20251=ORIENTED_EDGE ( 'NONE', *, *, #22154, .F. ) ;
#20252=CIRCLE ( 'NONE', #2899, 2.000000000000001776 ) ;
#20253=ORIENTED_EDGE ( 'NONE', *, *, #5046, .T. ) ;
#20254=CARTESIAN_POINT ( 'NONE',  ( -30.00000337463119848, -69.28203230275522628, -9.999999999999998224 ) ) ;
#20255=DIRECTION ( 'NONE',  ( -0.000000000000000000, -0.000000000000000000, 1.000000000000000000 ) ) ;
#20256=LINE ( 'NONE', #360, #22057 ) ;
#20257=CYLINDRICAL_SURFACE ( 'NONE', #16324, 2.000000000000001776 ) ;
#20258=DIRECTION ( 'NONE',  ( 0.000000000000000000, 0.000000000000000000, -1.000000000000000000 ) ) ;
#20259=VERTEX_POINT ( 'NONE', #28776 ) ;
#20260=CARTESIAN_POINT ( 'NONE',  ( -52.00000337463109190, 69.28203230275518365, -9.999999999999998224 ) ) ;
#20261=VECTOR ( 'NONE', #14900, 1000.000000000000000 ) ;
#20263=ADVANCED_FACE ( 'NONE', ( #14525 ), #15681, .F. ) ;
#20264=FACE_OUTER_BOUND ( 'NONE', #8243, .T. ) ;
#20265=ORIENTED_EDGE ( 'NONE', *, *, #5784, .T. ) ;
#20269=ORIENTED_EDGE ( 'NONE', *, *, #8533, .T. ) ;
#20270=ORIENTED_EDGE ( 'NONE', *, *, #3782, .F. ) ;
#20271=DIRECTION ( 'NONE',  ( -0.8660254037844455910, -0.4999999999999878431, 0.000000000000000000 ) ) ;
#20274=CARTESIAN_POINT ( 'NONE',  ( 11.99999662536861855, 69.28203230275516944, -9.999999999999998224 ) ) ;
#20275=CYLINDRICAL_SURFACE ( 'NONE', #37056, 2.000000000000000000 ) ;
#20276=ORIENTED_EDGE ( 'NONE', *, *, #12048, .T. ) ;
#20277=VECTOR ( 'NONE', #14522, 1000.000000000000000 ) ;
#20281=VERTEX_POINT ( 'NONE', #20937 ) ;
#20282=VECTOR ( 'NONE', #26129, 1000.000000000000000 ) ;
#20285=ADVANCED_FACE ( 'NONE', ( #27100 ), #27283, .T. ) ;
#20286=CIRCLE ( 'NONE', #3537, 2.000000000000001776 ) ;
#20289=CIRCLE ( 'NONE', #25104, 95.00000000000001421 ) ;
#20290=DIRECTION ( 'NONE',  ( -0.000000000000000000, -0.000000000000000000, 1.000000000000000000 ) ) ;
#20291=CARTESIAN_POINT ( 'NONE',  ( 35.19434990244975126, -52.39915983220758022, -4.999999999999997335 ) ) ;
#20292=ORIENTED_EDGE ( 'NONE', *, *, #3572, .F. ) ;
#20293=ORIENTED_EDGE ( 'NONE', *, *, #11843, .T. ) ;
#20295=DIRECTION ( 'NONE',  ( -1.000000000000000000, 0.000000000000000000, 0.000000000000000000 ) ) ;
#20296=EDGE_CURVE ( 'NONE', #30820, #12760, #1606, .T. ) ;
#20297=ORIENTED_EDGE ( 'NONE', *, *, #27040, .T. ) ;
#20298=DIRECTION ( 'NONE',  ( 0.000000000000000000, 0.000000000000000000, 1.000000000000000000 ) ) ;
#20299=AXIS2_PLACEMENT_3D ( 'NONE', #34101, #13655, #11202 ) ;
#20300=FACE_BOUND ( 'NONE', #13443, .T. ) ;
#20302=DIRECTION ( 'NONE',  ( -1.000000000000000000, 0.000000000000000000, -0.000000000000000000 ) ) ;
#20303=CARTESIAN_POINT ( 'NONE',  ( -72.00000337463100664, 51.96152422706637708, 17.49999999999999645 ) ) ;
#20304=DIRECTION ( 'NONE',  ( 0.000000000000000000, 0.000000000000000000, 1.000000000000000000 ) ) ;
#20305=CARTESIAN_POINT ( 'NONE',  ( -65.00000337463104927, -25.98076211353322051, -9.999999999999998224 ) ) ;
#20306=AXIS2_PLACEMENT_3D ( 'NONE', #6246, #2700, #3084 ) ;
#20307=EDGE_CURVE ( 'NONE', #20787, #25733, #25387, .T. ) ;
#20309=ORIENTED_EDGE ( 'NONE', *, *, #1405, .T. ) ;
#20310=CARTESIAN_POINT ( 'NONE',  ( -25.30168483247182820, 79.91940249752995840, -5.000000000000000000 ) ) ;
#20311=DIRECTION ( 'NONE',  ( 1.000000000000000000, 0.000000000000000000, 0.000000000000000000 ) ) ;
#20312=DIRECTION ( 'NONE',  ( -0.000000000000000000, -0.000000000000000000, 1.000000000000000000 ) ) ;
#20314=CIRCLE ( 'NONE', #8362, 2.000000000000001776 ) ;
#20317=CIRCLE ( 'NONE', #34093, 2.000000000000001776 ) ;
#20318=ORIENTED_EDGE ( 'NONE', *, *, #5572, .F. ) ;
#20319=CARTESIAN_POINT ( 'NONE',  ( 7.999996625368625658, 86.60254037844397601, -9.999999999999998224 ) ) ;
#20320=DIRECTION ( 'NONE',  ( 0.000000000000000000, 0.000000000000000000, 1.000000000000000000 ) ) ;
#20321=CARTESIAN_POINT ( 'NONE',  ( 7.999996625368618552, 69.28203230275516944, 17.49999999999999645 ) ) ;
#20322=ORIENTED_EDGE ( 'NONE', *, *, #15606, .F. ) ;
#20323=DIRECTION ( 'NONE',  ( -0.000000000000000000, -0.000000000000000000, 1.000000000000000000 ) ) ;
#20325=VERTEX_POINT ( 'NONE', #18679 ) ;
#20326=EDGE_CURVE ( 'NONE', #12419, #34764, #34352, .T. ) ;
#20327=CARTESIAN_POINT ( 'NONE',  ( -77.00000337463099243, -25.98076211353322051, -9.999999999999998224 ) ) ;
#20328=VERTEX_POINT ( 'NONE', #12271 ) ;
#20329=VECTOR ( 'NONE', #27341, 1000.000000000000000 ) ;
#20330=CARTESIAN_POINT ( 'NONE',  ( 83.67878100130371877, -27.78182860042797131, -4.999999999999997335 ) ) ;
#20331=EDGE_LOOP ( 'NONE', ( #18801, #36717, #15771, #21254 ) ) ;
#20332=ORIENTED_EDGE ( 'NONE', *, *, #14503, .T. ) ;
#20333=FACE_OUTER_BOUND ( 'NONE', #26034, .T. ) ;
#20334=DIRECTION ( 'NONE',  ( -1.053683889111837881E-14, -1.000000000000000000, 0.000000000000000000 ) ) ;
#20335=EDGE_CURVE ( 'NONE', #35643, #33480, #27751, .T. ) ;
#20336=EDGE_LOOP ( 'NONE', ( #4868, #10710, #27501, #8001 ) ) ;
#20337=FACE_OUTER_BOUND ( 'NONE', #3090, .T. ) ;
#20338=CIRCLE ( 'NONE', #32927, 2.000000000000001776 ) ;
#20339=CYLINDRICAL_SURFACE ( 'NONE', #29418, 2.000000000000001776 ) ;
#20342=EDGE_CURVE ( 'NONE', #3626, #11344, #6683, .T. ) ;
#20343=EDGE_LOOP ( 'NONE', ( #27587, #6066 ) ) ;
#20344=CARTESIAN_POINT ( 'NONE',  ( -12.97563234535667753, 90.60231327712331506, -4.999999999999997335 ) ) ;
#20345=CARTESIAN_POINT ( 'NONE',  ( 71.99999662536839651, 17.32050807568879236, -9.999999999999998224 ) ) ;
#20346=EDGE_LOOP ( 'NONE', ( #19142, #32372, #11810, #34351 ) ) ;
#20348=CARTESIAN_POINT ( 'NONE',  ( 32.99999662536855283, 60.62177826491078747, -9.999999999999998224 ) ) ;
#20349=DIRECTION ( 'NONE',  ( 0.000000000000000000, 0.000000000000000000, 1.000000000000000000 ) ) ;
#20350=CARTESIAN_POINT ( 'NONE',  ( 36.99999662536853862, 77.94228634059959404, -9.999999999999998224 ) ) ;
#20352=CARTESIAN_POINT ( 'NONE',  ( 4.279621169095998212, -62.97617850287780072, 12.49999999999999822 ) ) ;
#20353=CIRCLE ( 'NONE', #23951, 2.000000000000000000 ) ;
#20355=AXIS2_PLACEMENT_3D ( 'NONE', #34825, #9119, #31966 ) ;
#20356=DIRECTION ( 'NONE',  ( 0.000000000000000000, 0.000000000000000000, -1.000000000000000000 ) ) ;
#20357=CARTESIAN_POINT ( 'NONE',  ( -55.00000337463107059, 43.30127018922197379, 12.50000000000000000 ) ) ;
#20358=ORIENTED_EDGE ( 'NONE', *, *, #12802, .T. ) ;
#20359=EDGE_CURVE ( 'NONE', #7909, #19401, #11573, .T. ) ;
#20360=ORIENTED_EDGE ( 'NONE', *, *, #31840, .T. ) ;
#20361=VERTEX_POINT ( 'NONE', #6855 ) ;
#20362=DIRECTION ( 'NONE',  ( 0.000000000000000000, 0.000000000000000000, -1.000000000000000000 ) ) ;
#20363=CARTESIAN_POINT ( 'NONE',  ( 1.999996625368710257, -69.28203230275519786, 17.49999999999999645 ) ) ;
#20364=CYLINDRICAL_SURFACE ( 'NONE', #13459, 2.000000000000001776 ) ;
#20367=CARTESIAN_POINT ( 'NONE',  ( 24.99999662536859546, -77.94228634059960825, -9.999999999999998224 ) ) ;
#20368=ORIENTED_EDGE ( 'NONE', *, *, #16332, .T. ) ;
#20369=EDGE_CURVE ( 'NONE', #2346, #20659, #21292, .T. ) ;
#20371=CARTESIAN_POINT ( 'NONE',  ( 2.999996625368676728, -77.94228634059960825, -9.999999999999998224 ) ) ;
#20373=FACE_BOUND ( 'NONE', #28119, .T. ) ;
#20374=AXIS2_PLACEMENT_3D ( 'NONE', #21362, #1472, #26985 ) ;
#20375=FACE_OUTER_BOUND ( 'NONE', #32274, .T. ) ;
#20376=VECTOR ( 'NONE', #35590, 1000.000000000000000 ) ;
#20377=DIRECTION ( 'NONE',  ( 1.000000000000000000, 0.000000000000000000, 0.000000000000000000 ) ) ;
#20378=DIRECTION ( 'NONE',  ( 0.000000000000000000, 0.000000000000000000, 1.000000000000000000 ) ) ;
#20381=EDGE_CURVE ( 'NONE', #33432, #33197, #5014, .T. ) ;
#20383=DIRECTION ( 'NONE',  ( 0.000000000000000000, 0.000000000000000000, -1.000000000000000000 ) ) ;
#20384=EDGE_LOOP ( 'NONE', ( #34922, #19440 ) ) ;
#20385=CIRCLE ( 'NONE', #19, 27.00000000000001421 ) ;
#20386=DIRECTION ( 'NONE',  ( 0.000000000000000000, 0.000000000000000000, 1.000000000000000000 ) ) ;
#20387=CARTESIAN_POINT ( 'NONE',  ( 19.99999662536857770, 86.60254037844397601, 17.49999999999999645 ) ) ;
#20388=DIRECTION ( 'NONE',  ( -1.000000000000000000, 0.000000000000000000, 0.000000000000000000 ) ) ;
#20389=ORIENTED_EDGE ( 'NONE', *, *, #12762, .F. ) ;
#20390=ORIENTED_EDGE ( 'NONE', *, *, #27502, .T. ) ;
#20392=ORIENTED_EDGE ( 'NONE', *, *, #34972, .F. ) ;
#20394=ADVANCED_FACE ( 'NONE', ( #7611 ), #34542, .F. ) ;
#20395=CARTESIAN_POINT ( 'NONE',  ( 79.99999662536832545, -17.32050807568879591, 12.50000000000000000 ) ) ;
#20396=FACE_OUTER_BOUND ( 'NONE', #13833, .T. ) ;
#20397=EDGE_CURVE ( 'NONE', #17463, #3839, #31521, .T. ) ;
#20399=CARTESIAN_POINT ( 'NONE',  ( -55.00000337463107059, 43.30127018922197379, -5.000000000000000000 ) ) ;
#20400=ORIENTED_EDGE ( 'NONE', *, *, #35550, .T. ) ;
#20401=EDGE_CURVE ( 'NONE', #30139, #36972, #6207, .T. ) ;
#20403=CARTESIAN_POINT ( 'NONE',  ( -18.03953374218250971, 86.20686523360116382, 12.50000000000000000 ) ) ;
#20404=FACE_OUTER_BOUND ( 'NONE', #5421, .T. ) ;
#20407=ORIENTED_EDGE ( 'NONE', *, *, #28529, .T. ) ;
#20410=ORIENTED_EDGE ( 'NONE', *, *, #18323, .T. ) ;
#20411=ORIENTED_EDGE ( 'NONE', *, *, #22269, .T. ) ;
#20412=VECTOR ( 'NONE', #20807, 1000.000000000000000 ) ;
#20413=DIRECTION ( 'NONE',  ( 0.000000000000000000, 0.000000000000000000, 1.000000000000000000 ) ) ;
#20414=EDGE_LOOP ( 'NONE', ( #3632, #27154 ) ) ;
#20416=EDGE_CURVE ( 'NONE', #33988, #16224, #27486, .T. ) ;
#20417=DIRECTION ( 'NONE',  ( 0.000000000000000000, 0.000000000000000000, 1.000000000000000000 ) ) ;
#20418=ADVANCED_FACE ( 'NONE', ( #16242 ), #28726, .F. ) ;
#20419=FACE_BOUND ( 'NONE', #27385, .T. ) ;
#20421=ORIENTED_EDGE ( 'NONE', *, *, #14115, .F. ) ;
#20422=EDGE_CURVE ( 'NONE', #27517, #32313, #205, .T. ) ;
#20423=ORIENTED_EDGE ( 'NONE', *, *, #642, .F. ) ;
#20427=DIRECTION ( 'NONE',  ( 0.000000000000000000, 0.000000000000000000, 1.000000000000000000 ) ) ;
#20428=DIRECTION ( 'NONE',  ( -0.000000000000000000, 0.000000000000000000, -1.000000000000000000 ) ) ;
#20430=CARTESIAN_POINT ( 'NONE',  ( 71.20511420343271425, 36.23716514913449060, 12.50000000000000000 ) ) ;
#20431=CARTESIAN_POINT ( 'NONE',  ( -66.86787810013036903, 2.778182860042780700, -49.86348611802629449 ) ) ;
#20432=EDGE_LOOP ( 'NONE', ( #24640, #26939, #25383, #35691, #23276, #30897 ) ) ;
#20433=FACE_OUTER_BOUND ( 'NONE', #3823, .T. ) ;
#20434=CARTESIAN_POINT ( 'NONE',  ( 79.99999662536832545, -17.32050807568879591, 12.50000000000000000 ) ) ;
#20435=DIRECTION ( 'NONE',  ( 0.000000000000000000, 0.000000000000000000, 1.000000000000000000 ) ) ;
#20437=DIRECTION ( 'NONE',  ( -0.000000000000000000, 0.000000000000000000, -1.000000000000000000 ) ) ;
#20438=CARTESIAN_POINT ( 'NONE',  ( 7.999996625368618552, 69.28203230275516944, -9.999999999999998224 ) ) ;
#20439=ORIENTED_EDGE ( 'NONE', *, *, #27328, .F. ) ;
#20440=VERTEX_POINT ( 'NONE', #13234 ) ;
#20441=DIRECTION ( 'NONE',  ( 1.000000000000000000, 0.000000000000000000, 0.000000000000000000 ) ) ;
#20442=CARTESIAN_POINT ( 'NONE',  ( -87.00000337463093558, -25.98076211353322051, -5.000000000000000000 ) ) ;
#20445=DIRECTION ( 'NONE',  ( 1.000000000000000000, 0.000000000000000000, 0.000000000000000000 ) ) ;
#20448=ORIENTED_EDGE ( 'NONE', *, *, #18702, .F. ) ;
#20449=AXIS2_PLACEMENT_3D ( 'NONE', #25017, #25203, #36255 ) ;
#20450=CIRCLE ( 'NONE', #33649, 2.000000000000001776 ) ;
#20452=VERTEX_POINT ( 'NONE', #28532 ) ;
#20453=DIRECTION ( 'NONE',  ( 0.000000000000000000, 0.000000000000000000, 1.000000000000000000 ) ) ;
#20454=ADVANCED_FACE ( 'NONE', ( #24679 ), #36111, .F. ) ;
#20455=FACE_OUTER_BOUND ( 'NONE', #8448, .T. ) ;
#20456=DIRECTION ( 'NONE',  ( 0.000000000000000000, 0.000000000000000000, 1.000000000000000000 ) ) ;
#20457=EDGE_CURVE ( 'NONE', #11539, #32632, #18172, .T. ) ;
#20458=VERTEX_POINT ( 'NONE', #1971 ) ;
#20460=CARTESIAN_POINT ( 'NONE',  ( 4.279621169095998212, -62.97617850287780072, -4.999999999999997335 ) ) ;
#20461=DIRECTION ( 'NONE',  ( 1.000000000000000000, 0.000000000000000000, 0.000000000000000000 ) ) ;
#20462=CARTESIAN_POINT ( 'NONE',  ( 74.99999662536836809, -8.660254037844401509, -9.999999999999998224 ) ) ;
#20463=EDGE_LOOP ( 'NONE', ( #6010, #10910, #6730, #748 ) ) ;
#20464=DIRECTION ( 'NONE',  ( 0.000000000000000000, 0.000000000000000000, -1.000000000000000000 ) ) ;
#20465=FACE_BOUND ( 'NONE', #32217, .T. ) ;
#20468=DIRECTION ( 'NONE',  ( 1.000000000000000000, 0.000000000000000000, 0.000000000000000000 ) ) ;
#20469=CARTESIAN_POINT ( 'NONE',  ( 0.000000000000000000, 0.000000000000000000, 12.49999999999999822 ) ) ;
#20470=DIRECTION ( 'NONE',  ( 0.000000000000000000, 0.000000000000000000, 1.000000000000000000 ) ) ;
#20471=CIRCLE ( 'NONE', #3122, 2.000000000000001776 ) ;
#20472=CARTESIAN_POINT ( 'NONE',  ( -35.00000337463116296, 60.62177826491077326, 17.49999999999999645 ) ) ;
#20474=CARTESIAN_POINT ( 'NONE',  ( -75.00000337463097821, 8.660254037844374864, 17.49999999999999645 ) ) ;
#20475=DIRECTION ( 'NONE',  ( 1.000000000000000000, 0.000000000000000000, 0.000000000000000000 ) ) ;
#20478=ORIENTED_EDGE ( 'NONE', *, *, #25765, .T. ) ;
#20481=CARTESIAN_POINT ( 'NONE',  ( -45.00000337463111322, -77.94228634059960825, -5.000000000000000000 ) ) ;
#20482=DIRECTION ( 'NONE',  ( -1.000000000000000000, 0.000000000000000000, 0.000000000000000000 ) ) ;
#20483=CYLINDRICAL_SURFACE ( 'NONE', #8839, 2.000000000000001776 ) ;
#20484=ORIENTED_EDGE ( 'NONE', *, *, #27127, .F. ) ;
#20485=EDGE_CURVE ( 'NONE', #2978, #19796, #17578, .T. ) ;
#20486=CARTESIAN_POINT ( 'NONE',  ( -53.00000337463110611, -43.30127018922202353, -9.999999999999998224 ) ) ;
#20487=AXIS2_PLACEMENT_3D ( 'NONE', #34721, #15016, #26269 ) ;
#20488=EDGE_LOOP ( 'NONE', ( #26986, #19339, #27799, #23679 ) ) ;
#20490=ORIENTED_EDGE ( 'NONE', *, *, #6188, .T. ) ;
#20491=DIRECTION ( 'NONE',  ( 0.000000000000000000, 0.000000000000000000, 1.000000000000000000 ) ) ;
#20492=VERTEX_POINT ( 'NONE', #22746 ) ;
#20493=EDGE_LOOP ( 'NONE', ( #25596, #28439 ) ) ;
#20495=FACE_BOUND ( 'NONE', #22395, .T. ) ;
#20496=DIRECTION ( 'NONE',  ( 0.000000000000000000, 0.000000000000000000, 1.000000000000000000 ) ) ;
#20497=EDGE_CURVE ( 'NONE', #20792, #34742, #25972, .T. ) ;
#20498=ORIENTED_EDGE ( 'NONE', *, *, #36928, .F. ) ;
#20499=DIRECTION ( 'NONE',  ( -0.000000000000000000, -0.000000000000000000, 1.000000000000000000 ) ) ;
#20500=DIRECTION ( 'NONE',  ( 1.000000000000000000, 0.000000000000000000, 0.000000000000000000 ) ) ;
#20502=ORIENTED_EDGE ( 'NONE', *, *, #17249, .T. ) ;
#20503=FACE_OUTER_BOUND ( 'NONE', #23994, .T. ) ;
#20505=ORIENTED_EDGE ( 'NONE', *, *, #28258, .T. ) ;
#20506=LINE ( 'NONE', #20348, #26210 ) ;
#20507=DIRECTION ( 'NONE',  ( 1.000000000000000000, 0.000000000000000000, 0.000000000000000000 ) ) ;
#20511=AXIS2_PLACEMENT_3D ( 'NONE', #35834, #18586, #21742 ) ;
#20512=DIRECTION ( 'NONE',  ( 0.000000000000000000, 0.000000000000000000, 1.000000000000000000 ) ) ;
#20513=EDGE_CURVE ( 'NONE', #35481, #11539, #30752, .T. ) ;
#20514=DIRECTION ( 'NONE',  ( -0.000000000000000000, -0.000000000000000000, 1.000000000000000000 ) ) ;
#20515=ORIENTED_EDGE ( 'NONE', *, *, #3699, .T. ) ;
#20516=CARTESIAN_POINT ( 'NONE',  ( -42.00000337463114164, 69.28203230275516944, -9.999999999999998224 ) ) ;
#20520=ORIENTED_EDGE ( 'NONE', *, *, #249, .T. ) ;
#20522=ORIENTED_EDGE ( 'NONE', *, *, #12762, .T. ) ;
#20523=CIRCLE ( 'NONE', #28316, 2.000000000000001776 ) ;
#20524=DIRECTION ( 'NONE',  ( 0.000000000000000000, 0.000000000000000000, 1.000000000000000000 ) ) ;
#20525=DIRECTION ( 'NONE',  ( 0.000000000000000000, 0.000000000000000000, 1.000000000000000000 ) ) ;
#20527=EDGE_CURVE ( 'NONE', #8275, #911, #9031, .T. ) ;
#20528=DIRECTION ( 'NONE',  ( 1.000000000000000000, 0.000000000000000000, 0.000000000000000000 ) ) ;
#20530=LINE ( 'NONE', #3500, #35653 ) ;
#20531=ORIENTED_EDGE ( 'NONE', *, *, #16271, .F. ) ;
#20532=DIRECTION ( 'NONE',  ( 1.000000000000000000, 0.000000000000000000, 0.000000000000000000 ) ) ;
#20534=FACE_BOUND ( 'NONE', #18166, .T. ) ;
#20537=DIRECTION ( 'NONE',  ( 0.000000000000000000, 0.000000000000000000, 1.000000000000000000 ) ) ;
#20538=EDGE_CURVE ( 'NONE', #12874, #2651, #16415, .T. ) ;
#20539=ORIENTED_EDGE ( 'NONE', *, *, #22393, .T. ) ;
#20542=CIRCLE ( 'NONE', #883, 27.00000000000001421 ) ;
#20543=DIRECTION ( 'NONE',  ( -0.000000000000000000, -0.000000000000000000, 1.000000000000000000 ) ) ;
#20544=AXIS2_PLACEMENT_3D ( 'NONE', #23114, #34568, #31730 ) ;
#20545=CARTESIAN_POINT ( 'NONE',  ( -3.374631289687624047E-06, -69.28203230275519786, -9.999999999999998224 ) ) ;
#20547=ORIENTED_EDGE ( 'NONE', *, *, #9758, .T. ) ;
#20548=CARTESIAN_POINT ( 'NONE',  ( 79.99999662536832545, -34.64101615137759183, -9.999999999999998224 ) ) ;
#20549=DIRECTION ( 'NONE',  ( 1.000000000000000000, 0.000000000000000000, 0.000000000000000000 ) ) ;
#20550=DIRECTION ( 'NONE',  ( -1.000000000000000000, 0.000000000000000000, 0.000000000000000000 ) ) ;
#20551=VECTOR ( 'NONE', #477, 1000.000000000000000 ) ;
#20552=EDGE_CURVE ( 'NONE', #5293, #15920, #25994, .T. ) ;
#20553=ORIENTED_EDGE ( 'NONE', *, *, #32560, .T. ) ;
#20554=VERTEX_POINT ( 'NONE', #34906 ) ;
#20555=ADVANCED_FACE ( 'NONE', ( #20455 ), #17470, .F. ) ;
#20556=EDGE_LOOP ( 'NONE', ( #23765, #20851 ) ) ;
#20558=DIRECTION ( 'NONE',  ( 0.000000000000000000, 0.000000000000000000, 1.000000000000000000 ) ) ;
#20559=AXIS2_PLACEMENT_3D ( 'NONE', #3711, #6323, #17964 ) ;
#20561=FACE_OUTER_BOUND ( 'NONE', #13542, .T. ) ;
#20563=EDGE_CURVE ( 'NONE', #2260, #19941, #33791, .T. ) ;
#20564=CARTESIAN_POINT ( 'NONE',  ( -70.00000337463099243, 34.64101615137758472, 17.49999999999999645 ) ) ;
#20565=DIRECTION ( 'NONE',  ( 1.000000000000000000, 0.000000000000000000, 0.000000000000000000 ) ) ;
#20566=VERTEX_POINT ( 'NONE', #26838 ) ;
#20569=DIRECTION ( 'NONE',  ( 0.000000000000000000, 0.000000000000000000, 1.000000000000000000 ) ) ;
#20570=EDGE_CURVE ( 'NONE', #21403, #942, #32268, .T. ) ;
#20571=STYLED_ITEM ( 'NONE', ( #19343 ), #19388 ) ;
#20572=DIRECTION ( 'NONE',  ( 0.000000000000000000, 0.000000000000000000, 1.000000000000000000 ) ) ;
#20573=CARTESIAN_POINT ( 'NONE',  ( -35.00000337463116296, 77.94228634059957983, -9.999999999999998224 ) ) ;
#20575=FACE_BOUND ( 'NONE', #8959, .T. ) ;
#20576=ORIENTED_EDGE ( 'NONE', *, *, #28682, .T. ) ;
#20577=EDGE_LOOP ( 'NONE', ( #26330, #5609, #12702, #15306 ) ) ;
#20578=DIRECTION ( 'NONE',  ( 1.000000000000000000, 0.000000000000000000, 0.000000000000000000 ) ) ;
#20581=AXIS2_PLACEMENT_3D ( 'NONE', #4040, #15482, #10734 ) ;
#20583=EDGE_CURVE ( 'NONE', #11389, #4196, #9202, .T. ) ;
#20585=DIRECTION ( 'NONE',  ( 0.000000000000000000, 0.000000000000000000, 1.000000000000000000 ) ) ;
#20586=VERTEX_POINT ( 'NONE', #17638 ) ;
#20587=EDGE_LOOP ( 'NONE', ( #11434, #13828, #6486, #7973 ) ) ;
#20588=ORIENTED_EDGE ( 'NONE', *, *, #7763, .F. ) ;
#20589=CIRCLE ( 'NONE', #4454, 2.000000000000001776 ) ;
#20590=EDGE_CURVE ( 'NONE', #3095, #34263, #11026, .T. ) ;
#20592=EDGE_LOOP ( 'NONE', ( #2920, #34500, #16296, #11946 ) ) ;
#20593=CARTESIAN_POINT ( 'NONE',  ( -8.000003374631281972, 86.60254037844397601, -5.000000000000000000 ) ) ;
#20594=CIRCLE ( 'NONE', #14022, 2.000000000000001776 ) ;
#20595=EDGE_CURVE ( 'NONE', #13905, #2028, #5036, .T. ) ;
#20597=EDGE_LOOP ( 'NONE', ( #9205, #759, #18391, #13217 ) ) ;
#20599=DIRECTION ( 'NONE',  ( 1.000000000000000000, 0.000000000000000000, 0.000000000000000000 ) ) ;
#20601=DIRECTION ( 'NONE',  ( -1.000000000000000000, 0.000000000000000000, 0.000000000000000000 ) ) ;
#20602=VERTEX_POINT ( 'NONE', #29626 ) ;
#20603=CARTESIAN_POINT ( 'NONE',  ( -20.00000337463123756, -69.28203230275522628, -5.000000000000000000 ) ) ;
#20606=ORIENTED_EDGE ( 'NONE', *, *, #23024, .F. ) ;
#20607=DIRECTION ( 'NONE',  ( -0.000000000000000000, -0.000000000000000000, 1.000000000000000000 ) ) ;
#20608=CIRCLE ( 'NONE', #18848, 2.000000000000001776 ) ;
#20609=CARTESIAN_POINT ( 'NONE',  ( 69.99999662536841072, 51.96152422706640550, -9.999999999999998224 ) ) ;
#20612=ORIENTED_EDGE ( 'NONE', *, *, #32921, .F. ) ;
#20614=EDGE_CURVE ( 'NONE', #22212, #25823, #17021, .T. ) ;
#20616=CYLINDRICAL_SURFACE ( 'NONE', #7876, 2.000000000000001776 ) ;
#20618=CARTESIAN_POINT ( 'NONE',  ( -35.00000337463116296, 60.62177826491077326, -9.999999999999998224 ) ) ;
#20619=VERTEX_POINT ( 'NONE', #35299 ) ;
#20620=CARTESIAN_POINT ( 'NONE',  ( -55.00000337463107059, 60.62177826491078747, -9.999999999999998224 ) ) ;
#20621=DIRECTION ( 'NONE',  ( 0.000000000000000000, 0.000000000000000000, -1.000000000000000000 ) ) ;
#20625=VERTEX_POINT ( 'NONE', #26091 ) ;
#20626=DIRECTION ( 'NONE',  ( 0.000000000000000000, 0.000000000000000000, 1.000000000000000000 ) ) ;
#20628=CARTESIAN_POINT ( 'NONE',  ( -87.00000337463093558, -8.660254037844422825, -9.999999999999998224 ) ) ;
#20630=EDGE_CURVE ( 'NONE', #14854, #5583, #3214, .T. ) ;
#20631=VECTOR ( 'NONE', #23198, 1000.000000000000000 ) ;
#20632=DIRECTION ( 'NONE',  ( 0.000000000000000000, 0.000000000000000000, 1.000000000000000000 ) ) ;
#20634=EDGE_CURVE ( 'NONE', #32102, #17303, #7447, .T. ) ;
#20636=ORIENTED_EDGE ( 'NONE', *, *, #13716, .F. ) ;
#20638=CARTESIAN_POINT ( 'NONE',  ( -33.00000337463117006, -77.94228634059963667, -9.999999999999998224 ) ) ;
#20639=DIRECTION ( 'NONE',  ( 0.000000000000000000, 0.000000000000000000, 1.000000000000000000 ) ) ;
#20641=ORIENTED_EDGE ( 'NONE', *, *, #14936, .F. ) ;
#20643=FACE_BOUND ( 'NONE', #20493, .T. ) ;
#20644=EDGE_CURVE ( 'NONE', #21044, #2447, #13402, .T. ) ;
#20645=DIRECTION ( 'NONE',  ( 0.000000000000000000, 0.000000000000000000, 1.000000000000000000 ) ) ;
#20648=EDGE_LOOP ( 'NONE', ( #23123, #19010 ) ) ;
#20650=CIRCLE ( 'NONE', #11077, 2.000000000000001776 ) ;
#20652=CARTESIAN_POINT ( 'NONE',  ( -33.00000337463116296, 60.62177826491077326, 12.50000000000000000 ) ) ;
#20655=CARTESIAN_POINT ( 'NONE',  ( -72.00000337463100664, -17.32050807568882078, 12.50000000000000000 ) ) ;
#20656=DIRECTION ( 'NONE',  ( 0.000000000000000000, 0.000000000000000000, 1.000000000000000000 ) ) ;
#20657=CARTESIAN_POINT ( 'NONE',  ( -83.00000337463092137, -25.98076211353322051, -5.000000000000000000 ) ) ;
#20659=VERTEX_POINT ( 'NONE', #32450 ) ;
#20660=EDGE_CURVE ( 'NONE', #3561, #31490, #6825, .T. ) ;
#20661=ORIENTED_EDGE ( 'NONE', *, *, #8517, .T. ) ;
#20662=ORIENTED_EDGE ( 'NONE', *, *, #11756, .T. ) ;
#20663=ADVANCED_FACE ( 'NONE', ( #9954 ), #27747, .F. ) ;
#20664=AXIS2_PLACEMENT_3D ( 'NONE', #5715, #19797, #2535 ) ;
#20665=EDGE_CURVE ( 'NONE', #14875, #3002, #4720, .T. ) ;
#20666=CYLINDRICAL_SURFACE ( 'NONE', #26490, 2.000000000000000000 ) ;
#20667=DIRECTION ( 'NONE',  ( 0.000000000000000000, 0.000000000000000000, 1.000000000000000000 ) ) ;
#20669=ORIENTED_EDGE ( 'NONE', *, *, #23872, .T. ) ;
#20670=EDGE_LOOP ( 'NONE', ( #25052, #28478, #11016, #5908 ) ) ;
#20671=VERTEX_POINT ( 'NONE', #33190 ) ;
#20672=AXIS2_PLACEMENT_3D ( 'NONE', #11087, #18806, #30222 ) ;
#20674=CARTESIAN_POINT ( 'NONE',  ( 62.99999662536839651, -60.62177826491080168, 12.50000000000000000 ) ) ;
#20675=VERTEX_POINT ( 'NONE', #36201 ) ;
#20676=DIRECTION ( 'NONE',  ( 0.000000000000000000, 0.000000000000000000, -1.000000000000000000 ) ) ;
#20677=ORIENTED_EDGE ( 'NONE', *, *, #23295, .T. ) ;
#20678=CYLINDRICAL_SURFACE ( 'NONE', #9369, 2.000000000000001776 ) ;
#20681=ORIENTED_EDGE ( 'NONE', *, *, #455, .F. ) ;
#20683=CARTESIAN_POINT ( 'NONE',  ( 56.67878100130369035, -27.78182860042797131, -49.86348611802629449 ) ) ;
#20685=CARTESIAN_POINT ( 'NONE',  ( -88.00000337463090716, -1.040834085586084257E-14, -9.999999999999998224 ) ) ;
#20686=ORIENTED_EDGE ( 'NONE', *, *, #22714, .T. ) ;
#20691=DIRECTION ( 'NONE',  ( 0.000000000000000000, 0.000000000000000000, 1.000000000000000000 ) ) ;
#20692=CARTESIAN_POINT ( 'NONE',  ( -78.00000337463094979, 17.32050807568878525, -9.999999999999998224 ) ) ;
#20693=AXIS2_PLACEMENT_3D ( 'NONE', #8864, #32284, #28904 ) ;
#20694=ORIENTED_EDGE ( 'NONE', *, *, #26454, .F. ) ;
#20695=DIRECTION ( 'NONE',  ( 0.000000000000000000, 0.000000000000000000, 1.000000000000000000 ) ) ;
#20697=VERTEX_POINT ( 'NONE', #24404 ) ;
#20698=CARTESIAN_POINT ( 'NONE',  ( 34.99999662536853862, 77.94228634059959404, -9.999999999999998224 ) ) ;
#20699=CIRCLE ( 'NONE', #27903, 2.000000000000000000 ) ;
#20702=AXIS2_PLACEMENT_3D ( 'NONE', #12112, #29001, #17231 ) ;
#20705=DIRECTION ( 'NONE',  ( 0.000000000000000000, 0.000000000000000000, -1.000000000000000000 ) ) ;
#20708=CIRCLE ( 'NONE', #12316, 33.00000000000001421 ) ;
#20710=FACE_OUTER_BOUND ( 'NONE', #27525, .T. ) ;
#20711=ORIENTED_EDGE ( 'NONE', *, *, #32220, .F. ) ;
#20712=CIRCLE ( 'NONE', #7557, 33.00000000000001421 ) ;
#20713=ORIENTED_EDGE ( 'NONE', *, *, #9096, .F. ) ;
#20714=VERTEX_POINT ( 'NONE', #7708 ) ;
#20715=EDGE_CURVE ( 'NONE', #6695, #10470, #21397, .T. ) ;
#20717=CARTESIAN_POINT ( 'NONE',  ( -43.19957991610399972, -47.04203867989563292, 12.49999999999999822 ) ) ;
#20718=DIRECTION ( 'NONE',  ( 0.000000000000000000, 0.000000000000000000, 1.000000000000000000 ) ) ;
#20720=DIRECTION ( 'NONE',  ( 0.000000000000000000, 0.000000000000000000, -1.000000000000000000 ) ) ;
#20722=DIRECTION ( 'NONE',  ( 1.000000000000000000, 0.000000000000000000, 0.000000000000000000 ) ) ;
#20723=ORIENTED_EDGE ( 'NONE', *, *, #35203, .F. ) ;
#20724=LINE ( 'NONE', #6117, #11922 ) ;
#20725=EDGE_LOOP ( 'NONE', ( #106, #6285 ) ) ;
#20726=FACE_BOUND ( 'NONE', #34896, .T. ) ;
#20727=CIRCLE ( 'NONE', #12940, 2.000000000000000000 ) ;
#20728=CIRCLE ( 'NONE', #36907, 2.000000000000001776 ) ;
#20730=CARTESIAN_POINT ( 'NONE',  ( -55.00000337463107059, 60.62177826491078747, -9.999999999999998224 ) ) ;
#20731=FACE_BOUND ( 'NONE', #1649, .T. ) ;
#20732=ORIENTED_EDGE ( 'NONE', *, *, #34386, .F. ) ;
#20734=EDGE_CURVE ( 'NONE', #5725, #393, #15202, .T. ) ;
#20735=EDGE_CURVE ( 'NONE', #5193, #34910, #32629, .T. ) ;
#20736=AXIS2_PLACEMENT_3D ( 'NONE', #33233, #35344, #9635 ) ;
#20737=DIRECTION ( 'NONE',  ( 0.000000000000000000, 0.000000000000000000, -1.000000000000000000 ) ) ;
#20738=CARTESIAN_POINT ( 'NONE',  ( 74.99999662536836809, 43.30127018922198801, -5.000000000000000000 ) ) ;
#20739=DIRECTION ( 'NONE',  ( -1.000000000000000000, 0.000000000000000000, 0.000000000000000000 ) ) ;
#20740=ORIENTED_EDGE ( 'NONE', *, *, #6843, .F. ) ;
#20741=CARTESIAN_POINT ( 'NONE',  ( 51.99999662536848888, -51.96152422706640550, -9.999999999999998224 ) ) ;
#20743=DIRECTION ( 'NONE',  ( 1.000000000000000000, 0.000000000000000000, 0.000000000000000000 ) ) ;
#20744=DIRECTION ( 'NONE',  ( -1.000000000000000000, 0.000000000000000000, 0.000000000000000000 ) ) ;
#20745=VERTEX_POINT ( 'NONE', #2059 ) ;
#20746=EDGE_CURVE ( 'NONE', #16300, #28642, #30189, .T. ) ;
#20747=ORIENTED_EDGE ( 'NONE', *, *, #4159, .T. ) ;
#20748=AXIS2_PLACEMENT_3D ( 'NONE', #13847, #25293, #2593 ) ;
#20751=CARTESIAN_POINT ( 'NONE',  ( -56.52018970185234537, 35.83991598322119643, 12.49999999999999822 ) ) ;
#20752=DIRECTION ( 'NONE',  ( 0.000000000000000000, 0.000000000000000000, 1.000000000000000000 ) ) ;
#20753=AXIS2_PLACEMENT_3D ( 'NONE', #20460, #28538, #31880 ) ;
#20755=AXIS2_PLACEMENT_3D ( 'NONE', #32862, #10180, #18619 ) ;
#20756=DIRECTION ( 'NONE',  ( -0.000000000000000000, -0.000000000000000000, 1.000000000000000000 ) ) ;
#20758=VERTEX_POINT ( 'NONE', #12943 ) ;
#20759=EDGE_CURVE ( 'NONE', #10548, #15799, #18405, .T. ) ;
#20760=CARTESIAN_POINT ( 'NONE',  ( 36.99999662536855283, -60.62177826491080168, -9.999999999999998224 ) ) ;
#20761=DIRECTION ( 'NONE',  ( 1.000000000000000000, 0.000000000000000000, 0.000000000000000000 ) ) ;
#20762=CARTESIAN_POINT ( 'NONE',  ( 66.98486176412667703, -43.54685190870066691, 12.50000000000000000 ) ) ;
#20763=VERTEX_POINT ( 'NONE', #15959 ) ;
#20764=AXIS2_PLACEMENT_3D ( 'NONE', #9199, #20626, #17835 ) ;
#20765=VERTEX_POINT ( 'NONE', #15592 ) ;
#20768=ORIENTED_EDGE ( 'NONE', *, *, #34386, .T. ) ;
#20770=ORIENTED_EDGE ( 'NONE', *, *, #23499, .F. ) ;
#20771=CIRCLE ( 'NONE', #14289, 95.00000000000000000 ) ;
#20772=AXIS2_PLACEMENT_3D ( 'NONE', #7270, #18705, #30861 ) ;
#20775=FACE_BOUND ( 'NONE', #21161, .T. ) ;
#20776=EDGE_LOOP ( 'NONE', ( #25701, #31673 ) ) ;
#20778=EDGE_CURVE ( 'NONE', #14526, #9610, #23603, .T. ) ;
#20779=LINE ( 'NONE', #7104, #23017 ) ;
#20780=EDGE_LOOP ( 'NONE', ( #15993, #16883 ) ) ;
#20783=DIRECTION ( 'NONE',  ( 1.000000000000000000, 0.000000000000000000, 0.000000000000000000 ) ) ;
#20787=VERTEX_POINT ( 'NONE', #33016 ) ;
#20788=ORIENTED_EDGE ( 'NONE', *, *, #36220, .F. ) ;
#20789=EDGE_CURVE ( 'NONE', #26833, #25364, #1328, .T. ) ;
#20790=AXIS2_PLACEMENT_3D ( 'NONE', #24513, #27297, #35953 ) ;
#20791=ORIENTED_EDGE ( 'NONE', *, *, #16787, .F. ) ;
#20792=VERTEX_POINT ( 'NONE', #32838 ) ;
#20793=EDGE_CURVE ( 'NONE', #24333, #25826, #35647, .T. ) ;
#20794=ORIENTED_EDGE ( 'NONE', *, *, #2176, .T. ) ;
#20795=CARTESIAN_POINT ( 'NONE',  ( -53.00000337463106348, 43.30127018922197379, 12.50000000000000000 ) ) ;
#20796=AXIS2_PLACEMENT_3D ( 'NONE', #27515, #13426, #1441 ) ;
#20797=FACE_OUTER_BOUND ( 'NONE', #15863, .T. ) ;
#20799=AXIS2_PLACEMENT_3D ( 'NONE', #11914, #19989, #23374 ) ;
#20801=CIRCLE ( 'NONE', #11227, 3.000000000000002665 ) ;
#20802=CARTESIAN_POINT ( 'NONE',  ( -70.00000337463100664, -17.32050807568882078, -9.999999999999998224 ) ) ;
#20804=ORIENTED_EDGE ( 'NONE', *, *, #5914, .F. ) ;
#20806=AXIS2_PLACEMENT_3D ( 'NONE', #5025, #5581, #10849 ) ;
#20807=DIRECTION ( 'NONE',  ( 0.000000000000000000, 0.000000000000000000, 1.000000000000000000 ) ) ;
#20808=AXIS2_PLACEMENT_3D ( 'NONE', #30033, #30410, #24620 ) ;
#20809=DIRECTION ( 'NONE',  ( 0.000000000000000000, 0.000000000000000000, 1.000000000000000000 ) ) ;
#20810=VERTEX_POINT ( 'NONE', #30014 ) ;
#20811=DIRECTION ( 'NONE',  ( 1.000000000000000000, 0.000000000000000000, 0.000000000000000000 ) ) ;
#20812=DIRECTION ( 'NONE',  ( 1.000000000000000000, 0.000000000000000000, 0.000000000000000000 ) ) ;
#20814=AXIS2_PLACEMENT_3D ( 'NONE', #2988, #11762, #5794 ) ;
#20819=DIRECTION ( 'NONE',  ( 0.000000000000000000, 0.000000000000000000, 1.000000000000000000 ) ) ;
#20820=DIRECTION ( 'NONE',  ( 0.000000000000000000, 0.000000000000000000, 1.000000000000000000 ) ) ;
#20822=EDGE_LOOP ( 'NONE', ( #28645, #18150, #10899, #18371, #34588, #16560, #6943, #31517, #770, #28046, #2129, #2097 ) ) ;
#20823=EDGE_CURVE ( 'NONE', #731, #17978, #1891, .T. ) ;
#20824=DIRECTION ( 'NONE',  ( 1.000000000000000000, 0.000000000000000000, 0.000000000000000000 ) ) ;
#20825=FACE_OUTER_BOUND ( 'NONE', #13003, .T. ) ;
#20826=AXIS2_PLACEMENT_3D ( 'NONE', #6399, #20837, #32271 ) ;
#20827=ORIENTED_EDGE ( 'NONE', *, *, #5215, .F. ) ;
#20829=AXIS2_PLACEMENT_3D ( 'NONE', #2742, #25985, #6111 ) ;
#20831=CARTESIAN_POINT ( 'NONE',  ( -65.00000337463102085, 60.62177826491077326, -9.999999999999998224 ) ) ;
#20833=AXIS2_PLACEMENT_3D ( 'NONE', #17953, #9514, #32380 ) ;
#20834=DIRECTION ( 'NONE',  ( -1.000000000000000000, 0.000000000000000000, 0.000000000000000000 ) ) ;
#20835=CARTESIAN_POINT ( 'NONE',  ( 67.99999662536838230, -17.32050807568879947, -9.999999999999998224 ) ) ;
#20836=AXIS2_PLACEMENT_3D ( 'NONE', #13893, #5294, #25886 ) ;
#20837=DIRECTION ( 'NONE',  ( 0.000000000000000000, 0.000000000000000000, 1.000000000000000000 ) ) ;
#20838=ORIENTED_EDGE ( 'NONE', *, *, #22016, .F. ) ;
#20840=DIRECTION ( 'NONE',  ( -0.8660254037844381525, 0.5000000000000009992, 0.000000000000000000 ) ) ;
#20841=CARTESIAN_POINT ( 'NONE',  ( 35.19434990244975126, -52.39915983220758022, -49.22241343995298024 ) ) ;
#20843=EDGE_CURVE ( 'NONE', #17038, #21182, #19413, .T. ) ;
#20844=ORIENTED_EDGE ( 'NONE', *, *, #8447, .T. ) ;
#20845=DIRECTION ( 'NONE',  ( 0.000000000000000000, 0.000000000000000000, 1.000000000000000000 ) ) ;
#20846=DIRECTION ( 'NONE',  ( 0.000000000000000000, 0.000000000000000000, 1.000000000000000000 ) ) ;
#20847=DIRECTION ( 'NONE',  ( 1.000000000000000000, 0.000000000000000000, 0.000000000000000000 ) ) ;
#20849=AXIS2_PLACEMENT_3D ( 'NONE', #25456, #25838, #36896 ) ;
#20851=ORIENTED_EDGE ( 'NONE', *, *, #12302, .T. ) ;
#20852=CARTESIAN_POINT ( 'NONE',  ( -77.00000337463097821, 43.30127018922197379, -9.999999999999998224 ) ) ;
#20854=CYLINDRICAL_SURFACE ( 'NONE', #1212, 2.000000000000001776 ) ;
#20856=CARTESIAN_POINT ( 'NONE',  ( -73.00000337463097821, 25.98076211353318854, -9.999999999999998224 ) ) ;
#20857=ORIENTED_EDGE ( 'NONE', *, *, #31569, .F. ) ;
#20858=FACE_OUTER_BOUND ( 'NONE', #922, .T. ) ;
#20861=CARTESIAN_POINT ( 'NONE',  ( 31.99999662536857770, -69.28203230275519786, -9.999999999999998224 ) ) ;
#20862=AXIS2_PLACEMENT_3D ( 'NONE', #10623, #2174, #13810 ) ;
#20863=ORIENTED_EDGE ( 'NONE', *, *, #35904, .F. ) ;
#20864=ORIENTED_EDGE ( 'NONE', *, *, #5534, .T. ) ;
#20865=ADVANCED_FACE ( 'NONE', ( #13698 ), #33950, .T. ) ;
#20868=DIRECTION ( 'NONE',  ( 0.000000000000000000, 0.000000000000000000, 1.000000000000000000 ) ) ;
#20869=FACE_OUTER_BOUND ( 'NONE', #28845, .T. ) ;
#20870=EDGE_CURVE ( 'NONE', #30055, #6269, #15224, .T. ) ;
#20873=ORIENTED_EDGE ( 'NONE', *, *, #19034, .T. ) ;
#20874=ORIENTED_EDGE ( 'NONE', *, *, #35635, .F. ) ;
#20876=ADVANCED_FACE ( 'NONE', ( #22694 ), #5068, .T. ) ;
#20878=VERTEX_POINT ( 'NONE', #22318 ) ;
#20879=CARTESIAN_POINT ( 'NONE',  ( 31.99999662536857770, -69.28203230275519786, -5.000000000000000000 ) ) ;
#20882=CARTESIAN_POINT ( 'NONE',  ( -57.00000337463107059, 60.62177826491078747, -9.999999999999998224 ) ) ;
#20883=ORIENTED_EDGE ( 'NONE', *, *, #25021, .F. ) ;
#20884=EDGE_CURVE ( 'NONE', #31631, #31383, #20589, .T. ) ;
#20885=EDGE_LOOP ( 'NONE', ( #21149, #36757, #31946, #23672 ) ) ;
#20887=CARTESIAN_POINT ( 'NONE',  ( 79.99999662536832545, -17.32050807568879591, -5.000000000000000000 ) ) ;
#20889=CARTESIAN_POINT ( 'NONE',  ( 52.99999662536844625, 60.62177826491077326, -5.000000000000000000 ) ) ;
#20890=EDGE_LOOP ( 'NONE', ( #16486, #34981, #30194, #31715 ) ) ;
#20892=CARTESIAN_POINT ( 'NONE',  ( 67.99999662536836809, -34.64101615137759183, -9.999999999999998224 ) ) ;
#20893=AXIS2_PLACEMENT_3D ( 'NONE', #21246, #15453, #9810 ) ;
#20894=DIRECTION ( 'NONE',  ( 0.000000000000000000, 0.000000000000000000, -1.000000000000000000 ) ) ;
#20896=CARTESIAN_POINT ( 'NONE',  ( -20.00000337463123756, -86.60254037844400443, -9.999999999999998224 ) ) ;
#20898=DIRECTION ( 'NONE',  ( -1.000000000000000000, 0.000000000000000000, 0.000000000000000000 ) ) ;
#20899=ADVANCED_FACE ( 'NONE', ( #22146 ), #22496, .F. ) ;
#20900=ORIENTED_EDGE ( 'NONE', *, *, #5191, .F. ) ;
#20901=LINE ( 'NONE', #11890, #35114 ) ;
#20903=EDGE_CURVE ( 'NONE', #6546, #21552, #3876, .T. ) ;
#20904=AXIS2_PLACEMENT_3D ( 'NONE', #29116, #3451, #26323 ) ;
#20906=DIRECTION ( 'NONE',  ( 0.000000000000000000, 0.000000000000000000, 1.000000000000000000 ) ) ;
#20907=EDGE_CURVE ( 'NONE', #1764, #11378, #25318, .T. ) ;
#20908=DIRECTION ( 'NONE',  ( -1.000000000000000000, 0.000000000000000000, 0.000000000000000000 ) ) ;
#20909=FACE_OUTER_BOUND ( 'NONE', #32872, .T. ) ;
#20910=VECTOR ( 'NONE', #27377, 1000.000000000000000 ) ;
#20911=CARTESIAN_POINT ( 'NONE',  ( 84.99999662536831124, -8.660254037844397956, -5.000000000000000000 ) ) ;
#20912=CIRCLE ( 'NONE', #4756, 2.000000000000001776 ) ;
#20914=FACE_OUTER_BOUND ( 'NONE', #11975, .T. ) ;
#20915=CIRCLE ( 'NONE', #4758, 3.000000000000007105 ) ;
#20916=ORIENTED_EDGE ( 'NONE', *, *, #28258, .F. ) ;
#20917=CARTESIAN_POINT ( 'NONE',  ( -58.00000337463104216, 34.64101615137757051, -9.999999999999998224 ) ) ;
#20919=CARTESIAN_POINT ( 'NONE',  ( -67.00000337463102085, 60.62177826491077326, -5.000000000000000000 ) ) ;
#20920=EDGE_LOOP ( 'NONE', ( #23372, #34544 ) ) ;
#20921=VERTEX_POINT ( 'NONE', #5452 ) ;
#20923=CIRCLE ( 'NONE', #28701, 2.000000000000001776 ) ;
#20924=CARTESIAN_POINT ( 'NONE',  ( -65.00000337463104927, -43.30127018922202353, -9.999999999999998224 ) ) ;
#20925=CARTESIAN_POINT ( 'NONE',  ( 9.999996625368655856, -69.28203230275519786, -9.999999999999998224 ) ) ;
#20926=AXIS2_PLACEMENT_3D ( 'NONE', #26418, #9347, #15158 ) ;
#20928=CARTESIAN_POINT ( 'NONE',  ( 0.000000000000000000, 0.000000000000000000, 12.49999999999999822 ) ) ;
#20929=DIRECTION ( 'NONE',  ( 1.000000000000000000, 0.000000000000000000, 0.000000000000000000 ) ) ;
#20930=ORIENTED_EDGE ( 'NONE', *, *, #30865, .F. ) ;
#20932=DIRECTION ( 'NONE',  ( -1.000000000000000000, 0.000000000000000000, 0.000000000000000000 ) ) ;
#20933=EDGE_LOOP ( 'NONE', ( #6136, #17196 ) ) ;
#20934=FACE_BOUND ( 'NONE', #11132, .T. ) ;
#20935=AXIS2_PLACEMENT_3D ( 'NONE', #10055, #27099, #7608 ) ;
#20937=CARTESIAN_POINT ( 'NONE',  ( -18.00000337463124467, 69.28203230275516944, -5.000000000000000000 ) ) ;
#20939=PLANE ( 'NONE',  #15270 ) ;
#20942=CARTESIAN_POINT ( 'NONE',  ( -13.89091430021420237, -62.33939050065180254, 12.49999999999999822 ) ) ;
#20943=CIRCLE ( 'NONE', #13778, 3.499999999999989342 ) ;
#20944=LINE ( 'NONE', #26937, #27533 ) ;
#20946=ADVANCED_FACE ( 'NONE', ( #14048 ), #25497, .F. ) ;
#20947=EDGE_LOOP ( 'NONE', ( #28767, #2584 ) ) ;
#20948=LINE ( 'NONE', #23563, #30383 ) ;
#20949=CIRCLE ( 'NONE', #29315, 3.000000000000006217 ) ;
#20950=CARTESIAN_POINT ( 'NONE',  ( 44.99999662536849598, 60.62177826491077326, -5.000000000000000000 ) ) ;
#20951=DIRECTION ( 'NONE',  ( 1.000000000000000000, 0.000000000000000000, 0.000000000000000000 ) ) ;
#20952=EDGE_LOOP ( 'NONE', ( #19434, #1292 ) ) ;
#20953=EDGE_LOOP ( 'NONE', ( #22959, #35037 ) ) ;
#20954=VERTEX_POINT ( 'NONE', #2817 ) ;
#20956=CARTESIAN_POINT ( 'NONE',  ( -70.00000337463099243, 51.96152422706637708, -9.999999999999998224 ) ) ;
#20958=AXIS2_PLACEMENT_3D ( 'NONE', #10935, #2333, #16772 ) ;
#20960=DIRECTION ( 'NONE',  ( -1.000000000000000000, 0.000000000000000000, 0.000000000000000000 ) ) ;
#20961=AXIS2_PLACEMENT_3D ( 'NONE', #36366, #25122, #25290 ) ;
#20962=DIRECTION ( 'NONE',  ( 1.000000000000000000, 0.000000000000000000, 0.000000000000000000 ) ) ;
#20964=ORIENTED_EDGE ( 'NONE', *, *, #31020, .T. ) ;
#20965=ORIENTED_EDGE ( 'NONE', *, *, #4492, .T. ) ;
#20967=VECTOR ( 'NONE', #8540, 1000.000000000000000 ) ;
#20968=DIRECTION ( 'NONE',  ( 0.000000000000000000, 0.000000000000000000, -1.000000000000000000 ) ) ;
#20971=ORIENTED_EDGE ( 'NONE', *, *, #12053, .F. ) ;
#20973=FACE_BOUND ( 'NONE', #12820, .T. ) ;
#20974=ORIENTED_EDGE ( 'NONE', *, *, #36343, .T. ) ;
#20975=ORIENTED_EDGE ( 'NONE', *, *, #21903, .F. ) ;
#20976=VECTOR ( 'NONE', #23669, 1000.000000000000000 ) ;
#20977=CARTESIAN_POINT ( 'NONE',  ( -48.00000337463109190, 69.28203230275518365, -9.999999999999998224 ) ) ;
#20978=VERTEX_POINT ( 'NONE', #11428 ) ;
#20979=FACE_OUTER_BOUND ( 'NONE', #10058, .T. ) ;
#20980=DIRECTION ( 'NONE',  ( -1.000000000000000000, -1.798972493605576793E-15, 0.000000000000000000 ) ) ;
#20981=CARTESIAN_POINT ( 'NONE',  ( 76.99999662536835388, -43.30127018922199511, -9.999999999999998224 ) ) ;
#20982=CIRCLE ( 'NONE', #27579, 3.000000000000002665 ) ;
#20983=ADVANCED_FACE ( 'NONE', ( #34310 ), #22873, .F. ) ;
#20984=EDGE_LOOP ( 'NONE', ( #36874, #19855, #889, #8026 ) ) ;
#20985=ORIENTED_EDGE ( 'NONE', *, *, #16995, .T. ) ;
#20986=AXIS2_PLACEMENT_3D ( 'NONE', #30712, #10294, #16471 ) ;
#20990=DIRECTION ( 'NONE',  ( -1.000000000000000000, 0.000000000000000000, 0.000000000000000000 ) ) ;
#20991=CARTESIAN_POINT ( 'NONE',  ( 44.99999662536851019, -60.62177826491080168, 17.49999999999999645 ) ) ;
#20992=EDGE_LOOP ( 'NONE', ( #26313, #34070 ) ) ;
#20993=DIRECTION ( 'NONE',  ( 0.000000000000000000, 0.000000000000000000, -1.000000000000000000 ) ) ;
#20995=CYLINDRICAL_SURFACE ( 'NONE', #24951, 2.000000000000001776 ) ;
#20996=VERTEX_POINT ( 'NONE', #15157 ) ;
#20997=DIRECTION ( 'NONE',  ( 0.000000000000000000, 0.000000000000000000, 1.000000000000000000 ) ) ;
#20998=FACE_OUTER_BOUND ( 'NONE', #22213, .T. ) ;
#21000=CARTESIAN_POINT ( 'NONE',  ( 68.19434990244977257, -52.39915983220758022, 12.49999999999999822 ) ) ;
#21001=ORIENTED_EDGE ( 'NONE', *, *, #19962, .T. ) ;
#21003=CYLINDRICAL_SURFACE ( 'NONE', #24394, 2.000000000000001776 ) ;
#21004=EDGE_CURVE ( 'NONE', #7750, #35055, #24829, .T. ) ;
#21006=ORIENTED_EDGE ( 'NONE', *, *, #27853, .T. ) ;
#21007=CARTESIAN_POINT ( 'NONE',  ( -43.00000337463111322, 60.62177826491077326, 12.50000000000000000 ) ) ;
#21008=CARTESIAN_POINT ( 'NONE',  ( -72.00000337463100664, 51.96152422706637708, -5.000000000000000000 ) ) ;
#21009=AXIS2_PLACEMENT_3D ( 'NONE', #13849, #8236, #33367 ) ;
#21010=CARTESIAN_POINT ( 'NONE',  ( 74.99999662536836809, 8.660254037844394404, -9.999999999999998224 ) ) ;
#21013=ORIENTED_EDGE ( 'NONE', *, *, #35465, .F. ) ;
#21014=CYLINDRICAL_SURFACE ( 'NONE', #15354, 2.000000000000001776 ) ;
#21017=VERTEX_POINT ( 'NONE', #903 ) ;
#21018=CARTESIAN_POINT ( 'NONE',  ( -58.00000337463108480, -51.96152422706641971, 17.49999999999999645 ) ) ;
#21019=ORIENTED_EDGE ( 'NONE', *, *, #9178, .F. ) ;
#21020=CARTESIAN_POINT ( 'NONE',  ( 35.19434990244975126, -52.39915983220758022, 12.49999999999999822 ) ) ;
#21021=DIRECTION ( 'NONE',  ( 0.000000000000000000, 0.000000000000000000, -1.000000000000000000 ) ) ;
#21022=DIRECTION ( 'NONE',  ( -1.000000000000000000, 0.000000000000000000, 0.000000000000000000 ) ) ;
#21023=ORIENTED_EDGE ( 'NONE', *, *, #34118, .T. ) ;
#21024=ORIENTED_EDGE ( 'NONE', *, *, #16368, .T. ) ;
#21025=AXIS2_PLACEMENT_3D ( 'NONE', #18941, #1697, #4504 ) ;
#21026=DIRECTION ( 'NONE',  ( -0.000000000000000000, -0.000000000000000000, 1.000000000000000000 ) ) ;
#21028=EDGE_LOOP ( 'NONE', ( #22715, #29773, #4348, #33486, #24217 ) ) ;
#21030=FACE_BOUND ( 'NONE', #7747, .T. ) ;
#21031=DIRECTION ( 'NONE',  ( 0.000000000000000000, 0.000000000000000000, 1.000000000000000000 ) ) ;
#21032=CARTESIAN_POINT ( 'NONE',  ( 82.99999662536832545, 8.660254037844394404, 17.49999999999999645 ) ) ;
#21033=DIRECTION ( 'NONE',  ( 0.000000000000000000, 0.000000000000000000, 1.000000000000000000 ) ) ;
#21034=ORIENTED_EDGE ( 'NONE', *, *, #31276, .F. ) ;
#21035=LINE ( 'NONE', #20852, #35056 ) ;
#21036=ADVANCED_FACE ( 'NONE', ( #20979 ), #6162, .F. ) ;
#21038=EDGE_CURVE ( 'NONE', #35651, #12099, #9547, .T. ) ;
#21039=CARTESIAN_POINT ( 'NONE',  ( 9.999996625368655856, -69.28203230275519786, 12.50000000000000000 ) ) ;
#21040=ORIENTED_EDGE ( 'NONE', *, *, #21621, .F. ) ;
#21041=DIRECTION ( 'NONE',  ( -1.000000000000000000, 0.000000000000000000, 0.000000000000000000 ) ) ;
#21042=DIRECTION ( 'NONE',  ( 0.000000000000000000, 0.000000000000000000, -1.000000000000000000 ) ) ;
#21043=DIRECTION ( 'NONE',  ( -1.000000000000000000, 0.000000000000000000, 0.000000000000000000 ) ) ;
#21044=VERTEX_POINT ( 'NONE', #31667 ) ;
#21045=ORIENTED_EDGE ( 'NONE', *, *, #9196, .T. ) ;
#21046=CIRCLE ( 'NONE', #24055, 2.000000000000001776 ) ;
#21047=DIRECTION ( 'NONE',  ( 1.000000000000000000, 0.000000000000000000, 0.000000000000000000 ) ) ;
#21048=DIRECTION ( 'NONE',  ( 1.000000000000000000, 0.000000000000000000, 0.000000000000000000 ) ) ;
#21050=ORIENTED_EDGE ( 'NONE', *, *, #13967, .T. ) ;
#21051=CIRCLE ( 'NONE', #16281, 33.00000000000001421 ) ;
#21053=ORIENTED_EDGE ( 'NONE', *, *, #25592, .T. ) ;
#21054=DIRECTION ( 'NONE',  ( 0.000000000000000000, 0.000000000000000000, 1.000000000000000000 ) ) ;
#21055=ADVANCED_FACE ( 'NONE', ( #9346 ), #12324, .F. ) ;
#21057=ORIENTED_EDGE ( 'NONE', *, *, #19124, .F. ) ;
#21058=DIRECTION ( 'NONE',  ( -0.000000000000000000, -0.000000000000000000, 1.000000000000000000 ) ) ;
#21059=VERTEX_POINT ( 'NONE', #161 ) ;
#21060=ORIENTED_EDGE ( 'NONE', *, *, #9445, .F. ) ;
#21061=SHAPE_REPRESENTATION_RELATIONSHIP ( 'NONE' , 'NONE' ,  #26771, #20178 ) ;
#21062=PLANE ( 'NONE',  #5843 ) ;
#21063=LINE ( 'NONE', #3811, #8094 ) ;
#21064=ORIENTED_EDGE ( 'NONE', *, *, #11420, .T. ) ;
#21066=DIRECTION ( 'NONE',  ( 1.000000000000000000, 0.000000000000000000, 0.000000000000000000 ) ) ;
#21067=DIRECTION ( 'NONE',  ( 0.000000000000000000, 0.000000000000000000, 1.000000000000000000 ) ) ;
#21068=DIRECTION ( 'NONE',  ( 1.000000000000000000, 0.000000000000000000, 0.000000000000000000 ) ) ;
#21069=CARTESIAN_POINT ( 'NONE',  ( 76.99999662536836809, 8.660254037844394404, 17.49999999999999645 ) ) ;
#21070=EDGE_CURVE ( 'NONE', #14210, #21598, #5678, .T. ) ;
#21071=ORIENTED_EDGE ( 'NONE', *, *, #29083, .T. ) ;
#21072=CARTESIAN_POINT ( 'NONE',  ( -83.49774789488644444, 24.66044833507834610, -5.000000000000000000 ) ) ;
#21074=CIRCLE ( 'NONE', #13900, 2.000000000000001776 ) ;
#21076=EDGE_CURVE ( 'NONE', #24584, #10304, #31415, .T. ) ;
#21077=DIRECTION ( 'NONE',  ( -1.000000000000000000, -8.737866397512800437E-15, 0.000000000000000000 ) ) ;
#21078=FACE_OUTER_BOUND ( 'NONE', #34358, .T. ) ;
#21079=DIRECTION ( 'NONE',  ( 0.000000000000000000, 0.000000000000000000, 1.000000000000000000 ) ) ;
#21080=DIRECTION ( 'NONE',  ( 0.000000000000000000, 0.000000000000000000, 1.000000000000000000 ) ) ;
#21082=CARTESIAN_POINT ( 'NONE',  ( 39.99999662536853151, 69.28203230275518365, -9.999999999999998224 ) ) ;
#21083=EDGE_CURVE ( 'NONE', #9125, #12353, #9253, .T. ) ;
#21085=ORIENTED_EDGE ( 'NONE', *, *, #17225, .F. ) ;
#21086=CARTESIAN_POINT ( 'NONE',  ( 66.99999662536839651, -43.30127018922199511, -5.000000000000000000 ) ) ;
#21087=EDGE_CURVE ( 'NONE', #5560, #32910, #9847, .T. ) ;
#21090=EDGE_CURVE ( 'NONE', #27516, #2053, #35615, .T. ) ;
#21091=ORIENTED_EDGE ( 'NONE', *, *, #4326, .T. ) ;
#21092=ORIENTED_EDGE ( 'NONE', *, *, #28214, .T. ) ;
#21093=ORIENTED_EDGE ( 'NONE', *, *, #28684, .T. ) ;
#21094=DIRECTION ( 'NONE',  ( 0.000000000000000000, 0.000000000000000000, -1.000000000000000000 ) ) ;
#21095=CARTESIAN_POINT ( 'NONE',  ( 36.99999662536855283, 60.62177826491078747, -9.999999999999998224 ) ) ;
#21096=LINE ( 'NONE', #12259, #310 ) ;
#21097=ADVANCED_FACE ( 'NONE', ( #29022 ), #6346, .F. ) ;
#21098=EDGE_CURVE ( 'NONE', #10841, #31248, #12229, .T. ) ;
#21102=CARTESIAN_POINT ( 'NONE',  ( 9.999996625368655856, -86.60254037844400443, 12.50000000000000000 ) ) ;
#21103=ORIENTED_EDGE ( 'NONE', *, *, #28855, .T. ) ;
#21104=DIRECTION ( 'NONE',  ( 0.000000000000000000, 0.000000000000000000, 1.000000000000000000 ) ) ;
#21106=FACE_BOUND ( 'NONE', #7752, .T. ) ;
#21107=DIRECTION ( 'NONE',  ( 0.000000000000000000, 0.000000000000000000, 1.000000000000000000 ) ) ;
#21108=DIRECTION ( 'NONE',  ( 0.000000000000000000, 0.000000000000000000, 1.000000000000000000 ) ) ;
#21109=CARTESIAN_POINT ( 'NONE',  ( 49.99999662536848177, -51.96152422706640550, 12.50000000000000000 ) ) ;
#21111=LINE ( 'NONE', #17743, #35627 ) ;
#21113=DIRECTION ( 'NONE',  ( -0.000000000000000000, -0.000000000000000000, -1.000000000000000000 ) ) ;
#21114=CIRCLE ( 'NONE', #25908, 2.000000000000001776 ) ;
#21115=EDGE_CURVE ( 'NONE', #34695, #34700, #14631, .T. ) ;
#21116=FACE_OUTER_BOUND ( 'NONE', #11401, .T. ) ;
#21117=DIRECTION ( 'NONE',  ( 0.000000000000000000, 0.000000000000000000, 1.000000000000000000 ) ) ;
#21118=ORIENTED_EDGE ( 'NONE', *, *, #16812, .T. ) ;
#21120=CARTESIAN_POINT ( 'NONE',  ( -55.00000337463109901, -60.62177826491083010, -5.000000000000000000 ) ) ;
#21123=ORIENTED_EDGE ( 'NONE', *, *, #20457, .F. ) ;
#21124=ORIENTED_EDGE ( 'NONE', *, *, #15294, .T. ) ;
#21125=VECTOR ( 'NONE', #14015, 1000.000000000000000 ) ;
#21126=ORIENTED_EDGE ( 'NONE', *, *, #34380, .T. ) ;
#21129=CARTESIAN_POINT ( 'NONE',  ( 77.99999662536832545, -34.64101615137759183, 17.49999999999999645 ) ) ;
#21130=DIRECTION ( 'NONE',  ( -0.000000000000000000, 0.000000000000000000, -1.000000000000000000 ) ) ;
#21131=DIRECTION ( 'NONE',  ( 0.000000000000000000, 0.000000000000000000, 1.000000000000000000 ) ) ;
#21132=PLANE ( 'NONE',  #19406 ) ;
#21133=DIRECTION ( 'NONE',  ( 1.000000000000000000, 0.000000000000000000, 0.000000000000000000 ) ) ;
#21134=CIRCLE ( 'NONE', #36722, 3.499999999999996003 ) ;
#21135=DIRECTION ( 'NONE',  ( 0.000000000000000000, 0.000000000000000000, 1.000000000000000000 ) ) ;
#21136=EDGE_CURVE ( 'NONE', #19500, #25394, #28994, .T. ) ;
#21138=EDGE_CURVE ( 'NONE', #34583, #17059, #30799, .T. ) ;
#21140=AXIS2_PLACEMENT_3D ( 'NONE', #12563, #21185, #24017 ) ;
#21141=DIRECTION ( 'NONE',  ( 0.000000000000000000, 0.000000000000000000, 1.000000000000000000 ) ) ;
#21143=CARTESIAN_POINT ( 'NONE',  ( 39.99999662536853151, -69.28203230275519786, -5.000000000000000000 ) ) ;
#21144=ORIENTED_EDGE ( 'NONE', *, *, #5992, .F. ) ;
#21146=PLANE ( 'NONE',  #18532 ) ;
#21147=VERTEX_POINT ( 'NONE', #18908 ) ;
#21148=FACE_BOUND ( 'NONE', #18312, .T. ) ;
#21149=ORIENTED_EDGE ( 'NONE', *, *, #16907, .F. ) ;
#21150=AXIS2_PLACEMENT_3D ( 'NONE', #19932, #8503, #20116 ) ;
#21152=CYLINDRICAL_SURFACE ( 'NONE', #11628, 2.000000000000001776 ) ;
#21153=ORIENTED_EDGE ( 'NONE', *, *, #25592, .F. ) ;
#21155=CARTESIAN_POINT ( 'NONE',  ( 22.99999662536859901, -77.94228634059960825, -9.999999999999998224 ) ) ;
#21158=EDGE_LOOP ( 'NONE', ( #5459, #15739 ) ) ;
#21159=ORIENTED_EDGE ( 'NONE', *, *, #1313, .F. ) ;
#21160=CIRCLE ( 'NONE', #19377, 2.000000000000001776 ) ;
#21161=EDGE_LOOP ( 'NONE', ( #28245, #20035 ) ) ;
#21162=EDGE_CURVE ( 'NONE', #10635, #5101, #15854, .T. ) ;
#21163=ORIENTED_EDGE ( 'NONE', *, *, #25784, .T. ) ;
#21164=AXIS2_PLACEMENT_3D ( 'NONE', #21935, #33379, #17773 ) ;
#21168=VERTEX_POINT ( 'NONE', #15344 ) ;
#21171=DIRECTION ( 'NONE',  ( 1.000000000000000000, 0.000000000000000000, 0.000000000000000000 ) ) ;
#21172=ORIENTED_EDGE ( 'NONE', *, *, #6778, .T. ) ;
#21174=VECTOR ( 'NONE', #10607, 1000.000000000000000 ) ;
#21175=DIRECTION ( 'NONE',  ( 0.000000000000000000, 0.000000000000000000, 1.000000000000000000 ) ) ;
#21176=AXIS2_PLACEMENT_3D ( 'NONE', #14450, #25521, #34713 ) ;
#21177=CARTESIAN_POINT ( 'NONE',  ( -72.00000337463100664, 17.32050807568877460, -9.999999999999998224 ) ) ;
#21178=ORIENTED_EDGE ( 'NONE', *, *, #10307, .F. ) ;
#21180=DIRECTION ( 'NONE',  ( 0.000000000000000000, 0.000000000000000000, 1.000000000000000000 ) ) ;
#21181=VECTOR ( 'NONE', #28789, 1000.000000000000000 ) ;
#21182=VERTEX_POINT ( 'NONE', #1847 ) ;
#21183=ORIENTED_EDGE ( 'NONE', *, *, #29747, .T. ) ;
#21184=DIRECTION ( 'NONE',  ( 0.000000000000000000, 0.000000000000000000, 1.000000000000000000 ) ) ;
#21185=DIRECTION ( 'NONE',  ( -0.000000000000000000, 0.000000000000000000, -1.000000000000000000 ) ) ;
#21186=EDGE_CURVE ( 'NONE', #14195, #4901, #3266, .T. ) ;
#21187=CARTESIAN_POINT ( 'NONE',  ( -40.00000337463113453, 69.28203230275516944, -5.000000000000000000 ) ) ;
#21188=FACE_OUTER_BOUND ( 'NONE', #92, .T. ) ;
#21189=EDGE_LOOP ( 'NONE', ( #31835, #28865, #3734, #1587 ) ) ;
#21190=CARTESIAN_POINT ( 'NONE',  ( 4.999996625368676284, -77.94228634059960825, -5.000000000000000000 ) ) ;
#21191=CYLINDRICAL_SURFACE ( 'NONE', #32696, 95.00000000000001421 ) ;
#21192=AXIS2_PLACEMENT_3D ( 'NONE', #1264, #27311, #9705 ) ;
#21194=CYLINDRICAL_SURFACE ( 'NONE', #9395, 2.000000000000001776 ) ;
#21195=ORIENTED_EDGE ( 'NONE', *, *, #12075, .F. ) ;
#21196=CARTESIAN_POINT ( 'NONE',  ( -72.00000337463102085, -51.96152422706641971, -9.999999999999998224 ) ) ;
#21197=CARTESIAN_POINT ( 'NONE',  ( -82.00000337463094979, -17.32050807568882078, -9.999999999999998224 ) ) ;
#21198=AXIS2_PLACEMENT_3D ( 'NONE', #30166, #1688, #13123 ) ;
#21201=ORIENTED_EDGE ( 'NONE', *, *, #6688, .F. ) ;
#21202=EDGE_CURVE ( 'NONE', #12455, #10468, #1467, .T. ) ;
#21203=ORIENTED_EDGE ( 'NONE', *, *, #10096, .F. ) ;
#21204=DIRECTION ( 'NONE',  ( -1.000000000000000000, 0.000000000000000000, 0.000000000000000000 ) ) ;
#21205=CARTESIAN_POINT ( 'NONE',  ( 65.63757102168601421, 58.72612563608866765, 12.50000000000000000 ) ) ;
#21206=EDGE_CURVE ( 'NONE', #34302, #11641, #22429, .T. ) ;
#21207=DIRECTION ( 'NONE',  ( -0.8660254037844453689, -0.4999999999999882871, 0.000000000000000000 ) ) ;
#21208=CARTESIAN_POINT ( 'NONE',  ( -60.00000337463104216, 51.96152422706639129, 17.49999999999999645 ) ) ;
#21209=DIRECTION ( 'NONE',  ( 0.000000000000000000, 0.000000000000000000, 1.000000000000000000 ) ) ;
#21210=EDGE_LOOP ( 'NONE', ( #2385, #21352, #899, #24663 ) ) ;
#21212=AXIS2_PLACEMENT_3D ( 'NONE', #19349, #26720, #32915 ) ;
#21213=DIRECTION ( 'NONE',  ( 1.000000000000000000, 0.000000000000000000, 0.000000000000000000 ) ) ;
#21214=ADVANCED_FACE ( 'NONE', ( #36157 ), #9721, .F. ) ;
#21215=CARTESIAN_POINT ( 'NONE',  ( -78.00000337463094979, -2.428612866367529932E-14, -5.000000000000000000 ) ) ;
#21216=ORIENTED_EDGE ( 'NONE', *, *, #4171, .T. ) ;
#21219=CARTESIAN_POINT ( 'NONE',  ( 62.99999662536841072, 25.98076211353318854, -9.999999999999998224 ) ) ;
#21222=AXIS2_PLACEMENT_3D ( 'NONE', #4894, #36393, #10703 ) ;
#21223=ORIENTED_EDGE ( 'NONE', *, *, #9133, .F. ) ;
#21224=AXIS2_PLACEMENT_3D ( 'NONE', #11990, #9175, #29604 ) ;
#21225=DIRECTION ( 'NONE',  ( 1.000000000000000000, 0.000000000000000000, 0.000000000000000000 ) ) ;
#21226=EDGE_CURVE ( 'NONE', #13437, #33271, #21712, .T. ) ;
#21227=CARTESIAN_POINT ( 'NONE',  ( -80.00000337463094979, 34.64101615137757051, -9.999999999999998224 ) ) ;
#21229=ORIENTED_EDGE ( 'NONE', *, *, #17151, .T. ) ;
#21233=AXIS2_PLACEMENT_3D ( 'NONE', #1303, #29991, #12718 ) ;
#21234=ORIENTED_EDGE ( 'NONE', *, *, #8629, .F. ) ;
#21235=VERTEX_POINT ( 'NONE', #35800 ) ;
#21237=ORIENTED_EDGE ( 'NONE', *, *, #19426, .F. ) ;
#21238=VERTEX_POINT ( 'NONE', #33145 ) ;
#21239=ADVANCED_FACE ( 'NONE', ( #13098 ), #21541, .T. ) ;
#21240=AXIS2_PLACEMENT_3D ( 'NONE', #3038, #11452, #25728 ) ;
#21241=DIRECTION ( 'NONE',  ( 0.000000000000000000, 0.000000000000000000, 1.000000000000000000 ) ) ;
#21242=EDGE_CURVE ( 'NONE', #10050, #7613, #17049, .T. ) ;
#21244=ORIENTED_EDGE ( 'NONE', *, *, #22097, .T. ) ;
#21246=CARTESIAN_POINT ( 'NONE',  ( 19.99999662536861678, -86.60254037844400443, -9.999999999999998224 ) ) ;
#21247=CARTESIAN_POINT ( 'NONE',  ( 72.99999662536836809, 8.660254037844394404, -9.999999999999998224 ) ) ;
#21248=AXIS2_PLACEMENT_3D ( 'NONE', #8404, #19834, #23005 ) ;
#21249=EDGE_CURVE ( 'NONE', #31238, #35117, #13835, .T. ) ;
#21250=CARTESIAN_POINT ( 'NONE',  ( -32.00000337463119848, -69.28203230275522628, 17.49999999999999645 ) ) ;
#21251=LINE ( 'NONE', #32687, #33475 ) ;
#21253=CARTESIAN_POINT ( 'NONE',  ( 72.99999662536836809, -8.660254037844401509, -9.999999999999998224 ) ) ;
#21254=ORIENTED_EDGE ( 'NONE', *, *, #23035, .T. ) ;
#21256=ADVANCED_FACE ( 'NONE', ( #8214 ), #27888, .F. ) ;
#21257=DIRECTION ( 'NONE',  ( 0.000000000000000000, 0.000000000000000000, 1.000000000000000000 ) ) ;
#21258=DIRECTION ( 'NONE',  ( 1.000000000000000000, 0.000000000000000000, 0.000000000000000000 ) ) ;
#21259=DIRECTION ( 'NONE',  ( 1.000000000000000000, 0.000000000000000000, 0.000000000000000000 ) ) ;
#21261=EDGE_CURVE ( 'NONE', #1919, #36051, #28417, .T. ) ;
#21263=DIRECTION ( 'NONE',  ( 0.000000000000000000, 0.000000000000000000, 1.000000000000000000 ) ) ;
#21264=VERTEX_POINT ( 'NONE', #2211 ) ;
#21265=LINE ( 'NONE', #6831, #18413 ) ;
#21266=CIRCLE ( 'NONE', #13472, 2.000000000000001776 ) ;
#21267=CARTESIAN_POINT ( 'NONE',  ( -52.00000337463109190, 69.28203230275518365, -9.999999999999998224 ) ) ;
#21268=DIRECTION ( 'NONE',  ( 0.000000000000000000, 0.000000000000000000, 1.000000000000000000 ) ) ;
#21269=VECTOR ( 'NONE', #10647, 1000.000000000000000 ) ;
#21270=ORIENTED_EDGE ( 'NONE', *, *, #13040, .F. ) ;
#21271=AXIS2_PLACEMENT_3D ( 'NONE', #11960, #34681, #29395 ) ;
#21273=ORIENTED_EDGE ( 'NONE', *, *, #28990, .F. ) ;
#21275=CARTESIAN_POINT ( 'NONE',  ( -52.00000337463112032, -51.96152422706641971, -5.000000000000000000 ) ) ;
#21277=VERTEX_POINT ( 'NONE', #34098 ) ;
#21278=CIRCLE ( 'NONE', #5120, 3.499999999999989342 ) ;
#21279=CIRCLE ( 'NONE', #24281, 2.000000000000000000 ) ;
#21281=ADVANCED_FACE ( 'NONE', ( #5575 ), #27700, .F. ) ;
#21282=DIRECTION ( 'NONE',  ( 1.000000000000000000, 0.000000000000000000, 0.000000000000000000 ) ) ;
#21283=EDGE_LOOP ( 'NONE', ( #21573, #14798, #15024, #22962 ) ) ;
#21286=CARTESIAN_POINT ( 'NONE',  ( 76.99999662536836809, 25.98076211353319565, 17.49999999999999645 ) ) ;
#21288=CARTESIAN_POINT ( 'NONE',  ( -22.00000337463122690, 86.60254037844397601, 12.50000000000000000 ) ) ;
#21290=CIRCLE ( 'NONE', #11724, 2.000000000000001776 ) ;
#21291=EDGE_CURVE ( 'NONE', #34992, #4407, #5708, .T. ) ;
#21292=LINE ( 'NONE', #32733, #3212 ) ;
#21293=AXIS2_PLACEMENT_3D ( 'NONE', #22205, #28189, #22373 ) ;
#21294=ORIENTED_EDGE ( 'NONE', *, *, #34929, .F. ) ;
#21295=CARTESIAN_POINT ( 'NONE',  ( 22.99999662536859901, -77.94228634059960825, -5.000000000000000000 ) ) ;
#21297=VECTOR ( 'NONE', #10359, 1000.000000000000000 ) ;
#21298=AXIS2_PLACEMENT_3D ( 'NONE', #11916, #26367, #31610 ) ;
#21299=AXIS2_PLACEMENT_3D ( 'NONE', #13261, #35779, #27323 ) ;
#21300=DIRECTION ( 'NONE',  ( 1.000000000000000000, 0.000000000000000000, 0.000000000000000000 ) ) ;
#21301=FACE_OUTER_BOUND ( 'NONE', #28787, .T. ) ;
#21303=VERTEX_POINT ( 'NONE', #2768 ) ;
#21305=DIRECTION ( 'NONE',  ( 1.000000000000000000, 0.000000000000000000, 0.000000000000000000 ) ) ;
#21306=CARTESIAN_POINT ( 'NONE',  ( -10.00000337463127842, -69.28203230275519786, -5.000000000000000000 ) ) ;
#21307=VERTEX_POINT ( 'NONE', #16287 ) ;
#21308=ORIENTED_EDGE ( 'NONE', *, *, #22194, .F. ) ;
#21309=EDGE_CURVE ( 'NONE', #5741, #6801, #36254, .T. ) ;
#21310=EDGE_LOOP ( 'NONE', ( #27616, #12791, #5763, #35792 ) ) ;
#21311=FACE_OUTER_BOUND ( 'NONE', #33024, .T. ) ;
#21312=CARTESIAN_POINT ( 'NONE',  ( -20.00000337463124112, 69.28203230275516944, -9.999999999999998224 ) ) ;
#21313=CIRCLE ( 'NONE', #3354, 2.000000000000001776 ) ;
#21314=DIRECTION ( 'NONE',  ( 0.000000000000000000, -0.000000000000000000, -1.000000000000000000 ) ) ;
#21316=AXIS2_PLACEMENT_3D ( 'NONE', #19172, #10336, #33030 ) ;
#21317=CARTESIAN_POINT ( 'NONE',  ( -43.19957991610399972, -47.04203867989563292, 12.49999999999999822 ) ) ;
#21318=DIRECTION ( 'NONE',  ( 0.000000000000000000, 0.000000000000000000, -1.000000000000000000 ) ) ;
#21319=CIRCLE ( 'NONE', #26115, 2.000000000000001776 ) ;
#21320=CYLINDRICAL_SURFACE ( 'NONE', #31007, 2.000000000000001776 ) ;
#21322=ORIENTED_EDGE ( 'NONE', *, *, #33709, .T. ) ;
#21323=AXIS2_PLACEMENT_3D ( 'NONE', #28558, #33650, #16389 ) ;
#21325=FACE_OUTER_BOUND ( 'NONE', #25455, .T. ) ;
#21326=VECTOR ( 'NONE', #20639, 1000.000000000000000 ) ;
#21327=ADVANCED_FACE ( 'NONE', ( #2580 ), #25452, .F. ) ;
#21328=PLANE ( 'NONE',  #34347 ) ;
#21330=EDGE_CURVE ( 'NONE', #29660, #24005, #19651, .T. ) ;
#21331=CARTESIAN_POINT ( 'NONE',  ( -68.00000337463099243, 51.96152422706637708, -9.999999999999998224 ) ) ;
#21333=DIRECTION ( 'NONE',  ( 0.000000000000000000, 0.000000000000000000, 1.000000000000000000 ) ) ;
#21334=AXIS2_PLACEMENT_3D ( 'NONE', #14514, #14687, #12217 ) ;
#21335=ADVANCED_FACE ( 'NONE', ( #36891 ), #5411, .F. ) ;
#21336=FACE_BOUND ( 'NONE', #14260, .T. ) ;
#21337=VERTEX_POINT ( 'NONE', #25109 ) ;
#21340=CARTESIAN_POINT ( 'NONE',  ( 34.99999662536855283, -60.62177826491080168, -9.999999999999998224 ) ) ;
#21341=VERTEX_POINT ( 'NONE', #30700 ) ;
#21345=DIRECTION ( 'NONE',  ( 1.000000000000000000, 0.000000000000000000, 0.000000000000000000 ) ) ;
#21347=ORIENTED_EDGE ( 'NONE', *, *, #2626, .T. ) ;
#21348=DIRECTION ( 'NONE',  ( 0.000000000000000000, 0.000000000000000000, 1.000000000000000000 ) ) ;
#21350=VECTOR ( 'NONE', #22362, 1000.000000000000000 ) ;
#21351=ADVANCED_FACE ( 'NONE', ( #30882 ), #28085, .F. ) ;
#21352=ORIENTED_EDGE ( 'NONE', *, *, #28098, .F. ) ;
#21355=EDGE_CURVE ( 'NONE', #28135, #35764, #1496, .T. ) ;
#21357=AXIS2_PLACEMENT_3D ( 'NONE', #30669, #27847, #2175 ) ;
#21359=EDGE_CURVE ( 'NONE', #2691, #14593, #20071, .T. ) ;
#21360=DIRECTION ( 'NONE',  ( 0.000000000000000000, 0.000000000000000000, -1.000000000000000000 ) ) ;
#21361=EDGE_CURVE ( 'NONE', #3947, #35128, #26658, .T. ) ;
#21362=CARTESIAN_POINT ( 'NONE',  ( -70.00000337463099243, -2.428612866367529932E-14, -9.999999999999998224 ) ) ;
#21363=VERTEX_POINT ( 'NONE', #14950 ) ;
#21365=CYLINDRICAL_SURFACE ( 'NONE', #24979, 2.000000000000001776 ) ;
#21366=ORIENTED_EDGE ( 'NONE', *, *, #5992, .T. ) ;
#21367=CARTESIAN_POINT ( 'NONE',  ( -42.00000337463114164, -69.28203230275519786, 12.50000000000000000 ) ) ;
#21368=AXIS2_PLACEMENT_3D ( 'NONE', #17297, #29068, #6204 ) ;
#21369=CARTESIAN_POINT ( 'NONE',  ( -70.00000337463100664, -17.32050807568882078, -9.999999999999998224 ) ) ;
#21371=CYLINDRICAL_SURFACE ( 'NONE', #8905, 2.000000000000001776 ) ;
#21372=CYLINDRICAL_SURFACE ( 'NONE', #7604, 27.00000000000001066 ) ;
#21373=FACE_OUTER_BOUND ( 'NONE', #34226, .T. ) ;
#21374=VERTEX_POINT ( 'NONE', #34823 ) ;
#21375=AXIS2_PLACEMENT_3D ( 'NONE', #25164, #36409, #22707 ) ;
#21376=ORIENTED_EDGE ( 'NONE', *, *, #25271, .F. ) ;
#21377=DIRECTION ( 'NONE',  ( 1.000000000000000000, 0.000000000000000000, 0.000000000000000000 ) ) ;
#21379=AXIS2_PLACEMENT_3D ( 'NONE', #18195, #957, #3408 ) ;
#21382=DIRECTION ( 'NONE',  ( 1.000000000000000000, 0.000000000000000000, 0.000000000000000000 ) ) ;
#21383=AXIS2_PLACEMENT_3D ( 'NONE', #23522, #32502, #1019 ) ;
#21385=AXIS2_PLACEMENT_3D ( 'NONE', #8896, #30384, #36396 ) ;
#21386=CARTESIAN_POINT ( 'NONE',  ( 84.99999662536832545, 25.98076211353319565, 17.49999999999999645 ) ) ;
#21387=AXIS2_PLACEMENT_3D ( 'NONE', #10135, #35630, #18380 ) ;
#21389=AXIS2_PLACEMENT_3D ( 'NONE', #13697, #25153, #10876 ) ;
#21390=CIRCLE ( 'NONE', #26178, 95.00000000000001421 ) ;
#21391=ORIENTED_EDGE ( 'NONE', *, *, #11484, .T. ) ;
#21392=FACE_OUTER_BOUND ( 'NONE', #27429, .T. ) ;
#21393=ORIENTED_EDGE ( 'NONE', *, *, #25440, .F. ) ;
#21394=AXIS2_PLACEMENT_3D ( 'NONE', #5378, #19614, #10621 ) ;
#21395=CARTESIAN_POINT ( 'NONE',  ( -58.88972745734155723, 34.00000000000049027, -4.999999999999997335 ) ) ;
#21396=CIRCLE ( 'NONE', #5238, 2.000000000000001776 ) ;
#21397=LINE ( 'NONE', #21197, #25409 ) ;
#21399=ORIENTED_EDGE ( 'NONE', *, *, #11060, .F. ) ;
#21402=CIRCLE ( 'NONE', #35206, 2.000000000000001776 ) ;
#21403=VERTEX_POINT ( 'NONE', #9116 ) ;
#21405=EDGE_CURVE ( 'NONE', #16746, #10350, #23755, .T. ) ;
#21406=FACE_BOUND ( 'NONE', #2477, .T. ) ;
#21407=CARTESIAN_POINT ( 'NONE',  ( -5.000003374631307729, 77.94228634059957983, -9.999999999999998224 ) ) ;
#21408=DIRECTION ( 'NONE',  ( 1.000000000000000000, 0.000000000000000000, 0.000000000000000000 ) ) ;
#21411=ORIENTED_EDGE ( 'NONE', *, *, #23567, .F. ) ;
#21412=DIRECTION ( 'NONE',  ( 0.000000000000000000, 0.000000000000000000, -1.000000000000000000 ) ) ;
#21413=AXIS2_PLACEMENT_3D ( 'NONE', #27916, #18932, #30359 ) ;
#21416=VERTEX_POINT ( 'NONE', #14749 ) ;
#21418=DIRECTION ( 'NONE',  ( 0.000000000000000000, 0.000000000000000000, 1.000000000000000000 ) ) ;
#21419=FACE_BOUND ( 'NONE', #6041, .T. ) ;
#21420=VECTOR ( 'NONE', #34793, 1000.000000000000000 ) ;
#21421=ORIENTED_EDGE ( 'NONE', *, *, #2064, .F. ) ;
#21422=ORIENTED_EDGE ( 'NONE', *, *, #18072, .F. ) ;
#21423=VECTOR ( 'NONE', #21426, 1000.000000000000000 ) ;
#21424=CARTESIAN_POINT ( 'NONE',  ( 32.99999662536853862, 77.94228634059959404, -9.999999999999998224 ) ) ;
#21426=DIRECTION ( 'NONE',  ( 0.000000000000000000, 0.000000000000000000, 1.000000000000000000 ) ) ;
#21427=ORIENTED_EDGE ( 'NONE', *, *, #30554, .T. ) ;
#21428=ORIENTED_EDGE ( 'NONE', *, *, #35966, .T. ) ;
#21429=CIRCLE ( 'NONE', #32197, 2.000000000000000000 ) ;
#21430=EDGE_LOOP ( 'NONE', ( #23620, #14029, #13382, #4140 ) ) ;
#21431=EDGE_CURVE ( 'NONE', #13150, #34663, #24854, .T. ) ;
#21432=EDGE_CURVE ( 'NONE', #28343, #4869, #29617, .T. ) ;
#21433=AXIS2_PLACEMENT_3D ( 'NONE', #12286, #11941, #3697 ) ;
#21434=CYLINDRICAL_SURFACE ( 'NONE', #2135, 2.000000000000000000 ) ;
#21435=AXIS2_PLACEMENT_3D ( 'NONE', #63, #16776, #5887 ) ;
#21436=VERTEX_POINT ( 'NONE', #35207 ) ;
#21438=DIRECTION ( 'NONE',  ( -0.000000000000000000, -0.000000000000000000, 1.000000000000000000 ) ) ;
#21439=ORIENTED_EDGE ( 'NONE', *, *, #35048, .F. ) ;
#21440=ORIENTED_EDGE ( 'NONE', *, *, #10435, .T. ) ;
#21441=AXIS2_PLACEMENT_3D ( 'NONE', #2312, #36991, #11300 ) ;
#21443=CARTESIAN_POINT ( 'NONE',  ( -72.00000337463102085, -34.64101615137762025, 17.49999999999999645 ) ) ;
#21445=VERTEX_POINT ( 'NONE', #23558 ) ;
#21446=ORIENTED_EDGE ( 'NONE', *, *, #1152, .F. ) ;
#21447=DIRECTION ( 'NONE',  ( 1.000000000000000000, 0.000000000000000000, 0.000000000000000000 ) ) ;
#21448=CIRCLE ( 'NONE', #10077, 2.000000000000001776 ) ;
#21449=CARTESIAN_POINT ( 'NONE',  ( -15.00000337463125710, -77.94228634059960825, 12.50000000000000000 ) ) ;
#21450=LINE ( 'NONE', #29498, #18678 ) ;
#21451=CYLINDRICAL_SURFACE ( 'NONE', #1095, 2.000000000000001776 ) ;
#21452=VERTEX_POINT ( 'NONE', #3312 ) ;
#21453=DIRECTION ( 'NONE',  ( -1.000000000000000000, 0.000000000000000000, 0.000000000000000000 ) ) ;
#21454=VECTOR ( 'NONE', #20456, 1000.000000000000000 ) ;
#21455=VERTEX_POINT ( 'NONE', #11742 ) ;
#21456=EDGE_CURVE ( 'NONE', #5647, #27967, #18248, .T. ) ;
#21457=DIRECTION ( 'NONE',  ( 0.000000000000000000, 0.000000000000000000, 1.000000000000000000 ) ) ;
#21458=CIRCLE ( 'NONE', #5306, 2.000000000000001776 ) ;
#21459=CYLINDRICAL_SURFACE ( 'NONE', #13019, 2.000000000000001776 ) ;
#21461=CARTESIAN_POINT ( 'NONE',  ( -65.00000337463104927, -43.30127018922202353, -9.999999999999998224 ) ) ;
#21462=FACE_OUTER_BOUND ( 'NONE', #9447, .T. ) ;
#21463=CIRCLE ( 'NONE', #19001, 2.000000000000001776 ) ;
#21464=CARTESIAN_POINT ( 'NONE',  ( 24.99999662536857059, 77.94228634059957983, -9.999999999999998224 ) ) ;
#21465=CIRCLE ( 'NONE', #12453, 2.000000000000001776 ) ;
#21467=ORIENTED_EDGE ( 'NONE', *, *, #17457, .F. ) ;
#21468=DIRECTION ( 'NONE',  ( 0.000000000000000000, 0.000000000000000000, 1.000000000000000000 ) ) ;
#21469=DIRECTION ( 'NONE',  ( 0.000000000000000000, 0.000000000000000000, 1.000000000000000000 ) ) ;
#21470=DIRECTION ( 'NONE',  ( 0.000000000000000000, 0.000000000000000000, 1.000000000000000000 ) ) ;
#21471=CIRCLE ( 'NONE', #586, 2.000000000000001776 ) ;
#21474=EDGE_LOOP ( 'NONE', ( #6437, #8684 ) ) ;
#21475=ORIENTED_EDGE ( 'NONE', *, *, #4874, .F. ) ;
#21476=EDGE_CURVE ( 'NONE', #7527, #11869, #34433, .T. ) ;
#21477=CARTESIAN_POINT ( 'NONE',  ( 66.98486176412667703, -43.54685190870066691, -5.000000000000000000 ) ) ;
#21478=CARTESIAN_POINT ( 'NONE',  ( 64.99999662536839651, -60.62177826491080168, -9.999999999999998224 ) ) ;
#21479=DIRECTION ( 'NONE',  ( 0.000000000000000000, 0.000000000000000000, 1.000000000000000000 ) ) ;
#21480=ORIENTED_EDGE ( 'NONE', *, *, #5860, .F. ) ;
#21481=AXIS2_PLACEMENT_3D ( 'NONE', #1066, #26750, #14565 ) ;
#21483=CARTESIAN_POINT ( 'NONE',  ( 58.48108235278871803, 36.97203788308964789, -49.86561046011506448 ) ) ;
#21485=DIRECTION ( 'NONE',  ( 0.000000000000000000, 0.000000000000000000, 1.000000000000000000 ) ) ;
#21486=ORIENTED_EDGE ( 'NONE', *, *, #23539, .T. ) ;
#21487=DIRECTION ( 'NONE',  ( 1.000000000000000000, 0.000000000000000000, 0.000000000000000000 ) ) ;
#21488=ADVANCED_FACE ( 'NONE', ( #29373 ), #26551, .F. ) ;
#21489=ORIENTED_EDGE ( 'NONE', *, *, #36702, .T. ) ;
#21490=AXIS2_PLACEMENT_3D ( 'NONE', #119, #14744, #25997 ) ;
#21491=DIRECTION ( 'NONE',  ( 1.000000000000000000, 0.000000000000000000, -0.000000000000000000 ) ) ;
#21492=EDGE_CURVE ( 'NONE', #12315, #20659, #3294, .T. ) ;
#21493=DIRECTION ( 'NONE',  ( -1.000000000000000000, 0.000000000000000000, 0.000000000000000000 ) ) ;
#21494=LINE ( 'NONE', #10795, #30526 ) ;
#21495=AXIS2_PLACEMENT_3D ( 'NONE', #2906, #31372, #34225 ) ;
#21496=ORIENTED_EDGE ( 'NONE', *, *, #22695, .T. ) ;
#21497=DIRECTION ( 'NONE',  ( -1.000000000000000000, 0.000000000000000000, 0.000000000000000000 ) ) ;
#21498=CIRCLE ( 'NONE', #32873, 27.00000000000001776 ) ;
#21499=CARTESIAN_POINT ( 'NONE',  ( -70.47608876694631874, -59.13646009116124702, -49.22241343995298024 ) ) ;
#21500=CARTESIAN_POINT ( 'NONE',  ( -67.00000337463106348, -60.62177826491083010, -9.999999999999998224 ) ) ;
#21501=CARTESIAN_POINT ( 'NONE',  ( 74.99999662536836809, 8.660254037844394404, 12.50000000000000000 ) ) ;
#21502=ORIENTED_EDGE ( 'NONE', *, *, #10501, .T. ) ;
#21503=DIRECTION ( 'NONE',  ( 0.000000000000000000, 0.000000000000000000, 1.000000000000000000 ) ) ;
#21504=DIRECTION ( 'NONE',  ( 0.000000000000000000, 0.000000000000000000, 1.000000000000000000 ) ) ;
#21505=DIRECTION ( 'NONE',  ( 1.000000000000000000, 0.000000000000000000, 0.000000000000000000 ) ) ;
#21506=EDGE_CURVE ( 'NONE', #15689, #16094, #6877, .T. ) ;
#21508=VECTOR ( 'NONE', #1664, 1000.000000000000000 ) ;
#21509=ORIENTED_EDGE ( 'NONE', *, *, #28916, .F. ) ;
#21510=CIRCLE ( 'NONE', #20926, 2.000000000000001776 ) ;
#21511=DIRECTION ( 'NONE',  ( 1.000000000000000000, 0.000000000000000000, 0.000000000000000000 ) ) ;
#21512=DIRECTION ( 'NONE',  ( 0.000000000000000000, 0.000000000000000000, 1.000000000000000000 ) ) ;
#21514=CARTESIAN_POINT ( 'NONE',  ( -10.00000337463128197, 86.60254037844397601, -9.999999999999998224 ) ) ;
#21515=EDGE_LOOP ( 'NONE', ( #6593, #24693 ) ) ;
#21516=VECTOR ( 'NONE', #13223, 1000.000000000000000 ) ;
#21517=ADVANCED_FACE ( 'NONE', ( #20198 ), #8947, .F. ) ;
#21518=DIRECTION ( 'NONE',  ( -1.000000000000000000, 0.000000000000000000, 0.000000000000000000 ) ) ;
#21524=ORIENTED_EDGE ( 'NONE', *, *, #4522, .T. ) ;
#21525=CARTESIAN_POINT ( 'NONE',  ( -83.00000337463092137, 25.98076211353317433, -5.000000000000000000 ) ) ;
#21526=AXIS2_PLACEMENT_3D ( 'NONE', #33667, #21669, #33097 ) ;
#21527=DIRECTION ( 'NONE',  ( -1.000000000000000000, 0.000000000000000000, 0.000000000000000000 ) ) ;
#21529=CIRCLE ( 'NONE', #16748, 2.000000000000001776 ) ;
#21531=ORIENTED_EDGE ( 'NONE', *, *, #23866, .T. ) ;
#21532=LINE ( 'NONE', #27877, #35693 ) ;
#21533=EDGE_CURVE ( 'NONE', #18729, #32725, #33245, .T. ) ;
#21534=CARTESIAN_POINT ( 'NONE',  ( 76.99999662536836809, -8.660254037844401509, -9.999999999999998224 ) ) ;
#21535=AXIS2_PLACEMENT_3D ( 'NONE', #12491, #1615, #865 ) ;
#21536=ORIENTED_EDGE ( 'NONE', *, *, #35053, .T. ) ;
#21538=AXIS2_PLACEMENT_3D ( 'NONE', #4675, #7467, #7288 ) ;
#21539=CARTESIAN_POINT ( 'NONE',  ( 69.99999662536841072, 51.96152422706640550, -9.999999999999998224 ) ) ;
#21540=EDGE_LOOP ( 'NONE', ( #26586, #34171 ) ) ;
#21541=PLANE ( 'NONE',  #27211 ) ;
#21542=DIRECTION ( 'NONE',  ( 0.000000000000000000, 0.000000000000000000, 1.000000000000000000 ) ) ;
#21543=CARTESIAN_POINT ( 'NONE',  ( -58.88972745734203329, -33.99999999999965894, 12.49999999999999822 ) ) ;
#21544=VERTEX_POINT ( 'NONE', #14560 ) ;
#21545=DIRECTION ( 'NONE',  ( 1.000000000000000000, 0.000000000000000000, 0.000000000000000000 ) ) ;
#21546=CARTESIAN_POINT ( 'NONE',  ( 59.99999662536843914, -34.64101615137759893, -5.000000000000000000 ) ) ;
#21547=AXIS2_PLACEMENT_3D ( 'NONE', #35932, #13036, #1409 ) ;
#21548=ORIENTED_EDGE ( 'NONE', *, *, #31934, .F. ) ;
#21549=EDGE_LOOP ( 'NONE', ( #34879, #14405, #11457, #36208 ) ) ;
#21550=CIRCLE ( 'NONE', #5397, 2.000000000000001776 ) ;
#21551=EDGE_CURVE ( 'NONE', #2028, #13905, #20650, .T. ) ;
#21552=VERTEX_POINT ( 'NONE', #30296 ) ;
#21554=AXIS2_PLACEMENT_3D ( 'NONE', #22375, #19382, #10771 ) ;
#21556=EDGE_CURVE ( 'NONE', #32159, #33756, #30824, .T. ) ;
#21557=ORIENTED_EDGE ( 'NONE', *, *, #31094, .F. ) ;
#21558=DIRECTION ( 'NONE',  ( 1.000000000000000000, 0.000000000000000000, 0.000000000000000000 ) ) ;
#21561=ORIENTED_EDGE ( 'NONE', *, *, #22493, .T. ) ;
#21563=EDGE_CURVE ( 'NONE', #18966, #8725, #29020, .T. ) ;
#21564=DIRECTION ( 'NONE',  ( 0.000000000000000000, 0.000000000000000000, -1.000000000000000000 ) ) ;
#21566=CARTESIAN_POINT ( 'NONE',  ( 82.99999662536832545, 25.98076211353319565, -9.999999999999998224 ) ) ;
#21567=CARTESIAN_POINT ( 'NONE',  ( 79.99999662536833966, 34.64101615137759183, -5.000000000000000000 ) ) ;
#21568=EDGE_CURVE ( 'NONE', #25550, #16224, #17658, .T. ) ;
#21569=AXIS2_PLACEMENT_3D ( 'NONE', #13965, #2373, #36504 ) ;
#21570=CARTESIAN_POINT ( 'NONE',  ( 61.99999662536842493, 51.96152422706639129, 17.49999999999999645 ) ) ;
#21572=DIRECTION ( 'NONE',  ( 0.000000000000000000, 0.000000000000000000, 1.000000000000000000 ) ) ;
#21573=ORIENTED_EDGE ( 'NONE', *, *, #26979, .F. ) ;
#21575=CARTESIAN_POINT ( 'NONE',  ( 39.99999662536853151, -69.28203230275519786, -9.999999999999998224 ) ) ;
#21576=DIRECTION ( 'NONE',  ( -1.000000000000000000, 0.000000000000000000, 0.000000000000000000 ) ) ;
#21577=CARTESIAN_POINT ( 'NONE',  ( -62.33939050065184517, 13.89091430021398565, 12.49999999999999822 ) ) ;
#21578=CIRCLE ( 'NONE', #30570, 2.000000000000001776 ) ;
#21580=EDGE_LOOP ( 'NONE', ( #17950, #4949, #7371, #13094, #8401, #9066, #22585, #20411, #19354, #4501 ) ) ;
#21582=DIRECTION ( 'NONE',  ( 1.000000000000000000, 0.000000000000000000, 0.000000000000000000 ) ) ;
#21584=CARTESIAN_POINT ( 'NONE',  ( -43.00000337463111322, 60.62177826491077326, -9.999999999999998224 ) ) ;
#21585=EDGE_CURVE ( 'NONE', #5993, #281, #27290, .T. ) ;
#21586=CARTESIAN_POINT ( 'NONE',  ( 0.000000000000000000, -55.00000000000000000, -10.00000000000000000 ) ) ;
#21587=ORIENTED_EDGE ( 'NONE', *, *, #28206, .T. ) ;
#21588=EDGE_CURVE ( 'NONE', #31151, #27157, #12288, .T. ) ;
#21589=VECTOR ( 'NONE', #35065, 1000.000000000000000 ) ;
#21590=EDGE_CURVE ( 'NONE', #10255, #17870, #29731, .T. ) ;
#21591=CARTESIAN_POINT ( 'NONE',  ( -85.00000337463092137, 8.660254037844389075, -5.000000000000000000 ) ) ;
#21592=AXIS2_PLACEMENT_3D ( 'NONE', #36956, #14440, #8812 ) ;
#21596=CARTESIAN_POINT ( 'NONE',  ( -31.02796211690907668, 59.29837256189569672, 12.49999999999999645 ) ) ;
#21597=VERTEX_POINT ( 'NONE', #3860 ) ;
#21598=VERTEX_POINT ( 'NONE', #1423 ) ;
#21600=DIRECTION ( 'NONE',  ( 0.000000000000000000, 0.000000000000000000, 1.000000000000000000 ) ) ;
#21601=FACE_BOUND ( 'NONE', #35654, .T. ) ;
#21602=DIRECTION ( 'NONE',  ( 0.000000000000000000, 0.000000000000000000, 1.000000000000000000 ) ) ;
#21604=LINE ( 'NONE', #35661, #12326 ) ;
#21605=ORIENTED_EDGE ( 'NONE', *, *, #34648, .T. ) ;
#21607=DIRECTION ( 'NONE',  ( 0.000000000000000000, 0.000000000000000000, 1.000000000000000000 ) ) ;
#21610=ORIENTED_EDGE ( 'NONE', *, *, #12224, .F. ) ;
#21611=DIRECTION ( 'NONE',  ( 0.000000000000000000, 0.000000000000000000, -1.000000000000000000 ) ) ;
#21613=ORIENTED_EDGE ( 'NONE', *, *, #31791, .F. ) ;
#21614=EDGE_LOOP ( 'NONE', ( #16400, #34324, #3458, #7043 ) ) ;
#21615=CYLINDRICAL_SURFACE ( 'NONE', #19313, 2.000000000000001776 ) ;
#21616=DIRECTION ( 'NONE',  ( 0.000000000000000000, 0.000000000000000000, 1.000000000000000000 ) ) ;
#21618=EDGE_LOOP ( 'NONE', ( #7865, #15037, #19078, #30523 ) ) ;
#21619=VERTEX_POINT ( 'NONE', #26935 ) ;
#21620=ORIENTED_EDGE ( 'NONE', *, *, #14498, .T. ) ;
#21621=EDGE_CURVE ( 'NONE', #26836, #4724, #28472, .T. ) ;
#21622=DIRECTION ( 'NONE',  ( -0.000000000000000000, -0.000000000000000000, 1.000000000000000000 ) ) ;
#21623=EDGE_CURVE ( 'NONE', #32378, #18828, #25488, .T. ) ;
#21624=ORIENTED_EDGE ( 'NONE', *, *, #20634, .F. ) ;
#21625=ADVANCED_FACE ( 'NONE', ( #32375 ), #12667, .F. ) ;
#21626=EDGE_LOOP ( 'NONE', ( #31017, #23759 ) ) ;
#21627=LINE ( 'NONE', #32879, #23195 ) ;
#21628=ORIENTED_EDGE ( 'NONE', *, *, #10435, .F. ) ;
#21629=VERTEX_POINT ( 'NONE', #32543 ) ;
#21630=DIRECTION ( 'NONE',  ( -0.000000000000000000, 0.000000000000000000, -1.000000000000000000 ) ) ;
#21631=FACE_OUTER_BOUND ( 'NONE', #11092, .T. ) ;
#21632=ORIENTED_EDGE ( 'NONE', *, *, #12735, .T. ) ;
#21633=ORIENTED_EDGE ( 'NONE', *, *, #30612, .T. ) ;
#21634=CYLINDRICAL_SURFACE ( 'NONE', #19692, 2.000000000000001776 ) ;
#21635=CARTESIAN_POINT ( 'NONE',  ( -18.00000337463123046, 86.60254037844397601, -5.000000000000000000 ) ) ;
#21636=CARTESIAN_POINT ( 'NONE',  ( 1.999996625368665182, 69.28203230275516944, 17.49999999999999645 ) ) ;
#21637=CARTESIAN_POINT ( 'NONE',  ( 59.29837256189581041, 31.02796211690886707, -49.86561046011506448 ) ) ;
#21638=EDGE_LOOP ( 'NONE', ( #15631, #1550, #16793, #21605, #16187, #5780 ) ) ;
#21639=DIRECTION ( 'NONE',  ( 0.000000000000000000, 0.000000000000000000, -1.000000000000000000 ) ) ;
#21640=ORIENTED_EDGE ( 'NONE', *, *, #11005, .T. ) ;
#21642=DIRECTION ( 'NONE',  ( 1.000000000000000000, 0.000000000000000000, 0.000000000000000000 ) ) ;
#21643=DIRECTION ( 'NONE',  ( 0.000000000000000000, 0.000000000000000000, -1.000000000000000000 ) ) ;
#21644=CARTESIAN_POINT ( 'NONE',  ( 59.13646009116148150, -70.47608876694609137, -49.22241343995298024 ) ) ;
#21646=CARTESIAN_POINT ( 'NONE',  ( -67.00000337463104927, -43.30127018922202353, -9.999999999999998224 ) ) ;
#21648=DIRECTION ( 'NONE',  ( 0.000000000000000000, 0.000000000000000000, 1.000000000000000000 ) ) ;
#21649=ORIENTED_EDGE ( 'NONE', *, *, #7559, .T. ) ;
#21650=DIRECTION ( 'NONE',  ( 1.000000000000000000, 0.000000000000000000, 0.000000000000000000 ) ) ;
#21651=CIRCLE ( 'NONE', #5485, 3.499999999999987566 ) ;
#21652=CARTESIAN_POINT ( 'NONE',  ( 0.000000000000000000, -55.00000000000000000, -10.00000000000000000 ) ) ;
#21653=DIRECTION ( 'NONE',  ( -1.000000000000000000, 0.000000000000000000, 0.000000000000000000 ) ) ;
#21655=EDGE_CURVE ( 'NONE', #25696, #25394, #12894, .T. ) ;
#21656=ORIENTED_EDGE ( 'NONE', *, *, #25903, .T. ) ;
#21657=VERTEX_POINT ( 'NONE', #35753 ) ;
#21658=FACE_OUTER_BOUND ( 'NONE', #33927, .T. ) ;
#21659=DIRECTION ( 'NONE',  ( 0.000000000000000000, 0.000000000000000000, 1.000000000000000000 ) ) ;
#21660=VERTEX_POINT ( 'NONE', #10064 ) ;
#21661=DIRECTION ( 'NONE',  ( 1.000000000000000000, 0.000000000000000000, 0.000000000000000000 ) ) ;
#21662=DIRECTION ( 'NONE',  ( 1.000000000000000000, 0.000000000000000000, 0.000000000000000000 ) ) ;
#21663=ORIENTED_EDGE ( 'NONE', *, *, #35108, .T. ) ;
#21664=ADVANCED_FACE ( 'NONE', ( #24505 ), #7425, .T. ) ;
#21667=FACE_BOUND ( 'NONE', #33537, .T. ) ;
#21669=DIRECTION ( 'NONE',  ( 0.000000000000000000, 0.000000000000000000, 1.000000000000000000 ) ) ;
#21670=CARTESIAN_POINT ( 'NONE',  ( -31.02796211690907668, 59.29837256189569672, -49.86561046011506448 ) ) ;
#21674=CARTESIAN_POINT ( 'NONE',  ( -47.63139720814438505, -27.49999999999955591, -10.00000000000000178 ) ) ;
#21675=DIRECTION ( 'NONE',  ( 1.000000000000000000, 0.000000000000000000, 0.000000000000000000 ) ) ;
#21676=CYLINDRICAL_SURFACE ( 'NONE', #24580, 3.000000000000002665 ) ;
#21677=DIRECTION ( 'NONE',  ( 0.000000000000000000, 0.000000000000000000, 1.000000000000000000 ) ) ;
#21679=ORIENTED_EDGE ( 'NONE', *, *, #4095, .F. ) ;
#21680=CARTESIAN_POINT ( 'NONE',  ( -13.00000337463126066, 77.94228634059957983, -9.999999999999998224 ) ) ;
#21681=FACE_OUTER_BOUND ( 'NONE', #12607, .T. ) ;
#21682=CARTESIAN_POINT ( 'NONE',  ( 21.99999662536857770, 86.60254037844397601, 17.49999999999999645 ) ) ;
#21683=ADVANCED_FACE ( 'NONE', ( #22601 ), #34054, .F. ) ;
#21684=ORIENTED_EDGE ( 'NONE', *, *, #3027, .T. ) ;
#21685=ORIENTED_EDGE ( 'NONE', *, *, #18987, .T. ) ;
#21686=EDGE_CURVE ( 'NONE', #29469, #10997, #30852, .T. ) ;
#21687=CARTESIAN_POINT ( 'NONE',  ( -36.97203788308986105, 58.48108235278859013, -49.86561046011506448 ) ) ;
#21688=CARTESIAN_POINT ( 'NONE',  ( 17.99999662536861678, -86.60254037844400443, -9.999999999999998224 ) ) ;
#21689=CARTESIAN_POINT ( 'NONE',  ( 84.99999662536832545, 25.98076211353319565, 12.50000000000000000 ) ) ;
#21690=EDGE_CURVE ( 'NONE', #15799, #23723, #26067, .T. ) ;
#21691=ORIENTED_EDGE ( 'NONE', *, *, #5790, .T. ) ;
#21692=AXIS2_PLACEMENT_3D ( 'NONE', #22158, #32851, #10335 ) ;
#21693=DIRECTION ( 'NONE',  ( -0.5000000000000094369, -0.8660254037844332675, 0.000000000000000000 ) ) ;
#21695=DIRECTION ( 'NONE',  ( -1.000000000000000000, 0.000000000000000000, 0.000000000000000000 ) ) ;
#21696=DIRECTION ( 'NONE',  ( 1.000000000000000000, 0.000000000000000000, 0.000000000000000000 ) ) ;
#21697=EDGE_LOOP ( 'NONE', ( #32169, #33647, #21366, #35494 ) ) ;
#21698=VERTEX_POINT ( 'NONE', #5370 ) ;
#21701=EDGE_LOOP ( 'NONE', ( #35624, #26346 ) ) ;
#21703=PLANE ( 'NONE',  #28103 ) ;
#21704=ORIENTED_EDGE ( 'NONE', *, *, #5784, .F. ) ;
#21707=DIRECTION ( 'NONE',  ( 0.000000000000000000, 0.000000000000000000, 1.000000000000000000 ) ) ;
#21708=ORIENTED_EDGE ( 'NONE', *, *, #5444, .T. ) ;
#21709=DIRECTION ( 'NONE',  ( 0.000000000000000000, 0.000000000000000000, -1.000000000000000000 ) ) ;
#21711=EDGE_CURVE ( 'NONE', #33530, #29480, #29644, .T. ) ;
#21712=LINE ( 'NONE', #21155, #7474 ) ;
#21713=AXIS2_PLACEMENT_3D ( 'NONE', #1724, #10718, #13712 ) ;
#21714=FACE_OUTER_BOUND ( 'NONE', #30202, .T. ) ;
#21715=CARTESIAN_POINT ( 'NONE',  ( 71.99999662536839651, -17.32050807568879947, -9.999999999999998224 ) ) ;
#21717=EDGE_LOOP ( 'NONE', ( #24877, #10976, #2750, #19637, #19869, #29122, #36649, #28446, #11360, #11338, #23739, #10174, #19502, #7588, #32766, #35504, #36333, #33352, #22603, #9363, #9987, #5807, #22640, #31478 ) ) ;
#21718=VECTOR ( 'NONE', #21268, 1000.000000000000000 ) ;
#21719=LINE ( 'NONE', #36355, #35838 ) ;
#21721=DIRECTION ( 'NONE',  ( -1.000000000000000000, 0.000000000000000000, 0.000000000000000000 ) ) ;
#21723=VERTEX_POINT ( 'NONE', #19799 ) ;
#21725=DIRECTION ( 'NONE',  ( -0.000000000000000000, -0.000000000000000000, 1.000000000000000000 ) ) ;
#21726=VERTEX_POINT ( 'NONE', #19414 ) ;
#21727=ADVANCED_FACE ( 'NONE', ( #4979 ), #1976, .F. ) ;
#21728=CARTESIAN_POINT ( 'NONE',  ( 2.999996625368676728, -77.94228634059960825, 12.50000000000000000 ) ) ;
#21729=DIRECTION ( 'NONE',  ( 0.8660254037844415942, 0.4999999999999949485, 0.000000000000000000 ) ) ;
#21730=DIRECTION ( 'NONE',  ( 0.000000000000000000, 0.000000000000000000, 1.000000000000000000 ) ) ;
#21731=AXIS2_PLACEMENT_3D ( 'NONE', #33003, #4321, #4703 ) ;
#21732=CARTESIAN_POINT ( 'NONE',  ( 17.99999662536861678, -86.60254037844400443, 12.50000000000000000 ) ) ;
#21733=ADVANCED_FACE ( 'NONE', ( #31040 ), #4816, .F. ) ;
#21735=CARTESIAN_POINT ( 'NONE',  ( 77.99999662536832545, -17.32050807568879591, -5.000000000000000000 ) ) ;
#21736=LINE ( 'NONE', #1133, #26176 ) ;
#21737=LINE ( 'NONE', #30362, #16656 ) ;
#21738=ORIENTED_EDGE ( 'NONE', *, *, #30281, .F. ) ;
#21740=DIRECTION ( 'NONE',  ( 1.000000000000000000, 0.000000000000000000, 0.000000000000000000 ) ) ;
#21741=CIRCLE ( 'NONE', #34917, 2.000000000000001776 ) ;
#21742=DIRECTION ( 'NONE',  ( 1.000000000000000000, 0.000000000000000000, 0.000000000000000000 ) ) ;
#21743=LINE ( 'NONE', #24586, #33022 ) ;
#21744=CARTESIAN_POINT ( 'NONE',  ( -87.00000337463093558, -25.98076211353322051, -9.999999999999998224 ) ) ;
#21745=VERTEX_POINT ( 'NONE', #36667 ) ;
#21746=DIRECTION ( 'NONE',  ( -1.000000000000000000, 0.000000000000000000, 0.000000000000000000 ) ) ;
#21747=LINE ( 'NONE', #36388, #12304 ) ;
#21749=DIRECTION ( 'NONE',  ( 0.000000000000000000, 0.000000000000000000, 1.000000000000000000 ) ) ;
#21751=CARTESIAN_POINT ( 'NONE',  ( 79.99999662536832545, -34.64101615137759183, -9.999999999999998224 ) ) ;
#21754=CARTESIAN_POINT ( 'NONE',  ( 86.99999662536831124, -8.660254037844397956, -5.000000000000000000 ) ) ;
#21755=EDGE_CURVE ( 'NONE', #9228, #23602, #14691, .T. ) ;
#21758=EDGE_CURVE ( 'NONE', #9216, #11639, #11685, .T. ) ;
#21760=VERTEX_POINT ( 'NONE', #14154 ) ;
#21763=CARTESIAN_POINT ( 'NONE',  ( -68.00000337463102085, -34.64101615137762025, 17.49999999999999645 ) ) ;
#21764=EDGE_LOOP ( 'NONE', ( #21237, #12034 ) ) ;
#21765=CARTESIAN_POINT ( 'NONE',  ( 47.99999662536846756, -69.28203230275519786, 12.50000000000000000 ) ) ;
#21766=AXIS2_PLACEMENT_3D ( 'NONE', #30253, #30802, #19578 ) ;
#21768=DIRECTION ( 'NONE',  ( 0.000000000000000000, 0.000000000000000000, -1.000000000000000000 ) ) ;
#21769=DIRECTION ( 'NONE',  ( 0.000000000000000000, 0.000000000000000000, 1.000000000000000000 ) ) ;
#21771=ORIENTED_EDGE ( 'NONE', *, *, #12668, .T. ) ;
#21772=CIRCLE ( 'NONE', #5606, 2.000000000000001776 ) ;
#21773=CARTESIAN_POINT ( 'NONE',  ( -16.49657687835743403, 93.55673653615991725, 12.49999999999999822 ) ) ;
#21775=EDGE_CURVE ( 'NONE', #14243, #7403, #31219, .T. ) ;
#21776=ORIENTED_EDGE ( 'NONE', *, *, #34579, .T. ) ;
#21777=DIRECTION ( 'NONE',  ( 0.000000000000000000, 0.000000000000000000, 1.000000000000000000 ) ) ;
#21778=FACE_BOUND ( 'NONE', #26220, .T. ) ;
#21779=EDGE_LOOP ( 'NONE', ( #25435, #22790, #26538, #28489, #761 ) ) ;
#21781=VERTEX_POINT ( 'NONE', #16805 ) ;
#21782=DIRECTION ( 'NONE',  ( 0.000000000000000000, 0.000000000000000000, 1.000000000000000000 ) ) ;
#21784=CARTESIAN_POINT ( 'NONE',  ( -78.00000337463094979, -17.32050807568882078, -9.999999999999998224 ) ) ;
#21785=ORIENTED_EDGE ( 'NONE', *, *, #10289, .F. ) ;
#21787=EDGE_LOOP ( 'NONE', ( #31195, #10330 ) ) ;
#21788=AXIS2_PLACEMENT_3D ( 'NONE', #21109, #15114, #12662 ) ;
#21789=DIRECTION ( 'NONE',  ( -1.000000000000000000, 0.000000000000000000, 0.000000000000000000 ) ) ;
#21791=CIRCLE ( 'NONE', #17581, 3.000000000000002665 ) ;
#21792=ORIENTED_EDGE ( 'NONE', *, *, #35996, .F. ) ;
#21793=EDGE_CURVE ( 'NONE', #27693, #5293, #32647, .T. ) ;
#21794=CARTESIAN_POINT ( 'NONE',  ( -80.69570745083950669, 15.44540918807064500, 12.50000000000000000 ) ) ;
#21795=ORIENTED_EDGE ( 'NONE', *, *, #20069, .F. ) ;
#21797=EDGE_CURVE ( 'NONE', #35238, #8932, #13962, .T. ) ;
#21798=DIRECTION ( 'NONE',  ( 0.000000000000000000, 0.000000000000000000, 1.000000000000000000 ) ) ;
#21800=EDGE_LOOP ( 'NONE', ( #11308, #19951 ) ) ;
#21801=ORIENTED_EDGE ( 'NONE', *, *, #17143, .T. ) ;
#21803=DIRECTION ( 'NONE',  ( 0.000000000000000000, 0.000000000000000000, 1.000000000000000000 ) ) ;
#21804=DIRECTION ( 'NONE',  ( -0.4999999999999979461, 0.8660254037844397068, 0.000000000000000000 ) ) ;
#21806=DIRECTION ( 'NONE',  ( -0.000000000000000000, -0.000000000000000000, 1.000000000000000000 ) ) ;
#21807=AXIS2_PLACEMENT_3D ( 'NONE', #18667, #21094, #36609 ) ;
#21808=VERTEX_POINT ( 'NONE', #29325 ) ;
#21809=FACE_OUTER_BOUND ( 'NONE', #17357, .T. ) ;
#21810=ORIENTED_EDGE ( 'NONE', *, *, #28649, .F. ) ;
#21811=CARTESIAN_POINT ( 'NONE',  ( 52.99999662536844625, 43.30127018922198801, -5.000000000000000000 ) ) ;
#21813=PLANE ( 'NONE',  #36975 ) ;
#21815=ADVANCED_FACE ( 'NONE', ( #17515 ), #15079, .F. ) ;
#21816=CYLINDRICAL_SURFACE ( 'NONE', #17064, 2.000000000000001776 ) ;
#21817=AXIS2_PLACEMENT_3D ( 'NONE', #18961, #4519, #10158 ) ;
#21819=FACE_OUTER_BOUND ( 'NONE', #19822, .T. ) ;
#21820=ADVANCED_FACE ( 'NONE', ( #9076 ), #31761, .T. ) ;
#21821=AXIS2_PLACEMENT_3D ( 'NONE', #2038, #7873, #30720 ) ;
#21824=ORIENTED_EDGE ( 'NONE', *, *, #19574, .F. ) ;
#21825=DIRECTION ( 'NONE',  ( 1.000000000000000000, 0.000000000000000000, 0.000000000000000000 ) ) ;
#21827=CARTESIAN_POINT ( 'NONE',  ( 64.99999662536839651, -60.62177826491080168, -9.999999999999998224 ) ) ;
#21828=VERTEX_POINT ( 'NONE', #12056 ) ;
#21829=ORIENTED_EDGE ( 'NONE', *, *, #10349, .T. ) ;
#21830=VERTEX_POINT ( 'NONE', #17898 ) ;
#21832=CARTESIAN_POINT ( 'NONE',  ( 72.99999662536836809, 8.660254037844394404, -9.999999999999998224 ) ) ;
#21833=CYLINDRICAL_SURFACE ( 'NONE', #10963, 2.000000000000001776 ) ;
#21834=CIRCLE ( 'NONE', #27820, 2.000000000000001776 ) ;
#21835=EDGE_LOOP ( 'NONE', ( #16347, #5422, #33495, #19488, #33021 ) ) ;
#21836=AXIS2_PLACEMENT_3D ( 'NONE', #14281, #25890, #17283 ) ;
#21837=DIRECTION ( 'NONE',  ( -1.000000000000000000, 0.000000000000000000, 0.000000000000000000 ) ) ;
#21838=DIRECTION ( 'NONE',  ( 0.000000000000000000, 0.000000000000000000, 1.000000000000000000 ) ) ;
#21839=ORIENTED_EDGE ( 'NONE', *, *, #9666, .T. ) ;
#21841=ORIENTED_EDGE ( 'NONE', *, *, #23999, .F. ) ;
#21842=FACE_BOUND ( 'NONE', #3009, .T. ) ;
#21845=AXIS2_PLACEMENT_3D ( 'NONE', #26036, #17046, #17589 ) ;
#21848=DIRECTION ( 'NONE',  ( 0.000000000000000000, 0.000000000000000000, 1.000000000000000000 ) ) ;
#21849=AXIS2_PLACEMENT_3D ( 'NONE', #34604, #8904, #17516 ) ;
#21850=CARTESIAN_POINT ( 'NONE',  ( -65.00000337463102085, 43.30127018922198801, -9.999999999999998224 ) ) ;
#21851=ORIENTED_EDGE ( 'NONE', *, *, #7592, .T. ) ;
#21852=CARTESIAN_POINT ( 'NONE',  ( 30.89873427475420442, -67.49533964939347186, 12.50000000000000000 ) ) ;
#21856=CIRCLE ( 'NONE', #6275, 2.000000000000001776 ) ;
#21858=DIRECTION ( 'NONE',  ( 0.000000000000000000, 0.000000000000000000, 1.000000000000000000 ) ) ;
#21859=CARTESIAN_POINT ( 'NONE',  ( 64.99999662536839651, 60.62177826491078747, 12.50000000000000000 ) ) ;
#21862=VECTOR ( 'NONE', #9267, 1000.000000000000000 ) ;
#21864=DIRECTION ( 'NONE',  ( 0.000000000000000000, -0.000000000000000000, -1.000000000000000000 ) ) ;
#21869=PLANE ( 'NONE',  #3984 ) ;
#21870=DIRECTION ( 'NONE',  ( -1.000000000000000000, 0.000000000000000000, 0.000000000000000000 ) ) ;
#21871=CIRCLE ( 'NONE', #6878, 2.000000000000001776 ) ;
#21872=DIRECTION ( 'NONE',  ( -0.8660254037844449249, -0.4999999999999888978, 0.000000000000000000 ) ) ;
#21874=VERTEX_POINT ( 'NONE', #31386 ) ;
#21875=DIRECTION ( 'NONE',  ( 0.000000000000000000, 0.000000000000000000, 1.000000000000000000 ) ) ;
#21878=DIRECTION ( 'NONE',  ( 0.000000000000000000, 0.000000000000000000, 1.000000000000000000 ) ) ;
#21879=ORIENTED_EDGE ( 'NONE', *, *, #12635, .T. ) ;
#21881=CARTESIAN_POINT ( 'NONE',  ( 69.99999662536839651, 17.32050807568879236, -9.999999999999998224 ) ) ;
#21882=AXIS2_PLACEMENT_3D ( 'NONE', #13236, #4060, #9856 ) ;
#21883=DIRECTION ( 'NONE',  ( 0.000000000000000000, 0.000000000000000000, -1.000000000000000000 ) ) ;
#21884=EDGE_LOOP ( 'NONE', ( #18612, #9561 ) ) ;
#21885=CIRCLE ( 'NONE', #4524, 3.000000000000002665 ) ;
#21886=CYLINDRICAL_SURFACE ( 'NONE', #2979, 2.000000000000001776 ) ;
#21887=ORIENTED_EDGE ( 'NONE', *, *, #22710, .F. ) ;
#21889=EDGE_CURVE ( 'NONE', #13878, #32590, #26339, .T. ) ;
#21890=AXIS2_PLACEMENT_3D ( 'NONE', #17629, #26276, #3402 ) ;
#21891=AXIS2_PLACEMENT_3D ( 'NONE', #33536, #27871, #2007 ) ;
#21892=ADVANCED_FACE ( 'NONE', ( #647 ), #20339, .F. ) ;
#21894=CIRCLE ( 'NONE', #2550, 2.000000000000001776 ) ;
#21896=ORIENTED_EDGE ( 'NONE', *, *, #29456, .F. ) ;
#21897=EDGE_CURVE ( 'NONE', #17282, #12923, #22802, .T. ) ;
#21899=VERTEX_POINT ( 'NONE', #28775 ) ;
#21901=CIRCLE ( 'NONE', #16495, 2.000000000000001776 ) ;
#21902=CARTESIAN_POINT ( 'NONE',  ( 79.99999662536832545, -34.64101615137759183, 12.50000000000000000 ) ) ;
#21903=EDGE_CURVE ( 'NONE', #2842, #32102, #31246, .T. ) ;
#21904=CARTESIAN_POINT ( 'NONE',  ( 47.63139720814400846, -27.50000000000022737, -5.000000000000000000 ) ) ;
#21906=VERTEX_POINT ( 'NONE', #6262 ) ;
#21907=DIRECTION ( 'NONE',  ( 0.000000000000000000, 0.000000000000000000, 1.000000000000000000 ) ) ;
#21909=DIRECTION ( 'NONE',  ( 0.000000000000000000, 0.000000000000000000, 1.000000000000000000 ) ) ;
#21910=ORIENTED_EDGE ( 'NONE', *, *, #33894, .T. ) ;
#21912=ORIENTED_EDGE ( 'NONE', *, *, #14885, .F. ) ;
#21913=CIRCLE ( 'NONE', #1533, 2.000000000000000000 ) ;
#21914=EDGE_CURVE ( 'NONE', #12792, #13768, #25962, .T. ) ;
#21916=EDGE_LOOP ( 'NONE', ( #24184, #25221, #29864, #22863, #587 ) ) ;
#21917=CARTESIAN_POINT ( 'NONE',  ( -45.00000337463111322, -77.94228634059960825, 12.50000000000000000 ) ) ;
#21918=CARTESIAN_POINT ( 'NONE',  ( -55.00000337463110611, -43.30127018922202353, 17.49999999999999645 ) ) ;
#21919=CIRCLE ( 'NONE', #17708, 2.000000000000001776 ) ;
#21920=AXIS2_PLACEMENT_3D ( 'NONE', #12831, #1407, #20722 ) ;
#21921=CIRCLE ( 'NONE', #3365, 2.000000000000000000 ) ;
#21924=FACE_OUTER_BOUND ( 'NONE', #5862, .T. ) ;
#21925=CARTESIAN_POINT ( 'NONE',  ( 35.19434990244975126, -52.39915983220758022, -4.999999999999997335 ) ) ;
#21928=CIRCLE ( 'NONE', #7554, 3.000000000000002665 ) ;
#21929=DIRECTION ( 'NONE',  ( 0.000000000000000000, 0.000000000000000000, 1.000000000000000000 ) ) ;
#21930=EDGE_LOOP ( 'NONE', ( #26496, #35517, #3352, #16644 ) ) ;
#21932=ORIENTED_EDGE ( 'NONE', *, *, #20401, .F. ) ;
#21933=CARTESIAN_POINT ( 'NONE',  ( -43.00000337463111322, 77.94228634059959404, 17.49999999999999645 ) ) ;
#21935=CARTESIAN_POINT ( 'NONE',  ( 47.63139720814418610, 27.49999999999988987, -5.000000000000000000 ) ) ;
#21936=DIRECTION ( 'NONE',  ( 0.000000000000000000, 0.000000000000000000, 1.000000000000000000 ) ) ;
#21937=CARTESIAN_POINT ( 'NONE',  ( 52.99999662536844625, 60.62177826491077326, -9.999999999999998224 ) ) ;
#21938=ORIENTED_EDGE ( 'NONE', *, *, #17262, .F. ) ;
#21942=ORIENTED_EDGE ( 'NONE', *, *, #23634, .F. ) ;
#21943=EDGE_CURVE ( 'NONE', #10270, #3670, #16274, .T. ) ;
#21945=CARTESIAN_POINT ( 'NONE',  ( 56.99999662536844625, -60.62177826491080168, -9.999999999999998224 ) ) ;
#21946=VERTEX_POINT ( 'NONE', #34958 ) ;
#21948=AXIS2_PLACEMENT_3D ( 'NONE', #21449, #33062, #18644 ) ;
#21949=AXIS2_PLACEMENT_3D ( 'NONE', #1320, #3530, #15519 ) ;
#21950=DIRECTION ( 'NONE',  ( 0.000000000000000000, 0.000000000000000000, 1.000000000000000000 ) ) ;
#21953=AXIS2_PLACEMENT_3D ( 'NONE', #15309, #1255, #21505 ) ;
#21954=EDGE_CURVE ( 'NONE', #5770, #21147, #33043, .T. ) ;
#21956=EDGE_LOOP ( 'NONE', ( #35383, #11099, #1982, #31826, #12042 ) ) ;
#21957=EDGE_LOOP ( 'NONE', ( #22378, #11564, #29482, #15075 ) ) ;
#21958=CIRCLE ( 'NONE', #10585, 3.499999999999991562 ) ;
#21959=VERTEX_POINT ( 'NONE', #15642 ) ;
#21960=CARTESIAN_POINT ( 'NONE',  ( -56.67878100130369035, 27.78182860042797131, 12.49999999999999822 ) ) ;
#21962=DIRECTION ( 'NONE',  ( 0.000000000000000000, 0.000000000000000000, 1.000000000000000000 ) ) ;
#21963=CARTESIAN_POINT ( 'NONE',  ( 69.99999662536839651, 17.32050807568879236, -9.999999999999998224 ) ) ;
#21964=CARTESIAN_POINT ( 'NONE',  ( -52.00000337463109190, 51.96152422706637708, -9.999999999999998224 ) ) ;
#21965=ORIENTED_EDGE ( 'NONE', *, *, #28677, .T. ) ;
#21966=DIRECTION ( 'NONE',  ( 0.000000000000000000, 0.000000000000000000, 1.000000000000000000 ) ) ;
#21967=EDGE_CURVE ( 'NONE', #7306, #17105, #95, .T. ) ;
#21969=CIRCLE ( 'NONE', #9970, 2.000000000000001776 ) ;
#21970=CARTESIAN_POINT ( 'NONE',  ( 69.99999662536838230, -51.96152422706639840, -9.999999999999998224 ) ) ;
#21971=ORIENTED_EDGE ( 'NONE', *, *, #607, .T. ) ;
#21972=DIRECTION ( 'NONE',  ( -1.000000000000000000, 8.737866397512802015E-15, 0.000000000000000000 ) ) ;
#21973=CARTESIAN_POINT ( 'NONE',  ( -75.00000337463097821, 43.30127018922197379, 12.50000000000000000 ) ) ;
#21974=AXIS2_PLACEMENT_3D ( 'NONE', #16240, #30282, #23945 ) ;
#21975=VERTEX_POINT ( 'NONE', #26892 ) ;
#21976=EDGE_CURVE ( 'NONE', #8413, #31278, #1562, .T. ) ;
#21977=CIRCLE ( 'NONE', #19600, 2.000000000000001776 ) ;
#21978=ORIENTED_EDGE ( 'NONE', *, *, #21405, .T. ) ;
#21979=AXIS2_PLACEMENT_3D ( 'NONE', #1941, #36637, #4778 ) ;
#21980=EDGE_CURVE ( 'NONE', #27665, #1500, #21046, .T. ) ;
#21981=CYLINDRICAL_SURFACE ( 'NONE', #29479, 2.000000000000001776 ) ;
#21984=VERTEX_POINT ( 'NONE', #12438 ) ;
#21985=ORIENTED_EDGE ( 'NONE', *, *, #11357, .T. ) ;
#21986=ORIENTED_EDGE ( 'NONE', *, *, #24153, .T. ) ;
#21987=VECTOR ( 'NONE', #8481, 1000.000000000000000 ) ;
#21988=FACE_BOUND ( 'NONE', #3259, .T. ) ;
#21989=VERTEX_POINT ( 'NONE', #18249 ) ;
#21990=AXIS2_PLACEMENT_3D ( 'NONE', #31350, #28739, #34203 ) ;
#21991=CYLINDRICAL_SURFACE ( 'NONE', #23779, 2.000000000000001776 ) ;
#21992=ORIENTED_EDGE ( 'NONE', *, *, #17873, .T. ) ;
#21993=AXIS2_PLACEMENT_3D ( 'NONE', #6562, #17799, #25875 ) ;
#21994=VERTEX_POINT ( 'NONE', #23702 ) ;
#21995=DIRECTION ( 'NONE',  ( 0.000000000000000000, 0.000000000000000000, 1.000000000000000000 ) ) ;
#21996=EDGE_CURVE ( 'NONE', #6695, #21745, #702, .T. ) ;
#21997=AXIS2_PLACEMENT_3D ( 'NONE', #27637, #27812, #4595 ) ;
#21998=CARTESIAN_POINT ( 'NONE',  ( -38.00000337463113453, 69.28203230275516944, 17.49999999999999645 ) ) ;
#21999=VERTEX_POINT ( 'NONE', #21636 ) ;
#22000=ORIENTED_EDGE ( 'NONE', *, *, #16787, .T. ) ;
#22001=CARTESIAN_POINT ( 'NONE',  ( 49.99999662536846756, 69.28203230275516944, 12.50000000000000000 ) ) ;
#22002=CARTESIAN_POINT ( 'NONE',  ( 19.99999662536861678, -69.28203230275519786, -9.999999999999998224 ) ) ;
#22003=AXIS2_PLACEMENT_3D ( 'NONE', #30826, #5162, #1969 ) ;
#22004=AXIS2_PLACEMENT_3D ( 'NONE', #34842, #23409, #34471 ) ;
#22007=VECTOR ( 'NONE', #23512, 1000.000000000000000 ) ;
#22008=ORIENTED_EDGE ( 'NONE', *, *, #27736, .T. ) ;
#22009=DIRECTION ( 'NONE',  ( 0.000000000000000000, 0.000000000000000000, 1.000000000000000000 ) ) ;
#22010=FACE_BOUND ( 'NONE', #13260, .T. ) ;
#22011=DIRECTION ( 'NONE',  ( -1.000000000000000000, 0.000000000000000000, 0.000000000000000000 ) ) ;
#22012=FACE_BOUND ( 'NONE', #355, .T. ) ;
#22013=AXIS2_PLACEMENT_3D ( 'NONE', #14955, #31632, #12100 ) ;
#22014=CARTESIAN_POINT ( 'NONE',  ( 24.99999662536859546, -77.94228634059960825, 12.50000000000000000 ) ) ;
#22015=CARTESIAN_POINT ( 'NONE',  ( 14.99999662536863632, -77.94228634059960825, -9.999999999999998224 ) ) ;
#22016=EDGE_CURVE ( 'NONE', #33332, #2655, #7893, .T. ) ;
#22017=DIRECTION ( 'NONE',  ( -0.000000000000000000, -0.000000000000000000, 1.000000000000000000 ) ) ;
#22021=EDGE_CURVE ( 'NONE', #9668, #30108, #10008, .T. ) ;
#22022=CARTESIAN_POINT ( 'NONE',  ( -80.00000337463094979, -2.428612866367529932E-14, -5.000000000000000000 ) ) ;
#22023=AXIS2_PLACEMENT_3D ( 'NONE', #670, #31783, #28964 ) ;
#22024=CIRCLE ( 'NONE', #35820, 2.000000000000001776 ) ;
#22025=CARTESIAN_POINT ( 'NONE',  ( -2.000003374631334818, 69.28203230275516944, 17.49999999999999645 ) ) ;
#22026=LINE ( 'NONE', #19225, #33720 ) ;
#22027=AXIS2_PLACEMENT_3D ( 'NONE', #14481, #28540, #31717 ) ;
#22028=EDGE_LOOP ( 'NONE', ( #29119, #2652, #31844, #8631 ) ) ;
#22029=ADVANCED_FACE ( 'NONE', ( #24250 ), #12230, .F. ) ;
#22030=ORIENTED_EDGE ( 'NONE', *, *, #31399, .T. ) ;
#22031=ORIENTED_EDGE ( 'NONE', *, *, #15370, .F. ) ;
#22032=CIRCLE ( 'NONE', #2272, 27.00000000000001776 ) ;
#22033=DIRECTION ( 'NONE',  ( 1.000000000000000000, 0.000000000000000000, 0.000000000000000000 ) ) ;
#22034=CYLINDRICAL_SURFACE ( 'NONE', #15763, 2.000000000000001776 ) ;
#22036=VERTEX_POINT ( 'NONE', #21250 ) ;
#22037=EDGE_CURVE ( 'NONE', #2002, #13910, #21450, .T. ) ;
#22038=CARTESIAN_POINT ( 'NONE',  ( -75.00000337463099243, -25.98076211353322051, -9.999999999999998224 ) ) ;
#22039=CARTESIAN_POINT ( 'NONE',  ( 0.000000000000000000, 0.000000000000000000, -10.00000000000000000 ) ) ;
#22040=ORIENTED_EDGE ( 'NONE', *, *, #31, .T. ) ;
#22042=ORIENTED_EDGE ( 'NONE', *, *, #35104, .F. ) ;
#22043=FACE_BOUND ( 'NONE', #12012, .T. ) ;
#22045=EDGE_CURVE ( 'NONE', #26530, #11321, #15814, .T. ) ;
#22047=CARTESIAN_POINT ( 'NONE',  ( -70.00000337463102085, -51.96152422706641971, -5.000000000000000000 ) ) ;
#22050=AXIS2_PLACEMENT_3D ( 'NONE', #6045, #3767, #28728 ) ;
#22053=ADVANCED_FACE ( 'NONE', ( #1376 ), #1207, .T. ) ;
#22055=CARTESIAN_POINT ( 'NONE',  ( 25.30168577890723469, -79.91940132325416357, -5.000000000000000000 ) ) ;
#22057=VECTOR ( 'NONE', #6365, 1000.000000000000000 ) ;
#22059=AXIS2_PLACEMENT_3D ( 'NONE', #20950, #3140, #32180 ) ;
#22060=CARTESIAN_POINT ( 'NONE',  ( -30.00000337463118427, 69.28203230275516944, 17.49999999999999645 ) ) ;
#22062=CIRCLE ( 'NONE', #15471, 2.000000000000001776 ) ;
#22063=ORIENTED_EDGE ( 'NONE', *, *, #17378, .F. ) ;
#22064=DIRECTION ( 'NONE',  ( 1.000000000000000000, 0.000000000000000000, 0.000000000000000000 ) ) ;
#22065=CARTESIAN_POINT ( 'NONE',  ( 79.99999662536833966, 17.32050807568879236, 12.50000000000000000 ) ) ;
#22067=CARTESIAN_POINT ( 'NONE',  ( 32.99999662536855283, 60.62177826491078747, 17.49999999999999645 ) ) ;
#22068=CARTESIAN_POINT ( 'NONE',  ( -63.00000337463102085, 43.30127018922198801, 12.50000000000000000 ) ) ;
#22069=CARTESIAN_POINT ( 'NONE',  ( 34.99999662536855283, -77.94228634059960825, -5.000000000000000000 ) ) ;
#22072=EDGE_LOOP ( 'NONE', ( #398, #12524 ) ) ;
#22073=LINE ( 'NONE', #21687, #9977 ) ;
#22077=VERTEX_POINT ( 'NONE', #18821 ) ;
#22079=VECTOR ( 'NONE', #28133, 1000.000000000000000 ) ;
#22082=CIRCLE ( 'NONE', #1084, 2.000000000000001776 ) ;
#22083=DIRECTION ( 'NONE',  ( -1.000000000000000000, 0.000000000000000000, 0.000000000000000000 ) ) ;
#22084=LINE ( 'NONE', #33528, #20376 ) ;
#22085=ORIENTED_EDGE ( 'NONE', *, *, #30510, .F. ) ;
#22086=ORIENTED_EDGE ( 'NONE', *, *, #1170, .F. ) ;
#22087=CARTESIAN_POINT ( 'NONE',  ( 2.778182860043481472, 66.86787810013034061, -4.999999999999997335 ) ) ;
#22088=AXIS2_PLACEMENT_3D ( 'NONE', #21567, #4314, #32996 ) ;
#22089=FACE_OUTER_BOUND ( 'NONE', #28492, .T. ) ;
#22090=ORIENTED_EDGE ( 'NONE', *, *, #25143, .T. ) ;
#22093=EDGE_LOOP ( 'NONE', ( #2805, #19332 ) ) ;
#22094=DIRECTION ( 'NONE',  ( 0.000000000000000000, 0.000000000000000000, 1.000000000000000000 ) ) ;
#22096=CARTESIAN_POINT ( 'NONE',  ( -3.374631289687624047E-06, -69.28203230275519786, -9.999999999999998224 ) ) ;
#22097=EDGE_CURVE ( 'NONE', #3118, #26973, #31810, .T. ) ;
#22099=ORIENTED_EDGE ( 'NONE', *, *, #7074, .T. ) ;
#22102=DIRECTION ( 'NONE',  ( 1.000000000000000000, 0.000000000000000000, 0.000000000000000000 ) ) ;
#22103=AXIS2_PLACEMENT_3D ( 'NONE', #2583, #11009, #25454 ) ;
#22104=DIRECTION ( 'NONE',  ( 1.000000000000000000, 0.000000000000000000, 0.000000000000000000 ) ) ;
#22105=PLANE ( 'NONE',  #17923 ) ;
#22106=ORIENTED_EDGE ( 'NONE', *, *, #27672, .F. ) ;
#22107=CARTESIAN_POINT ( 'NONE',  ( 69.99999662536839651, 17.32050807568879236, -5.000000000000000000 ) ) ;
#22108=CIRCLE ( 'NONE', #33489, 2.000000000000001776 ) ;
#22110=CARTESIAN_POINT ( 'NONE',  ( -48.00000337463109190, 69.28203230275518365, 12.50000000000000000 ) ) ;
#22111=ORIENTED_EDGE ( 'NONE', *, *, #16808, .F. ) ;
#22112=ORIENTED_EDGE ( 'NONE', *, *, #2638, .T. ) ;
#22113=VECTOR ( 'NONE', #22219, 1000.000000000000000 ) ;
#22116=DIRECTION ( 'NONE',  ( 0.000000000000000000, 0.000000000000000000, 1.000000000000000000 ) ) ;
#22117=DIRECTION ( 'NONE',  ( -1.000000000000000000, 0.000000000000000000, 0.000000000000000000 ) ) ;
#22120=PLANE ( 'NONE',  #13226 ) ;
#22122=DIRECTION ( 'NONE',  ( 1.000000000000000000, 0.000000000000000000, 0.000000000000000000 ) ) ;
#22123=AXIS2_PLACEMENT_3D ( 'NONE', #32511, #6826, #18262 ) ;
#22126=LINE ( 'NONE', #19676, #20209 ) ;
#22128=ORIENTED_EDGE ( 'NONE', *, *, #28832, .T. ) ;
#22129=ORIENTED_EDGE ( 'NONE', *, *, #6240, .F. ) ;
#22130=AXIS2_PLACEMENT_3D ( 'NONE', #12941, #16329, #1889 ) ;
#22132=CIRCLE ( 'NONE', #25719, 2.000000000000001776 ) ;
#22133=DIRECTION ( 'NONE',  ( 0.000000000000000000, 0.000000000000000000, 1.000000000000000000 ) ) ;
#22134=CARTESIAN_POINT ( 'NONE',  ( 69.61830985333858735, 36.60425714729669977, 12.50000000000000000 ) ) ;
#22135=DIRECTION ( 'NONE',  ( 0.000000000000000000, 0.000000000000000000, 1.000000000000000000 ) ) ;
#22136=VERTEX_POINT ( 'NONE', #36449 ) ;
#22139=DIRECTION ( 'NONE',  ( 0.000000000000000000, 0.000000000000000000, 1.000000000000000000 ) ) ;
#22140=ORIENTED_EDGE ( 'NONE', *, *, #26612, .F. ) ;
#22142=FACE_OUTER_BOUND ( 'NONE', #26151, .T. ) ;
#22143=ORIENTED_EDGE ( 'NONE', *, *, #14543, .T. ) ;
#22144=AXIS2_PLACEMENT_3D ( 'NONE', #26964, #14979, #35031 ) ;
#22145=CARTESIAN_POINT ( 'NONE',  ( 76.99999662536835388, -25.98076211353319565, 17.49999999999999645 ) ) ;
#22146=FACE_OUTER_BOUND ( 'NONE', #1454, .T. ) ;
#22147=AXIS2_PLACEMENT_3D ( 'NONE', #3093, #2361, #85 ) ;
#22148=CARTESIAN_POINT ( 'NONE',  ( -88.00000337463090716, -1.040834085586084257E-14, -9.999999999999998224 ) ) ;
#22149=ORIENTED_EDGE ( 'NONE', *, *, #9684, .F. ) ;
#22150=VERTEX_POINT ( 'NONE', #10923 ) ;
#22151=AXIS2_PLACEMENT_3D ( 'NONE', #13006, #18258, #33069 ) ;
#22152=ORIENTED_EDGE ( 'NONE', *, *, #28430, .F. ) ;
#22153=DIRECTION ( 'NONE',  ( 0.000000000000000000, 0.000000000000000000, 1.000000000000000000 ) ) ;
#22154=EDGE_CURVE ( 'NONE', #20878, #18995, #9081, .T. ) ;
#22155=DIRECTION ( 'NONE',  ( -0.000000000000000000, -0.000000000000000000, 1.000000000000000000 ) ) ;
#22156=AXIS2_PLACEMENT_3D ( 'NONE', #19836, #22449, #19653 ) ;
#22157=CARTESIAN_POINT ( 'NONE',  ( -62.00000337463108480, -51.96152422706641971, 17.49999999999999645 ) ) ;
#22158=CARTESIAN_POINT ( 'NONE',  ( 52.39915983220795681, 35.19434990244919703, 12.49999999999999822 ) ) ;
#22160=EDGE_CURVE ( 'NONE', #28884, #35505, #11103, .T. ) ;
#22161=ORIENTED_EDGE ( 'NONE', *, *, #22187, .F. ) ;
#22162=DIRECTION ( 'NONE',  ( 0.000000000000000000, 0.000000000000000000, 1.000000000000000000 ) ) ;
#22163=CARTESIAN_POINT ( 'NONE',  ( -66.50936994187880202, 41.98909163213660634, 12.50000000000000000 ) ) ;
#22164=DIRECTION ( 'NONE',  ( -1.000000000000000000, 0.000000000000000000, 0.000000000000000000 ) ) ;
#22165=ORIENTED_EDGE ( 'NONE', *, *, #6465, .T. ) ;
#22166=CARTESIAN_POINT ( 'NONE',  ( 4.279621169095998212, -62.97617850287780072, -4.999999999999997335 ) ) ;
#22170=ORIENTED_EDGE ( 'NONE', *, *, #27375, .T. ) ;
#22171=ORIENTED_EDGE ( 'NONE', *, *, #8694, .T. ) ;
#22172=EDGE_CURVE ( 'NONE', #15168, #19680, #9685, .T. ) ;
#22174=DIRECTION ( 'NONE',  ( -1.156482317317870344E-14, -1.000000000000000000, 0.000000000000000000 ) ) ;
#22175=VECTOR ( 'NONE', #25380, 1000.000000000000000 ) ;
#22176=CARTESIAN_POINT ( 'NONE',  ( -90.60231327712325822, -15.97563234535699017, 12.49999999999999822 ) ) ;
#22178=ORIENTED_EDGE ( 'NONE', *, *, #32355, .F. ) ;
#22179=ORIENTED_EDGE ( 'NONE', *, *, #25459, .T. ) ;
#22182=CIRCLE ( 'NONE', #14387, 27.00000000000001421 ) ;
#22184=FACE_OUTER_BOUND ( 'NONE', #4387, .T. ) ;
#22185=ORIENTED_EDGE ( 'NONE', *, *, #15843, .F. ) ;
#22187=EDGE_CURVE ( 'NONE', #21959, #19593, #32417, .T. ) ;
#22188=CARTESIAN_POINT ( 'NONE',  ( -23.00000337463120559, 77.94228634059957983, 12.50000000000000000 ) ) ;
#22189=DIRECTION ( 'NONE',  ( 1.000000000000000000, 0.000000000000000000, -0.000000000000000000 ) ) ;
#22190=ORIENTED_EDGE ( 'NONE', *, *, #35057, .T. ) ;
#22191=ORIENTED_EDGE ( 'NONE', *, *, #18620, .T. ) ;
#22192=PLANE ( 'NONE',  #31090 ) ;
#22194=EDGE_CURVE ( 'NONE', #9891, #3388, #30620, .T. ) ;
#22195=DIRECTION ( 'NONE',  ( -1.000000000000000000, 0.000000000000000000, 0.000000000000000000 ) ) ;
#22196=DIRECTION ( 'NONE',  ( 1.000000000000000000, 0.000000000000000000, 0.000000000000000000 ) ) ;
#22198=CARTESIAN_POINT ( 'NONE',  ( -65.00000337463104927, -25.98076211353322051, -9.999999999999998224 ) ) ;
#22199=EDGE_CURVE ( 'NONE', #14210, #9631, #19207, .T. ) ;
#22200=CIRCLE ( 'NONE', #35967, 3.499999999999989342 ) ;
#22201=FACE_BOUND ( 'NONE', #17793, .T. ) ;
#22202=DIRECTION ( 'NONE',  ( 0.000000000000000000, 0.000000000000000000, -1.000000000000000000 ) ) ;
#22203=DIRECTION ( 'NONE',  ( 1.000000000000000000, 0.000000000000000000, -0.000000000000000000 ) ) ;
#22204=FACE_OUTER_BOUND ( 'NONE', #1046, .T. ) ;
#22205=CARTESIAN_POINT ( 'NONE',  ( -15.00000337463126066, 77.94228634059957983, -9.999999999999998224 ) ) ;
#22206=CARTESIAN_POINT ( 'NONE',  ( 34.99999662536855283, 60.62177826491078747, -9.999999999999998224 ) ) ;
#22207=CARTESIAN_POINT ( 'NONE',  ( 47.99999662536848177, -51.96152422706640550, -9.999999999999998224 ) ) ;
#22208=EDGE_LOOP ( 'NONE', ( #18056, #13888 ) ) ;
#22209=LINE ( 'NONE', #18658, #26197 ) ;
#22212=VERTEX_POINT ( 'NONE', #13921 ) ;
#22213=EDGE_LOOP ( 'NONE', ( #12550, #32256, #27212, #27772 ) ) ;
#22214=VERTEX_POINT ( 'NONE', #7566 ) ;
#22215=ADVANCED_FACE ( 'NONE', ( #22363 ), #30994, .F. ) ;
#22216=CARTESIAN_POINT ( 'NONE',  ( 29.97040607558719572, -71.28181339061548272, 12.50000000000000000 ) ) ;
#22217=CARTESIAN_POINT ( 'NONE',  ( 49.99999662536846756, 51.96152422706637708, -9.999999999999998224 ) ) ;
#22218=ORIENTED_EDGE ( 'NONE', *, *, #30281, .T. ) ;
#22219=DIRECTION ( 'NONE',  ( 0.000000000000000000, 0.000000000000000000, 1.000000000000000000 ) ) ;
#22220=DIRECTION ( 'NONE',  ( 0.000000000000000000, 0.000000000000000000, 1.000000000000000000 ) ) ;
#22221=EDGE_LOOP ( 'NONE', ( #24645, #14551, #17757, #4842, #1812, #24953, #35958, #6417, #32393, #25639, #4990, #8712 ) ) ;
#22222=CIRCLE ( 'NONE', #35411, 27.00000000000001421 ) ;
#22223=CARTESIAN_POINT ( 'NONE',  ( 54.99999662536844625, 43.30127018922198801, -9.999999999999998224 ) ) ;
#22224=ORIENTED_EDGE ( 'NONE', *, *, #7338, .T. ) ;
#22225=CARTESIAN_POINT ( 'NONE',  ( 19.99999662536857770, 86.60254037844397601, -9.999999999999998224 ) ) ;
#22226=ADVANCED_FACE ( 'NONE', ( #8322 ), #5327, .F. ) ;
#22227=DIRECTION ( 'NONE',  ( 0.000000000000000000, 0.000000000000000000, 1.000000000000000000 ) ) ;
#22229=EDGE_CURVE ( 'NONE', #15168, #16940, #13752, .T. ) ;
#22230=VERTEX_POINT ( 'NONE', #31182 ) ;
#22233=CARTESIAN_POINT ( 'NONE',  ( 2.999996625368676728, -77.94228634059960825, -9.999999999999998224 ) ) ;
#22234=CARTESIAN_POINT ( 'NONE',  ( -5.000003374631269537, -77.94228634059960825, -5.000000000000000000 ) ) ;
#22235=VERTEX_POINT ( 'NONE', #27442 ) ;
#22236=DIRECTION ( 'NONE',  ( 1.000000000000000000, 0.000000000000000000, 0.000000000000000000 ) ) ;
#22237=CARTESIAN_POINT ( 'NONE',  ( -56.74224907228983739, 68.66839587347264739, 12.49999999999999645 ) ) ;
#22238=EDGE_CURVE ( 'NONE', #16919, #22507, #19016, .T. ) ;
#22239=VERTEX_POINT ( 'NONE', #4771 ) ;
#22240=DIRECTION ( 'NONE',  ( 1.000000000000000000, 0.000000000000000000, 0.000000000000000000 ) ) ;
#22241=EDGE_CURVE ( 'NONE', #31097, #17803, #34242, .T. ) ;
#22242=AXIS2_PLACEMENT_3D ( 'NONE', #33380, #7694, #27923 ) ;
#22243=DIRECTION ( 'NONE',  ( 0.000000000000000000, -0.000000000000000000, -1.000000000000000000 ) ) ;
#22244=DIRECTION ( 'NONE',  ( 1.000000000000000000, 0.000000000000000000, 0.000000000000000000 ) ) ;
#22246=ORIENTED_EDGE ( 'NONE', *, *, #12132, .F. ) ;
#22248=CARTESIAN_POINT ( 'NONE',  ( 7.999996625368656744, -86.60254037844400443, -9.999999999999998224 ) ) ;
#22249=CARTESIAN_POINT ( 'NONE',  ( 90.60231327712337190, 15.97563234535636134, -4.999999999999997335 ) ) ;
#22250=EDGE_CURVE ( 'NONE', #1670, #22617, #10654, .T. ) ;
#22251=ADVANCED_FACE ( 'NONE', ( #31344 ), #12015, .F. ) ;
#22253=ORIENTED_EDGE ( 'NONE', *, *, #33685, .F. ) ;
#22254=EDGE_LOOP ( 'NONE', ( #6633, #21118, #96, #6020, #11010, #28363 ) ) ;
#22255=EDGE_CURVE ( 'NONE', #34871, #30085, #28603, .T. ) ;
#22256=LINE ( 'NONE', #13628, #7439 ) ;
#22258=DIRECTION ( 'NONE',  ( 0.000000000000000000, 0.000000000000000000, 1.000000000000000000 ) ) ;
#22259=ORIENTED_EDGE ( 'NONE', *, *, #11263, .T. ) ;
#22260=ORIENTED_EDGE ( 'NONE', *, *, #36629, .T. ) ;
#22261=DIRECTION ( 'NONE',  ( -1.000000000000000000, 0.000000000000000000, 0.000000000000000000 ) ) ;
#22263=DIRECTION ( 'NONE',  ( 1.000000000000000000, 0.000000000000000000, 0.000000000000000000 ) ) ;
#22265=CARTESIAN_POINT ( 'NONE',  ( -31.83425564451526668, -89.42901512340343118, -49.86348611802629449 ) ) ;
#22268=FACE_BOUND ( 'NONE', #22664, .T. ) ;
#22269=EDGE_CURVE ( 'NONE', #20675, #21723, #25038, .T. ) ;
#22270=FACE_OUTER_BOUND ( 'NONE', #7297, .T. ) ;
#22273=EDGE_LOOP ( 'NONE', ( #1274, #36221, #34623, #16699 ) ) ;
#22275=CARTESIAN_POINT ( 'NONE',  ( 74.99999662536836809, 8.660254037844394404, -9.999999999999998224 ) ) ;
#22277=FACE_OUTER_BOUND ( 'NONE', #3603, .T. ) ;
#22278=VERTEX_POINT ( 'NONE', #34549 ) ;
#22279=DIRECTION ( 'NONE',  ( 0.000000000000000000, 0.000000000000000000, 1.000000000000000000 ) ) ;
#22280=EDGE_CURVE ( 'NONE', #36878, #18695, #3450, .T. ) ;
#22281=FACE_OUTER_BOUND ( 'NONE', #12883, .T. ) ;
#22283=EDGE_LOOP ( 'NONE', ( #22633, #29550, #25136, #27615 ) ) ;
#22284=ORIENTED_EDGE ( 'NONE', *, *, #20746, .T. ) ;
#22285=AXIS2_PLACEMENT_3D ( 'NONE', #35110, #24040, #9774 ) ;
#22286=CARTESIAN_POINT ( 'NONE',  ( 42.99999662536850309, -60.62177826491080168, -5.000000000000000000 ) ) ;
#22288=DIRECTION ( 'NONE',  ( 0.000000000000000000, 0.000000000000000000, 1.000000000000000000 ) ) ;
#22290=EDGE_CURVE ( 'NONE', #34086, #14414, #23819, .T. ) ;
#22291=EDGE_CURVE ( 'NONE', #8626, #18158, #7034, .T. ) ;
#22292=DIRECTION ( 'NONE',  ( 1.000000000000000000, 0.000000000000000000, 0.000000000000000000 ) ) ;
#22293=ADVANCED_FACE ( 'NONE', ( #3416 ), #11838, .F. ) ;
#22294=EDGE_CURVE ( 'NONE', #9342, #26254, #49, .T. ) ;
#22301=VERTEX_POINT ( 'NONE', #36999 ) ;
#22302=VECTOR ( 'NONE', #29270, 1000.000000000000000 ) ;
#22304=CARTESIAN_POINT ( 'NONE',  ( 67.99999662536838230, -3.224517592124143893E-15, -9.999999999999998224 ) ) ;
#22305=FACE_OUTER_BOUND ( 'NONE', #33114, .T. ) ;
#22307=LINE ( 'NONE', #33749, #6529 ) ;
#22308=VERTEX_POINT ( 'NONE', #23098 ) ;
#22310=FACE_OUTER_BOUND ( 'NONE', #19344, .T. ) ;
#22311=ORIENTED_EDGE ( 'NONE', *, *, #21249, .F. ) ;
#22314=DIRECTION ( 'NONE',  ( 0.000000000000000000, 0.000000000000000000, 1.000000000000000000 ) ) ;
#22315=EDGE_LOOP ( 'NONE', ( #5866, #2250 ) ) ;
#22316=EDGE_CURVE ( 'NONE', #11237, #29382, #9208, .T. ) ;
#22318=CARTESIAN_POINT ( 'NONE',  ( 32.99999662536855283, -77.94228634059960825, 12.50000000000000000 ) ) ;
#22319=DIRECTION ( 'NONE',  ( 1.000000000000000000, 0.000000000000000000, 0.000000000000000000 ) ) ;
#22321=ORIENTED_EDGE ( 'NONE', *, *, #3932, .T. ) ;
#22322=EDGE_LOOP ( 'NONE', ( #14604, #6438 ) ) ;
#22323=CIRCLE ( 'NONE', #6761, 33.00000000000002132 ) ;
#22324=ORIENTED_EDGE ( 'NONE', *, *, #13487, .F. ) ;
#22325=CARTESIAN_POINT ( 'NONE',  ( 74.99999662536836809, -8.660254037844401509, 12.50000000000000000 ) ) ;
#22326=DIRECTION ( 'NONE',  ( 1.000000000000000000, 0.000000000000000000, 0.000000000000000000 ) ) ;
#22327=DIRECTION ( 'NONE',  ( 0.000000000000000000, 0.000000000000000000, 1.000000000000000000 ) ) ;
#22328=CYLINDRICAL_SURFACE ( 'NONE', #24107, 2.000000000000000000 ) ;
#22330=ORIENTED_EDGE ( 'NONE', *, *, #8848, .F. ) ;
#22331=DIRECTION ( 'NONE',  ( 0.000000000000000000, 0.000000000000000000, 1.000000000000000000 ) ) ;
#22332=DIRECTION ( 'NONE',  ( -1.000000000000000000, 0.000000000000000000, 0.000000000000000000 ) ) ;
#22333=VECTOR ( 'NONE', #22666, 1000.000000000000000 ) ;
#22334=ADVANCED_FACE ( 'NONE', ( #25756 ), #17306, .F. ) ;
#22336=EDGE_LOOP ( 'NONE', ( #21034, #35446, #30425, #3177 ) ) ;
#22338=CYLINDRICAL_SURFACE ( 'NONE', #20836, 2.000000000000001776 ) ;
#22339=CYLINDRICAL_SURFACE ( 'NONE', #17163, 27.00000000000001421 ) ;
#22341=VERTEX_POINT ( 'NONE', #16923 ) ;
#22344=DIRECTION ( 'NONE',  ( 1.000000000000000000, 0.000000000000000000, 0.000000000000000000 ) ) ;
#22348=FACE_BOUND ( 'NONE', #21158, .T. ) ;
#22349=CIRCLE ( 'NONE', #14574, 3.000000000000002665 ) ;
#22350=VERTEX_POINT ( 'NONE', #14102 ) ;
#22353=EDGE_CURVE ( 'NONE', #20996, #20810, #4665, .T. ) ;
#22354=ORIENTED_EDGE ( 'NONE', *, *, #25844, .T. ) ;
#22355=DIRECTION ( 'NONE',  ( -1.000000000000000000, 0.000000000000000000, 0.000000000000000000 ) ) ;
#22356=CIRCLE ( 'NONE', #11554, 2.000000000000001776 ) ;
#22357=DIRECTION ( 'NONE',  ( 1.000000000000000000, 0.000000000000000000, 0.000000000000000000 ) ) ;
#22360=ORIENTED_EDGE ( 'NONE', *, *, #15790, .F. ) ;
#22361=CYLINDRICAL_SURFACE ( 'NONE', #35896, 2.000000000000001776 ) ;
#22362=DIRECTION ( 'NONE',  ( 0.000000000000000000, 0.000000000000000000, 1.000000000000000000 ) ) ;
#22363=FACE_OUTER_BOUND ( 'NONE', #13109, .T. ) ;
#22365=EDGE_CURVE ( 'NONE', #31133, #15574, #11801, .T. ) ;
#22366=VERTEX_POINT ( 'NONE', #8491 ) ;
#22367=FACE_OUTER_BOUND ( 'NONE', #26312, .T. ) ;
#22368=FACE_BOUND ( 'NONE', #9667, .T. ) ;
#22369=DIRECTION ( 'NONE',  ( -1.000000000000000000, 0.000000000000000000, 0.000000000000000000 ) ) ;
#22370=CIRCLE ( 'NONE', #28939, 2.000000000000001776 ) ;
#22371=DIRECTION ( 'NONE',  ( 0.000000000000000000, 0.000000000000000000, 1.000000000000000000 ) ) ;
#22372=CARTESIAN_POINT ( 'NONE',  ( -22.00000337463124112, -69.28203230275522628, -9.999999999999998224 ) ) ;
#22373=DIRECTION ( 'NONE',  ( 1.000000000000000000, 0.000000000000000000, 0.000000000000000000 ) ) ;
#22374=VECTOR ( 'NONE', #3534, 1000.000000000000000 ) ;
#22375=CARTESIAN_POINT ( 'NONE',  ( 69.99999662536839651, -17.32050807568879947, -5.000000000000000000 ) ) ;
#22376=EDGE_CURVE ( 'NONE', #14128, #575, #23201, .T. ) ;
#22377=DIRECTION ( 'NONE',  ( 0.000000000000000000, 0.000000000000000000, 1.000000000000000000 ) ) ;
#22378=ORIENTED_EDGE ( 'NONE', *, *, #31754, .F. ) ;
#22379=CARTESIAN_POINT ( 'NONE',  ( -56.67878100130369035, 27.78182860042797131, -4.999999999999997335 ) ) ;
#22380=DIRECTION ( 'NONE',  ( 1.000000000000000000, 0.000000000000000000, 0.000000000000000000 ) ) ;
#22381=CARTESIAN_POINT ( 'NONE',  ( -55.00000337463110611, -43.30127018922202353, -9.999999999999998224 ) ) ;
#22382=AXIS2_PLACEMENT_3D ( 'NONE', #29926, #4251, #13399 ) ;
#22383=ORIENTED_EDGE ( 'NONE', *, *, #3892, .F. ) ;
#22384=VERTEX_POINT ( 'NONE', #31881 ) ;
#22386=AXIS2_PLACEMENT_3D ( 'NONE', #23870, #35318, #9615 ) ;
#22388=CARTESIAN_POINT ( 'NONE',  ( 30.89873427475420442, -67.49533964939347186, -5.000000000000000000 ) ) ;
#22390=EDGE_CURVE ( 'NONE', #15915, #25880, #16035, .T. ) ;
#22392=ORIENTED_EDGE ( 'NONE', *, *, #23310, .T. ) ;
#22393=EDGE_CURVE ( 'NONE', #32118, #3085, #13022, .T. ) ;
#22394=DIRECTION ( 'NONE',  ( -0.000000000000000000, -0.000000000000000000, 1.000000000000000000 ) ) ;
#22395=EDGE_LOOP ( 'NONE', ( #5027, #12708 ) ) ;
#22396=DIRECTION ( 'NONE',  ( 1.000000000000000000, 0.000000000000000000, 0.000000000000000000 ) ) ;
#22398=CARTESIAN_POINT ( 'NONE',  ( 76.99999662536836809, 43.30127018922198801, -9.999999999999998224 ) ) ;
#22399=CARTESIAN_POINT ( 'NONE',  ( 2.999996625368645198, 77.94228634059957983, 17.49999999999999645 ) ) ;
#22400=EDGE_CURVE ( 'NONE', #10468, #4318, #32778, .T. ) ;
#22402=DIRECTION ( 'NONE',  ( -1.000000000000000000, 0.000000000000000000, 0.000000000000000000 ) ) ;
#22404=DIRECTION ( 'NONE',  ( -1.000000000000000000, 0.000000000000000000, 0.000000000000000000 ) ) ;
#22406=EDGE_CURVE ( 'NONE', #12950, #36279, #30393, .T. ) ;
#22407=VERTEX_POINT ( 'NONE', #18029 ) ;
#22408=AXIS2_PLACEMENT_3D ( 'NONE', #34885, #24179, #15372 ) ;
#22409=CARTESIAN_POINT ( 'NONE',  ( -35.00000337463116296, 77.94228634059957983, 12.50000000000000000 ) ) ;
#22410=FACE_OUTER_BOUND ( 'NONE', #9490, .T. ) ;
#22411=ORIENTED_EDGE ( 'NONE', *, *, #28274, .T. ) ;
#22412=DIRECTION ( 'NONE',  ( 0.000000000000000000, 0.000000000000000000, -1.000000000000000000 ) ) ;
#22414=CARTESIAN_POINT ( 'NONE',  ( -69.61831313460106685, -36.60425647305652319, 12.50000000000000000 ) ) ;
#22416=ORIENTED_EDGE ( 'NONE', *, *, #17665, .F. ) ;
#22417=VERTEX_POINT ( 'NONE', #24357 ) ;
#22420=DIRECTION ( 'NONE',  ( 0.000000000000000000, 0.000000000000000000, 1.000000000000000000 ) ) ;
#22421=CIRCLE ( 'NONE', #31408, 2.000000000000001776 ) ;
#22422=ADVANCED_FACE ( 'NONE', ( #4477 ), #1465, .F. ) ;
#22424=VERTEX_POINT ( 'NONE', #10666 ) ;
#22425=CARTESIAN_POINT ( 'NONE',  ( 11.99999662536862566, 86.60254037844397601, -9.999999999999998224 ) ) ;
#22426=DIRECTION ( 'NONE',  ( -1.000000000000000000, 0.000000000000000000, 0.000000000000000000 ) ) ;
#22427=DIRECTION ( 'NONE',  ( 0.000000000000000000, 0.000000000000000000, 1.000000000000000000 ) ) ;
#22428=ORIENTED_EDGE ( 'NONE', *, *, #19101, .T. ) ;
#22429=CIRCLE ( 'NONE', #6261, 2.000000000000001776 ) ;
#22430=EDGE_CURVE ( 'NONE', #30579, #29460, #27346, .T. ) ;
#22431=AXIS2_PLACEMENT_3D ( 'NONE', #11424, #17785, #23593 ) ;
#22432=ORIENTED_EDGE ( 'NONE', *, *, #36460, .F. ) ;
#22433=DIRECTION ( 'NONE',  ( -1.000000000000000000, 0.000000000000000000, 0.000000000000000000 ) ) ;
#22435=DIRECTION ( 'NONE',  ( 0.000000000000000000, 0.000000000000000000, 1.000000000000000000 ) ) ;
#22436=ORIENTED_EDGE ( 'NONE', *, *, #32258, .F. ) ;
#22437=EDGE_CURVE ( 'NONE', #16822, #17617, #33355, .T. ) ;
#22438=DIRECTION ( 'NONE',  ( 1.000000000000000000, 0.000000000000000000, 0.000000000000000000 ) ) ;
#22439=ORIENTED_EDGE ( 'NONE', *, *, #2511, .T. ) ;
#22440=FACE_BOUND ( 'NONE', #17683, .T. ) ;
#22441=DIRECTION ( 'NONE',  ( 1.000000000000000000, 0.000000000000000000, 0.000000000000000000 ) ) ;
#22442=VECTOR ( 'NONE', #35400, 1000.000000000000000 ) ;
#22443=CIRCLE ( 'NONE', #23055, 2.000000000000001776 ) ;
#22446=AXIS2_PLACEMENT_3D ( 'NONE', #8245, #14415, #5437 ) ;
#22447=DIRECTION ( 'NONE',  ( 1.000000000000000000, 0.000000000000000000, 0.000000000000000000 ) ) ;
#22449=DIRECTION ( 'NONE',  ( 0.000000000000000000, 0.000000000000000000, 1.000000000000000000 ) ) ;
#22450=LINE ( 'NONE', #33901, #23898 ) ;
#22451=ORIENTED_EDGE ( 'NONE', *, *, #25651, .T. ) ;
#22452=DIRECTION ( 'NONE',  ( 1.000000000000000000, 0.000000000000000000, 0.000000000000000000 ) ) ;
#22453=DIRECTION ( 'NONE',  ( 0.000000000000000000, 0.000000000000000000, 1.000000000000000000 ) ) ;
#22454=CARTESIAN_POINT ( 'NONE',  ( 0.000000000000000000, 0.000000000000000000, 12.49999999999999822 ) ) ;
#22457=ORIENTED_EDGE ( 'NONE', *, *, #21456, .T. ) ;
#22458=ORIENTED_EDGE ( 'NONE', *, *, #15537, .T. ) ;
#22459=PLANE ( 'NONE',  #1747 ) ;
#22460=ORIENTED_EDGE ( 'NONE', *, *, #32946, .F. ) ;
#22461=DIRECTION ( 'NONE',  ( 0.000000000000000000, 0.000000000000000000, 1.000000000000000000 ) ) ;
#22463=DIRECTION ( 'NONE',  ( 0.000000000000000000, 0.000000000000000000, 1.000000000000000000 ) ) ;
#22464=EDGE_CURVE ( 'NONE', #16555, #4566, #19620, .T. ) ;
#22467=CARTESIAN_POINT ( 'NONE',  ( -17.00000337463126243, 77.94228634059957983, -9.999999999999998224 ) ) ;
#22469=EDGE_CURVE ( 'NONE', #16050, #29585, #13644, .T. ) ;
#22472=CIRCLE ( 'NONE', #27879, 2.000000000000001776 ) ;
#22473=FACE_OUTER_BOUND ( 'NONE', #26432, .T. ) ;
#22474=CIRCLE ( 'NONE', #13475, 2.000000000000000000 ) ;
#22475=ORIENTED_EDGE ( 'NONE', *, *, #16086, .F. ) ;
#22477=AXIS2_PLACEMENT_3D ( 'NONE', #35422, #20569, #23413 ) ;
#22478=ORIENTED_EDGE ( 'NONE', *, *, #9403, .T. ) ;
#22481=DIRECTION ( 'NONE',  ( 0.000000000000000000, 0.000000000000000000, 1.000000000000000000 ) ) ;
#22482=FACE_OUTER_BOUND ( 'NONE', #16200, .T. ) ;
#22483=EDGE_CURVE ( 'NONE', #10350, #27052, #2866, .T. ) ;
#22484=VERTEX_POINT ( 'NONE', #32275 ) ;
#22485=EDGE_CURVE ( 'NONE', #14513, #7356, #32173, .T. ) ;
#22486=AXIS2_PLACEMENT_3D ( 'NONE', #35568, #9859, #21300 ) ;
#22487=VECTOR ( 'NONE', #5190, 1000.000000000000000 ) ;
#22490=EDGE_LOOP ( 'NONE', ( #22909, #331, #18381, #25288 ) ) ;
#22491=CARTESIAN_POINT ( 'NONE',  ( -63.00000337463104927, -25.98076211353322051, -5.000000000000000000 ) ) ;
#22493=EDGE_CURVE ( 'NONE', #28322, #18808, #435, .T. ) ;
#22494=CYLINDRICAL_SURFACE ( 'NONE', #21389, 2.000000000000001776 ) ;
#22495=ADVANCED_FACE ( 'NONE', ( #10117 ), #7294, .T. ) ;
#22496=CYLINDRICAL_SURFACE ( 'NONE', #3852, 2.000000000000001776 ) ;
#22497=EDGE_CURVE ( 'NONE', #14414, #19227, #24730, .T. ) ;
#22498=CARTESIAN_POINT ( 'NONE',  ( -73.00000337463100664, -43.30127018922202353, 17.49999999999999645 ) ) ;
#22499=EDGE_CURVE ( 'NONE', #16356, #32680, #10466, .T. ) ;
#22500=ORIENTED_EDGE ( 'NONE', *, *, #24373, .T. ) ;
#22501=ORIENTED_EDGE ( 'NONE', *, *, #33924, .T. ) ;
#22502=AXIS2_PLACEMENT_3D ( 'NONE', #26570, #1439, #9884 ) ;
#22503=CIRCLE ( 'NONE', #11123, 2.000000000000001776 ) ;
#22504=EDGE_LOOP ( 'NONE', ( #10786, #6900, #5436, #20358 ) ) ;
#22505=AXIS2_PLACEMENT_3D ( 'NONE', #9675, #4415, #1595 ) ;
#22506=CIRCLE ( 'NONE', #15899, 2.000000000000001776 ) ;
#22507=VERTEX_POINT ( 'NONE', #2971 ) ;
#22509=DIRECTION ( 'NONE',  ( 0.000000000000000000, 0.000000000000000000, 1.000000000000000000 ) ) ;
#22510=CARTESIAN_POINT ( 'NONE',  ( 59.99999662536845335, 34.64101615137759893, 12.50000000000000000 ) ) ;
#22511=CARTESIAN_POINT ( 'NONE',  ( 34.99999662536855283, -77.94228634059960825, -9.999999999999998224 ) ) ;
#22512=AXIS2_PLACEMENT_3D ( 'NONE', #33118, #19260, #36517 ) ;
#22513=DIRECTION ( 'NONE',  ( 0.000000000000000000, 0.000000000000000000, 1.000000000000000000 ) ) ;
#22514=CARTESIAN_POINT ( 'NONE',  ( 64.99999662536839651, -43.30127018922199511, 12.50000000000000000 ) ) ;
#22516=DIRECTION ( 'NONE',  ( -1.000000000000000000, 0.000000000000000000, 0.000000000000000000 ) ) ;
#22517=CIRCLE ( 'NONE', #9934, 2.000000000000001776 ) ;
#22518=DIRECTION ( 'NONE',  ( 1.000000000000000000, 0.000000000000000000, 0.000000000000000000 ) ) ;
#22519=LINE ( 'NONE', #28864, #3830 ) ;
#22520=ORIENTED_EDGE ( 'NONE', *, *, #29786, .F. ) ;
#22522=DIRECTION ( 'NONE',  ( 0.000000000000000000, 0.000000000000000000, 1.000000000000000000 ) ) ;
#22524=AXIS2_PLACEMENT_3D ( 'NONE', #29330, #26697, #6467 ) ;
#22525=ORIENTED_EDGE ( 'NONE', *, *, #196, .F. ) ;
#22526=CARTESIAN_POINT ( 'NONE',  ( 83.49774710563261237, -24.66044155380011915, 12.50000000000000000 ) ) ;
#22527=CIRCLE ( 'NONE', #32084, 2.000000000000001776 ) ;
#22530=CARTESIAN_POINT ( 'NONE',  ( -47.00000337463111322, 77.94228634059959404, -9.999999999999998224 ) ) ;
#22531=ORIENTED_EDGE ( 'NONE', *, *, #29345, .F. ) ;
#22532=ORIENTED_EDGE ( 'NONE', *, *, #246, .T. ) ;
#22533=CIRCLE ( 'NONE', #6354, 2.000000000000001776 ) ;
#22534=AXIS2_PLACEMENT_3D ( 'NONE', #35584, #9523, #15697 ) ;
#22535=VECTOR ( 'NONE', #944, 1000.000000000000000 ) ;
#22536=CIRCLE ( 'NONE', #13534, 2.000000000000001776 ) ;
#22537=CARTESIAN_POINT ( 'NONE',  ( 0.000000000000000000, 0.000000000000000000, 12.49999999999999822 ) ) ;
#22538=AXIS2_PLACEMENT_3D ( 'NONE', #2418, #25118, #10850 ) ;
#22539=ORIENTED_EDGE ( 'NONE', *, *, #25740, .F. ) ;
#22540=DIRECTION ( 'NONE',  ( 0.4999999999999919509, -0.8660254037844433705, 0.000000000000000000 ) ) ;
#22541=ORIENTED_EDGE ( 'NONE', *, *, #27985, .F. ) ;
#22544=CARTESIAN_POINT ( 'NONE',  ( 42.99999662536850309, -60.62177826491080168, -9.999999999999998224 ) ) ;
#22545=CARTESIAN_POINT ( 'NONE',  ( -32.49999999999947420, 56.29165124598880965, 12.49999999999999822 ) ) ;
#22546=EDGE_CURVE ( 'NONE', #16338, #30229, #29182, .T. ) ;
#22547=ORIENTED_EDGE ( 'NONE', *, *, #34354, .T. ) ;
#22550=CARTESIAN_POINT ( 'NONE',  ( -75.00000337463097821, 25.98076211353318854, -9.999999999999998224 ) ) ;
#22551=CIRCLE ( 'NONE', #11171, 2.000000000000001776 ) ;
#22553=CARTESIAN_POINT ( 'NONE',  ( 74.99999662536836809, 8.660254037844394404, -9.999999999999998224 ) ) ;
#22554=CIRCLE ( 'NONE', #10595, 2.000000000000001776 ) ;
#22555=VERTEX_POINT ( 'NONE', #11205 ) ;
#22557=FACE_BOUND ( 'NONE', #25991, .T. ) ;
#22560=VECTOR ( 'NONE', #5868, 1000.000000000000000 ) ;
#22562=DIRECTION ( 'NONE',  ( 0.000000000000000000, 0.000000000000000000, 1.000000000000000000 ) ) ;
#22563=VECTOR ( 'NONE', #27415, 1000.000000000000000 ) ;
#22565=CARTESIAN_POINT ( 'NONE',  ( 47.99999662536846756, -69.28203230275519786, -5.000000000000000000 ) ) ;
#22566=CARTESIAN_POINT ( 'NONE',  ( 44.99999662536849598, 60.62177826491077326, -9.999999999999998224 ) ) ;
#22567=ORIENTED_EDGE ( 'NONE', *, *, #26726, .F. ) ;
#22569=CYLINDRICAL_SURFACE ( 'NONE', #6358, 2.000000000000001776 ) ;
#22570=DIRECTION ( 'NONE',  ( 0.000000000000000000, 0.000000000000000000, 1.000000000000000000 ) ) ;
#22571=EDGE_CURVE ( 'NONE', #5770, #23807, #13658, .T. ) ;
#22572=EDGE_CURVE ( 'NONE', #11869, #7527, #21402, .T. ) ;
#22573=ORIENTED_EDGE ( 'NONE', *, *, #5589, .T. ) ;
#22574=AXIS2_PLACEMENT_3D ( 'NONE', #2489, #28526, #7923 ) ;
#22577=DIRECTION ( 'NONE',  ( 0.000000000000000000, 0.000000000000000000, 1.000000000000000000 ) ) ;
#22578=CARTESIAN_POINT ( 'NONE',  ( -77.00000337463099243, -25.98076211353322051, 12.50000000000000000 ) ) ;
#22579=ORIENTED_EDGE ( 'NONE', *, *, #3928, .F. ) ;
#22581=CIRCLE ( 'NONE', #21375, 2.000000000000001776 ) ;
#22582=DIRECTION ( 'NONE',  ( 0.000000000000000000, 0.000000000000000000, 1.000000000000000000 ) ) ;
#22585=ORIENTED_EDGE ( 'NONE', *, *, #27420, .T. ) ;
#22588=CARTESIAN_POINT ( 'NONE',  ( 4.279621169095998212, -62.97617850287780072, -4.999999999999997335 ) ) ;
#22590=ORIENTED_EDGE ( 'NONE', *, *, #24538, .T. ) ;
#22592=VECTOR ( 'NONE', #15089, 1000.000000000000000 ) ;
#22593=FACE_OUTER_BOUND ( 'NONE', #35421, .T. ) ;
#22594=DIRECTION ( 'NONE',  ( 1.000000000000000000, 0.000000000000000000, 0.000000000000000000 ) ) ;
#22595=ADVANCED_FACE ( 'NONE', ( #33904 ), #28266, .F. ) ;
#22596=EDGE_LOOP ( 'NONE', ( #16946, #32665, #32413, #31975 ) ) ;
#22597=CARTESIAN_POINT ( 'NONE',  ( 14.99999662536859901, 77.94228634059957983, 17.49999999999999645 ) ) ;
#22600=VECTOR ( 'NONE', #9947, 1000.000000000000000 ) ;
#22601=FACE_OUTER_BOUND ( 'NONE', #30530, .T. ) ;
#22603=ORIENTED_EDGE ( 'NONE', *, *, #22910, .T. ) ;
#22604=CARTESIAN_POINT ( 'NONE',  ( -70.47608876694631874, -59.13646009116124702, 12.49999999999999822 ) ) ;
#22605=CIRCLE ( 'NONE', #10646, 2.000000000000000000 ) ;
#22606=DIRECTION ( 'NONE',  ( -0.000000000000000000, -0.000000000000000000, -1.000000000000000000 ) ) ;
#22607=ORIENTED_EDGE ( 'NONE', *, *, #31767, .F. ) ;
#22610=CARTESIAN_POINT ( 'NONE',  ( 0.000000000000000000, 0.000000000000000000, -5.000000000000000000 ) ) ;
#22611=FACE_OUTER_BOUND ( 'NONE', #8476, .T. ) ;
#22613=AXIS2_PLACEMENT_3D ( 'NONE', #9405, #1855, #20840 ) ;
#22614=ORIENTED_EDGE ( 'NONE', *, *, #11684, .T. ) ;
#22616=EDGE_CURVE ( 'NONE', #210, #1373, #36988, .T. ) ;
#22617=VERTEX_POINT ( 'NONE', #5418 ) ;
#22619=DIRECTION ( 'NONE',  ( -1.000000000000000000, 0.000000000000000000, 0.000000000000000000 ) ) ;
#22620=ADVANCED_FACE ( 'NONE', ( #36715 ), #34277, .F. ) ;
#22621=AXIS2_PLACEMENT_3D ( 'NONE', #324, #14411, #34675 ) ;
#22622=AXIS2_PLACEMENT_3D ( 'NONE', #11512, #8528, #31573 ) ;
#22623=ORIENTED_EDGE ( 'NONE', *, *, #36124, .T. ) ;
#22627=LINE ( 'NONE', #31064, #29202 ) ;
#22629=ADVANCED_FACE ( 'NONE', ( #22281 ), #34106, .F. ) ;
#22631=AXIS2_PLACEMENT_3D ( 'NONE', #32505, #1021, #27246 ) ;
#22633=ORIENTED_EDGE ( 'NONE', *, *, #18978, .F. ) ;
#22635=ADVANCED_FACE ( 'NONE', ( #28639 ), #2220, .F. ) ;
#22636=CIRCLE ( 'NONE', #13663, 2.000000000000001776 ) ;
#22637=DIRECTION ( 'NONE',  ( 0.000000000000000000, 0.000000000000000000, 1.000000000000000000 ) ) ;
#22639=DIRECTION ( 'NONE',  ( 0.000000000000000000, 0.000000000000000000, 1.000000000000000000 ) ) ;
#22640=ORIENTED_EDGE ( 'NONE', *, *, #1632, .T. ) ;
#22642=CIRCLE ( 'NONE', #1112, 2.000000000000001776 ) ;
#22643=FACE_BOUND ( 'NONE', #1580, .T. ) ;
#22644=VECTOR ( 'NONE', #4824, 1000.000000000000000 ) ;
#22645=AXIS2_PLACEMENT_3D ( 'NONE', #7910, #15787, #24425 ) ;
#22646=DIRECTION ( 'NONE',  ( 0.000000000000000000, 0.000000000000000000, 1.000000000000000000 ) ) ;
#22647=ORIENTED_EDGE ( 'NONE', *, *, #21090, .T. ) ;
#22649=DIRECTION ( 'NONE',  ( -0.000000000000000000, -0.000000000000000000, 1.000000000000000000 ) ) ;
#22650=CIRCLE ( 'NONE', #8285, 3.000000000000002665 ) ;
#22652=DIRECTION ( 'NONE',  ( 1.000000000000000000, 0.000000000000000000, 0.000000000000000000 ) ) ;
#22653=CYLINDRICAL_SURFACE ( 'NONE', #35283, 2.000000000000001776 ) ;
#22654=ORIENTED_EDGE ( 'NONE', *, *, #33520, .T. ) ;
#22655=CARTESIAN_POINT ( 'NONE',  ( 39.99999662536853151, 69.28203230275518365, -9.999999999999998224 ) ) ;
#22656=DIRECTION ( 'NONE',  ( -1.000000000000000000, 0.000000000000000000, 0.000000000000000000 ) ) ;
#22657=AXIS2_PLACEMENT_3D ( 'NONE', #8578, #20012, #31441 ) ;
#22659=EDGE_CURVE ( 'NONE', #13352, #7812, #35233, .T. ) ;
#22660=ORIENTED_EDGE ( 'NONE', *, *, #4630, .T. ) ;
#22661=ORIENTED_EDGE ( 'NONE', *, *, #36011, .F. ) ;
#22663=EDGE_CURVE ( 'NONE', #17059, #16108, #30888, .T. ) ;
#22664=EDGE_LOOP ( 'NONE', ( #17440, #3832 ) ) ;
#22665=AXIS2_PLACEMENT_3D ( 'NONE', #17437, #23254, #3021 ) ;
#22666=DIRECTION ( 'NONE',  ( 0.000000000000000000, 0.000000000000000000, 1.000000000000000000 ) ) ;
#22667=CARTESIAN_POINT ( 'NONE',  ( -52.39915983220772233, -35.19434990244957362, -4.999999999999997335 ) ) ;
#22668=CIRCLE ( 'NONE', #10089, 2.000000000000001776 ) ;
#22669=DIRECTION ( 'NONE',  ( 0.000000000000000000, 0.000000000000000000, -1.000000000000000000 ) ) ;
#22670=AXIS2_PLACEMENT_3D ( 'NONE', #13125, #1483, #7488 ) ;
#22674=DIRECTION ( 'NONE',  ( -0.000000000000000000, -0.000000000000000000, 1.000000000000000000 ) ) ;
#22676=CIRCLE ( 'NONE', #28050, 2.000000000000001776 ) ;
#22677=VERTEX_POINT ( 'NONE', #30708 ) ;
#22679=AXIS2_PLACEMENT_3D ( 'NONE', #27241, #19371, #35703 ) ;
#22681=ADVANCED_FACE ( 'NONE', ( #19840 ), #11012, .F. ) ;
#22682=DIRECTION ( 'NONE',  ( 0.000000000000000000, 0.000000000000000000, 1.000000000000000000 ) ) ;
#22683=CARTESIAN_POINT ( 'NONE',  ( 84.99999662536832545, 8.660254037844394404, -5.000000000000000000 ) ) ;
#22686=FACE_BOUND ( 'NONE', #9708, .T. ) ;
#22687=CIRCLE ( 'NONE', #25668, 2.000000000000001776 ) ;
#22689=ORIENTED_EDGE ( 'NONE', *, *, #30744, .T. ) ;
#22691=CARTESIAN_POINT ( 'NONE',  ( -70.00000337463099243, 17.32050807568877460, -9.999999999999998224 ) ) ;
#22693=DIRECTION ( 'NONE',  ( -1.000000000000000000, 0.000000000000000000, 0.000000000000000000 ) ) ;
#22694=FACE_OUTER_BOUND ( 'NONE', #835, .T. ) ;
#22695=EDGE_CURVE ( 'NONE', #29460, #23785, #4092, .T. ) ;
#22696=DIRECTION ( 'NONE',  ( 0.000000000000000000, 0.000000000000000000, 1.000000000000000000 ) ) ;
#22697=AXIS2_PLACEMENT_3D ( 'NONE', #26879, #4366, #27224 ) ;
#22699=EDGE_CURVE ( 'NONE', #29605, #16351, #32808, .T. ) ;
#22700=ORIENTED_EDGE ( 'NONE', *, *, #18987, .F. ) ;
#22701=AXIS2_PLACEMENT_3D ( 'NONE', #28118, #25688, #19685 ) ;
#22703=EDGE_CURVE ( 'NONE', #2655, #35919, #37097, .T. ) ;
#22704=ORIENTED_EDGE ( 'NONE', *, *, #1729, .F. ) ;
#22705=VECTOR ( 'NONE', #27333, 1000.000000000000000 ) ;
#22707=DIRECTION ( 'NONE',  ( 1.000000000000000000, 0.000000000000000000, 0.000000000000000000 ) ) ;
#22708=AXIS2_PLACEMENT_3D ( 'NONE', #28785, #25974, #274 ) ;
#22709=DIRECTION ( 'NONE',  ( 1.000000000000000000, 0.000000000000000000, 0.000000000000000000 ) ) ;
#22710=EDGE_CURVE ( 'NONE', #12225, #7729, #6478, .T. ) ;
#22711=DIRECTION ( 'NONE',  ( -1.000000000000000000, 0.000000000000000000, -0.000000000000000000 ) ) ;
#22712=DIRECTION ( 'NONE',  ( 1.000000000000000000, 0.000000000000000000, 0.000000000000000000 ) ) ;
#22713=CYLINDRICAL_SURFACE ( 'NONE', #18950, 3.000000000000002665 ) ;
#22714=EDGE_CURVE ( 'NONE', #29420, #8519, #36435, .T. ) ;
#22715=ORIENTED_EDGE ( 'NONE', *, *, #33888, .F. ) ;
#22716=DIRECTION ( 'NONE',  ( 1.000000000000000000, 0.000000000000000000, 0.000000000000000000 ) ) ;
#22717=DIRECTION ( 'NONE',  ( 0.000000000000000000, 0.000000000000000000, -1.000000000000000000 ) ) ;
#22718=AXIS2_PLACEMENT_3D ( 'NONE', #7664, #36546, #19288 ) ;
#22719=CARTESIAN_POINT ( 'NONE',  ( -60.00000337463104216, 34.64101615137757051, 17.49999999999999645 ) ) ;
#22720=ORIENTED_EDGE ( 'NONE', *, *, #659, .F. ) ;
#22721=CARTESIAN_POINT ( 'NONE',  ( 49.99999662536846756, 51.96152422706637708, -9.999999999999998224 ) ) ;
#22722=AXIS2_PLACEMENT_3D ( 'NONE', #33630, #36797, #7933 ) ;
#22723=DIRECTION ( 'NONE',  ( 1.000000000000000000, 0.000000000000000000, 0.000000000000000000 ) ) ;
#22724=EDGE_CURVE ( 'NONE', #17922, #9816, #18472, .T. ) ;
#22726=EDGE_CURVE ( 'NONE', #16319, #2878, #26388, .T. ) ;
#22727=ORIENTED_EDGE ( 'NONE', *, *, #20369, .T. ) ;
#22728=LINE ( 'NONE', #11279, #29013 ) ;
#22729=EDGE_CURVE ( 'NONE', #32307, #2310, #27427, .T. ) ;
#22730=AXIS2_PLACEMENT_3D ( 'NONE', #29712, #35189, #35388 ) ;
#22731=DIRECTION ( 'NONE',  ( 1.000000000000000000, 0.000000000000000000, 0.000000000000000000 ) ) ;
#22734=DIRECTION ( 'NONE',  ( 1.000000000000000000, 0.000000000000000000, 0.000000000000000000 ) ) ;
#22741=CIRCLE ( 'NONE', #6560, 2.000000000000001776 ) ;
#22742=ORIENTED_EDGE ( 'NONE', *, *, #5654, .F. ) ;
#22743=DIRECTION ( 'NONE',  ( 0.000000000000000000, 0.000000000000000000, -1.000000000000000000 ) ) ;
#22744=ORIENTED_EDGE ( 'NONE', *, *, #12289, .T. ) ;
#22745=EDGE_LOOP ( 'NONE', ( #18157, #2178, #27116, #29846 ) ) ;
#22746=CARTESIAN_POINT ( 'NONE',  ( 32.49999999999987210, -56.29165124598858938, 12.49999999999999822 ) ) ;
#22747=LINE ( 'NONE', #16917, #4075 ) ;
#22749=AXIS2_PLACEMENT_3D ( 'NONE', #1063, #29376, #9862 ) ;
#22750=DIRECTION ( 'NONE',  ( 0.000000000000000000, 0.000000000000000000, 1.000000000000000000 ) ) ;
#22753=CARTESIAN_POINT ( 'NONE',  ( -72.00000337463102085, -51.96152422706641971, -9.999999999999998224 ) ) ;
#22754=AXIS2_PLACEMENT_3D ( 'NONE', #6689, #35402, #6863 ) ;
#22755=CARTESIAN_POINT ( 'NONE',  ( -33.00000337463116296, 77.94228634059957983, -9.999999999999998224 ) ) ;
#22756=DIRECTION ( 'NONE',  ( -0.000000000000000000, -0.000000000000000000, 1.000000000000000000 ) ) ;
#22757=DIRECTION ( 'NONE',  ( 1.000000000000000000, 0.000000000000000000, 0.000000000000000000 ) ) ;
#22758=ORIENTED_EDGE ( 'NONE', *, *, #10884, .F. ) ;
#22759=DIRECTION ( 'NONE',  ( 1.000000000000000000, 0.000000000000000000, 0.000000000000000000 ) ) ;
#22760=FACE_BOUND ( 'NONE', #1986, .T. ) ;
#22761=EDGE_CURVE ( 'NONE', #22972, #13489, #2895, .T. ) ;
#22762=DIRECTION ( 'NONE',  ( 0.000000000000000000, 0.000000000000000000, 1.000000000000000000 ) ) ;
#22763=CARTESIAN_POINT ( 'NONE',  ( 2.999999999999768630, -68.00000000000000000, 12.49999999999999822 ) ) ;
#22765=VECTOR ( 'NONE', #24285, 1000.000000000000000 ) ;
#22766=DIRECTION ( 'NONE',  ( -1.000000000000000000, 0.000000000000000000, -0.000000000000000000 ) ) ;
#22767=DIRECTION ( 'NONE',  ( 1.000000000000000000, 0.000000000000000000, 0.000000000000000000 ) ) ;
#22769=DIRECTION ( 'NONE',  ( 0.000000000000000000, 0.000000000000000000, -1.000000000000000000 ) ) ;
#22770=ORIENTED_EDGE ( 'NONE', *, *, #33830, .T. ) ;
#22771=DIRECTION ( 'NONE',  ( -1.000000000000000000, 0.000000000000000000, 0.000000000000000000 ) ) ;
#22774=DIRECTION ( 'NONE',  ( -1.000000000000000000, 0.000000000000000000, 0.000000000000000000 ) ) ;
#22776=EDGE_CURVE ( 'NONE', #28212, #19903, #26221, .T. ) ;
#22777=ORIENTED_EDGE ( 'NONE', *, *, #29661, .T. ) ;
#22778=ORIENTED_EDGE ( 'NONE', *, *, #29566, .T. ) ;
#22779=EDGE_CURVE ( 'NONE', #17325, #12004, #32201, .T. ) ;
#22780=EDGE_CURVE ( 'NONE', #27172, #34636, #4692, .T. ) ;
#22781=DIRECTION ( 'NONE',  ( 0.000000000000000000, 0.000000000000000000, 1.000000000000000000 ) ) ;
#22782=DIRECTION ( 'NONE',  ( 1.000000000000000000, 0.000000000000000000, 0.000000000000000000 ) ) ;
#22783=DIRECTION ( 'NONE',  ( -1.000000000000000000, 0.000000000000000000, 0.000000000000000000 ) ) ;
#22784=AXIS2_PLACEMENT_3D ( 'NONE', #24687, #27666, #13240 ) ;
#22785=ORIENTED_EDGE ( 'NONE', *, *, #12113, .F. ) ;
#22786=DIRECTION ( 'NONE',  ( 0.000000000000000000, -0.000000000000000000, -1.000000000000000000 ) ) ;
#22788=AXIS2_PLACEMENT_3D ( 'NONE', #36819, #20312, #6064 ) ;
#22789=CYLINDRICAL_SURFACE ( 'NONE', #13761, 2.000000000000001776 ) ;
#22790=ORIENTED_EDGE ( 'NONE', *, *, #9389, .T. ) ;
#22791=DIRECTION ( 'NONE',  ( -1.000000000000000000, 0.000000000000000000, 0.000000000000000000 ) ) ;
#22792=VERTEX_POINT ( 'NONE', #12101 ) ;
#22794=LINE ( 'NONE', #27833, #24392 ) ;
#22795=CYLINDRICAL_SURFACE ( 'NONE', #13625, 2.000000000000001776 ) ;
#22796=AXIS2_PLACEMENT_3D ( 'NONE', #30952, #14066, #25520 ) ;
#22798=DIRECTION ( 'NONE',  ( 0.000000000000000000, 0.000000000000000000, -1.000000000000000000 ) ) ;
#22801=ADVANCED_FACE ( 'NONE', ( #34458 ), #309, .F. ) ;
#22802=LINE ( 'NONE', #32124, #6682 ) ;
#22804=ORIENTED_EDGE ( 'NONE', *, *, #18685, .F. ) ;
#22805=CARTESIAN_POINT ( 'NONE',  ( 44.99999662536849598, -77.94228634059960825, -9.999999999999998224 ) ) ;
#22806=LINE ( 'NONE', #20345, #27561 ) ;
#22807=ORIENTED_EDGE ( 'NONE', *, *, #37042, .T. ) ;
#22809=DIRECTION ( 'NONE',  ( 0.000000000000000000, 0.000000000000000000, 1.000000000000000000 ) ) ;
#22810=CARTESIAN_POINT ( 'NONE',  ( -20.00000337463122690, 86.60254037844397601, -5.000000000000000000 ) ) ;
#22813=ORIENTED_EDGE ( 'NONE', *, *, #15550, .T. ) ;
#22814=LINE ( 'NONE', #22248, #32122 ) ;
#22815=DIRECTION ( 'NONE',  ( 1.000000000000000000, 0.000000000000000000, 0.000000000000000000 ) ) ;
#22816=EDGE_LOOP ( 'NONE', ( #22539, #2376, #35466, #21776, #29214 ) ) ;
#22817=VERTEX_POINT ( 'NONE', #15124 ) ;
#22818=AXIS2_PLACEMENT_3D ( 'NONE', #20020, #34668, #14964 ) ;
#22820=DIRECTION ( 'NONE',  ( 1.000000000000000000, 0.000000000000000000, 0.000000000000000000 ) ) ;
#22823=ORIENTED_EDGE ( 'NONE', *, *, #33084, .F. ) ;
#22824=EDGE_LOOP ( 'NONE', ( #3967, #27418 ) ) ;
#22826=DIRECTION ( 'NONE',  ( 1.000000000000000000, 0.000000000000000000, 0.000000000000000000 ) ) ;
#22827=VERTEX_POINT ( 'NONE', #14567 ) ;
#22828=CARTESIAN_POINT ( 'NONE',  ( -43.00000337463112743, -60.62177826491080168, -5.000000000000000000 ) ) ;
#22829=EDGE_LOOP ( 'NONE', ( #17264, #15902 ) ) ;
#22830=CARTESIAN_POINT ( 'NONE',  ( -42.00000337463114164, -69.28203230275519786, -9.999999999999998224 ) ) ;
#22831=DIRECTION ( 'NONE',  ( 0.000000000000000000, 0.000000000000000000, 1.000000000000000000 ) ) ;
#22832=DIRECTION ( 'NONE',  ( 0.000000000000000000, -0.000000000000000000, -1.000000000000000000 ) ) ;
#22833=VERTEX_POINT ( 'NONE', #29379 ) ;
#22834=EDGE_CURVE ( 'NONE', #7482, #36258, #33433, .T. ) ;
#22836=DIRECTION ( 'NONE',  ( 0.000000000000000000, 0.000000000000000000, 1.000000000000000000 ) ) ;
#22837=CYLINDRICAL_SURFACE ( 'NONE', #34133, 2.000000000000001776 ) ;
#22839=ORIENTED_EDGE ( 'NONE', *, *, #35156, .T. ) ;
#22840=DIRECTION ( 'NONE',  ( 1.000000000000000000, 0.000000000000000000, 0.000000000000000000 ) ) ;
#22841=CARTESIAN_POINT ( 'NONE',  ( -65.00000337463102085, 60.62177826491077326, -5.000000000000000000 ) ) ;
#22842=CARTESIAN_POINT ( 'NONE',  ( 64.99999662536842493, 43.30127018922200222, -9.999999999999998224 ) ) ;
#22843=EDGE_LOOP ( 'NONE', ( #35669, #20539 ) ) ;
#22844=EDGE_CURVE ( 'NONE', #30934, #26515, #2300, .T. ) ;
#22845=EDGE_LOOP ( 'NONE', ( #12322, #31920, #11497, #12049 ) ) ;
#22847=VERTEX_POINT ( 'NONE', #14957 ) ;
#22848=DIRECTION ( 'NONE',  ( 4.625929269271481378E-15, 1.000000000000000000, 0.000000000000000000 ) ) ;
#22849=VECTOR ( 'NONE', #34603, 1000.000000000000000 ) ;
#22850=CARTESIAN_POINT ( 'NONE',  ( 90.60231327712337190, 15.97563234535636134, 12.49999999999999822 ) ) ;
#22853=DIRECTION ( 'NONE',  ( -1.000000000000000000, 0.000000000000000000, 0.000000000000000000 ) ) ;
#22854=CIRCLE ( 'NONE', #15660, 2.000000000000001776 ) ;
#22856=DIRECTION ( 'NONE',  ( -1.047444401652940795E-14, -1.000000000000000000, 0.000000000000000000 ) ) ;
#22857=ORIENTED_EDGE ( 'NONE', *, *, #3610, .F. ) ;
#22860=CARTESIAN_POINT ( 'NONE',  ( -73.00000337463100664, -43.30127018922202353, 12.50000000000000000 ) ) ;
#22863=ORIENTED_EDGE ( 'NONE', *, *, #29247, .F. ) ;
#22865=FACE_BOUND ( 'NONE', #21884, .T. ) ;
#22866=ORIENTED_EDGE ( 'NONE', *, *, #7480, .F. ) ;
#22868=EDGE_CURVE ( 'NONE', #33, #34040, #18443, .T. ) ;
#22869=DIRECTION ( 'NONE',  ( 0.000000000000000000, 0.000000000000000000, 1.000000000000000000 ) ) ;
#22870=ORIENTED_EDGE ( 'NONE', *, *, #23921, .F. ) ;
#22871=DIRECTION ( 'NONE',  ( 0.000000000000000000, 0.000000000000000000, -1.000000000000000000 ) ) ;
#22872=EDGE_CURVE ( 'NONE', #16595, #14001, #16063, .T. ) ;
#22873=CYLINDRICAL_SURFACE ( 'NONE', #12836, 2.000000000000001776 ) ;
#22874=AXIS2_PLACEMENT_3D ( 'NONE', #30200, #4533, #18973 ) ;
#22875=CARTESIAN_POINT ( 'NONE',  ( -53.00000337463106348, 60.62177826491078747, 12.50000000000000000 ) ) ;
#22876=ORIENTED_EDGE ( 'NONE', *, *, #16935, .F. ) ;
#22879=EDGE_LOOP ( 'NONE', ( #36994, #25981 ) ) ;
#22881=EDGE_CURVE ( 'NONE', #10971, #6989, #10251, .T. ) ;
#22883=DIRECTION ( 'NONE',  ( 0.000000000000000000, 0.000000000000000000, 1.000000000000000000 ) ) ;
#22884=FACE_OUTER_BOUND ( 'NONE', #15830, .T. ) ;
#22887=CARTESIAN_POINT ( 'NONE',  ( -95.00000000000000000, 0.000000000000000000, 17.49999999999999645 ) ) ;
#22888=ORIENTED_EDGE ( 'NONE', *, *, #16993, .T. ) ;
#22889=CARTESIAN_POINT ( 'NONE',  ( 63.10544158860312081, 59.98094972882071829, -5.000000000000000000 ) ) ;
#22890=CARTESIAN_POINT ( 'NONE',  ( -80.00000337463096400, -34.64101615137762025, 17.49999999999999645 ) ) ;
#22891=DIRECTION ( 'NONE',  ( 1.000000000000000000, 0.000000000000000000, 0.000000000000000000 ) ) ;
#22892=ORIENTED_EDGE ( 'NONE', *, *, #2433, .F. ) ;
#22893=DIRECTION ( 'NONE',  ( 0.000000000000000000, 0.000000000000000000, 1.000000000000000000 ) ) ;
#22894=DIRECTION ( 'NONE',  ( 1.000000000000000000, 0.000000000000000000, 0.000000000000000000 ) ) ;
#22895=ORIENTED_EDGE ( 'NONE', *, *, #29531, .T. ) ;
#22896=ORIENTED_EDGE ( 'NONE', *, *, #7680, .T. ) ;
#22897=ADVANCED_FACE ( 'NONE', ( #4262 ), #10423, .F. ) ;
#22899=AXIS2_PLACEMENT_3D ( 'NONE', #24003, #919, #29796 ) ;
#22901=DIRECTION ( 'NONE',  ( 1.000000000000000000, 0.000000000000000000, 0.000000000000000000 ) ) ;
#22903=EDGE_LOOP ( 'NONE', ( #21244, #1736 ) ) ;
#22904=ORIENTED_EDGE ( 'NONE', *, *, #3325, .T. ) ;
#22905=CARTESIAN_POINT ( 'NONE',  ( 31.99999662536856704, 69.28203230275518365, 17.49999999999999645 ) ) ;
#22906=EDGE_CURVE ( 'NONE', #18966, #13116, #15691, .T. ) ;
#22909=ORIENTED_EDGE ( 'NONE', *, *, #33529, .F. ) ;
#22910=EDGE_CURVE ( 'NONE', #20554, #111, #13050, .T. ) ;
#22912=CARTESIAN_POINT ( 'NONE',  ( 21.99999662536859191, 69.28203230275516944, -9.999999999999998224 ) ) ;
#22914=ORIENTED_EDGE ( 'NONE', *, *, #639, .F. ) ;
#22915=AXIS2_PLACEMENT_3D ( 'NONE', #30216, #35871, #18797 ) ;
#22916=DIRECTION ( 'NONE',  ( 1.000000000000000000, 0.000000000000000000, 0.000000000000000000 ) ) ;
#22917=DIRECTION ( 'NONE',  ( 0.000000000000000000, 0.000000000000000000, -1.000000000000000000 ) ) ;
#22918=ORIENTED_EDGE ( 'NONE', *, *, #16304, .F. ) ;
#22919=VERTEX_POINT ( 'NONE', #30110 ) ;
#22920=CARTESIAN_POINT ( 'NONE',  ( 67.99999662536838230, -17.32050807568879947, -9.999999999999998224 ) ) ;
#22921=DIRECTION ( 'NONE',  ( 0.000000000000000000, 0.000000000000000000, 1.000000000000000000 ) ) ;
#22922=CARTESIAN_POINT ( 'NONE',  ( -70.00000337463099243, 51.96152422706637708, 12.50000000000000000 ) ) ;
#22924=EDGE_LOOP ( 'NONE', ( #14381, #31611, #26718 ) ) ;
#22925=FACE_OUTER_BOUND ( 'NONE', #2867, .T. ) ;
#22926=AXIS2_PLACEMENT_3D ( 'NONE', #25468, #34798, #3484 ) ;
#22927=FACE_BOUND ( 'NONE', #12192, .T. ) ;
#22928=AXIS2_PLACEMENT_3D ( 'NONE', #21827, #36468, #19387 ) ;
#22930=DIRECTION ( 'NONE',  ( -0.4999999999999979461, 0.8660254037844397068, 0.000000000000000000 ) ) ;
#22931=LINE ( 'NONE', #22372, #4547 ) ;
#22932=DIRECTION ( 'NONE',  ( 1.000000000000000000, 0.000000000000000000, 0.000000000000000000 ) ) ;
#22933=DIRECTION ( 'NONE',  ( 1.000000000000000000, 0.000000000000000000, 0.000000000000000000 ) ) ;
#22934=DIRECTION ( 'NONE',  ( 1.000000000000000000, 0.000000000000000000, 0.000000000000000000 ) ) ;
#22935=ORIENTED_EDGE ( 'NONE', *, *, #12852, .T. ) ;
#22936=FACE_OUTER_BOUND ( 'NONE', #14803, .T. ) ;
#22937=DIRECTION ( 'NONE',  ( 1.000000000000000000, 0.000000000000000000, -0.000000000000000000 ) ) ;
#22938=CARTESIAN_POINT ( 'NONE',  ( 9.999996625368655856, -69.28203230275519786, -9.999999999999998224 ) ) ;
#22939=ORIENTED_EDGE ( 'NONE', *, *, #33724, .T. ) ;
#22941=ORIENTED_EDGE ( 'NONE', *, *, #33520, .F. ) ;
#22942=EDGE_CURVE ( 'NONE', #12253, #14986, #23845, .T. ) ;
#22943=ORIENTED_EDGE ( 'NONE', *, *, #7349, .T. ) ;
#22944=DIRECTION ( 'NONE',  ( 0.000000000000000000, 0.000000000000000000, -1.000000000000000000 ) ) ;
#22945=DIRECTION ( 'NONE',  ( 1.000000000000000000, 0.000000000000000000, 0.000000000000000000 ) ) ;
#22946=ADVANCED_FACE ( 'NONE', ( #21681 ), #27499, .T. ) ;
#22948=ORIENTED_EDGE ( 'NONE', *, *, #89, .T. ) ;
#22951=AXIS2_PLACEMENT_3D ( 'NONE', #14916, #30899, #5236 ) ;
#22952=ORIENTED_EDGE ( 'NONE', *, *, #7390, .T. ) ;
#22953=DIRECTION ( 'NONE',  ( 0.000000000000000000, 0.000000000000000000, 1.000000000000000000 ) ) ;
#22954=VERTEX_POINT ( 'NONE', #18874 ) ;
#22955=ADVANCED_FACE ( 'NONE', ( #16256 ), #1067, .F. ) ;
#22956=DIRECTION ( 'NONE',  ( 0.000000000000000000, 0.000000000000000000, 1.000000000000000000 ) ) ;
#22957=ORIENTED_EDGE ( 'NONE', *, *, #16218, .F. ) ;
#22958=EDGE_CURVE ( 'NONE', #34330, #6458, #16675, .T. ) ;
#22959=ORIENTED_EDGE ( 'NONE', *, *, #35614, .T. ) ;
#22960=CARTESIAN_POINT ( 'NONE',  ( -38.00000337463113453, -69.28203230275519786, -9.999999999999998224 ) ) ;
#22961=FACE_OUTER_BOUND ( 'NONE', #4271, .T. ) ;
#22962=ORIENTED_EDGE ( 'NONE', *, *, #21758, .T. ) ;
#22968=EDGE_CURVE ( 'NONE', #32425, #25770, #4718, .T. ) ;
#22969=CARTESIAN_POINT ( 'NONE',  ( -68.00000337463099243, -2.428612866367529932E-14, -9.999999999999998224 ) ) ;
#22971=EDGE_CURVE ( 'NONE', #17289, #2363, #13075, .T. ) ;
#22972=VERTEX_POINT ( 'NONE', #5729 ) ;
#22974=FACE_OUTER_BOUND ( 'NONE', #12172, .T. ) ;
#22975=EDGE_CURVE ( 'NONE', #167, #21629, #34053, .T. ) ;
#22976=ORIENTED_EDGE ( 'NONE', *, *, #1514, .F. ) ;
#22977=DIRECTION ( 'NONE',  ( 0.5000000000000038858, 0.8660254037844362651, 0.000000000000000000 ) ) ;
#22978=CARTESIAN_POINT ( 'NONE',  ( -58.00000337463104216, 34.64101615137757051, -9.999999999999998224 ) ) ;
#22980=DIRECTION ( 'NONE',  ( 0.000000000000000000, 0.000000000000000000, 1.000000000000000000 ) ) ;
#22982=AXIS2_PLACEMENT_3D ( 'NONE', #6615, #3976, #30031 ) ;
#22983=VERTEX_POINT ( 'NONE', #8373 ) ;
#22984=PLANE ( 'NONE',  #7603 ) ;
#22985=DIRECTION ( 'NONE',  ( 0.000000000000000000, 0.000000000000000000, 1.000000000000000000 ) ) ;
#22986=AXIS2_PLACEMENT_3D ( 'NONE', #7227, #1394, #14921 ) ;
#22987=VERTEX_POINT ( 'NONE', #22068 ) ;
#22988=ORIENTED_EDGE ( 'NONE', *, *, #33329, .T. ) ;
#22989=VERTEX_POINT ( 'NONE', #19254 ) ;
#22991=DIRECTION ( 'NONE',  ( 0.000000000000000000, 0.000000000000000000, 1.000000000000000000 ) ) ;
#22994=AXIS2_PLACEMENT_3D ( 'NONE', #31063, #34078, #19437 ) ;
#22995=CARTESIAN_POINT ( 'NONE',  ( -55.00000337463107059, 43.30127018922197379, -9.999999999999998224 ) ) ;
#22996=ORIENTED_EDGE ( 'NONE', *, *, #5235, .F. ) ;
#22997=CYLINDRICAL_SURFACE ( 'NONE', #25126, 2.000000000000001776 ) ;
#22999=FACE_OUTER_BOUND ( 'NONE', #16704, .T. ) ;
#23000=AXIS2_PLACEMENT_3D ( 'NONE', #3958, #32061, #6398 ) ;
#23001=CARTESIAN_POINT ( 'NONE',  ( 6.999996625368676284, -77.94228634059960825, 12.50000000000000000 ) ) ;
#23005=DIRECTION ( 'NONE',  ( 1.000000000000000000, 0.000000000000000000, 0.000000000000000000 ) ) ;
#23006=DIRECTION ( 'NONE',  ( 0.000000000000000000, 0.000000000000000000, 1.000000000000000000 ) ) ;
#23009=VERTEX_POINT ( 'NONE', #2725 ) ;
#23010=DIRECTION ( 'NONE',  ( 0.000000000000000000, 0.000000000000000000, -1.000000000000000000 ) ) ;
#23011=CARTESIAN_POINT ( 'NONE',  ( -35.00000337463116296, 77.94228634059957983, 12.50000000000000000 ) ) ;
#23012=CARTESIAN_POINT ( 'NONE',  ( -50.00000337463109190, 51.96152422706637708, -5.000000000000000000 ) ) ;
#23013=ORIENTED_EDGE ( 'NONE', *, *, #19551, .T. ) ;
#23014=CIRCLE ( 'NONE', #8055, 2.000000000000001776 ) ;
#23016=VERTEX_POINT ( 'NONE', #27670 ) ;
#23017=VECTOR ( 'NONE', #17982, 1000.000000000000000 ) ;
#23018=CARTESIAN_POINT ( 'NONE',  ( 9.999996625368618552, 69.28203230275516944, 17.49999999999999645 ) ) ;
#23019=CIRCLE ( 'NONE', #6853, 2.000000000000001776 ) ;
#23020=DIRECTION ( 'NONE',  ( 0.000000000000000000, 0.000000000000000000, 1.000000000000000000 ) ) ;
#23021=DIRECTION ( 'NONE',  ( 0.000000000000000000, 0.000000000000000000, 1.000000000000000000 ) ) ;
#23022=DIRECTION ( 'NONE',  ( 0.000000000000000000, 0.000000000000000000, 1.000000000000000000 ) ) ;
#23023=CARTESIAN_POINT ( 'NONE',  ( -27.78182860042817026, -56.67878100130359087, 12.49999999999999822 ) ) ;
#23024=EDGE_CURVE ( 'NONE', #27066, #17904, #27455, .T. ) ;
#23025=DIRECTION ( 'NONE',  ( 0.000000000000000000, 0.000000000000000000, -1.000000000000000000 ) ) ;
#23026=ADVANCED_FACE ( 'NONE', ( #5546 ), #36311, .F. ) ;
#23027=VERTEX_POINT ( 'NONE', #19616 ) ;
#23028=EDGE_LOOP ( 'NONE', ( #24555, #31763, #21489, #11190 ) ) ;
#23029=CARTESIAN_POINT ( 'NONE',  ( -75.00000337463097821, -8.660254037844422825, -9.999999999999998224 ) ) ;
#23030=AXIS2_PLACEMENT_3D ( 'NONE', #34510, #8817, #364 ) ;
#23031=DIRECTION ( 'NONE',  ( 0.000000000000000000, 0.000000000000000000, 1.000000000000000000 ) ) ;
#23032=CIRCLE ( 'NONE', #13441, 2.000000000000001776 ) ;
#23034=ORIENTED_EDGE ( 'NONE', *, *, #14907, .F. ) ;
#23035=EDGE_CURVE ( 'NONE', #8981, #8132, #21463, .T. ) ;
#23036=FACE_BOUND ( 'NONE', #20343, .T. ) ;
#23037=EDGE_LOOP ( 'NONE', ( #2082, #23048 ) ) ;
#23038=ORIENTED_EDGE ( 'NONE', *, *, #18865, .F. ) ;
#23039=DIRECTION ( 'NONE',  ( 0.000000000000000000, 0.000000000000000000, 1.000000000000000000 ) ) ;
#23043=AXIS2_PLACEMENT_3D ( 'NONE', #33239, #30233, #7560 ) ;
#23044=AXIS2_PLACEMENT_3D ( 'NONE', #20180, #16992, #287 ) ;
#23046=CARTESIAN_POINT ( 'NONE',  ( -68.00000337463102085, -51.96152422706641971, -9.999999999999998224 ) ) ;
#23047=EDGE_CURVE ( 'NONE', #16018, #6451, #7706, .T. ) ;
#23048=ORIENTED_EDGE ( 'NONE', *, *, #9994, .T. ) ;
#23049=ORIENTED_EDGE ( 'NONE', *, *, #14653, .T. ) ;
#23052=ORIENTED_EDGE ( 'NONE', *, *, #14400, .F. ) ;
#23053=VECTOR ( 'NONE', #20997, 1000.000000000000000 ) ;
#23054=DIRECTION ( 'NONE',  ( 0.000000000000000000, 0.000000000000000000, 1.000000000000000000 ) ) ;
#23055=AXIS2_PLACEMENT_3D ( 'NONE', #29694, #1218, #26158 ) ;
#23056=DIRECTION ( 'NONE',  ( 1.000000000000000000, 0.000000000000000000, 0.000000000000000000 ) ) ;
#23058=DIRECTION ( 'NONE',  ( -0.000000000000000000, -0.000000000000000000, 1.000000000000000000 ) ) ;
#23059=ORIENTED_EDGE ( 'NONE', *, *, #1825, .T. ) ;
#23060=AXIS2_PLACEMENT_3D ( 'NONE', #28249, #21883, #17379 ) ;
#23061=DIRECTION ( 'NONE',  ( 0.000000000000000000, 0.000000000000000000, 1.000000000000000000 ) ) ;
#23062=CIRCLE ( 'NONE', #11071, 2.000000000000001776 ) ;
#23063=DIRECTION ( 'NONE',  ( -0.000000000000000000, -0.000000000000000000, -1.000000000000000000 ) ) ;
#23064=ADVANCED_FACE ( 'NONE', ( #7820 ), #37054, .F. ) ;
#23065=DIRECTION ( 'NONE',  ( 0.000000000000000000, 0.000000000000000000, 1.000000000000000000 ) ) ;
#23066=VERTEX_POINT ( 'NONE', #4987 ) ;
#23067=LINE ( 'NONE', #2285, #35236 ) ;
#23069=CIRCLE ( 'NONE', #9902, 2.000000000000001776 ) ;
#23070=ORIENTED_EDGE ( 'NONE', *, *, #35469, .F. ) ;
#23072=FACE_OUTER_BOUND ( 'NONE', #20156, .T. ) ;
#23074=DIRECTION ( 'NONE',  ( 1.000000000000000000, 0.000000000000000000, 0.000000000000000000 ) ) ;
#23078=ORIENTED_EDGE ( 'NONE', *, *, #6512, .T. ) ;
#23079=CARTESIAN_POINT ( 'NONE',  ( -33.00000337463116296, 77.94228634059957983, -9.999999999999998224 ) ) ;
#23081=CARTESIAN_POINT ( 'NONE',  ( 17.99999662536861678, -86.60254037844400443, 17.49999999999999645 ) ) ;
#23082=EDGE_CURVE ( 'NONE', #36051, #5822, #5307, .T. ) ;
#23083=AXIS2_PLACEMENT_3D ( 'NONE', #24121, #10609, #16245 ) ;
#23085=AXIS2_PLACEMENT_3D ( 'NONE', #16934, #31353, #22766 ) ;
#23086=DIRECTION ( 'NONE',  ( 1.000000000000000000, 0.000000000000000000, 0.000000000000000000 ) ) ;
#23088=AXIS2_PLACEMENT_3D ( 'NONE', #31813, #31451, #6144 ) ;
#23089=AXIS2_PLACEMENT_3D ( 'NONE', #23684, #3799, #24440 ) ;
#23090=CIRCLE ( 'NONE', #32057, 2.000000000000001776 ) ;
#23091=VERTEX_POINT ( 'NONE', #8175 ) ;
#23092=AXIS2_PLACEMENT_3D ( 'NONE', #8390, #31245, #5008 ) ;
#23095=ORIENTED_EDGE ( 'NONE', *, *, #4341, .T. ) ;
#23096=ORIENTED_EDGE ( 'NONE', *, *, #19482, .T. ) ;
#23098=CARTESIAN_POINT ( 'NONE',  ( -84.88770934388888634, 10.65709906204123492, 12.50000000000000000 ) ) ;
#23099=AXIS2_PLACEMENT_3D ( 'NONE', #28381, #33842, #36660 ) ;
#23100=DIRECTION ( 'NONE',  ( 1.000000000000000000, 0.000000000000000000, 0.000000000000000000 ) ) ;
#23101=ADVANCED_FACE ( 'NONE', ( #25417 ), #1984, .T. ) ;
#23102=VERTEX_POINT ( 'NONE', #5179 ) ;
#23103=DIRECTION ( 'NONE',  ( 1.000000000000000000, 0.000000000000000000, 0.000000000000000000 ) ) ;
#23104=FACE_BOUND ( 'NONE', #9566, .T. ) ;
#23105=CARTESIAN_POINT ( 'NONE',  ( 47.99999662536846756, 69.28203230275516944, -9.999999999999998224 ) ) ;
#23107=DIRECTION ( 'NONE',  ( 0.000000000000000000, 0.000000000000000000, 1.000000000000000000 ) ) ;
#23108=CARTESIAN_POINT ( 'NONE',  ( -75.00000337463097821, 25.98076211353318854, -9.999999999999998224 ) ) ;
#23109=AXIS2_PLACEMENT_3D ( 'NONE', #12236, #35362, #31764 ) ;
#23110=ADVANCED_FACE ( 'NONE', ( #10810 ), #7986, .F. ) ;
#23111=LINE ( 'NONE', #29290, #7802 ) ;
#23113=EDGE_CURVE ( 'NONE', #15730, #2540, #12477, .T. ) ;
#23114=CARTESIAN_POINT ( 'NONE',  ( 84.99999662536831124, -8.660254037844397956, -9.999999999999998224 ) ) ;
#23115=ORIENTED_EDGE ( 'NONE', *, *, #31258, .F. ) ;
#23117=AXIS2_PLACEMENT_3D ( 'NONE', #8085, #22162, #13715 ) ;
#23118=( GEOMETRIC_REPRESENTATION_CONTEXT ( 3 ) GLOBAL_UNCERTAINTY_ASSIGNED_CONTEXT ( ( #17039 ) ) GLOBAL_UNIT_ASSIGNED_CONTEXT ( ( #10504, #15247, #1005 ) ) REPRESENTATION_CONTEXT ( 'NONE', 'WORKASPACE' ) );
#23121=AXIS2_PLACEMENT_3D ( 'NONE', #21312, #21512, #12296 ) ;
#23122=AXIS2_PLACEMENT_3D ( 'NONE', #24591, #13137, #7146 ) ;
#23123=ORIENTED_EDGE ( 'NONE', *, *, #9681, .T. ) ;
#23124=AXIS2_PLACEMENT_3D ( 'NONE', #13771, #64, #17128 ) ;
#23125=ORIENTED_EDGE ( 'NONE', *, *, #55, .F. ) ;
#23126=AXIS2_PLACEMENT_3D ( 'NONE', #8765, #28816, #3141 ) ;
#23127=ORIENTED_EDGE ( 'NONE', *, *, #36133, .T. ) ;
#23128=DIRECTION ( 'NONE',  ( 0.000000000000000000, 0.000000000000000000, 1.000000000000000000 ) ) ;
#23129=CARTESIAN_POINT ( 'NONE',  ( 84.99999662536832545, 8.660254037844394404, 12.50000000000000000 ) ) ;
#23130=DIRECTION ( 'NONE',  ( -1.000000000000000000, 0.000000000000000000, 0.000000000000000000 ) ) ;
#23131=ORIENTED_EDGE ( 'NONE', *, *, #32909, .T. ) ;
#23132=AXIS2_PLACEMENT_3D ( 'NONE', #22225, #5362, #16599 ) ;
#23133=CARTESIAN_POINT ( 'NONE',  ( 29.99999662536856349, 69.28203230275518365, -9.999999999999998224 ) ) ;
#23134=EDGE_CURVE ( 'NONE', #1955, #16077, #24470, .T. ) ;
#23135=EDGE_LOOP ( 'NONE', ( #3633, #34694, #10664 ) ) ;
#23138=DIRECTION ( 'NONE',  ( 0.000000000000000000, 0.000000000000000000, 1.000000000000000000 ) ) ;
#23139=ORIENTED_EDGE ( 'NONE', *, *, #31979, .T. ) ;
#23140=CIRCLE ( 'NONE', #13553, 2.000000000000001776 ) ;
#23141=EDGE_LOOP ( 'NONE', ( #33132, #17584, #4482 ) ) ;
#23143=VECTOR ( 'NONE', #23058, 1000.000000000000000 ) ;
#23144=CARTESIAN_POINT ( 'NONE',  ( -11.64413683707582337, -85.46375806488710225, -5.000000000000000000 ) ) ;
#23145=ORIENTED_EDGE ( 'NONE', *, *, #18624, .F. ) ;
#23150=AXIS2_PLACEMENT_3D ( 'NONE', #29098, #228, #8875 ) ;
#23153=VECTOR ( 'NONE', #27671, 1000.000000000000000 ) ;
#23154=EDGE_CURVE ( 'NONE', #31157, #8144, #2832, .T. ) ;
#23155=ORIENTED_EDGE ( 'NONE', *, *, #20907, .F. ) ;
#23156=CARTESIAN_POINT ( 'NONE',  ( -25.00000337463121980, -77.94228634059963667, -9.999999999999998224 ) ) ;
#23157=CARTESIAN_POINT ( 'NONE',  ( -68.00000337463099243, 34.64101615137758472, 12.50000000000000000 ) ) ;
#23158=EDGE_LOOP ( 'NONE', ( #1886, #21399 ) ) ;
#23159=EDGE_CURVE ( 'NONE', #29874, #4566, #17906, .T. ) ;
#23160=LINE ( 'NONE', #32333, #16637 ) ;
#23161=DIRECTION ( 'NONE',  ( -0.000000000000000000, -0.000000000000000000, 1.000000000000000000 ) ) ;
#23162=CARTESIAN_POINT ( 'NONE',  ( -8.000003374631281972, 86.60254037844397601, -9.999999999999998224 ) ) ;
#23163=DIRECTION ( 'NONE',  ( 0.000000000000000000, 0.000000000000000000, 1.000000000000000000 ) ) ;
#23164=AXIS2_PLACEMENT_3D ( 'NONE', #636, #28765, #32109 ) ;
#23165=EDGE_CURVE ( 'NONE', #11237, #27568, #32228, .T. ) ;
#23166=CARTESIAN_POINT ( 'NONE',  ( -83.67710216016716629, 27.48073957228723430, -5.000000000000000000 ) ) ;
#23167=ORIENTED_EDGE ( 'NONE', *, *, #22726, .T. ) ;
#23168=EDGE_CURVE ( 'NONE', #22827, #1125, #22668, .T. ) ;
#23169=DIRECTION ( 'NONE',  ( -0.000000000000000000, -0.000000000000000000, 1.000000000000000000 ) ) ;
#23170=CARTESIAN_POINT ( 'NONE',  ( -20.00000337463122690, 86.60254037844397601, 12.50000000000000000 ) ) ;
#23172=AXIS2_PLACEMENT_3D ( 'NONE', #18204, #9961, #29636 ) ;
#23173=ORIENTED_EDGE ( 'NONE', *, *, #25257, .F. ) ;
#23174=EDGE_LOOP ( 'NONE', ( #17995, #16566 ) ) ;
#23175=ORIENTED_EDGE ( 'NONE', *, *, #9420, .F. ) ;
#23176=AXIS2_PLACEMENT_3D ( 'NONE', #32601, #27360, #30352 ) ;
#23177=AXIS2_PLACEMENT_3D ( 'NONE', #19909, #17097, #592 ) ;
#23178=CARTESIAN_POINT ( 'NONE',  ( 24.99999662536857059, 77.94228634059957983, 17.49999999999999645 ) ) ;
#23179=CARTESIAN_POINT ( 'NONE',  ( 12.99999662536863632, -77.94228634059960825, -5.000000000000000000 ) ) ;
#23180=EDGE_CURVE ( 'NONE', #9210, #18862, #29336, .T. ) ;
#23181=AXIS2_PLACEMENT_3D ( 'NONE', #15071, #17890, #17691 ) ;
#23183=EDGE_CURVE ( 'NONE', #6394, #10047, #1114, .T. ) ;
#23184=VECTOR ( 'NONE', #25317, 1000.000000000000000 ) ;
#23185=AXIS2_PLACEMENT_3D ( 'NONE', #23359, #34795, #8719 ) ;
#23186=ADVANCED_FACE ( 'NONE', ( #17172 ), #23526, .T. ) ;
#23187=CYLINDRICAL_SURFACE ( 'NONE', #14679, 2.000000000000001776 ) ;
#23188=ORIENTED_EDGE ( 'NONE', *, *, #16075, .T. ) ;
#23189=EDGE_CURVE ( 'NONE', #17979, #15624, #25671, .T. ) ;
#23190=ADVANCED_FACE ( 'NONE', ( #6475 ), #31931, .F. ) ;
#23191=CARTESIAN_POINT ( 'NONE',  ( -30.00000337463119848, -69.28203230275522628, -5.000000000000000000 ) ) ;
#23192=VERTEX_POINT ( 'NONE', #34415 ) ;
#23193=FACE_BOUND ( 'NONE', #23318, .T. ) ;
#23194=AXIS2_PLACEMENT_3D ( 'NONE', #17951, #8763, #15307 ) ;
#23195=VECTOR ( 'NONE', #9801, 1000.000000000000000 ) ;
#23197=CARTESIAN_POINT ( 'NONE',  ( 46.99999662536849598, -77.94228634059960825, 12.50000000000000000 ) ) ;
#23198=DIRECTION ( 'NONE',  ( 0.000000000000000000, 0.000000000000000000, 1.000000000000000000 ) ) ;
#23201=CIRCLE ( 'NONE', #36406, 2.000000000000001776 ) ;
#23202=DIRECTION ( 'NONE',  ( 1.000000000000000000, 0.000000000000000000, 0.000000000000000000 ) ) ;
#23204=DIRECTION ( 'NONE',  ( 0.000000000000000000, 0.000000000000000000, 1.000000000000000000 ) ) ;
#23205=EDGE_LOOP ( 'NONE', ( #16396, #29050, #25137, #15100 ) ) ;
#23206=LINE ( 'NONE', #513, #19606 ) ;
#23207=DIRECTION ( 'NONE',  ( 1.000000000000000000, 0.000000000000000000, 0.000000000000000000 ) ) ;
#23208=CARTESIAN_POINT ( 'NONE',  ( 74.99999662536835388, -43.30127018922199511, -5.000000000000000000 ) ) ;
#23209=EDGE_LOOP ( 'NONE', ( #17477, #18807, #21985, #9238 ) ) ;
#23210=AXIS2_PLACEMENT_3D ( 'NONE', #10959, #2712, #30827 ) ;
#23211=EDGE_LOOP ( 'NONE', ( #26579, #7845, #2601, #23434, #15838 ) ) ;
#23212=EDGE_LOOP ( 'NONE', ( #19553, #27944, #11945, #6109 ) ) ;
#23213=DIRECTION ( 'NONE',  ( 0.000000000000000000, 0.000000000000000000, 1.000000000000000000 ) ) ;
#23214=AXIS2_PLACEMENT_3D ( 'NONE', #6270, #3475, #31586 ) ;
#23215=FACE_BOUND ( 'NONE', #18064, .T. ) ;
#23216=CIRCLE ( 'NONE', #14218, 2.000000000000001776 ) ;
#23218=CARTESIAN_POINT ( 'NONE',  ( 72.99999662536836809, -8.660254037844401509, -9.999999999999998224 ) ) ;
#23219=FACE_OUTER_BOUND ( 'NONE', #22490, .T. ) ;
#23221=AXIS2_PLACEMENT_3D ( 'NONE', #36041, #1723, #30757 ) ;
#23222=DIRECTION ( 'NONE',  ( 1.000000000000000000, 0.000000000000000000, 0.000000000000000000 ) ) ;
#23223=EDGE_LOOP ( 'NONE', ( #23038, #10900, #27285, #12751 ) ) ;
#23224=AXIS2_PLACEMENT_3D ( 'NONE', #26006, #34656, #693 ) ;
#23225=ADVANCED_FACE ( 'NONE', ( #99 ), #34966, .F. ) ;
#23226=ORIENTED_EDGE ( 'NONE', *, *, #11952, .T. ) ;
#23227=CARTESIAN_POINT ( 'NONE',  ( -72.00000337463100664, 17.32050807568877460, 17.49999999999999645 ) ) ;
#23229=EDGE_CURVE ( 'NONE', #1926, #17193, #828, .T. ) ;
#23230=DIRECTION ( 'NONE',  ( 0.000000000000000000, 0.000000000000000000, -1.000000000000000000 ) ) ;
#23231=EDGE_LOOP ( 'NONE', ( #13865, #29942, #19269, #24306 ) ) ;
#23232=VECTOR ( 'NONE', #27567, 1000.000000000000000 ) ;
#23233=DIRECTION ( 'NONE',  ( 0.000000000000000000, 0.000000000000000000, 1.000000000000000000 ) ) ;
#23235=ORIENTED_EDGE ( 'NONE', *, *, #8918, .T. ) ;
#23236=CARTESIAN_POINT ( 'NONE',  ( -4.279621169095561228, 62.97617850287782915, 12.49999999999999822 ) ) ;
#23237=ORIENTED_EDGE ( 'NONE', *, *, #5015, .F. ) ;
#23239=CARTESIAN_POINT ( 'NONE',  ( 59.99999662536842493, -51.96152422706639840, -5.000000000000000000 ) ) ;
#23240=AXIS2_PLACEMENT_3D ( 'NONE', #12993, #1555, #10200 ) ;
#23241=FACE_OUTER_BOUND ( 'NONE', #31446, .T. ) ;
#23242=ORIENTED_EDGE ( 'NONE', *, *, #16983, .T. ) ;
#23244=VERTEX_POINT ( 'NONE', #20163 ) ;
#23246=AXIS2_PLACEMENT_3D ( 'NONE', #35058, #9364, #32235 ) ;
#23247=ORIENTED_EDGE ( 'NONE', *, *, #30072, .T. ) ;
#23248=EDGE_CURVE ( 'NONE', #3582, #36402, #20771, .T. ) ;
#23250=ORIENTED_EDGE ( 'NONE', *, *, #455, .T. ) ;
#23251=EDGE_LOOP ( 'NONE', ( #2110, #8210, #29350, #33620 ) ) ;
#23253=DIRECTION ( 'NONE',  ( 0.4999999999999919509, -0.8660254037844432595, 0.000000000000000000 ) ) ;
#23254=DIRECTION ( 'NONE',  ( 0.000000000000000000, 0.000000000000000000, 1.000000000000000000 ) ) ;
#23256=DIRECTION ( 'NONE',  ( 0.000000000000000000, 0.000000000000000000, 1.000000000000000000 ) ) ;
#23257=AXIS2_PLACEMENT_3D ( 'NONE', #2095, #13529, #30973 ) ;
#23259=CARTESIAN_POINT ( 'NONE',  ( 4.999996625368645198, 77.94228634059957983, -5.000000000000000000 ) ) ;
#23260=ADVANCED_FACE ( 'NONE', ( #17360 ), #28782, .F. ) ;
#23261=AXIS2_PLACEMENT_3D ( 'NONE', #36257, #24252, #30061 ) ;
#23262=DIRECTION ( 'NONE',  ( 0.000000000000000000, 0.000000000000000000, 1.000000000000000000 ) ) ;
#23264=VERTEX_POINT ( 'NONE', #31769 ) ;
#23265=FACE_OUTER_BOUND ( 'NONE', #31178, .T. ) ;
#23267=CIRCLE ( 'NONE', #515, 2.000000000000001776 ) ;
#23272=CARTESIAN_POINT ( 'NONE',  ( 74.99999662536836809, 25.98076211353319565, -9.999999999999998224 ) ) ;
#23273=EDGE_CURVE ( 'NONE', #538, #22077, #30360, .T. ) ;
#23274=CARTESIAN_POINT ( 'NONE',  ( -75.00000337463100664, -43.30127018922202353, 12.50000000000000000 ) ) ;
#23275=CARTESIAN_POINT ( 'NONE',  ( 84.99999662536831124, -8.660254037844397956, -9.999999999999998224 ) ) ;
#23276=ORIENTED_EDGE ( 'NONE', *, *, #16243, .T. ) ;
#23277=VECTOR ( 'NONE', #11516, 1000.000000000000000 ) ;
#23278=CYLINDRICAL_SURFACE ( 'NONE', #18341, 33.00000000000001421 ) ;
#23279=CARTESIAN_POINT ( 'NONE',  ( -77.00000337463097821, -8.660254037844422825, -9.999999999999998224 ) ) ;
#23280=LINE ( 'NONE', #36982, #11093 ) ;
#23281=CIRCLE ( 'NONE', #3509, 2.000000000000001776 ) ;
#23282=VERTEX_POINT ( 'NONE', #3275 ) ;
#23283=AXIS2_PLACEMENT_3D ( 'NONE', #7961, #22786, #242 ) ;
#23286=AXIS2_PLACEMENT_3D ( 'NONE', #34481, #26028, #17243 ) ;
#23287=DIRECTION ( 'NONE',  ( 1.000000000000000000, 0.000000000000000000, 0.000000000000000000 ) ) ;
#23288=AXIS2_PLACEMENT_3D ( 'NONE', #20462, #3607, #28895 ) ;
#23289=CARTESIAN_POINT ( 'NONE',  ( 71.99999662536839651, -3.469446951953614189E-15, -9.999999999999998224 ) ) ;
#23290=EDGE_CURVE ( 'NONE', #25177, #20566, #14712, .T. ) ;
#23291=CARTESIAN_POINT ( 'NONE',  ( -95.00000000000001421, 1.163414459189985801E-14, -5.000000000000000000 ) ) ;
#23292=VERTEX_POINT ( 'NONE', #29506 ) ;
#23293=ORIENTED_EDGE ( 'NONE', *, *, #27980, .T. ) ;
#23294=CARTESIAN_POINT ( 'NONE',  ( 86.99999662536832545, 25.98076211353319565, 12.50000000000000000 ) ) ;
#23295=EDGE_CURVE ( 'NONE', #31156, #25326, #10017, .T. ) ;
#23296=DIRECTION ( 'NONE',  ( -1.047444401652940007E-14, -1.000000000000000000, 0.000000000000000000 ) ) ;
#23298=EDGE_LOOP ( 'NONE', ( #23332, #26601 ) ) ;
#23299=CARTESIAN_POINT ( 'NONE',  ( 27.78182860042856461, 56.67878100130339902, -4.999999999999997335 ) ) ;
#23300=AXIS2_PLACEMENT_3D ( 'NONE', #29780, #6724, #35435 ) ;
#23301=FACE_BOUND ( 'NONE', #80, .T. ) ;
#23303=ADVANCED_FACE ( 'NONE', ( #30246 ), #9653, .T. ) ;
#23304=AXIS2_PLACEMENT_3D ( 'NONE', #4293, #16113, #27702 ) ;
#23305=DIRECTION ( 'NONE',  ( 0.000000000000000000, 0.000000000000000000, 1.000000000000000000 ) ) ;
#23307=DIRECTION ( 'NONE',  ( 1.000000000000000000, 0.000000000000000000, 0.000000000000000000 ) ) ;
#23308=CARTESIAN_POINT ( 'NONE',  ( 72.99999662536836809, 8.660254037844394404, -9.999999999999998224 ) ) ;
#23309=DIRECTION ( 'NONE',  ( 0.000000000000000000, 0.000000000000000000, 1.000000000000000000 ) ) ;
#23310=EDGE_CURVE ( 'NONE', #28932, #32680, #17203, .T. ) ;
#23311=CIRCLE ( 'NONE', #16736, 2.000000000000001776 ) ;
#23313=ORIENTED_EDGE ( 'NONE', *, *, #15713, .F. ) ;
#23314=CARTESIAN_POINT ( 'NONE',  ( 11.64412580323855018, 85.46375187899521109, -5.000000000000000000 ) ) ;
#23315=PLANE ( 'NONE',  #17738 ) ;
#23317=AXIS2_PLACEMENT_3D ( 'NONE', #36340, #13264, #25100 ) ;
#23318=EDGE_LOOP ( 'NONE', ( #2534, #34872 ) ) ;
#23319=EDGE_LOOP ( 'NONE', ( #25598, #9678, #13381, #2744 ) ) ;
#23320=CIRCLE ( 'NONE', #18537, 2.000000000000001776 ) ;
#23322=FACE_OUTER_BOUND ( 'NONE', #9233, .T. ) ;
#23323=ADVANCED_FACE ( 'NONE', ( #33070 ), #27073, .F. ) ;
#23324=CARTESIAN_POINT ( 'NONE',  ( 93.36492675454790913, 17.14523346298246409, 12.49999999999999822 ) ) ;
#23325=AXIS2_PLACEMENT_3D ( 'NONE', #6657, #14719, #26709 ) ;
#23327=ORIENTED_EDGE ( 'NONE', *, *, #15587, .T. ) ;
#23328=CYLINDRICAL_SURFACE ( 'NONE', #11892, 2.000000000000001776 ) ;
#23329=EDGE_CURVE ( 'NONE', #31662, #19701, #4663, .T. ) ;
#23330=CIRCLE ( 'NONE', #15538, 2.000000000000001776 ) ;
#23331=AXIS2_PLACEMENT_3D ( 'NONE', #31044, #27842, #13807 ) ;
#23332=ORIENTED_EDGE ( 'NONE', *, *, #30114, .F. ) ;
#23335=AXIS2_PLACEMENT_3D ( 'NONE', #28437, #28262, #31085 ) ;
#23336=FACE_OUTER_BOUND ( 'NONE', #633, .T. ) ;
#23337=ORIENTED_EDGE ( 'NONE', *, *, #9423, .T. ) ;
#23338=ORIENTED_EDGE ( 'NONE', *, *, #13569, .F. ) ;
#23339=ADVANCED_FACE ( 'NONE', ( #4222 ), #27451, .T. ) ;
#23340=CARTESIAN_POINT ( 'NONE',  ( 39.99999662536853151, 69.28203230275518365, 17.49999999999999645 ) ) ;
#23341=DIRECTION ( 'NONE',  ( -1.000000000000000000, 0.000000000000000000, -0.000000000000000000 ) ) ;
#23342=ADVANCED_FACE ( 'NONE', ( #21078 ), #1382, .F. ) ;
#23343=DIRECTION ( 'NONE',  ( -1.000000000000000000, 0.000000000000000000, 0.000000000000000000 ) ) ;
#23347=AXIS2_PLACEMENT_3D ( 'NONE', #24673, #10403, #33283 ) ;
#23349=CARTESIAN_POINT ( 'NONE',  ( 81.99999662536832545, -17.32050807568879591, -9.999999999999998224 ) ) ;
#23350=ORIENTED_EDGE ( 'NONE', *, *, #6074, .T. ) ;
#23351=CARTESIAN_POINT ( 'NONE',  ( 0.000000000000000000, 0.000000000000000000, 12.49999999999999822 ) ) ;
#23352=CYLINDRICAL_SURFACE ( 'NONE', #2993, 2.000000000000001776 ) ;
#23354=AXIS2_PLACEMENT_3D ( 'NONE', #9613, #24045, #30206 ) ;
#23355=DIRECTION ( 'NONE',  ( 0.000000000000000000, 0.000000000000000000, 1.000000000000000000 ) ) ;
#23356=ADVANCED_FACE ( 'NONE', ( #15821 ), #21459, .F. ) ;
#23357=CARTESIAN_POINT ( 'NONE',  ( -50.00000337463112032, -51.96152422706641971, -9.999999999999998224 ) ) ;
#23358=CIRCLE ( 'NONE', #4788, 2.000000000000000000 ) ;
#23359=CARTESIAN_POINT ( 'NONE',  ( -35.00000337463116296, -60.62177826491080168, -9.999999999999998224 ) ) ;
#23360=DIRECTION ( 'NONE',  ( 1.000000000000000000, 0.000000000000000000, 0.000000000000000000 ) ) ;
#23361=CARTESIAN_POINT ( 'NONE',  ( -5.000003374631269537, -77.94228634059960825, 12.50000000000000000 ) ) ;
#23362=EDGE_CURVE ( 'NONE', #32711, #33803, #20801, .T. ) ;
#23363=AXIS2_PLACEMENT_3D ( 'NONE', #9137, #4090, #20962 ) ;
#23364=DIRECTION ( 'NONE',  ( 0.000000000000000000, 0.000000000000000000, 1.000000000000000000 ) ) ;
#23365=ORIENTED_EDGE ( 'NONE', *, *, #16117, .T. ) ;
#23367=AXIS2_PLACEMENT_3D ( 'NONE', #17355, #19802, #11350 ) ;
#23368=FACE_OUTER_BOUND ( 'NONE', #17450, .T. ) ;
#23369=DIRECTION ( 'NONE',  ( -1.000000000000000000, 0.000000000000000000, 0.000000000000000000 ) ) ;
#23370=ORIENTED_EDGE ( 'NONE', *, *, #28161, .F. ) ;
#23371=EDGE_LOOP ( 'NONE', ( #23901, #20588, #23188, #22614 ) ) ;
#23372=ORIENTED_EDGE ( 'NONE', *, *, #21758, .F. ) ;
#23373=DIRECTION ( 'NONE',  ( 1.000000000000000000, 0.000000000000000000, 0.000000000000000000 ) ) ;
#23374=DIRECTION ( 'NONE',  ( 1.000000000000000000, 0.000000000000000000, 0.000000000000000000 ) ) ;
#23375=CARTESIAN_POINT ( 'NONE',  ( 47.63139720814418610, 27.49999999999988987, -10.00000000000000178 ) ) ;
#23376=AXIS2_PLACEMENT_3D ( 'NONE', #36743, #10314, #2052 ) ;
#23378=CARTESIAN_POINT ( 'NONE',  ( -38.00000337463113453, 69.28203230275516944, -9.999999999999998224 ) ) ;
#23379=ORIENTED_EDGE ( 'NONE', *, *, #4087, .F. ) ;
#23380=CIRCLE ( 'NONE', #616, 2.000000000000001776 ) ;
#23381=LINE ( 'NONE', #850, #24529 ) ;
#23383=FACE_BOUND ( 'NONE', #25107, .T. ) ;
#23384=AXIS2_PLACEMENT_3D ( 'NONE', #24737, #35999, #16669 ) ;
#23386=CARTESIAN_POINT ( 'NONE',  ( 41.99999662536853151, 69.28203230275518365, -9.999999999999998224 ) ) ;
#23388=DIRECTION ( 'NONE',  ( 0.000000000000000000, 0.000000000000000000, 1.000000000000000000 ) ) ;
#23390=VERTEX_POINT ( 'NONE', #12636 ) ;
#23391=DIRECTION ( 'NONE',  ( 0.000000000000000000, 0.000000000000000000, 1.000000000000000000 ) ) ;
#23393=DIRECTION ( 'NONE',  ( 0.000000000000000000, 0.000000000000000000, -1.000000000000000000 ) ) ;
#23394=FACE_OUTER_BOUND ( 'NONE', #7102, .T. ) ;
#23396=ORIENTED_EDGE ( 'NONE', *, *, #32863, .T. ) ;
#23397=CARTESIAN_POINT ( 'NONE',  ( 76.99999662536835388, -25.98076211353319565, 12.50000000000000000 ) ) ;
#23399=DIRECTION ( 'NONE',  ( 1.000000000000000000, 0.000000000000000000, 0.000000000000000000 ) ) ;
#23400=ORIENTED_EDGE ( 'NONE', *, *, #33414, .T. ) ;
#23401=VERTEX_POINT ( 'NONE', #24084 ) ;
#23403=AXIS2_PLACEMENT_3D ( 'NONE', #6320, #22669, #28452 ) ;
#23404=ORIENTED_EDGE ( 'NONE', *, *, #8740, .F. ) ;
#23405=DIRECTION ( 'NONE',  ( -1.000000000000000000, 0.000000000000000000, 0.000000000000000000 ) ) ;
#23406=DIRECTION ( 'NONE',  ( 1.000000000000000000, 0.000000000000000000, 0.000000000000000000 ) ) ;
#23407=CARTESIAN_POINT ( 'NONE',  ( 62.97617850287784336, 4.279621169095339184, -4.999999999999997335 ) ) ;
#23408=CARTESIAN_POINT ( 'NONE',  ( 68.66839587347284635, 56.74224907228958870, -4.999999999999997335 ) ) ;
#23409=DIRECTION ( 'NONE',  ( 0.000000000000000000, 0.000000000000000000, -1.000000000000000000 ) ) ;
#23410=CARTESIAN_POINT ( 'NONE',  ( 87.99999662536828282, 2.449293598294703949E-16, 17.49999999999999645 ) ) ;
#23411=ORIENTED_EDGE ( 'NONE', *, *, #23552, .T. ) ;
#23412=ORIENTED_EDGE ( 'NONE', *, *, #33856, .T. ) ;
#23413=DIRECTION ( 'NONE',  ( 1.000000000000000000, 0.000000000000000000, 0.000000000000000000 ) ) ;
#23415=CARTESIAN_POINT ( 'NONE',  ( -2.778182860042071933, 69.13212189986968781, -4.999999999999997335 ) ) ;
#23416=EDGE_CURVE ( 'NONE', #28072, #15480, #12418, .T. ) ;
#23417=FACE_OUTER_BOUND ( 'NONE', #2257, .T. ) ;
#23418=ORIENTED_EDGE ( 'NONE', *, *, #33529, .T. ) ;
#23419=FACE_BOUND ( 'NONE', #17222, .T. ) ;
#23420=ORIENTED_EDGE ( 'NONE', *, *, #8641, .F. ) ;
#23421=EDGE_LOOP ( 'NONE', ( #14329, #13879, #19178, #33743 ) ) ;
#23425=ORIENTED_EDGE ( 'NONE', *, *, #19716, .T. ) ;
#23426=DIRECTION ( 'NONE',  ( 1.000000000000000000, 0.000000000000000000, 0.000000000000000000 ) ) ;
#23427=CARTESIAN_POINT ( 'NONE',  ( 44.99999662536849598, 60.62177826491077326, -9.999999999999998224 ) ) ;
#23428=DIRECTION ( 'NONE',  ( 1.000000000000000000, 0.000000000000000000, 0.000000000000000000 ) ) ;
#23429=VERTEX_POINT ( 'NONE', #36261 ) ;
#23430=ORIENTED_EDGE ( 'NONE', *, *, #24225, .T. ) ;
#23431=EDGE_CURVE ( 'NONE', #36358, #15508, #8241, .T. ) ;
#23432=ORIENTED_EDGE ( 'NONE', *, *, #16584, .T. ) ;
#23433=EDGE_CURVE ( 'NONE', #33197, #33432, #2240, .T. ) ;
#23434=ORIENTED_EDGE ( 'NONE', *, *, #25069, .F. ) ;
#23437=CARTESIAN_POINT ( 'NONE',  ( 67.99999662536838230, -3.224517592124143893E-15, -9.999999999999998224 ) ) ;
#23438=ADVANCED_FACE ( 'NONE', ( #33640 ), #7770, .F. ) ;
#23439=EDGE_LOOP ( 'NONE', ( #14619, #14799, #25682, #18410 ) ) ;
#23440=CIRCLE ( 'NONE', #21025, 2.000000000000000000 ) ;
#23441=CARTESIAN_POINT ( 'NONE',  ( 1.999996625368696490, -86.60254037844400443, -9.999999999999998224 ) ) ;
#23442=DIRECTION ( 'NONE',  ( 1.000000000000000000, 0.000000000000000000, 0.000000000000000000 ) ) ;
#23443=DIRECTION ( 'NONE',  ( 1.000000000000000000, 0.000000000000000000, 0.000000000000000000 ) ) ;
#23444=VERTEX_POINT ( 'NONE', #27629 ) ;
#23445=DIRECTION ( 'NONE',  ( 0.000000000000000000, 0.000000000000000000, -1.000000000000000000 ) ) ;
#23446=LINE ( 'NONE', #34884, #2422 ) ;
#23447=CARTESIAN_POINT ( 'NONE',  ( -65.00000337463102085, 25.98076211353317433, 12.50000000000000000 ) ) ;
#23448=ORIENTED_EDGE ( 'NONE', *, *, #12393, .F. ) ;
#23449=CARTESIAN_POINT ( 'NONE',  ( -30.00000337463119848, -69.28203230275522628, -9.999999999999998224 ) ) ;
#23450=CARTESIAN_POINT ( 'NONE',  ( -63.00000337463104927, -25.98076211353322051, -9.999999999999998224 ) ) ;
#23451=EDGE_LOOP ( 'NONE', ( #5363, #18063 ) ) ;
#23452=ORIENTED_EDGE ( 'NONE', *, *, #15836, .F. ) ;
#23453=DIRECTION ( 'NONE',  ( 0.000000000000000000, 0.000000000000000000, -1.000000000000000000 ) ) ;
#23454=DIRECTION ( 'NONE',  ( 0.000000000000000000, 0.000000000000000000, -1.000000000000000000 ) ) ;
#23455=DIRECTION ( 'NONE',  ( 0.000000000000000000, 0.000000000000000000, -1.000000000000000000 ) ) ;
#23457=ORIENTED_EDGE ( 'NONE', *, *, #15967, .T. ) ;
#23459=CARTESIAN_POINT ( 'NONE',  ( -68.00000337463099243, 34.64101615137758472, -9.999999999999998224 ) ) ;
#23460=CARTESIAN_POINT ( 'NONE',  ( -78.00000337463094979, 17.32050807568878525, 17.49999999999999645 ) ) ;
#23461=FACE_OUTER_BOUND ( 'NONE', #5012, .T. ) ;
#23462=ORIENTED_EDGE ( 'NONE', *, *, #36536, .T. ) ;
#23463=VECTOR ( 'NONE', #30443, 1000.000000000000000 ) ;
#23464=CIRCLE ( 'NONE', #12665, 2.000000000000001776 ) ;
#23465=DIRECTION ( 'NONE',  ( 1.000000000000000000, 0.000000000000000000, 0.000000000000000000 ) ) ;
#23466=EDGE_LOOP ( 'NONE', ( #21308, #35137, #12364, #12115 ) ) ;
#23467=LINE ( 'NONE', #15401, #5736 ) ;
#23468=CARTESIAN_POINT ( 'NONE',  ( 44.99999662536849598, 60.62177826491077326, 17.49999999999999645 ) ) ;
#23470=ORIENTED_EDGE ( 'NONE', *, *, #30741, .T. ) ;
#23471=VERTEX_POINT ( 'NONE', #11313 ) ;
#23472=CARTESIAN_POINT ( 'NONE',  ( 74.99999662536835388, -25.98076211353319565, 17.49999999999999645 ) ) ;
#23473=DIRECTION ( 'NONE',  ( 1.000000000000000000, 0.000000000000000000, 0.000000000000000000 ) ) ;
#23474=DIRECTION ( 'NONE',  ( -1.000000000000000000, 0.000000000000000000, 0.000000000000000000 ) ) ;
#23476=DIRECTION ( 'NONE',  ( 0.000000000000000000, 0.000000000000000000, 1.000000000000000000 ) ) ;
#23477=EDGE_CURVE ( 'NONE', #33271, #20440, #7031, .T. ) ;
#23478=FACE_BOUND ( 'NONE', #19955, .T. ) ;
#23479=DIRECTION ( 'NONE',  ( 0.000000000000000000, 0.000000000000000000, 1.000000000000000000 ) ) ;
#23480=CARTESIAN_POINT ( 'NONE',  ( 27.99999662536855993, 69.28203230275518365, 12.50000000000000000 ) ) ;
#23481=DIRECTION ( 'NONE',  ( -1.000000000000000000, 0.000000000000000000, 0.000000000000000000 ) ) ;
#23482=ORIENTED_EDGE ( 'NONE', *, *, #10957, .T. ) ;
#23483=DIRECTION ( 'NONE',  ( -1.000000000000000000, 0.000000000000000000, -0.000000000000000000 ) ) ;
#23484=CARTESIAN_POINT ( 'NONE',  ( 49.99999662536846756, 69.28203230275516944, -9.999999999999998224 ) ) ;
#23485=AXIS2_PLACEMENT_3D ( 'NONE', #411, #5877, #2505 ) ;
#23486=DIRECTION ( 'NONE',  ( 1.000000000000000000, 0.000000000000000000, 0.000000000000000000 ) ) ;
#23488=CYLINDRICAL_SURFACE ( 'NONE', #25624, 2.000000000000001776 ) ;
#23489=CARTESIAN_POINT ( 'NONE',  ( 81.99999662536833966, 17.32050807568879236, -9.999999999999998224 ) ) ;
#23491=ORIENTED_EDGE ( 'NONE', *, *, #31226, .F. ) ;
#23493=ORIENTED_EDGE ( 'NONE', *, *, #2444, .T. ) ;
#23494=DIRECTION ( 'NONE',  ( 0.000000000000000000, 0.000000000000000000, 1.000000000000000000 ) ) ;
#23495=FACE_OUTER_BOUND ( 'NONE', #28813, .T. ) ;
#23496=DIRECTION ( 'NONE',  ( 0.000000000000000000, 0.000000000000000000, -1.000000000000000000 ) ) ;
#23498=ORIENTED_EDGE ( 'NONE', *, *, #19497, .T. ) ;
#23499=EDGE_CURVE ( 'NONE', #7111, #36249, #9441, .T. ) ;
#23500=CIRCLE ( 'NONE', #7339, 2.000000000000001776 ) ;
#23502=AXIS2_PLACEMENT_3D ( 'NONE', #29861, #24798, #35500 ) ;
#23503=ORIENTED_EDGE ( 'NONE', *, *, #12726, .T. ) ;
#23504=DIRECTION ( 'NONE',  ( 1.000000000000000000, 0.000000000000000000, 0.000000000000000000 ) ) ;
#23506=VERTEX_POINT ( 'NONE', #19214 ) ;
#23507=CARTESIAN_POINT ( 'NONE',  ( -75.00000337463097821, 43.30127018922197379, -9.999999999999998224 ) ) ;
#23508=ORIENTED_EDGE ( 'NONE', *, *, #35810, .F. ) ;
#23510=EDGE_CURVE ( 'NONE', #8606, #16595, #8125, .T. ) ;
#23511=DIRECTION ( 'NONE',  ( -0.000000000000000000, -0.000000000000000000, 1.000000000000000000 ) ) ;
#23512=DIRECTION ( 'NONE',  ( 0.000000000000000000, 0.000000000000000000, 1.000000000000000000 ) ) ;
#23513=FACE_OUTER_BOUND ( 'NONE', #35302, .T. ) ;
#23515=VERTEX_POINT ( 'NONE', #37005 ) ;
#23518=DIRECTION ( 'NONE',  ( 0.000000000000000000, 0.000000000000000000, 1.000000000000000000 ) ) ;
#23520=ORIENTED_EDGE ( 'NONE', *, *, #11211, .F. ) ;
#23521=DIRECTION ( 'NONE',  ( 1.000000000000000000, 0.000000000000000000, 0.000000000000000000 ) ) ;
#23522=CARTESIAN_POINT ( 'NONE',  ( -20.00000337463123756, -69.28203230275522628, 12.50000000000000000 ) ) ;
#23523=EDGE_LOOP ( 'NONE', ( #15805, #18871, #26669, #1183 ) ) ;
#23524=EDGE_CURVE ( 'NONE', #19449, #5559, #31558, .T. ) ;
#23525=CARTESIAN_POINT ( 'NONE',  ( 31.99999662536857770, -69.28203230275519786, 12.50000000000000000 ) ) ;
#23526=CYLINDRICAL_SURFACE ( 'NONE', #14872, 3.000000000000002665 ) ;
#23528=CARTESIAN_POINT ( 'NONE',  ( -43.00000337463111322, -77.94228634059960825, -9.999999999999998224 ) ) ;
#23529=AXIS2_PLACEMENT_3D ( 'NONE', #14460, #12164, #17621 ) ;
#23530=CARTESIAN_POINT ( 'NONE',  ( 52.39915983220795681, 35.19434990244919703, 12.49999999999999822 ) ) ;
#23531=CARTESIAN_POINT ( 'NONE',  ( 84.99999662536831124, -25.98076211353319565, 12.50000000000000000 ) ) ;
#23533=DIRECTION ( 'NONE',  ( -1.000000000000000000, 0.000000000000000000, 0.000000000000000000 ) ) ;
#23535=CARTESIAN_POINT ( 'NONE',  ( 1.999996625368672287, 86.60254037844397601, -9.999999999999998224 ) ) ;
#23537=VERTEX_POINT ( 'NONE', #10765 ) ;
#23539=EDGE_CURVE ( 'NONE', #22150, #3127, #16032, .T. ) ;
#23541=DIRECTION ( 'NONE',  ( 0.000000000000000000, 0.000000000000000000, -1.000000000000000000 ) ) ;
#23542=DIRECTION ( 'NONE',  ( -1.000000000000000000, 0.000000000000000000, 0.000000000000000000 ) ) ;
#23545=EDGE_LOOP ( 'NONE', ( #15435, #23127, #21841, #22823 ) ) ;
#23546=DIRECTION ( 'NONE',  ( 0.000000000000000000, 0.000000000000000000, 1.000000000000000000 ) ) ;
#23548=EDGE_LOOP ( 'NONE', ( #36379, #12292, #29011, #18357 ) ) ;
#23549=FACE_BOUND ( 'NONE', #3795, .T. ) ;
#23551=CIRCLE ( 'NONE', #7393, 1.999999999999998224 ) ;
#23552=EDGE_CURVE ( 'NONE', #18905, #5915, #7652, .T. ) ;
#23553=DIRECTION ( 'NONE',  ( -1.000000000000000000, 0.000000000000000000, 0.000000000000000000 ) ) ;
#23554=CARTESIAN_POINT ( 'NONE',  ( -77.00000337463097821, 25.98076211353318854, -5.000000000000000000 ) ) ;
#23555=ORIENTED_EDGE ( 'NONE', *, *, #4630, .F. ) ;
#23558=CARTESIAN_POINT ( 'NONE',  ( 2.778182860042562208, -69.13212189986967360, 12.49999999999999645 ) ) ;
#23559=AXIS2_PLACEMENT_3D ( 'NONE', #5684, #22769, #2686 ) ;
#23560=DIRECTION ( 'NONE',  ( 0.000000000000000000, 0.000000000000000000, 1.000000000000000000 ) ) ;
#23561=DIRECTION ( 'NONE',  ( 0.000000000000000000, 0.000000000000000000, 1.000000000000000000 ) ) ;
#23562=VERTEX_POINT ( 'NONE', #36456 ) ;
#23563=CARTESIAN_POINT ( 'NONE',  ( 61.25926521283101067, -32.16008401677932227, -49.22241343995298024 ) ) ;
#23564=DIRECTION ( 'NONE',  ( 0.000000000000000000, 0.000000000000000000, 1.000000000000000000 ) ) ;
#23565=DIRECTION ( 'NONE',  ( 0.000000000000000000, 0.000000000000000000, 1.000000000000000000 ) ) ;
#23566=EDGE_LOOP ( 'NONE', ( #32488, #24976, #23247, #31773 ) ) ;
#23567=EDGE_CURVE ( 'NONE', #14423, #17871, #1031, .T. ) ;
#23568=ORIENTED_EDGE ( 'NONE', *, *, #11293, .T. ) ;
#23569=VERTEX_POINT ( 'NONE', #2504 ) ;
#23571=CARTESIAN_POINT ( 'NONE',  ( -78.00000337463094979, -2.428612866367529932E-14, -9.999999999999998224 ) ) ;
#23572=ADVANCED_FACE ( 'NONE', ( #2329 ), #13758, .F. ) ;
#23573=CIRCLE ( 'NONE', #3234, 3.000000000000001332 ) ;
#23574=DIRECTION ( 'NONE',  ( -0.8660254037844449249, -0.4999999999999888423, 0.000000000000000000 ) ) ;
#23575=ORIENTED_EDGE ( 'NONE', *, *, #1709, .F. ) ;
#23576=EDGE_CURVE ( 'NONE', #16224, #16338, #14809, .T. ) ;
#23577=LINE ( 'NONE', #138, #17569 ) ;
#23579=CARTESIAN_POINT ( 'NONE',  ( 69.99999662536839651, 17.32050807568879236, 17.49999999999999645 ) ) ;
#23581=AXIS2_PLACEMENT_3D ( 'NONE', #7801, #10409, #34188 ) ;
#23582=ORIENTED_EDGE ( 'NONE', *, *, #34537, .F. ) ;
#23584=AXIS2_PLACEMENT_3D ( 'NONE', #24787, #36418, #10342 ) ;
#23585=DIRECTION ( 'NONE',  ( 0.000000000000000000, 0.000000000000000000, 1.000000000000000000 ) ) ;
#23586=EDGE_LOOP ( 'NONE', ( #30524, #10088, #21427, #31495 ) ) ;
#23588=VERTEX_POINT ( 'NONE', #17313 ) ;
#23589=ADVANCED_FACE ( 'NONE', ( #31536 ), #5674, .F. ) ;
#23590=FACE_BOUND ( 'NONE', #15888, .T. ) ;
#23592=EDGE_LOOP ( 'NONE', ( #13421, #29004, #24147, #32430 ) ) ;
#23593=DIRECTION ( 'NONE',  ( -1.000000000000000000, 0.000000000000000000, 0.000000000000000000 ) ) ;
#23597=DIRECTION ( 'NONE',  ( -1.000000000000000000, 0.000000000000000000, 0.000000000000000000 ) ) ;
#23598=DIRECTION ( 'NONE',  ( 0.000000000000000000, 0.000000000000000000, 1.000000000000000000 ) ) ;
#23599=CARTESIAN_POINT ( 'NONE',  ( -77.00000337463100664, -43.30127018922202353, -9.999999999999998224 ) ) ;
#23602=VERTEX_POINT ( 'NONE', #31723 ) ;
#23603=CIRCLE ( 'NONE', #27780, 27.00000000000001421 ) ;
#23604=ORIENTED_EDGE ( 'NONE', *, *, #11003, .F. ) ;
#23605=ADVANCED_FACE ( 'NONE', ( #3612 ), #28547, .F. ) ;
#23607=DIRECTION ( 'NONE',  ( 1.000000000000000000, 0.000000000000000000, 0.000000000000000000 ) ) ;
#23609=DIRECTION ( 'NONE',  ( -0.000000000000000000, -0.000000000000000000, 1.000000000000000000 ) ) ;
#23611=ORIENTED_EDGE ( 'NONE', *, *, #15294, .F. ) ;
#23613=DIRECTION ( 'NONE',  ( 0.000000000000000000, 0.000000000000000000, 1.000000000000000000 ) ) ;
#23615=ORIENTED_EDGE ( 'NONE', *, *, #27206, .F. ) ;
#23616=CARTESIAN_POINT ( 'NONE',  ( 39.99999662536853151, -69.28203230275519786, -9.999999999999998224 ) ) ;
#23617=EDGE_CURVE ( 'NONE', #6269, #6911, #8668, .T. ) ;
#23618=CARTESIAN_POINT ( 'NONE',  ( -2.000003374631303732, -86.60254037844400443, -9.999999999999998224 ) ) ;
#23620=ORIENTED_EDGE ( 'NONE', *, *, #7602, .F. ) ;
#23621=DIRECTION ( 'NONE',  ( 1.000000000000000000, 0.000000000000000000, 0.000000000000000000 ) ) ;
#23622=AXIS2_PLACEMENT_3D ( 'NONE', #4483, #24565, #7988 ) ;
#23623=EDGE_CURVE ( 'NONE', #21452, #23390, #37017, .T. ) ;
#23624=CYLINDRICAL_SURFACE ( 'NONE', #25568, 2.000000000000001776 ) ;
#23625=EDGE_CURVE ( 'NONE', #35979, #16326, #15041, .T. ) ;
#23626=ORIENTED_EDGE ( 'NONE', *, *, #27611, .F. ) ;
#23627=AXIS2_PLACEMENT_3D ( 'NONE', #30172, #10490, #19314 ) ;
#23631=DIRECTION ( 'NONE',  ( 0.000000000000000000, 0.000000000000000000, -1.000000000000000000 ) ) ;
#23633=EDGE_LOOP ( 'NONE', ( #383, #22939, #14787, #22579 ) ) ;
#23634=EDGE_CURVE ( 'NONE', #4217, #30962, #30424, .T. ) ;
#23635=AXIS2_PLACEMENT_3D ( 'NONE', #15907, #10280, #24350 ) ;
#23637=CIRCLE ( 'NONE', #9848, 2.000000000000001776 ) ;
#23638=EDGE_CURVE ( 'NONE', #12313, #19362, #17233, .T. ) ;
#23639=DIRECTION ( 'NONE',  ( 1.000000000000000000, 0.000000000000000000, 0.000000000000000000 ) ) ;
#23640=EDGE_CURVE ( 'NONE', #10635, #9991, #19926, .T. ) ;
#23641=CIRCLE ( 'NONE', #7479, 2.000000000000000000 ) ;
#23643=EDGE_CURVE ( 'NONE', #12555, #25896, #33431, .T. ) ;
#23646=CARTESIAN_POINT ( 'NONE',  ( -85.00000337463092137, 25.98076211353317433, -9.999999999999998224 ) ) ;
#23648=DIRECTION ( 'NONE',  ( 0.000000000000000000, 0.000000000000000000, -1.000000000000000000 ) ) ;
#23650=CIRCLE ( 'NONE', #29009, 27.00000000000001776 ) ;
#23652=CARTESIAN_POINT ( 'NONE',  ( -80.00000337463094979, 17.32050807568878525, -5.000000000000000000 ) ) ;
#23653=DIRECTION ( 'NONE',  ( 1.000000000000000000, 0.000000000000000000, 0.000000000000000000 ) ) ;
#23654=DIRECTION ( 'NONE',  ( -1.000000000000000000, 0.000000000000000000, 0.000000000000000000 ) ) ;
#23655=VECTOR ( 'NONE', #14974, 1000.000000000000000 ) ;
#23657=CARTESIAN_POINT ( 'NONE',  ( 16.99999662536863454, -77.94228634059960825, 17.49999999999999645 ) ) ;
#23658=FACE_BOUND ( 'NONE', #24672, .T. ) ;
#23660=DIRECTION ( 'NONE',  ( 0.000000000000000000, 0.000000000000000000, -1.000000000000000000 ) ) ;
#23661=FACE_OUTER_BOUND ( 'NONE', #34037, .T. ) ;
#23662=VERTEX_POINT ( 'NONE', #23105 ) ;
#23663=PLANE ( 'NONE',  #35678 ) ;
#23666=ORIENTED_EDGE ( 'NONE', *, *, #67, .T. ) ;
#23667=DIRECTION ( 'NONE',  ( 0.000000000000000000, 0.000000000000000000, 1.000000000000000000 ) ) ;
#23668=DIRECTION ( 'NONE',  ( -1.000000000000000000, 0.000000000000000000, 0.000000000000000000 ) ) ;
#23669=DIRECTION ( 'NONE',  ( 0.000000000000000000, 0.000000000000000000, 1.000000000000000000 ) ) ;
#23671=VERTEX_POINT ( 'NONE', #25922 ) ;
#23672=ORIENTED_EDGE ( 'NONE', *, *, #7367, .T. ) ;
#23673=AXIS2_PLACEMENT_3D ( 'NONE', #7389, #27075, #24468 ) ;
#23675=CYLINDRICAL_SURFACE ( 'NONE', #7975, 2.000000000000000000 ) ;
#23676=AXIS2_PLACEMENT_3D ( 'NONE', #4587, #19218, #35530 ) ;
#23678=ORIENTED_EDGE ( 'NONE', *, *, #4124, .F. ) ;
#23679=ORIENTED_EDGE ( 'NONE', *, *, #22316, .F. ) ;
#23680=ORIENTED_EDGE ( 'NONE', *, *, #21355, .T. ) ;
#23681=AXIS2_PLACEMENT_3D ( 'NONE', #4925, #1922, #21789 ) ;
#23682=CIRCLE ( 'NONE', #20062, 1.999999999999998224 ) ;
#23683=AXIS2_PLACEMENT_3D ( 'NONE', #13634, #28247, #22433 ) ;
#23684=CARTESIAN_POINT ( 'NONE',  ( 27.78182860042856461, 56.67878100130339902, -49.86348611802629449 ) ) ;
#23685=CIRCLE ( 'NONE', #2733, 2.000000000000000000 ) ;
#23686=VERTEX_POINT ( 'NONE', #34558 ) ;
#23689=ORIENTED_EDGE ( 'NONE', *, *, #18480, .F. ) ;
#23691=EDGE_LOOP ( 'NONE', ( #20389, #20368, #11958 ) ) ;
#23693=VERTEX_POINT ( 'NONE', #34366 ) ;
#23694=AXIS2_PLACEMENT_3D ( 'NONE', #23966, #18318, #4083 ) ;
#23695=CARTESIAN_POINT ( 'NONE',  ( 17.99999662536861678, -69.28203230275519786, 12.50000000000000000 ) ) ;
#23696=FACE_BOUND ( 'NONE', #27892, .T. ) ;
#23698=ORIENTED_EDGE ( 'NONE', *, *, #19334, .F. ) ;
#23700=DIRECTION ( 'NONE',  ( 0.000000000000000000, 0.000000000000000000, 1.000000000000000000 ) ) ;
#23702=CARTESIAN_POINT ( 'NONE',  ( -28.00000337463119493, -69.28203230275522628, -5.000000000000000000 ) ) ;
#23703=CARTESIAN_POINT ( 'NONE',  ( 89.99999662536828282, 0.000000000000000000, 17.49999999999999645 ) ) ;
#23704=AXIS2_PLACEMENT_3D ( 'NONE', #35908, #27249, #33459 ) ;
#23706=CARTESIAN_POINT ( 'NONE',  ( -85.00000337463092137, -8.660254037844422825, -9.999999999999998224 ) ) ;
#23707=CARTESIAN_POINT ( 'NONE',  ( 54.99999662536844625, -60.62177826491080168, -9.999999999999998224 ) ) ;
#23708=ORIENTED_EDGE ( 'NONE', *, *, #4871, .T. ) ;
#23709=DIRECTION ( 'NONE',  ( 0.000000000000000000, 0.000000000000000000, -1.000000000000000000 ) ) ;
#23712=DIRECTION ( 'NONE',  ( 1.000000000000000000, 0.000000000000000000, 0.000000000000000000 ) ) ;
#23713=AXIS2_PLACEMENT_3D ( 'NONE', #34674, #32195, #34287 ) ;
#23715=AXIS2_PLACEMENT_3D ( 'NONE', #1882, #27738, #13138 ) ;
#23716=AXIS2_PLACEMENT_3D ( 'NONE', #2353, #2148, #25049 ) ;
#23718=CARTESIAN_POINT ( 'NONE',  ( -57.00000337463107059, 43.30127018922197379, -5.000000000000000000 ) ) ;
#23719=CIRCLE ( 'NONE', #7549, 33.00000000000001421 ) ;
#23720=AXIS2_PLACEMENT_3D ( 'NONE', #23855, #15913, #35305 ) ;
#23722=DIRECTION ( 'NONE',  ( 1.000000000000000000, 0.000000000000000000, 0.000000000000000000 ) ) ;
#23723=VERTEX_POINT ( 'NONE', #20108 ) ;
#23724=LINE ( 'NONE', #32143, #19007 ) ;
#23726=CARTESIAN_POINT ( 'NONE',  ( -68.00000337463099243, 51.96152422706637708, 17.49999999999999645 ) ) ;
#23727=CYLINDRICAL_SURFACE ( 'NONE', #15186, 2.000000000000001776 ) ;
#23729=ADVANCED_FACE ( 'NONE', ( #8861 ), #11649, .F. ) ;
#23733=CARTESIAN_POINT ( 'NONE',  ( 64.99999662536842493, 43.30127018922200222, 12.50000000000000000 ) ) ;
#23734=DIRECTION ( 'NONE',  ( 0.000000000000000000, 0.000000000000000000, -1.000000000000000000 ) ) ;
#23735=CIRCLE ( 'NONE', #12931, 65.00000000000000000 ) ;
#23736=LINE ( 'NONE', #1593, #2362 ) ;
#23737=AXIS2_PLACEMENT_3D ( 'NONE', #14614, #362, #31843 ) ;
#23738=DIRECTION ( 'NONE',  ( 0.000000000000000000, 0.000000000000000000, 1.000000000000000000 ) ) ;
#23739=ORIENTED_EDGE ( 'NONE', *, *, #107, .T. ) ;
#23740=ADVANCED_FACE ( 'NONE', ( #14657 ), #3424, .F. ) ;
#23741=DIRECTION ( 'NONE',  ( 1.000000000000000000, 0.000000000000000000, 0.000000000000000000 ) ) ;
#23742=ORIENTED_EDGE ( 'NONE', *, *, #3430, .F. ) ;
#23744=FACE_BOUND ( 'NONE', #6779, .T. ) ;
#23745=CIRCLE ( 'NONE', #12939, 2.000000000000001776 ) ;
#23746=AXIS2_PLACEMENT_3D ( 'NONE', #21190, #30179, #21746 ) ;
#23747=CIRCLE ( 'NONE', #5785, 3.000000000000002665 ) ;
#23748=CIRCLE ( 'NONE', #17166, 33.00000000000001421 ) ;
#23749=DIRECTION ( 'NONE',  ( 0.000000000000000000, 0.000000000000000000, 1.000000000000000000 ) ) ;
#23751=ORIENTED_EDGE ( 'NONE', *, *, #35330, .T. ) ;
#23754=AXIS2_PLACEMENT_3D ( 'NONE', #17887, #23138, #3639 ) ;
#23755=LINE ( 'NONE', #29183, #7500 ) ;
#23756=DIRECTION ( 'NONE',  ( -0.000000000000000000, -0.000000000000000000, -1.000000000000000000 ) ) ;
#23757=DIRECTION ( 'NONE',  ( 1.000000000000000000, 0.000000000000000000, 0.000000000000000000 ) ) ;
#23759=ORIENTED_EDGE ( 'NONE', *, *, #26338, .F. ) ;
#23760=CARTESIAN_POINT ( 'NONE',  ( -20.00000337463122690, 86.60254037844397601, 12.50000000000000000 ) ) ;
#23762=DIRECTION ( 'NONE',  ( 1.000000000000000000, 0.000000000000000000, 0.000000000000000000 ) ) ;
#23763=EDGE_CURVE ( 'NONE', #8255, #2201, #15437, .T. ) ;
#23764=AXIS2_PLACEMENT_3D ( 'NONE', #34749, #26465, #6604 ) ;
#23765=ORIENTED_EDGE ( 'NONE', *, *, #26140, .T. ) ;
#23766=ORIENTED_EDGE ( 'NONE', *, *, #2142, .T. ) ;
#23767=VECTOR ( 'NONE', #16128, 1000.000000000000000 ) ;
#23768=EDGE_LOOP ( 'NONE', ( #36613, #26981, #18595, #19814 ) ) ;
#23769=EDGE_CURVE ( 'NONE', #1092, #13427, #22024, .T. ) ;
#23771=FACE_OUTER_BOUND ( 'NONE', #5703, .T. ) ;
#23772=AXIS2_PLACEMENT_3D ( 'NONE', #7056, #27657, #7419 ) ;
#23775=CARTESIAN_POINT ( 'NONE',  ( -18.00000337463123756, -86.60254037844400443, 17.49999999999999645 ) ) ;
#23776=LINE ( 'NONE', #32956, #13503 ) ;
#23778=ORIENTED_EDGE ( 'NONE', *, *, #11367, .T. ) ;
#23779=AXIS2_PLACEMENT_3D ( 'NONE', #33438, #2656, #27787 ) ;
#23780=VERTEX_POINT ( 'NONE', #24415 ) ;
#23782=DIRECTION ( 'NONE',  ( -1.000000000000000000, 0.000000000000000000, 0.000000000000000000 ) ) ;
#23783=ORIENTED_EDGE ( 'NONE', *, *, #13111, .T. ) ;
#23784=DIRECTION ( 'NONE',  ( 0.000000000000000000, 0.000000000000000000, -1.000000000000000000 ) ) ;
#23785=VERTEX_POINT ( 'NONE', #7343 ) ;
#23786=AXIS2_PLACEMENT_3D ( 'NONE', #1254, #27299, #30304 ) ;
#23787=AXIS2_PLACEMENT_3D ( 'NONE', #18886, #22258, #16437 ) ;
#23788=CIRCLE ( 'NONE', #16003, 2.000000000000001776 ) ;
#23791=FACE_BOUND ( 'NONE', #29518, .T. ) ;
#23793=VERTEX_POINT ( 'NONE', #3775 ) ;
#23796=CIRCLE ( 'NONE', #4012, 2.000000000000001776 ) ;
#23797=ADVANCED_FACE ( 'NONE', ( #30199 ), #15213, .F. ) ;
#23798=CIRCLE ( 'NONE', #11238, 2.000000000000001776 ) ;
#23799=DIRECTION ( 'NONE',  ( 0.000000000000000000, 0.000000000000000000, 1.000000000000000000 ) ) ;
#23800=CARTESIAN_POINT ( 'NONE',  ( -67.00000337463104927, -43.30127018922202353, 17.49999999999999645 ) ) ;
#23802=EDGE_CURVE ( 'NONE', #19362, #12313, #25648, .T. ) ;
#23803=VERTEX_POINT ( 'NONE', #18608 ) ;
#23804=VERTEX_POINT ( 'NONE', #970 ) ;
#23805=CIRCLE ( 'NONE', #34574, 2.000000000000000000 ) ;
#23806=EDGE_LOOP ( 'NONE', ( #9588, #15462 ) ) ;
#23807=VERTEX_POINT ( 'NONE', #30024 ) ;
#23809=DIRECTION ( 'NONE',  ( 0.000000000000000000, 0.000000000000000000, 1.000000000000000000 ) ) ;
#23810=CARTESIAN_POINT ( 'NONE',  ( -52.00000337463109190, 51.96152422706637708, -9.999999999999998224 ) ) ;
#23811=ORIENTED_EDGE ( 'NONE', *, *, #29136, .F. ) ;
#23812=AXIS2_PLACEMENT_3D ( 'NONE', #15322, #21318, #26767 ) ;
#23813=DIRECTION ( 'NONE',  ( 1.000000000000000000, 0.000000000000000000, 0.000000000000000000 ) ) ;
#23817=ORIENTED_EDGE ( 'NONE', *, *, #20903, .F. ) ;
#23819=CIRCLE ( 'NONE', #24409, 2.000000000000001776 ) ;
#23821=EDGE_CURVE ( 'NONE', #30697, #11450, #34027, .T. ) ;
#23822=AXIS2_PLACEMENT_3D ( 'NONE', #27601, #21777, #24982 ) ;
#23825=DIRECTION ( 'NONE',  ( 1.000000000000000000, 0.000000000000000000, 0.000000000000000000 ) ) ;
#23826=DIRECTION ( 'NONE',  ( 0.000000000000000000, 0.000000000000000000, 1.000000000000000000 ) ) ;
#23827=ORIENTED_EDGE ( 'NONE', *, *, #18702, .T. ) ;
#23829=CIRCLE ( 'NONE', #2850, 2.000000000000001776 ) ;
#23831=DIRECTION ( 'NONE',  ( -0.000000000000000000, -0.000000000000000000, 1.000000000000000000 ) ) ;
#23832=FACE_OUTER_BOUND ( 'NONE', #36348, .T. ) ;
#23833=CARTESIAN_POINT ( 'NONE',  ( 64.99999662536841072, -25.98076211353320275, -9.999999999999998224 ) ) ;
#23834=ORIENTED_EDGE ( 'NONE', *, *, #21976, .F. ) ;
#23838=EDGE_CURVE ( 'NONE', #24005, #200, #6474, .T. ) ;
#23839=VECTOR ( 'NONE', #30987, 1000.000000000000000 ) ;
#23840=EDGE_LOOP ( 'NONE', ( #31776, #35853, #14789, #7254, #12633 ) ) ;
#23841=ADVANCED_FACE ( 'NONE', ( #10171 ), #32282, .T. ) ;
#23843=CARTESIAN_POINT ( 'NONE',  ( -53.72397537678465085, -62.16182779291699489, 12.50000000000000000 ) ) ;
#23844=ORIENTED_EDGE ( 'NONE', *, *, #19124, .T. ) ;
#23845=CIRCLE ( 'NONE', #7681, 2.000000000000000000 ) ;
#23846=DIRECTION ( 'NONE',  ( 0.000000000000000000, 0.000000000000000000, 1.000000000000000000 ) ) ;
#23847=ADVANCED_FACE ( 'NONE', ( #1516 ), #33028, .F. ) ;
#23848=DIRECTION ( 'NONE',  ( -1.000000000000000000, 0.000000000000000000, 0.000000000000000000 ) ) ;
#23849=AXIS2_PLACEMENT_3D ( 'NONE', #18790, #30766, #33211 ) ;
#23850=CYLINDRICAL_SURFACE ( 'NONE', #20826, 1.999999999999998224 ) ;
#23851=ORIENTED_EDGE ( 'NONE', *, *, #25666, .T. ) ;
#23852=ORIENTED_EDGE ( 'NONE', *, *, #19716, .F. ) ;
#23853=ADVANCED_FACE ( 'NONE', ( #9773 ), #4172, .F. ) ;
#23854=EDGE_CURVE ( 'NONE', #22239, #13283, #8269, .T. ) ;
#23855=CARTESIAN_POINT ( 'NONE',  ( 64.99999662536841072, -25.98076211353320275, -5.000000000000000000 ) ) ;
#23857=CARTESIAN_POINT ( 'NONE',  ( 83.47442710120355969, -31.09745072740822991, 12.49999999999999645 ) ) ;
#23858=FACE_BOUND ( 'NONE', #33822, .T. ) ;
#23859=DIRECTION ( 'NONE',  ( 1.000000000000000000, 0.000000000000000000, 0.000000000000000000 ) ) ;
#23860=DIRECTION ( 'NONE',  ( -1.000000000000000000, 0.000000000000000000, 0.000000000000000000 ) ) ;
#23861=CIRCLE ( 'NONE', #7698, 2.000000000000001776 ) ;
#23862=CARTESIAN_POINT ( 'NONE',  ( 83.67878100130370456, -27.78182860042797131, -49.86348611802629449 ) ) ;
#23863=EDGE_CURVE ( 'NONE', #35244, #16038, #24437, .T. ) ;
#23864=ORIENTED_EDGE ( 'NONE', *, *, #11293, .F. ) ;
#23865=DIRECTION ( 'NONE',  ( 1.000000000000000000, 0.000000000000000000, 0.000000000000000000 ) ) ;
#23866=EDGE_CURVE ( 'NONE', #21698, #26530, #21429, .T. ) ;
#23867=CARTESIAN_POINT ( 'NONE',  ( 69.99999662536838230, -51.96152422706639840, -5.000000000000000000 ) ) ;
#23868=ADVANCED_FACE ( 'NONE', ( #29842 ), #4731, .T. ) ;
#23869=CIRCLE ( 'NONE', #14894, 2.000000000000001776 ) ;
#23870=CARTESIAN_POINT ( 'NONE',  ( -31.46585318596190106, -86.45172111230344569, -49.86348611802629449 ) ) ;
#23871=EDGE_LOOP ( 'NONE', ( #35096, #33128, #28329, #12535 ) ) ;
#23872=EDGE_CURVE ( 'NONE', #29309, #17608, #10652, .T. ) ;
#23873=DIRECTION ( 'NONE',  ( 0.000000000000000000, 0.000000000000000000, 1.000000000000000000 ) ) ;
#23874=AXIS2_PLACEMENT_3D ( 'NONE', #3373, #31841, #14060 ) ;
#23875=FACE_OUTER_BOUND ( 'NONE', #10989, .T. ) ;
#23876=CARTESIAN_POINT ( 'NONE',  ( 49.99999662536846756, 69.28203230275516944, 17.49999999999999645 ) ) ;
#23877=AXIS2_PLACEMENT_3D ( 'NONE', #2546, #34246, #31230 ) ;
#23878=EDGE_LOOP ( 'NONE', ( #14641, #36566 ) ) ;
#23880=DIRECTION ( 'NONE',  ( -1.000000000000000000, 0.000000000000000000, 0.000000000000000000 ) ) ;
#23881=CARTESIAN_POINT ( 'NONE',  ( 2.999996625368645198, 77.94228634059957983, -9.999999999999998224 ) ) ;
#23883=ORIENTED_EDGE ( 'NONE', *, *, #14543, .F. ) ;
#23884=ORIENTED_EDGE ( 'NONE', *, *, #20595, .F. ) ;
#23885=VERTEX_POINT ( 'NONE', #10717 ) ;
#23886=CIRCLE ( 'NONE', #507, 2.000000000000001776 ) ;
#23887=AXIS2_PLACEMENT_3D ( 'NONE', #13362, #32890, #22196 ) ;
#23888=DIRECTION ( 'NONE',  ( 1.000000000000000000, 0.000000000000000000, 0.000000000000000000 ) ) ;
#23889=EDGE_CURVE ( 'NONE', #1670, #725, #16889, .T. ) ;
#23890=ORIENTED_EDGE ( 'NONE', *, *, #34845, .F. ) ;
#23891=FACE_OUTER_BOUND ( 'NONE', #10754, .T. ) ;
#23893=DIRECTION ( 'NONE',  ( 0.000000000000000000, 0.000000000000000000, 1.000000000000000000 ) ) ;
#23894=ORIENTED_EDGE ( 'NONE', *, *, #25361, .T. ) ;
#23895=VERTEX_POINT ( 'NONE', #33771 ) ;
#23898=VECTOR ( 'NONE', #8218, 1000.000000000000000 ) ;
#23900=ORIENTED_EDGE ( 'NONE', *, *, #22971, .T. ) ;
#23901=ORIENTED_EDGE ( 'NONE', *, *, #16072, .F. ) ;
#23902=EDGE_CURVE ( 'NONE', #30974, #5388, #19710, .T. ) ;
#23905=CARTESIAN_POINT ( 'NONE',  ( 71.99999662536838230, -34.64101615137759183, -5.000000000000000000 ) ) ;
#23908=ORIENTED_EDGE ( 'NONE', *, *, #11553, .T. ) ;
#23910=CARTESIAN_POINT ( 'NONE',  ( 27.99999662536855993, 69.28203230275518365, -9.999999999999998224 ) ) ;
#23911=CIRCLE ( 'NONE', #34087, 2.000000000000001776 ) ;
#23913=DIRECTION ( 'NONE',  ( 1.000000000000000000, 0.000000000000000000, 0.000000000000000000 ) ) ;
#23914=CARTESIAN_POINT ( 'NONE',  ( -68.00000000000000000, 0.000000000000000000, -4.999999999999997335 ) ) ;
#23915=CYLINDRICAL_SURFACE ( 'NONE', #10604, 2.000000000000001776 ) ;
#23916=AXIS2_PLACEMENT_3D ( 'NONE', #13304, #27176, #30571 ) ;
#23917=DIRECTION ( 'NONE',  ( 0.000000000000000000, 0.000000000000000000, 1.000000000000000000 ) ) ;
#23918=EDGE_CURVE ( 'NONE', #35505, #14063, #25035, .T. ) ;
#23919=CIRCLE ( 'NONE', #7746, 33.00000000000001421 ) ;
#23920=DIRECTION ( 'NONE',  ( 0.000000000000000000, 0.000000000000000000, 1.000000000000000000 ) ) ;
#23921=EDGE_CURVE ( 'NONE', #6911, #3619, #26218, .T. ) ;
#23922=EDGE_CURVE ( 'NONE', #3470, #35481, #7063, .T. ) ;
#23924=VERTEX_POINT ( 'NONE', #18972 ) ;
#23925=CARTESIAN_POINT ( 'NONE',  ( 27.78182860042856461, 56.67878100130339902, -4.999999999999997335 ) ) ;
#23926=DIRECTION ( 'NONE',  ( 1.000000000000000000, 0.000000000000000000, 0.000000000000000000 ) ) ;
#23927=DIRECTION ( 'NONE',  ( 0.000000000000000000, 0.000000000000000000, 1.000000000000000000 ) ) ;
#23928=EDGE_LOOP ( 'NONE', ( #14106, #1252, #35931, #14874, #11678, #37072 ) ) ;
#23931=VERTEX_POINT ( 'NONE', #13326 ) ;
#23932=AXIS2_PLACEMENT_3D ( 'NONE', #31630, #6130, #17748 ) ;
#23933=DIRECTION ( 'NONE',  ( 0.000000000000000000, 0.000000000000000000, -1.000000000000000000 ) ) ;
#23934=DIRECTION ( 'NONE',  ( 0.000000000000000000, 0.000000000000000000, 1.000000000000000000 ) ) ;
#23935=AXIS2_PLACEMENT_3D ( 'NONE', #2496, #25201, #36446 ) ;
#23937=DIRECTION ( 'NONE',  ( 0.000000000000000000, 0.000000000000000000, 1.000000000000000000 ) ) ;
#23938=DIRECTION ( 'NONE',  ( 0.000000000000000000, 0.000000000000000000, 1.000000000000000000 ) ) ;
#23939=ORIENTED_EDGE ( 'NONE', *, *, #36946, .T. ) ;
#23940=DIRECTION ( 'NONE',  ( 1.000000000000000000, 0.000000000000000000, 0.000000000000000000 ) ) ;
#23941=ORIENTED_EDGE ( 'NONE', *, *, #34548, .F. ) ;
#23942=FACE_BOUND ( 'NONE', #1994, .T. ) ;
#23943=CIRCLE ( 'NONE', #4780, 2.000000000000001776 ) ;
#23944=EDGE_CURVE ( 'NONE', #23091, #37038, #11827, .T. ) ;
#23945=DIRECTION ( 'NONE',  ( -0.5000000000000098810, -0.8660254037844328234, 0.000000000000000000 ) ) ;
#23947=ORIENTED_EDGE ( 'NONE', *, *, #34294, .F. ) ;
#23949=AXIS2_PLACEMENT_3D ( 'NONE', #1337, #4170, #6605 ) ;
#23951=AXIS2_PLACEMENT_3D ( 'NONE', #8369, #34412, #11891 ) ;
#23952=DIRECTION ( 'NONE',  ( -0.000000000000000000, -0.000000000000000000, 1.000000000000000000 ) ) ;
#23953=CARTESIAN_POINT ( 'NONE',  ( 0.000000000000000000, 0.000000000000000000, -5.000000000000000000 ) ) ;
#23954=ORIENTED_EDGE ( 'NONE', *, *, #11363, .T. ) ;
#23955=DIRECTION ( 'NONE',  ( 1.000000000000000000, 0.000000000000000000, 0.000000000000000000 ) ) ;
#23957=CARTESIAN_POINT ( 'NONE',  ( -17.14523346298279449, 93.36492675454785228, -49.86561046011506448 ) ) ;
#23958=CARTESIAN_POINT ( 'NONE',  ( -18.00000337463124467, 69.28203230275516944, 17.49999999999999645 ) ) ;
#23959=EDGE_LOOP ( 'NONE', ( #1507, #34846, #3247, #25300 ) ) ;
#23960=ORIENTED_EDGE ( 'NONE', *, *, #24770, .T. ) ;
#23961=ADVANCED_FACE ( 'NONE', ( #11066 ), #19170, .F. ) ;
#23962=ORIENTED_EDGE ( 'NONE', *, *, #7456, .T. ) ;
#23963=CARTESIAN_POINT ( 'NONE',  ( -68.66839587347244844, -56.74224907229008608, -4.999999999999997335 ) ) ;
#23964=CARTESIAN_POINT ( 'NONE',  ( -57.00000337463109901, -60.62177826491083010, 17.49999999999999645 ) ) ;
#23966=CARTESIAN_POINT ( 'NONE',  ( 44.99999662536851019, 77.94228634059959404, 17.49999999999999645 ) ) ;
#23967=AXIS2_PLACEMENT_3D ( 'NONE', #32856, #10340, #12764 ) ;
#23968=CARTESIAN_POINT ( 'NONE',  ( 34.99999662536855283, -60.62177826491080168, 12.50000000000000000 ) ) ;
#23969=CARTESIAN_POINT ( 'NONE',  ( -35.19434990244938888, 52.39915983220783602, 12.49999999999999822 ) ) ;
#23971=CARTESIAN_POINT ( 'NONE',  ( -56.67878100130369035, 27.78182860042797131, 12.49999999999999822 ) ) ;
#23972=ORIENTED_EDGE ( 'NONE', *, *, #15391, .T. ) ;
#23973=ORIENTED_EDGE ( 'NONE', *, *, #17801, .F. ) ;
#23975=CIRCLE ( 'NONE', #15593, 2.000000000000001776 ) ;
#23976=DIRECTION ( 'NONE',  ( -1.156482317317870344E-14, -1.000000000000000000, 0.000000000000000000 ) ) ;
#23977=ORIENTED_EDGE ( 'NONE', *, *, #26640, .F. ) ;
#23978=CARTESIAN_POINT ( 'NONE',  ( -4.279621169095561228, 62.97617850287782915, -4.999999999999997335 ) ) ;
#23981=DIRECTION ( 'NONE',  ( 0.000000000000000000, 0.000000000000000000, -1.000000000000000000 ) ) ;
#23982=ORIENTED_EDGE ( 'NONE', *, *, #21655, .F. ) ;
#23983=ORIENTED_EDGE ( 'NONE', *, *, #20884, .T. ) ;
#23985=FACE_OUTER_BOUND ( 'NONE', #28780, .T. ) ;
#23986=ORIENTED_EDGE ( 'NONE', *, *, #5568, .F. ) ;
#23989=EDGE_CURVE ( 'NONE', #20259, #30504, #36593, .T. ) ;
#23991=DIRECTION ( 'NONE',  ( 0.000000000000000000, 0.000000000000000000, 1.000000000000000000 ) ) ;
#23992=AXIS2_PLACEMENT_3D ( 'NONE', #6777, #12592, #36046 ) ;
#23994=EDGE_LOOP ( 'NONE', ( #7922, #11991, #25101, #34803 ) ) ;
#23995=ORIENTED_EDGE ( 'NONE', *, *, #16587, .F. ) ;
#23997=VERTEX_POINT ( 'NONE', #22157 ) ;
#23998=DIRECTION ( 'NONE',  ( 0.000000000000000000, 0.000000000000000000, 1.000000000000000000 ) ) ;
#23999=EDGE_CURVE ( 'NONE', #25033, #12814, #22642, .T. ) ;
#24001=ORIENTED_EDGE ( 'NONE', *, *, #28962, .F. ) ;
#24002=DIRECTION ( 'NONE',  ( 1.000000000000000000, 0.000000000000000000, 0.000000000000000000 ) ) ;
#24003=CARTESIAN_POINT ( 'NONE',  ( 69.99999662536841072, 51.96152422706640550, -5.000000000000000000 ) ) ;
#24004=CARTESIAN_POINT ( 'NONE',  ( -50.00000337463109190, 69.28203230275518365, -5.000000000000000000 ) ) ;
#24005=VERTEX_POINT ( 'NONE', #30945 ) ;
#24006=LINE ( 'NONE', #24371, #23053 ) ;
#24008=DIRECTION ( 'NONE',  ( 1.000000000000000000, 0.000000000000000000, 0.000000000000000000 ) ) ;
#24009=VERTEX_POINT ( 'NONE', #5285 ) ;
#24010=FACE_OUTER_BOUND ( 'NONE', #12826, .T. ) ;
#24012=ORIENTED_EDGE ( 'NONE', *, *, #12961, .T. ) ;
#24013=EDGE_CURVE ( 'NONE', #36949, #30459, #15465, .T. ) ;
#24014=ORIENTED_EDGE ( 'NONE', *, *, #22255, .T. ) ;
#24015=DIRECTION ( 'NONE',  ( 0.000000000000000000, 0.000000000000000000, 1.000000000000000000 ) ) ;
#24016=EDGE_CURVE ( 'NONE', #26329, #8382, #24611, .T. ) ;
#24017=DIRECTION ( 'NONE',  ( 0.4999999999999924505, -0.8660254037844429265, 0.000000000000000000 ) ) ;
#24018=VECTOR ( 'NONE', #35274, 1000.000000000000000 ) ;
#24020=DIRECTION ( 'NONE',  ( 0.000000000000000000, 0.000000000000000000, 1.000000000000000000 ) ) ;
#24021=ORIENTED_EDGE ( 'NONE', *, *, #33614, .T. ) ;
#24022=EDGE_CURVE ( 'NONE', #22555, #27665, #22082, .T. ) ;
#24026=EDGE_CURVE ( 'NONE', #29140, #36953, #16672, .T. ) ;
#24027=CARTESIAN_POINT ( 'NONE',  ( 17.14523346298344109, -93.36492675454773860, 12.49999999999999822 ) ) ;
#24028=ORIENTED_EDGE ( 'NONE', *, *, #3610, .T. ) ;
#24029=DIRECTION ( 'NONE',  ( -0.000000000000000000, -0.000000000000000000, 1.000000000000000000 ) ) ;
#24030=CARTESIAN_POINT ( 'NONE',  ( -85.00000337463092137, -8.660254037844422825, -9.999999999999998224 ) ) ;
#24031=EDGE_CURVE ( 'NONE', #29299, #29323, #35842, .T. ) ;
#24032=DIRECTION ( 'NONE',  ( 0.000000000000000000, 0.000000000000000000, 1.000000000000000000 ) ) ;
#24034=ORIENTED_EDGE ( 'NONE', *, *, #34380, .F. ) ;
#24035=AXIS2_PLACEMENT_3D ( 'NONE', #2995, #11235, #29358 ) ;
#24036=ORIENTED_EDGE ( 'NONE', *, *, #5221, .T. ) ;
#24039=DIRECTION ( 'NONE',  ( 0.000000000000000000, 0.000000000000000000, 1.000000000000000000 ) ) ;
#24040=DIRECTION ( 'NONE',  ( -0.000000000000000000, -0.000000000000000000, 1.000000000000000000 ) ) ;
#24041=DIRECTION ( 'NONE',  ( 0.000000000000000000, 0.000000000000000000, 1.000000000000000000 ) ) ;
#24042=ORIENTED_EDGE ( 'NONE', *, *, #16979, .F. ) ;
#24043=CARTESIAN_POINT ( 'NONE',  ( 71.99999662536839651, -17.32050807568879947, -9.999999999999998224 ) ) ;
#24044=EDGE_CURVE ( 'NONE', #34902, #12512, #20256, .T. ) ;
#24045=DIRECTION ( 'NONE',  ( 0.000000000000000000, 0.000000000000000000, 1.000000000000000000 ) ) ;
#24046=CARTESIAN_POINT ( 'NONE',  ( -45.00000337463111322, -77.94228634059960825, -9.999999999999998224 ) ) ;
#24049=CARTESIAN_POINT ( 'NONE',  ( -70.00000337463099243, 17.32050807568877460, -9.999999999999998224 ) ) ;
#24050=DIRECTION ( 'NONE',  ( -1.000000000000000000, 0.000000000000000000, 0.000000000000000000 ) ) ;
#24051=LINE ( 'NONE', #21219, #3031 ) ;
#24053=EDGE_CURVE ( 'NONE', #25880, #15915, #32226, .T. ) ;
#24054=ORIENTED_EDGE ( 'NONE', *, *, #673, .F. ) ;
#24055=AXIS2_PLACEMENT_3D ( 'NONE', #13000, #819, #4014 ) ;
#24056=EDGE_CURVE ( 'NONE', #35643, #7161, #20248, .T. ) ;
#24057=CARTESIAN_POINT ( 'NONE',  ( 64.99999662536841072, 25.98076211353318854, -9.999999999999998224 ) ) ;
#24058=FACE_OUTER_BOUND ( 'NONE', #19902, .T. ) ;
#24062=ORIENTED_EDGE ( 'NONE', *, *, #12802, .F. ) ;
#24063=VERTEX_POINT ( 'NONE', #11603 ) ;
#24064=DIRECTION ( 'NONE',  ( -1.000000000000000000, 1.798972493605577187E-15, 0.000000000000000000 ) ) ;
#24065=VERTEX_POINT ( 'NONE', #2831 ) ;
#24066=ORIENTED_EDGE ( 'NONE', *, *, #21492, .F. ) ;
#24067=CARTESIAN_POINT ( 'NONE',  ( 56.99999662536844625, 43.30127018922198801, -9.999999999999998224 ) ) ;
#24068=ORIENTED_EDGE ( 'NONE', *, *, #8535, .F. ) ;
#24070=CARTESIAN_POINT ( 'NONE',  ( -52.00000337463109190, 69.28203230275518365, -9.999999999999998224 ) ) ;
#24071=EDGE_CURVE ( 'NONE', #32385, #15477, #4089, .T. ) ;
#24072=CARTESIAN_POINT ( 'NONE',  ( 51.99999662536847467, 51.96152422706637708, -9.999999999999998224 ) ) ;
#24073=EDGE_LOOP ( 'NONE', ( #2952, #32748, #9887, #14039, #8701 ) ) ;
#24075=LINE ( 'NONE', #32683, #34080 ) ;
#24077=DIRECTION ( 'NONE',  ( 0.000000000000000000, 0.000000000000000000, 1.000000000000000000 ) ) ;
#24078=LINE ( 'NONE', #32499, #28052 ) ;
#24081=AXIS2_PLACEMENT_3D ( 'NONE', #37006, #26104, #31537 ) ;
#24082=ORIENTED_EDGE ( 'NONE', *, *, #19470, .T. ) ;
#24083=DIRECTION ( 'NONE',  ( -0.000000000000000000, -0.000000000000000000, 1.000000000000000000 ) ) ;
#24084=CARTESIAN_POINT ( 'NONE',  ( -82.00000337463094979, 34.64101615137757051, 12.50000000000000000 ) ) ;
#24085=DIRECTION ( 'NONE',  ( 1.000000000000000000, 0.000000000000000000, 0.000000000000000000 ) ) ;
#24087=EDGE_CURVE ( 'NONE', #35523, #29052, #33456, .T. ) ;
#24088=CARTESIAN_POINT ( 'NONE',  ( -3.374631327851540519E-06, 86.60254037844397601, 12.50000000000000000 ) ) ;
#24089=DIRECTION ( 'NONE',  ( 0.000000000000000000, 0.000000000000000000, 1.000000000000000000 ) ) ;
#24090=EDGE_LOOP ( 'NONE', ( #20332, #10153, #30478 ) ) ;
#24091=EDGE_CURVE ( 'NONE', #23264, #1584, #17864, .T. ) ;
#24092=DIRECTION ( 'NONE',  ( -0.000000000000000000, -0.000000000000000000, 1.000000000000000000 ) ) ;
#24093=CARTESIAN_POINT ( 'NONE',  ( -50.00000337463112032, -51.96152422706641971, 12.50000000000000000 ) ) ;
#24094=CARTESIAN_POINT ( 'NONE',  ( 66.50937412064257614, -41.98910420248104458, 12.50000000000000000 ) ) ;
#24095=ORIENTED_EDGE ( 'NONE', *, *, #20614, .F. ) ;
#24096=ADVANCED_FACE ( 'NONE', ( #9167 ), #11794, .F. ) ;
#24097=AXIS2_PLACEMENT_3D ( 'NONE', #30038, #4192, #15431 ) ;
#24098=EDGE_LOOP ( 'NONE', ( #23611, #5450, #35612, #24839 ) ) ;
#24100=CARTESIAN_POINT ( 'NONE',  ( -10.00000337463128730, 69.28203230275516944, 12.50000000000000000 ) ) ;
#24101=CARTESIAN_POINT ( 'NONE',  ( 43.19957991610432657, 47.04203867989531318, 12.49999999999999822 ) ) ;
#24102=DIRECTION ( 'NONE',  ( 0.000000000000000000, 0.000000000000000000, -1.000000000000000000 ) ) ;
#24103=ADVANCED_FACE ( 'NONE', ( #17605 ), #3182, .F. ) ;
#24104=CARTESIAN_POINT ( 'NONE',  ( -60.00000337463107059, -34.64101615137762025, 17.49999999999999645 ) ) ;
#24107=AXIS2_PLACEMENT_3D ( 'NONE', #13885, #33772, #5463 ) ;
#24108=DIRECTION ( 'NONE',  ( 0.000000000000000000, 0.000000000000000000, 1.000000000000000000 ) ) ;
#24109=EDGE_LOOP ( 'NONE', ( #17395, #16833 ) ) ;
#24110=DIRECTION ( 'NONE',  ( 0.000000000000000000, 0.000000000000000000, 1.000000000000000000 ) ) ;
#24111=EDGE_LOOP ( 'NONE', ( #18139, #1036 ) ) ;
#24112=CARTESIAN_POINT ( 'NONE',  ( -75.00000337463097821, 8.660254037844374864, -9.999999999999998224 ) ) ;
#24113=EDGE_CURVE ( 'NONE', #7182, #9631, #14288, .T. ) ;
#24114=EDGE_CURVE ( 'NONE', #3735, #1626, #5889, .T. ) ;
#24115=DIRECTION ( 'NONE',  ( 0.000000000000000000, 0.000000000000000000, 1.000000000000000000 ) ) ;
#24116=DIRECTION ( 'NONE',  ( 0.000000000000000000, 0.000000000000000000, -1.000000000000000000 ) ) ;
#24117=EDGE_CURVE ( 'NONE', #3385, #30697, #17290, .T. ) ;
#24121=CARTESIAN_POINT ( 'NONE',  ( 4.999996625368645198, 77.94228634059957983, 12.50000000000000000 ) ) ;
#24122=DIRECTION ( 'NONE',  ( 0.000000000000000000, 0.000000000000000000, -1.000000000000000000 ) ) ;
#24123=AXIS2_PLACEMENT_3D ( 'NONE', #12926, #35463, #32617 ) ;
#24124=CARTESIAN_POINT ( 'NONE',  ( 74.99999662536836809, 43.30127018922198801, -9.999999999999998224 ) ) ;
#24125=CARTESIAN_POINT ( 'NONE',  ( -58.88972745734203329, -33.99999999999965894, 12.49999999999999822 ) ) ;
#24126=ORIENTED_EDGE ( 'NONE', *, *, #4095, .T. ) ;
#24128=CARTESIAN_POINT ( 'NONE',  ( 29.99999662536857770, -69.28203230275519786, 12.50000000000000000 ) ) ;
#24129=CARTESIAN_POINT ( 'NONE',  ( 51.99999662536847467, -69.28203230275519786, -9.999999999999998224 ) ) ;
#24130=ORIENTED_EDGE ( 'NONE', *, *, #8137, .T. ) ;
#24131=ORIENTED_EDGE ( 'NONE', *, *, #17408, .F. ) ;
#24133=ORIENTED_EDGE ( 'NONE', *, *, #2321, .F. ) ;
#24134=CIRCLE ( 'NONE', #753, 2.000000000000001776 ) ;
#24135=DIRECTION ( 'NONE',  ( 0.000000000000000000, -0.000000000000000000, -1.000000000000000000 ) ) ;
#24136=CARTESIAN_POINT ( 'NONE',  ( 60.93295298011005201, 19.13981058454729123, 12.49999999999999822 ) ) ;
#24137=DIRECTION ( 'NONE',  ( -1.000000000000000000, 0.000000000000000000, 0.000000000000000000 ) ) ;
#24138=DIRECTION ( 'NONE',  ( 1.000000000000000000, 0.000000000000000000, 0.000000000000000000 ) ) ;
#24139=CARTESIAN_POINT ( 'NONE',  ( -62.00000337463107769, -34.64101615137762025, -9.999999999999998224 ) ) ;
#24141=VERTEX_POINT ( 'NONE', #28497 ) ;
#24142=EDGE_LOOP ( 'NONE', ( #17880, #32500, #11509, #20864 ) ) ;
#24143=PLANE ( 'NONE',  #13506 ) ;
#24144=DIRECTION ( 'NONE',  ( 0.000000000000000000, 0.000000000000000000, 1.000000000000000000 ) ) ;
#24146=FACE_OUTER_BOUND ( 'NONE', #18713, .T. ) ;
#24147=ORIENTED_EDGE ( 'NONE', *, *, #33958, .T. ) ;
#24149=FACE_BOUND ( 'NONE', #33885, .T. ) ;
#24150=ORIENTED_EDGE ( 'NONE', *, *, #8159, .F. ) ;
#24153=EDGE_CURVE ( 'NONE', #26082, #21989, #8623, .T. ) ;
#24155=EDGE_LOOP ( 'NONE', ( #25232, #20048 ) ) ;
#24158=DIRECTION ( 'NONE',  ( 0.000000000000000000, 0.000000000000000000, -1.000000000000000000 ) ) ;
#24159=CARTESIAN_POINT ( 'NONE',  ( 13.89091430021463935, 62.33939050065170306, 12.49999999999999822 ) ) ;
#24160=DIRECTION ( 'NONE',  ( 0.000000000000000000, 0.000000000000000000, -1.000000000000000000 ) ) ;
#24161=ORIENTED_EDGE ( 'NONE', *, *, #24997, .T. ) ;
#24162=VECTOR ( 'NONE', #34722, 1000.000000000000000 ) ;
#24163=ORIENTED_EDGE ( 'NONE', *, *, #2414, .T. ) ;
#24165=CIRCLE ( 'NONE', #27746, 1.999999999999998224 ) ;
#24167=DIRECTION ( 'NONE',  ( 1.000000000000000000, 0.000000000000000000, 0.000000000000000000 ) ) ;
#24168=DIRECTION ( 'NONE',  ( 1.000000000000000000, 0.000000000000000000, 0.000000000000000000 ) ) ;
#24169=VERTEX_POINT ( 'NONE', #20057 ) ;
#24171=FACE_OUTER_BOUND ( 'NONE', #30093, .T. ) ;
#24172=EDGE_CURVE ( 'NONE', #26391, #12033, #8874, .T. ) ;
#24173=ORIENTED_EDGE ( 'NONE', *, *, #33724, .F. ) ;
#24174=DIRECTION ( 'NONE',  ( 1.000000000000000000, 0.000000000000000000, 0.000000000000000000 ) ) ;
#24176=AXIS2_PLACEMENT_3D ( 'NONE', #3856, #32371, #35941 ) ;
#24177=DIRECTION ( 'NONE',  ( 0.000000000000000000, 0.000000000000000000, 1.000000000000000000 ) ) ;
#24178=AXIS2_PLACEMENT_3D ( 'NONE', #17073, #16727, #25338 ) ;
#24179=DIRECTION ( 'NONE',  ( 0.000000000000000000, 0.000000000000000000, -1.000000000000000000 ) ) ;
#24181=CARTESIAN_POINT ( 'NONE',  ( 42.99999662536850309, 77.94228634059959404, -9.999999999999998224 ) ) ;
#24182=CIRCLE ( 'NONE', #30143, 2.000000000000001776 ) ;
#24183=ORIENTED_EDGE ( 'NONE', *, *, #5637, .T. ) ;
#24184=ORIENTED_EDGE ( 'NONE', *, *, #1295, .F. ) ;
#24185=EDGE_CURVE ( 'NONE', #15311, #4442, #28646, .T. ) ;
#24187=DIRECTION ( 'NONE',  ( 1.000000000000000000, 0.000000000000000000, 0.000000000000000000 ) ) ;
#24188=DIRECTION ( 'NONE',  ( -1.000000000000000000, 0.000000000000000000, 0.000000000000000000 ) ) ;
#24189=DIRECTION ( 'NONE',  ( 0.000000000000000000, 0.000000000000000000, 1.000000000000000000 ) ) ;
#24190=ORIENTED_EDGE ( 'NONE', *, *, #2974, .F. ) ;
#24191=CARTESIAN_POINT ( 'NONE',  ( -20.00000337463124112, 69.28203230275516944, 12.50000000000000000 ) ) ;
#24193=AXIS2_PLACEMENT_3D ( 'NONE', #11568, #23021, #9526 ) ;
#24194=ORIENTED_EDGE ( 'NONE', *, *, #15768, .F. ) ;
#24195=ADVANCED_FACE ( 'NONE', ( #34505 ), #8813, .F. ) ;
#24196=CARTESIAN_POINT ( 'NONE',  ( 0.000000000000000000, 0.000000000000000000, -5.000000000000000000 ) ) ;
#24197=ORIENTED_EDGE ( 'NONE', *, *, #33329, .F. ) ;
#24198=CARTESIAN_POINT ( 'NONE',  ( -75.00000337463097821, 25.98076211353318854, -5.000000000000000000 ) ) ;
#24200=DIRECTION ( 'NONE',  ( 0.000000000000000000, 0.000000000000000000, 1.000000000000000000 ) ) ;
#24202=DIRECTION ( 'NONE',  ( 0.000000000000000000, 0.000000000000000000, 1.000000000000000000 ) ) ;
#24203=ORIENTED_EDGE ( 'NONE', *, *, #25459, .F. ) ;
#24204=ORIENTED_EDGE ( 'NONE', *, *, #22365, .T. ) ;
#24205=ORIENTED_EDGE ( 'NONE', *, *, #25717, .T. ) ;
#24208=CARTESIAN_POINT ( 'NONE',  ( -12.97563234535667753, 90.60231327712331506, -49.86561046011506448 ) ) ;
#24209=AXIS2_PLACEMENT_3D ( 'NONE', #12340, #23998, #15170 ) ;
#24210=DIRECTION ( 'NONE',  ( 1.000000000000000000, 0.000000000000000000, 0.000000000000000000 ) ) ;
#24211=DIRECTION ( 'NONE',  ( -0.4999999999999979461, 0.8660254037844397068, 0.000000000000000000 ) ) ;
#24212=DIRECTION ( 'NONE',  ( 0.000000000000000000, 0.000000000000000000, 1.000000000000000000 ) ) ;
#24213=ORIENTED_EDGE ( 'NONE', *, *, #15291, .F. ) ;
#24214=DIRECTION ( 'NONE',  ( -1.000000000000000000, 0.000000000000000000, 0.000000000000000000 ) ) ;
#24215=VECTOR ( 'NONE', #10984, 1000.000000000000000 ) ;
#24216=DIRECTION ( 'NONE',  ( 0.000000000000000000, 0.000000000000000000, 1.000000000000000000 ) ) ;
#24217=ORIENTED_EDGE ( 'NONE', *, *, #17644, .F. ) ;
#24218=DIRECTION ( 'NONE',  ( 0.000000000000000000, 0.000000000000000000, 1.000000000000000000 ) ) ;
#24220=CYLINDRICAL_SURFACE ( 'NONE', #32729, 2.000000000000001776 ) ;
#24221=AXIS2_PLACEMENT_3D ( 'NONE', #10110, #26788, #27144 ) ;
#24222=ORIENTED_EDGE ( 'NONE', *, *, #12880, .T. ) ;
#24223=CIRCLE ( 'NONE', #12837, 95.00000000000000000 ) ;
#24225=EDGE_CURVE ( 'NONE', #35478, #17057, #35448, .T. ) ;
#24226=CARTESIAN_POINT ( 'NONE',  ( 35.83991598322140248, 56.52018970185221036, -4.999999999999997335 ) ) ;
#24228=LINE ( 'NONE', #1186, #21423 ) ;
#24230=VERTEX_POINT ( 'NONE', #15003 ) ;
#24231=VERTEX_POINT ( 'NONE', #32599 ) ;
#24233=AXIS2_PLACEMENT_3D ( 'NONE', #26058, #23061, #31845 ) ;
#24236=EDGE_LOOP ( 'NONE', ( #20723, #36071, #18432, #31433 ) ) ;
#24238=VERTEX_POINT ( 'NONE', #9733 ) ;
#24239=ORIENTED_EDGE ( 'NONE', *, *, #27473, .F. ) ;
#24240=VECTOR ( 'NONE', #7692, 1000.000000000000000 ) ;
#24241=EDGE_CURVE ( 'NONE', #28829, #24245, #13071, .T. ) ;
#24244=ORIENTED_EDGE ( 'NONE', *, *, #23154, .F. ) ;
#24245=VERTEX_POINT ( 'NONE', #18368 ) ;
#24246=FACE_OUTER_BOUND ( 'NONE', #24274, .T. ) ;
#24247=DIRECTION ( 'NONE',  ( 0.000000000000000000, 0.000000000000000000, -1.000000000000000000 ) ) ;
#24248=AXIS2_PLACEMENT_3D ( 'NONE', #29539, #1060, #7065 ) ;
#24250=FACE_OUTER_BOUND ( 'NONE', #36197, .T. ) ;
#24252=DIRECTION ( 'NONE',  ( 0.000000000000000000, 0.000000000000000000, 1.000000000000000000 ) ) ;
#24253=EDGE_LOOP ( 'NONE', ( #31068, #8767, #6845, #26169 ) ) ;
#24254=CARTESIAN_POINT ( 'NONE',  ( 56.67878100130369035, -27.78182860042797131, -4.999999999999997335 ) ) ;
#24255=EDGE_CURVE ( 'NONE', #1094, #30126, #2922, .T. ) ;
#24259=DIRECTION ( 'NONE',  ( 0.000000000000000000, 0.000000000000000000, 1.000000000000000000 ) ) ;
#24260=DIRECTION ( 'NONE',  ( 1.000000000000000000, 0.000000000000000000, 0.000000000000000000 ) ) ;
#24262=CARTESIAN_POINT ( 'NONE',  ( 69.99999662536839651, 17.32050807568879236, -9.999999999999998224 ) ) ;
#24265=EDGE_LOOP ( 'NONE', ( #18548, #33827, #11680 ) ) ;
#24266=DIRECTION ( 'NONE',  ( -1.000000000000000000, 0.000000000000000000, 0.000000000000000000 ) ) ;
#24268=CARTESIAN_POINT ( 'NONE',  ( -10.00000337463127842, -69.28203230275519786, -9.999999999999998224 ) ) ;
#24269=DIRECTION ( 'NONE',  ( 0.000000000000000000, 0.000000000000000000, 1.000000000000000000 ) ) ;
#24271=VERTEX_POINT ( 'NONE', #1299 ) ;
#24272=CIRCLE ( 'NONE', #8110, 2.000000000000001776 ) ;
#24273=ORIENTED_EDGE ( 'NONE', *, *, #21115, .T. ) ;
#24274=EDGE_LOOP ( 'NONE', ( #5198, #5948, #33764, #27201 ) ) ;
#24275=ADVANCED_FACE ( 'NONE', ( #4127 ), #15364, .T. ) ;
#24277=CARTESIAN_POINT ( 'NONE',  ( 87.99999662536828282, 2.449293598294703949E-16, -5.000000000000000000 ) ) ;
#24278=CARTESIAN_POINT ( 'NONE',  ( -2.000003374631303732, -86.60254037844400443, 12.50000000000000000 ) ) ;
#24279=ORIENTED_EDGE ( 'NONE', *, *, #28921, .T. ) ;
#24280=AXIS2_PLACEMENT_3D ( 'NONE', #6492, #6289, #20528 ) ;
#24281=AXIS2_PLACEMENT_3D ( 'NONE', #21514, #12681, #3707 ) ;
#24284=VERTEX_POINT ( 'NONE', #17996 ) ;
#24285=DIRECTION ( 'NONE',  ( -0.000000000000000000, -0.000000000000000000, -1.000000000000000000 ) ) ;
#24286=VERTEX_POINT ( 'NONE', #29422 ) ;
#24287=DIRECTION ( 'NONE',  ( -1.000000000000000000, 0.000000000000000000, 0.000000000000000000 ) ) ;
#24288=EDGE_CURVE ( 'NONE', #11378, #25226, #24465, .T. ) ;
#24291=CIRCLE ( 'NONE', #15319, 2.000000000000001776 ) ;
#24292=CARTESIAN_POINT ( 'NONE',  ( 87.99999662536828282, 2.449293598294706414E-16, -9.999999999999998224 ) ) ;
#24293=ADVANCED_FACE ( 'NONE', ( #26987 ), #12546, .F. ) ;
#24295=ORIENTED_EDGE ( 'NONE', *, *, #11380, .F. ) ;
#24297=CIRCLE ( 'NONE', #22502, 2.000000000000001776 ) ;
#24298=AXIS2_PLACEMENT_3D ( 'NONE', #10313, #19150, #7503 ) ;
#24300=CIRCLE ( 'NONE', #18301, 2.000000000000001776 ) ;
#24301=EDGE_CURVE ( 'NONE', #17303, #32102, #29231, .T. ) ;
#24304=DIRECTION ( 'NONE',  ( 1.000000000000000000, 0.000000000000000000, 0.000000000000000000 ) ) ;
#24306=ORIENTED_EDGE ( 'NONE', *, *, #27886, .F. ) ;
#24307=CARTESIAN_POINT ( 'NONE',  ( 64.99999662536842493, 43.30127018922200222, 17.49999999999999645 ) ) ;
#24308=EDGE_CURVE ( 'NONE', #15434, #26833, #21458, .T. ) ;
#24311=EDGE_CURVE ( 'NONE', #5101, #10635, #27450, .T. ) ;
#24312=VECTOR ( 'NONE', #18544, 1000.000000000000000 ) ;
#24313=VERTEX_POINT ( 'NONE', #23554 ) ;
#24314=ORIENTED_EDGE ( 'NONE', *, *, #33872, .T. ) ;
#24316=PLANE ( 'NONE',  #24960 ) ;
#24319=EDGE_CURVE ( 'NONE', #29609, #5247, #11738, .T. ) ;
#24320=CARTESIAN_POINT ( 'NONE',  ( 7.999996625368618552, 69.28203230275516944, -9.999999999999998224 ) ) ;
#24321=ORIENTED_EDGE ( 'NONE', *, *, #8853, .F. ) ;
#24322=ADVANCED_FACE ( 'NONE', ( #12091, #11549, #34269, #17943, #34448, #20731, #20193 ), #28629, .F. ) ;
#24323=CIRCLE ( 'NONE', #15345, 2.000000000000001776 ) ;
#24324=EDGE_CURVE ( 'NONE', #25888, #4290, #28674, .T. ) ;
#24325=FACE_OUTER_BOUND ( 'NONE', #14664, .T. ) ;
#24327=ADVANCED_FACE ( 'NONE', ( #26191 ), #32168, .F. ) ;
#24333=VERTEX_POINT ( 'NONE', #23197 ) ;
#24336=CARTESIAN_POINT ( 'NONE',  ( 69.99999662536839651, -17.32050807568879947, 12.50000000000000000 ) ) ;
#24337=AXIS2_PLACEMENT_3D ( 'NONE', #1856, #28094, #5419 ) ;
#24338=CARTESIAN_POINT ( 'NONE',  ( -52.00000337463112032, -51.96152422706641971, -9.999999999999998224 ) ) ;
#24339=VERTEX_POINT ( 'NONE', #6504 ) ;
#24340=DIRECTION ( 'NONE',  ( 1.000000000000000000, 0.000000000000000000, 0.000000000000000000 ) ) ;
#24342=CARTESIAN_POINT ( 'NONE',  ( -87.00000337463093558, -25.98076211353322051, -9.999999999999998224 ) ) ;
#24343=AXIS2_PLACEMENT_3D ( 'NONE', #25233, #2529, #13952 ) ;
#24344=DIRECTION ( 'NONE',  ( 0.000000000000000000, 0.000000000000000000, 1.000000000000000000 ) ) ;
#24346=ORIENTED_EDGE ( 'NONE', *, *, #35075, .T. ) ;
#24347=CARTESIAN_POINT ( 'NONE',  ( 0.000000000000000000, 0.000000000000000000, -5.000000000000000000 ) ) ;
#24349=AXIS2_PLACEMENT_3D ( 'NONE', #15210, #35106, #3772 ) ;
#24350=DIRECTION ( 'NONE',  ( 0.5000000000000039968, 0.8660254037844363761, 0.000000000000000000 ) ) ;
#24351=AXIS2_PLACEMENT_3D ( 'NONE', #4129, #24740, #26989 ) ;
#24353=CARTESIAN_POINT ( 'NONE',  ( -67.00000337463104927, -25.98076211353322051, -9.999999999999998224 ) ) ;
#24355=PLANE ( 'NONE',  #26236 ) ;
#24357=CARTESIAN_POINT ( 'NONE',  ( 2.778182860043481028, 66.86787810013034061, 12.49999999999999822 ) ) ;
#24361=CIRCLE ( 'NONE', #33949, 2.000000000000000000 ) ;
#24362=ORIENTED_EDGE ( 'NONE', *, *, #20307, .T. ) ;
#24363=CIRCLE ( 'NONE', #12338, 2.000000000000001776 ) ;
#24364=ORIENTED_EDGE ( 'NONE', *, *, #16458, .T. ) ;
#24365=LINE ( 'NONE', #18365, #14034 ) ;
#24367=ORIENTED_EDGE ( 'NONE', *, *, #10591, .F. ) ;
#24368=DIRECTION ( 'NONE',  ( -1.000000000000000000, 0.000000000000000000, -0.000000000000000000 ) ) ;
#24369=DIRECTION ( 'NONE',  ( 0.000000000000000000, 0.000000000000000000, -1.000000000000000000 ) ) ;
#24371=CARTESIAN_POINT ( 'NONE',  ( -2.000003374631334818, 69.28203230275516944, -9.999999999999998224 ) ) ;
#24372=AXIS2_PLACEMENT_3D ( 'NONE', #8105, #30981, #5313 ) ;
#24373=EDGE_CURVE ( 'NONE', #14204, #33302, #18498, .T. ) ;
#24374=LINE ( 'NONE', #35825, #20412 ) ;
#24375=EDGE_CURVE ( 'NONE', #23282, #11624, #1141, .T. ) ;
#24377=CARTESIAN_POINT ( 'NONE',  ( -82.00000337463096400, -34.64101615137762025, -9.999999999999998224 ) ) ;
#24381=VERTEX_POINT ( 'NONE', #28805 ) ;
#24382=CIRCLE ( 'NONE', #12987, 2.000000000000001776 ) ;
#24383=ORIENTED_EDGE ( 'NONE', *, *, #3953, .T. ) ;
#24384=DIRECTION ( 'NONE',  ( 1.000000000000000000, 0.000000000000000000, 0.000000000000000000 ) ) ;
#24387=CARTESIAN_POINT ( 'NONE',  ( 66.99999662536839651, -43.30127018922199511, 12.50000000000000000 ) ) ;
#24389=DIRECTION ( 'NONE',  ( -1.000000000000000000, 0.000000000000000000, 0.000000000000000000 ) ) ;
#24390=EDGE_CURVE ( 'NONE', #12599, #20765, #29746, .T. ) ;
#24391=VERTEX_POINT ( 'NONE', #5957 ) ;
#24392=VECTOR ( 'NONE', #2711, 1000.000000000000000 ) ;
#24393=CARTESIAN_POINT ( 'NONE',  ( 62.99999662536841072, 25.98076211353318854, -9.999999999999998224 ) ) ;
#24394=AXIS2_PLACEMENT_3D ( 'NONE', #12725, #9744, #7135 ) ;
#24395=DIRECTION ( 'NONE',  ( 0.000000000000000000, 0.000000000000000000, 1.000000000000000000 ) ) ;
#24396=AXIS2_PLACEMENT_3D ( 'NONE', #22810, #28950, #14163 ) ;
#24397=ORIENTED_EDGE ( 'NONE', *, *, #24044, .T. ) ;
#24400=CIRCLE ( 'NONE', #27388, 2.000000000000001776 ) ;
#24401=ADVANCED_FACE ( 'NONE', ( #11926 ), #17389, .F. ) ;
#24402=FACE_OUTER_BOUND ( 'NONE', #28676, .T. ) ;
#24404=CARTESIAN_POINT ( 'NONE',  ( 67.99999662536836809, -34.64101615137759183, 12.50000000000000000 ) ) ;
#24407=ORIENTED_EDGE ( 'NONE', *, *, #10744, .F. ) ;
#24408=AXIS2_PLACEMENT_3D ( 'NONE', #10931, #22202, #19376 ) ;
#24409=AXIS2_PLACEMENT_3D ( 'NONE', #17647, #213, #34745 ) ;
#24412=VERTEX_POINT ( 'NONE', #17741 ) ;
#24414=FACE_BOUND ( 'NONE', #17304, .T. ) ;
#24415=CARTESIAN_POINT ( 'NONE',  ( -52.00000337463109190, 69.28203230275518365, 17.49999999999999645 ) ) ;
#24416=CARTESIAN_POINT ( 'NONE',  ( -83.67710216016716629, 27.48073957228723430, 12.50000000000000000 ) ) ;
#24418=EDGE_LOOP ( 'NONE', ( #1565, #4895 ) ) ;
#24420=AXIS2_PLACEMENT_3D ( 'NONE', #29673, #12618, #17891 ) ;
#24421=CARTESIAN_POINT ( 'NONE',  ( -62.97617850287781494, -4.279621169095772615, 12.49999999999999822 ) ) ;
#24422=EDGE_CURVE ( 'NONE', #4180, #14960, #26863, .T. ) ;
#24424=ORIENTED_EDGE ( 'NONE', *, *, #35551, .T. ) ;
#24425=DIRECTION ( 'NONE',  ( -0.8660254037844380415, 0.5000000000000009992, 0.000000000000000000 ) ) ;
#24427=AXIS2_PLACEMENT_3D ( 'NONE', #25804, #26155, #12239 ) ;
#24428=VERTEX_POINT ( 'NONE', #3513 ) ;
#24429=ORIENTED_EDGE ( 'NONE', *, *, #35048, .T. ) ;
#24430=AXIS2_PLACEMENT_3D ( 'NONE', #34582, #17495, #26673 ) ;
#24431=DIRECTION ( 'NONE',  ( -1.000000000000000000, 0.000000000000000000, -0.000000000000000000 ) ) ;
#24432=LINE ( 'NONE', #35872, #25376 ) ;
#24434=EDGE_LOOP ( 'NONE', ( #6785, #701, #29322, #22501 ) ) ;
#24435=ORIENTED_EDGE ( 'NONE', *, *, #12113, .T. ) ;
#24436=AXIS2_PLACEMENT_3D ( 'NONE', #13985, #13821, #2392 ) ;
#24437=CIRCLE ( 'NONE', #1057, 2.000000000000001776 ) ;
#24438=ORIENTED_EDGE ( 'NONE', *, *, #137, .F. ) ;
#24439=VECTOR ( 'NONE', #35576, 1000.000000000000000 ) ;
#24440=DIRECTION ( 'NONE',  ( 1.000000000000000000, 0.000000000000000000, 0.000000000000000000 ) ) ;
#24441=CIRCLE ( 'NONE', #8274, 2.000000000000001776 ) ;
#24442=ORIENTED_EDGE ( 'NONE', *, *, #33140, .F. ) ;
#24443=EDGE_CURVE ( 'NONE', #19786, #11022, #26376, .T. ) ;
#24444=VERTEX_POINT ( 'NONE', #3466 ) ;
#24446=ORIENTED_EDGE ( 'NONE', *, *, #30515, .F. ) ;
#24449=CIRCLE ( 'NONE', #35241, 2.000000000000001776 ) ;
#24450=CARTESIAN_POINT ( 'NONE',  ( 0.000000000000000000, 0.000000000000000000, -5.000000000000000000 ) ) ;
#24451=FACE_OUTER_BOUND ( 'NONE', #22596, .T. ) ;
#24452=ORIENTED_EDGE ( 'NONE', *, *, #23433, .F. ) ;
#24454=EDGE_LOOP ( 'NONE', ( #36984, #7508 ) ) ;
#24455=LINE ( 'NONE', #35895, #31664 ) ;
#24456=CARTESIAN_POINT ( 'NONE',  ( -33.00000337463116296, -60.62177826491080168, -5.000000000000000000 ) ) ;
#24459=EDGE_CURVE ( 'NONE', #30221, #22077, #17514, .T. ) ;
#24460=ORIENTED_EDGE ( 'NONE', *, *, #33227, .T. ) ;
#24461=CYLINDRICAL_SURFACE ( 'NONE', #7595, 2.000000000000000000 ) ;
#24462=CIRCLE ( 'NONE', #19058, 2.000000000000001776 ) ;
#24463=ORIENTED_EDGE ( 'NONE', *, *, #8447, .F. ) ;
#24465=CIRCLE ( 'NONE', #8306, 2.000000000000000000 ) ;
#24466=CARTESIAN_POINT ( 'NONE',  ( 0.000000000000000000, 0.000000000000000000, -5.000000000000000000 ) ) ;
#24468=DIRECTION ( 'NONE',  ( -1.000000000000000000, 0.000000000000000000, 0.000000000000000000 ) ) ;
#24469=DIRECTION ( 'NONE',  ( 0.000000000000000000, 0.000000000000000000, -1.000000000000000000 ) ) ;
#24470=CIRCLE ( 'NONE', #1710, 2.000000000000001776 ) ;
#24471=DIRECTION ( 'NONE',  ( 0.000000000000000000, 0.000000000000000000, 1.000000000000000000 ) ) ;
#24472=CIRCLE ( 'NONE', #25096, 2.000000000000001776 ) ;
#24473=EDGE_CURVE ( 'NONE', #25394, #24524, #22108, .T. ) ;
#24475=ORIENTED_EDGE ( 'NONE', *, *, #3481, .T. ) ;
#24476=LINE ( 'NONE', #7399, #27373 ) ;
#24477=FACE_OUTER_BOUND ( 'NONE', #1317, .T. ) ;
#24478=CYLINDRICAL_SURFACE ( 'NONE', #4966, 2.000000000000001776 ) ;
#24479=AXIS2_PLACEMENT_3D ( 'NONE', #15579, #27005, #21382 ) ;
#24481=CIRCLE ( 'NONE', #15479, 2.000000000000001776 ) ;
#24483=ORIENTED_EDGE ( 'NONE', *, *, #28430, .T. ) ;
#24487=EDGE_CURVE ( 'NONE', #985, #12428, #9075, .T. ) ;
#24491=CARTESIAN_POINT ( 'NONE',  ( -65.00000337463104927, -25.98076211353322051, 12.50000000000000000 ) ) ;
#24492=ORIENTED_EDGE ( 'NONE', *, *, #16794, .T. ) ;
#24493=EDGE_CURVE ( 'NONE', #14843, #18158, #14897, .T. ) ;
#24494=CARTESIAN_POINT ( 'NONE',  ( -60.00000337463104216, 51.96152422706639129, 12.50000000000000000 ) ) ;
#24497=DIRECTION ( 'NONE',  ( 1.000000000000000000, 0.000000000000000000, 0.000000000000000000 ) ) ;
#24498=DIRECTION ( 'NONE',  ( 0.000000000000000000, 0.000000000000000000, 1.000000000000000000 ) ) ;
#24500=VECTOR ( 'NONE', #15801, 1000.000000000000000 ) ;
#24501=ADVANCED_FACE ( 'NONE', ( #26336 ), #34956, .F. ) ;
#24502=ORIENTED_EDGE ( 'NONE', *, *, #17585, .F. ) ;
#24504=AXIS2_PLACEMENT_3D ( 'NONE', #33933, #147, #16692 ) ;
#24505=FACE_OUTER_BOUND ( 'NONE', #12908, .T. ) ;
#24506=FACE_OUTER_BOUND ( 'NONE', #33087, .T. ) ;
#24507=AXIS2_PLACEMENT_3D ( 'NONE', #11194, #22831, #17006 ) ;
#24509=CARTESIAN_POINT ( 'NONE',  ( 32.99999662536853862, 77.94228634059959404, -5.000000000000000000 ) ) ;
#24510=CARTESIAN_POINT ( 'NONE',  ( 69.99999662536839651, 34.64101615137758472, 12.50000000000000000 ) ) ;
#24512=VECTOR ( 'NONE', #12068, 1000.000000000000000 ) ;
#24513=CARTESIAN_POINT ( 'NONE',  ( 79.99999662536833966, 17.32050807568879236, -9.999999999999998224 ) ) ;
#24514=DIRECTION ( 'NONE',  ( 0.000000000000000000, 0.000000000000000000, 1.000000000000000000 ) ) ;
#24515=CYLINDRICAL_SURFACE ( 'NONE', #24964, 1.999999999999998224 ) ;
#24516=VERTEX_POINT ( 'NONE', #25960 ) ;
#24517=AXIS2_PLACEMENT_3D ( 'NONE', #36159, #28263, #10462 ) ;
#24519=AXIS2_PLACEMENT_3D ( 'NONE', #2020, #19287, #27538 ) ;
#24522=CARTESIAN_POINT ( 'NONE',  ( 89.67878100130370456, -27.78182860042797131, -49.86348611802629449 ) ) ;
#24523=EDGE_CURVE ( 'NONE', #5915, #18905, #29854, .T. ) ;
#24524=VERTEX_POINT ( 'NONE', #31921 ) ;
#24526=CYLINDRICAL_SURFACE ( 'NONE', #35585, 2.000000000000001776 ) ;
#24527=CARTESIAN_POINT ( 'NONE',  ( 79.99999662536833966, 34.64101615137759183, 12.50000000000000000 ) ) ;
#24529=VECTOR ( 'NONE', #29171, 1000.000000000000000 ) ;
#24530=CARTESIAN_POINT ( 'NONE',  ( -75.00000337463097821, 43.30127018922197379, -9.999999999999998224 ) ) ;
#24531=ORIENTED_EDGE ( 'NONE', *, *, #34311, .T. ) ;
#24533=ORIENTED_EDGE ( 'NONE', *, *, #10827, .T. ) ;
#24534=DIRECTION ( 'NONE',  ( 0.000000000000000000, 0.000000000000000000, 1.000000000000000000 ) ) ;
#24535=VECTOR ( 'NONE', #21848, 1000.000000000000000 ) ;
#24536=DIRECTION ( 'NONE',  ( 0.4999999999999922839, -0.8660254037844431485, 0.000000000000000000 ) ) ;
#24537=ORIENTED_EDGE ( 'NONE', *, *, #5529, .T. ) ;
#24538=EDGE_CURVE ( 'NONE', #20697, #21238, #20148, .T. ) ;
#24539=CIRCLE ( 'NONE', #19737, 2.000000000000001776 ) ;
#24541=ADVANCED_FACE ( 'NONE', ( #5916 ), #28774, .F. ) ;
#24543=DIRECTION ( 'NONE',  ( 0.000000000000000000, 0.000000000000000000, 1.000000000000000000 ) ) ;
#24544=CARTESIAN_POINT ( 'NONE',  ( -80.00000337463094979, 17.32050807568878525, 12.50000000000000000 ) ) ;
#24545=CIRCLE ( 'NONE', #21535, 2.000000000000001776 ) ;
#24546=EDGE_LOOP ( 'NONE', ( #11505, #13056 ) ) ;
#24547=AXIS2_PLACEMENT_3D ( 'NONE', #1461, #21542, #1663 ) ;
#24553=LINE ( 'NONE', #5021, #17784 ) ;
#24555=ORIENTED_EDGE ( 'NONE', *, *, #35816, .F. ) ;
#24557=DIRECTION ( 'NONE',  ( -1.000000000000000000, 0.000000000000000000, 0.000000000000000000 ) ) ;
#24558=CARTESIAN_POINT ( 'NONE',  ( -63.00000337463106348, -60.62177826491083010, -9.999999999999998224 ) ) ;
#24559=DIRECTION ( 'NONE',  ( 1.000000000000000000, 0.000000000000000000, 0.000000000000000000 ) ) ;
#24560=CIRCLE ( 'NONE', #34725, 27.00000000000001066 ) ;
#24563=VECTOR ( 'NONE', #8050, 1000.000000000000000 ) ;
#24564=ORIENTED_EDGE ( 'NONE', *, *, #14238, .T. ) ;
#24565=DIRECTION ( 'NONE',  ( 0.000000000000000000, 0.000000000000000000, 1.000000000000000000 ) ) ;
#24568=ORIENTED_EDGE ( 'NONE', *, *, #33958, .F. ) ;
#24570=CIRCLE ( 'NONE', #9564, 2.000000000000000000 ) ;
#24572=CARTESIAN_POINT ( 'NONE',  ( 72.99999662536836809, -8.660254037844401509, 12.50000000000000000 ) ) ;
#24574=CARTESIAN_POINT ( 'NONE',  ( 19.99999662536858835, 69.28203230275516944, -9.999999999999998224 ) ) ;
#24576=VECTOR ( 'NONE', #6818, 1000.000000000000000 ) ;
#24578=CARTESIAN_POINT ( 'NONE',  ( -80.00000337463094979, 34.64101615137757051, 12.50000000000000000 ) ) ;
#24579=EDGE_CURVE ( 'NONE', #25853, #23244, #8902, .T. ) ;
#24580=AXIS2_PLACEMENT_3D ( 'NONE', #33303, #10617, #22064 ) ;
#24581=CARTESIAN_POINT ( 'NONE',  ( -10.00000337463128730, 69.28203230275516944, -9.999999999999998224 ) ) ;
#24582=CARTESIAN_POINT ( 'NONE',  ( 35.19434990244975126, -52.39915983220758022, -4.999999999999997335 ) ) ;
#24584=VERTEX_POINT ( 'NONE', #29131 ) ;
#24585=DIRECTION ( 'NONE',  ( 1.000000000000000000, 0.000000000000000000, 0.000000000000000000 ) ) ;
#24586=CARTESIAN_POINT ( 'NONE',  ( -68.00000337463099243, 51.96152422706637708, -9.999999999999998224 ) ) ;
#24588=DIRECTION ( 'NONE',  ( 0.000000000000000000, 0.000000000000000000, 1.000000000000000000 ) ) ;
#24589=ADVANCED_FACE ( 'NONE', ( #20337 ), #9461, .T. ) ;
#24590=EDGE_LOOP ( 'NONE', ( #24668, #900, #9000, #9049 ) ) ;
#24591=CARTESIAN_POINT ( 'NONE',  ( 69.99999662536839651, 34.64101615137758472, 12.50000000000000000 ) ) ;
#24592=CARTESIAN_POINT ( 'NONE',  ( -12.00000337463128197, 86.60254037844397601, 12.50000000000000000 ) ) ;
#24593=CYLINDRICAL_SURFACE ( 'NONE', #23376, 2.000000000000001776 ) ;
#24594=ORIENTED_EDGE ( 'NONE', *, *, #21070, .T. ) ;
#24595=DIRECTION ( 'NONE',  ( 1.000000000000000000, 0.000000000000000000, 0.000000000000000000 ) ) ;
#24596=CIRCLE ( 'NONE', #35370, 2.000000000000001776 ) ;
#24597=EDGE_LOOP ( 'NONE', ( #7782, #4337 ) ) ;
#24598=EDGE_CURVE ( 'NONE', #6801, #5741, #2328, .T. ) ;
#24599=CARTESIAN_POINT ( 'NONE',  ( 42.99999662536848888, 60.62177826491077326, -9.999999999999998224 ) ) ;
#24601=DIRECTION ( 'NONE',  ( 0.000000000000000000, 0.000000000000000000, 1.000000000000000000 ) ) ;
#24602=ADVANCED_FACE ( 'NONE', ( #32495 ), #12434, .F. ) ;
#24603=CARTESIAN_POINT ( 'NONE',  ( -61.25926521283079040, 32.16008401677976281, -4.999999999999997335 ) ) ;
#24604=EDGE_CURVE ( 'NONE', #22954, #13911, #32257, .T. ) ;
#24605=VERTEX_POINT ( 'NONE', #12623 ) ;
#24608=ORIENTED_EDGE ( 'NONE', *, *, #6212, .F. ) ;
#24609=CARTESIAN_POINT ( 'NONE',  ( 35.19434990244975126, -52.39915983220758022, 12.49999999999999822 ) ) ;
#24610=CARTESIAN_POINT ( 'NONE',  ( -72.00000337463100664, -17.32050807568882078, -9.999999999999998224 ) ) ;
#24611=LINE ( 'NONE', #1903, #18468 ) ;
#24612=DIRECTION ( 'NONE',  ( 1.000000000000000000, 0.000000000000000000, 0.000000000000000000 ) ) ;
#24616=DIRECTION ( 'NONE',  ( 1.000000000000000000, 0.000000000000000000, 0.000000000000000000 ) ) ;
#24617=AXIS2_PLACEMENT_3D ( 'NONE', #8420, #31645, #3147 ) ;
#24618=DIRECTION ( 'NONE',  ( -1.000000000000000000, 0.000000000000000000, 0.000000000000000000 ) ) ;
#24619=VERTEX_POINT ( 'NONE', #18457 ) ;
#24620=DIRECTION ( 'NONE',  ( 1.000000000000000000, 0.000000000000000000, 0.000000000000000000 ) ) ;
#24621=CARTESIAN_POINT ( 'NONE',  ( 82.99999662536832545, 25.98076211353319565, -9.999999999999998224 ) ) ;
#24622=EDGE_CURVE ( 'NONE', #25195, #24912, #18818, .T. ) ;
#24623=ORIENTED_EDGE ( 'NONE', *, *, #12116, .T. ) ;
#24624=ORIENTED_EDGE ( 'NONE', *, *, #31984, .T. ) ;
#24625=CARTESIAN_POINT ( 'NONE',  ( -80.00000337463094979, 34.64101615137757051, 17.49999999999999645 ) ) ;
#24626=CARTESIAN_POINT ( 'NONE',  ( 9.999996625368655856, -86.60254037844400443, -9.999999999999998224 ) ) ;
#24630=ORIENTED_EDGE ( 'NONE', *, *, #24598, .F. ) ;
#24632=ORIENTED_EDGE ( 'NONE', *, *, #10808, .T. ) ;
#24633=FACE_OUTER_BOUND ( 'NONE', #11074, .T. ) ;
#24635=ORIENTED_EDGE ( 'NONE', *, *, #9805, .T. ) ;
#24636=DIRECTION ( 'NONE',  ( -0.000000000000000000, -0.000000000000000000, 1.000000000000000000 ) ) ;
#24637=DIRECTION ( 'NONE',  ( 0.000000000000000000, 0.000000000000000000, 1.000000000000000000 ) ) ;
#24638=ADVANCED_FACE ( 'NONE', ( #18246 ), #21634, .F. ) ;
#24639=ORIENTED_EDGE ( 'NONE', *, *, #5667, .T. ) ;
#24640=ORIENTED_EDGE ( 'NONE', *, *, #6671, .F. ) ;
#24641=CARTESIAN_POINT ( 'NONE',  ( 69.99999662536838230, -34.64101615137759183, -9.999999999999998224 ) ) ;
#24642=CARTESIAN_POINT ( 'NONE',  ( 19.13981058454793072, -60.93295298010985306, 12.49999999999999822 ) ) ;
#24643=DIRECTION ( 'NONE',  ( 0.000000000000000000, 0.000000000000000000, 1.000000000000000000 ) ) ;
#24644=CARTESIAN_POINT ( 'NONE',  ( 74.99999662536836809, -8.660254037844401509, -9.999999999999998224 ) ) ;
#24645=ORIENTED_EDGE ( 'NONE', *, *, #11776, .F. ) ;
#24646=DIRECTION ( 'NONE',  ( 0.000000000000000000, 0.000000000000000000, 1.000000000000000000 ) ) ;
#24647=VERTEX_POINT ( 'NONE', #30058 ) ;
#24649=DIRECTION ( 'NONE',  ( 0.000000000000000000, 0.000000000000000000, -1.000000000000000000 ) ) ;
#24650=CARTESIAN_POINT ( 'NONE',  ( -28.00000337463119493, -69.28203230275522628, 17.49999999999999645 ) ) ;
#24651=CYLINDRICAL_SURFACE ( 'NONE', #26081, 3.499999999999989342 ) ;
#24652=CARTESIAN_POINT ( 'NONE',  ( 42.99999662536848888, -77.94228634059960825, -9.999999999999998224 ) ) ;
#24653=CARTESIAN_POINT ( 'NONE',  ( 87.83969979969882047, 14.80603122773025504, -4.999999999999997335 ) ) ;
#24655=ORIENTED_EDGE ( 'NONE', *, *, #33247, .F. ) ;
#24656=DIRECTION ( 'NONE',  ( 0.000000000000000000, 0.000000000000000000, 1.000000000000000000 ) ) ;
#24657=AXIS2_PLACEMENT_3D ( 'NONE', #27571, #30175, #7318 ) ;
#24659=CARTESIAN_POINT ( 'NONE',  ( -45.00000337463112743, -60.62177826491080168, -5.000000000000000000 ) ) ;
#24661=ADVANCED_FACE ( 'NONE', ( #7011 ), #4010, .F. ) ;
#24662=ORIENTED_EDGE ( 'NONE', *, *, #30366, .F. ) ;
#24663=ORIENTED_EDGE ( 'NONE', *, *, #33222, .F. ) ;
#24666=DIRECTION ( 'NONE',  ( 0.000000000000000000, 0.000000000000000000, 1.000000000000000000 ) ) ;
#24667=EDGE_CURVE ( 'NONE', #12006, #20765, #24075, .T. ) ;
#24668=ORIENTED_EDGE ( 'NONE', *, *, #1175, .F. ) ;
#24670=ADVANCED_FACE ( 'NONE', ( #27059 ), #33061, .F. ) ;
#24671=CYLINDRICAL_SURFACE ( 'NONE', #20092, 2.000000000000001776 ) ;
#24672=EDGE_LOOP ( 'NONE', ( #5083, #6549 ) ) ;
#24673=CARTESIAN_POINT ( 'NONE',  ( 34.99999662536855283, -60.62177826491080168, -5.000000000000000000 ) ) ;
#24674=ORIENTED_EDGE ( 'NONE', *, *, #32987, .F. ) ;
#24675=CYLINDRICAL_SURFACE ( 'NONE', #13543, 2.000000000000001776 ) ;
#24676=CARTESIAN_POINT ( 'NONE',  ( 47.99999662536846756, -69.28203230275519786, 17.49999999999999645 ) ) ;
#24677=CARTESIAN_POINT ( 'NONE',  ( -7.000003374631269537, -77.94228634059960825, -9.999999999999998224 ) ) ;
#24678=AXIS2_PLACEMENT_3D ( 'NONE', #19754, #33246, #2320 ) ;
#24679=FACE_OUTER_BOUND ( 'NONE', #17095, .T. ) ;
#24680=ADVANCED_FACE ( 'NONE', ( #12793 ), #16011, .F. ) ;
#24681=ORIENTED_EDGE ( 'NONE', *, *, #89, .F. ) ;
#24682=CYLINDRICAL_SURFACE ( 'NONE', #7512, 27.00000000000001421 ) ;
#24684=DIRECTION ( 'NONE',  ( 1.000000000000000000, 0.000000000000000000, 0.000000000000000000 ) ) ;
#24685=DIRECTION ( 'NONE',  ( 1.000000000000000000, 0.000000000000000000, 0.000000000000000000 ) ) ;
#24686=EDGE_LOOP ( 'NONE', ( #11089, #29928, #23827, #26321, #2872 ) ) ;
#24687=CARTESIAN_POINT ( 'NONE',  ( 79.99999662536833966, 17.32050807568879236, -5.000000000000000000 ) ) ;
#24688=CARTESIAN_POINT ( 'NONE',  ( 2.999996625368676728, -77.94228634059960825, -9.999999999999998224 ) ) ;
#24689=EDGE_LOOP ( 'NONE', ( #29069, #36980, #29108, #10324 ) ) ;
#24690=DIRECTION ( 'NONE',  ( 1.000000000000000000, 0.000000000000000000, 0.000000000000000000 ) ) ;
#24691=CARTESIAN_POINT ( 'NONE',  ( 64.99999662536839651, 60.62177826491078747, -5.000000000000000000 ) ) ;
#24693=ORIENTED_EDGE ( 'NONE', *, *, #22464, .T. ) ;
#24694=ADVANCED_FACE ( 'NONE', ( #24246 ), #12996, .F. ) ;
#24696=DIRECTION ( 'NONE',  ( -0.000000000000000000, -0.000000000000000000, 1.000000000000000000 ) ) ;
#24697=DIRECTION ( 'NONE',  ( 0.000000000000000000, 0.000000000000000000, -1.000000000000000000 ) ) ;
#24701=AXIS2_PLACEMENT_3D ( 'NONE', #3613, #12391, #23860 ) ;
#24702=CARTESIAN_POINT ( 'NONE',  ( -45.00000337463112743, -60.62177826491080168, 12.50000000000000000 ) ) ;
#24704=EDGE_CURVE ( 'NONE', #26494, #25226, #24455, .T. ) ;
#24705=DIRECTION ( 'NONE',  ( 0.000000000000000000, 0.000000000000000000, -1.000000000000000000 ) ) ;
#24707=ORIENTED_EDGE ( 'NONE', *, *, #20552, .F. ) ;
#24708=ORIENTED_EDGE ( 'NONE', *, *, #36539, .T. ) ;
#24709=CARTESIAN_POINT ( 'NONE',  ( -32.16008401677955675, -61.25926521283091830, -4.999999999999997335 ) ) ;
#24710=ADVANCED_FACE ( 'NONE', ( #27236 ), #1558, .F. ) ;
#24712=ORIENTED_EDGE ( 'NONE', *, *, #15512, .T. ) ;
#24713=CARTESIAN_POINT ( 'NONE',  ( 69.99999662536841072, 51.96152422706640550, 12.50000000000000000 ) ) ;
#24715=LINE ( 'NONE', #7097, #24312 ) ;
#24716=AXIS2_PLACEMENT_3D ( 'NONE', #12774, #9790, #15990 ) ;
#24717=DIRECTION ( 'NONE',  ( 0.000000000000000000, 0.000000000000000000, 1.000000000000000000 ) ) ;
#24718=ORIENTED_EDGE ( 'NONE', *, *, #14403, .F. ) ;
#24720=VERTEX_POINT ( 'NONE', #30439 ) ;
#24724=CIRCLE ( 'NONE', #33692, 2.000000000000000000 ) ;
#24725=CYLINDRICAL_SURFACE ( 'NONE', #24547, 2.000000000000001776 ) ;
#24726=DIRECTION ( 'NONE',  ( 0.000000000000000000, 0.000000000000000000, 1.000000000000000000 ) ) ;
#24729=CARTESIAN_POINT ( 'NONE',  ( 86.99999662536832545, 25.98076211353319565, 17.49999999999999645 ) ) ;
#24730=LINE ( 'NONE', #24558, #35787 ) ;
#24731=DIRECTION ( 'NONE',  ( 0.000000000000000000, 0.000000000000000000, 1.000000000000000000 ) ) ;
#24732=ORIENTED_EDGE ( 'NONE', *, *, #31220, .T. ) ;
#24734=ORIENTED_EDGE ( 'NONE', *, *, #19958, .T. ) ;
#24735=EDGE_LOOP ( 'NONE', ( #19631, #480, #12903, #18534 ) ) ;
#24736=ADVANCED_FACE ( 'NONE', ( #13359 ), #36996, .F. ) ;
#24737=CARTESIAN_POINT ( 'NONE',  ( 64.99999662536839651, -43.30127018922199511, 17.49999999999999645 ) ) ;
#24738=ORIENTED_EDGE ( 'NONE', *, *, #14200, .T. ) ;
#24740=DIRECTION ( 'NONE',  ( 0.000000000000000000, 0.000000000000000000, -1.000000000000000000 ) ) ;
#24741=VECTOR ( 'NONE', #13684, 1000.000000000000000 ) ;
#24742=CARTESIAN_POINT ( 'NONE',  ( 33.21453428580180400, -78.84346569788027637, -5.000000000000000000 ) ) ;
#24743=DIRECTION ( 'NONE',  ( 0.000000000000000000, 0.000000000000000000, -1.000000000000000000 ) ) ;
#24745=DIRECTION ( 'NONE',  ( 0.000000000000000000, 0.000000000000000000, 1.000000000000000000 ) ) ;
#24747=LINE ( 'NONE', #1486, #4701 ) ;
#24748=ORIENTED_EDGE ( 'NONE', *, *, #27891, .F. ) ;
#24749=ORIENTED_EDGE ( 'NONE', *, *, #30749, .T. ) ;
#24751=EDGE_CURVE ( 'NONE', #8894, #26711, #8489, .T. ) ;
#24753=DIRECTION ( 'NONE',  ( 0.000000000000000000, 0.000000000000000000, -1.000000000000000000 ) ) ;
#24754=CARTESIAN_POINT ( 'NONE',  ( 36.99999662536855283, -77.94228634059960825, -9.999999999999998224 ) ) ;
#24755=VERTEX_POINT ( 'NONE', #16758 ) ;
#24756=DIRECTION ( 'NONE',  ( 0.000000000000000000, 0.000000000000000000, 1.000000000000000000 ) ) ;
#24758=ORIENTED_EDGE ( 'NONE', *, *, #24053, .T. ) ;
#24760=DIRECTION ( 'NONE',  ( 0.000000000000000000, 0.000000000000000000, 1.000000000000000000 ) ) ;
#24761=CIRCLE ( 'NONE', #8584, 2.000000000000001776 ) ;
#24762=ORIENTED_EDGE ( 'NONE', *, *, #25711, .F. ) ;
#24763=PRESENTATION_STYLE_ASSIGNMENT (( #33587 ) ) ;
#24764=CARTESIAN_POINT ( 'NONE',  ( -35.00000337463116296, 77.94228634059957983, -9.999999999999998224 ) ) ;
#24765=CIRCLE ( 'NONE', #3205, 3.000000000000007105 ) ;
#24766=DIRECTION ( 'NONE',  ( 0.000000000000000000, 0.000000000000000000, 1.000000000000000000 ) ) ;
#24767=EDGE_CURVE ( 'NONE', #15438, #8840, #13918, .T. ) ;
#24768=CARTESIAN_POINT ( 'NONE',  ( -5.000003374631269537, -77.94228634059960825, -5.000000000000000000 ) ) ;
#24769=ORIENTED_EDGE ( 'NONE', *, *, #27978, .F. ) ;
#24770=EDGE_CURVE ( 'NONE', #698, #24284, #32281, .T. ) ;
#24771=ORIENTED_EDGE ( 'NONE', *, *, #6174, .F. ) ;
#24772=AXIS2_PLACEMENT_3D ( 'NONE', #7245, #12841, #15862 ) ;
#24773=ADVANCED_FACE ( 'NONE', ( #2111 ), #22192, .F. ) ;
#24776=VECTOR ( 'NONE', #9220, 1000.000000000000000 ) ;
#24779=DIRECTION ( 'NONE',  ( 0.000000000000000000, 0.000000000000000000, 1.000000000000000000 ) ) ;
#24780=DIRECTION ( 'NONE',  ( 1.000000000000000000, 0.000000000000000000, 0.000000000000000000 ) ) ;
#24781=CARTESIAN_POINT ( 'NONE',  ( -72.00000337463100664, 34.64101615137758472, -9.999999999999998224 ) ) ;
#24783=ORIENTED_EDGE ( 'NONE', *, *, #32837, .F. ) ;
#24784=DIRECTION ( 'NONE',  ( 0.000000000000000000, 0.000000000000000000, 1.000000000000000000 ) ) ;
#24786=CARTESIAN_POINT ( 'NONE',  ( 69.99999662536839651, -3.469446951953614189E-15, -5.000000000000000000 ) ) ;
#24787=CARTESIAN_POINT ( 'NONE',  ( 19.99999662536861678, -69.28203230275519786, -9.999999999999998224 ) ) ;
#24789=DIRECTION ( 'NONE',  ( 1.000000000000000000, 0.000000000000000000, 0.000000000000000000 ) ) ;
#24790=DIRECTION ( 'NONE',  ( 0.000000000000000000, 0.000000000000000000, 1.000000000000000000 ) ) ;
#24791=EDGE_CURVE ( 'NONE', #7889, #27142, #7761, .T. ) ;
#24792=ORIENTED_EDGE ( 'NONE', *, *, #33421, .F. ) ;
#24793=EDGE_CURVE ( 'NONE', #25244, #5952, #2970, .T. ) ;
#24795=VERTEX_POINT ( 'NONE', #33446 ) ;
#24797=EDGE_CURVE ( 'NONE', #15477, #32385, #34689, .T. ) ;
#24798=DIRECTION ( 'NONE',  ( 0.000000000000000000, 0.000000000000000000, -1.000000000000000000 ) ) ;
#24801=CARTESIAN_POINT ( 'NONE',  ( 62.99999662536839651, 60.62177826491078747, -9.999999999999998224 ) ) ;
#24803=VERTEX_POINT ( 'NONE', #36627 ) ;
#24804=ORIENTED_EDGE ( 'NONE', *, *, #23838, .T. ) ;
#24806=CARTESIAN_POINT ( 'NONE',  ( 67.99999662536836809, -51.96152422706639840, -9.999999999999998224 ) ) ;
#24808=ORIENTED_EDGE ( 'NONE', *, *, #29809, .F. ) ;
#24809=FACE_BOUND ( 'NONE', #6727, .T. ) ;
#24810=EDGE_LOOP ( 'NONE', ( #27191, #32912, #22478, #36587 ) ) ;
#24811=ORIENTED_EDGE ( 'NONE', *, *, #3496, .T. ) ;
#24812=DIRECTION ( 'NONE',  ( 1.000000000000000000, 0.000000000000000000, 0.000000000000000000 ) ) ;
#24814=LINE ( 'NONE', #18815, #7502 ) ;
#24815=ORIENTED_EDGE ( 'NONE', *, *, #2676, .F. ) ;
#24816=EDGE_LOOP ( 'NONE', ( #15094, #35508, #21839 ) ) ;
#24818=DIRECTION ( 'NONE',  ( 0.000000000000000000, 0.000000000000000000, 1.000000000000000000 ) ) ;
#24820=CYLINDRICAL_SURFACE ( 'NONE', #7713, 2.000000000000000000 ) ;
#24822=EDGE_LOOP ( 'NONE', ( #18506, #713, #23327 ) ) ;
#24823=DIRECTION ( 'NONE',  ( 0.000000000000000000, 0.000000000000000000, 1.000000000000000000 ) ) ;
#24824=FACE_BOUND ( 'NONE', #13989, .T. ) ;
#24826=FACE_BOUND ( 'NONE', #20556, .T. ) ;
#24828=CARTESIAN_POINT ( 'NONE',  ( -65.00000337463104927, -25.98076211353322051, -9.999999999999998224 ) ) ;
#24829=CIRCLE ( 'NONE', #8644, 2.000000000000001776 ) ;
#24832=CIRCLE ( 'NONE', #2061, 2.000000000000001776 ) ;
#24833=CARTESIAN_POINT ( 'NONE',  ( -17.14523346298280160, 93.36492675454785228, -4.999999999999997335 ) ) ;
#24835=CARTESIAN_POINT ( 'NONE',  ( 57.99999662536842493, 51.96152422706639129, -9.999999999999998224 ) ) ;
#24837=DIRECTION ( 'NONE',  ( -1.000000000000000000, 0.000000000000000000, 0.000000000000000000 ) ) ;
#24839=ORIENTED_EDGE ( 'NONE', *, *, #36064, .F. ) ;
#24841=AXIS2_PLACEMENT_3D ( 'NONE', #20603, #34880, #34708 ) ;
#24842=ADVANCED_FACE ( 'NONE', ( #2316 ), #22361, .F. ) ;
#24843=CARTESIAN_POINT ( 'NONE',  ( -70.00000337463099243, 34.64101615137758472, -9.999999999999998224 ) ) ;
#24844=CARTESIAN_POINT ( 'NONE',  ( -43.00000337463111322, 60.62177826491077326, -9.999999999999998224 ) ) ;
#24845=AXIS2_PLACEMENT_3D ( 'NONE', #29984, #32986, #13112 ) ;
#24847=CIRCLE ( 'NONE', #21240, 2.000000000000001776 ) ;
#24848=FACE_OUTER_BOUND ( 'NONE', #7213, .T. ) ;
#24849=CARTESIAN_POINT ( 'NONE',  ( 49.99999662536846756, 69.28203230275516944, -9.999999999999998224 ) ) ;
#24850=VERTEX_POINT ( 'NONE', #8116 ) ;
#24851=DIRECTION ( 'NONE',  ( 1.000000000000000000, 0.000000000000000000, 0.000000000000000000 ) ) ;
#24853=FACE_BOUND ( 'NONE', #6759, .T. ) ;
#24854=CIRCLE ( 'NONE', #28444, 2.000000000000001776 ) ;
#24855=AXIS2_PLACEMENT_3D ( 'NONE', #5063, #16499, #27933 ) ;
#24856=VECTOR ( 'NONE', #2948, 1000.000000000000000 ) ;
#24860=ORIENTED_EDGE ( 'NONE', *, *, #19735, .T. ) ;
#24861=CARTESIAN_POINT ( 'NONE',  ( 76.99999662536835388, -43.30127018922199511, -9.999999999999998224 ) ) ;
#24863=EDGE_CURVE ( 'NONE', #8511, #6351, #10757, .T. ) ;
#24864=CARTESIAN_POINT ( 'NONE',  ( 56.67878100130369035, -27.78182860042797131, 12.49999999999999822 ) ) ;
#24865=DIRECTION ( 'NONE',  ( 1.000000000000000000, 0.000000000000000000, 0.000000000000000000 ) ) ;
#24866=AXIS2_PLACEMENT_3D ( 'NONE', #30163, #27161, #9567 ) ;
#24867=ORIENTED_EDGE ( 'NONE', *, *, #28554, .F. ) ;
#24868=DIRECTION ( 'NONE',  ( 0.000000000000000000, 0.000000000000000000, 1.000000000000000000 ) ) ;
#24869=CARTESIAN_POINT ( 'NONE',  ( -45.00000337463111322, 60.62177826491077326, -9.999999999999998224 ) ) ;
#24870=ORIENTED_EDGE ( 'NONE', *, *, #12341, .T. ) ;
#24873=CARTESIAN_POINT ( 'NONE',  ( -2.374207310413330682E-13, -68.00000000000000000, 12.49999999999999822 ) ) ;
#24874=DIRECTION ( 'NONE',  ( -1.000000000000000000, 0.000000000000000000, -0.000000000000000000 ) ) ;
#24875=AXIS2_PLACEMENT_3D ( 'NONE', #34812, #25822, #5947 ) ;
#24876=ORIENTED_EDGE ( 'NONE', *, *, #5679, .F. ) ;
#24877=ORIENTED_EDGE ( 'NONE', *, *, #11475, .F. ) ;
#24878=DIRECTION ( 'NONE',  ( 0.4999999999999919509, -0.8660254037844432595, 0.000000000000000000 ) ) ;
#24879=CARTESIAN_POINT ( 'NONE',  ( 79.99999662536832545, -17.32050807568879591, -9.999999999999998224 ) ) ;
#24880=AXIS2_PLACEMENT_3D ( 'NONE', #33715, #25279, #14003 ) ;
#24882=LINE ( 'NONE', #33317, #24908 ) ;
#24883=ORIENTED_EDGE ( 'NONE', *, *, #6316, .F. ) ;
#24884=ORIENTED_EDGE ( 'NONE', *, *, #14938, .F. ) ;
#24885=EDGE_CURVE ( 'NONE', #33342, #22150, #30990, .T. ) ;
#24887=CARTESIAN_POINT ( 'NONE',  ( 76.99999662536835388, -43.30127018922199511, 17.49999999999999645 ) ) ;
#24890=ORIENTED_EDGE ( 'NONE', *, *, #7890, .F. ) ;
#24891=VERTEX_POINT ( 'NONE', #35043 ) ;
#24892=LINE ( 'NONE', #35596, #4528 ) ;
#24893=VECTOR ( 'NONE', #31384, 1000.000000000000000 ) ;
#24894=CARTESIAN_POINT ( 'NONE',  ( -65.00000337463102085, 60.62177826491077326, 17.49999999999999645 ) ) ;
#24895=ORIENTED_EDGE ( 'NONE', *, *, #14932, .T. ) ;
#24896=CIRCLE ( 'NONE', #15298, 2.000000000000001776 ) ;
#24897=CYLINDRICAL_SURFACE ( 'NONE', #23317, 2.000000000000001776 ) ;
#24898=ORIENTED_EDGE ( 'NONE', *, *, #36244, .F. ) ;
#24899=FACE_OUTER_BOUND ( 'NONE', #27295, .T. ) ;
#24900=CIRCLE ( 'NONE', #8720, 2.000000000000001776 ) ;
#24901=CIRCLE ( 'NONE', #29663, 1.999999999999998224 ) ;
#24902=CIRCLE ( 'NONE', #23092, 3.000000000000002665 ) ;
#24903=LINE ( 'NONE', #8013, #22705 ) ;
#24904=ADVANCED_FACE ( 'NONE', ( #14304 ), #723, .F. ) ;
#24907=EDGE_CURVE ( 'NONE', #8706, #34583, #6547, .T. ) ;
#24908=VECTOR ( 'NONE', #7440, 1000.000000000000000 ) ;
#24909=DIRECTION ( 'NONE',  ( -0.000000000000000000, -0.000000000000000000, 1.000000000000000000 ) ) ;
#24910=CARTESIAN_POINT ( 'NONE',  ( 74.99999662536836809, -8.660254037844401509, 12.50000000000000000 ) ) ;
#24911=DIRECTION ( 'NONE',  ( 1.000000000000000000, 0.000000000000000000, 0.000000000000000000 ) ) ;
#24912=VERTEX_POINT ( 'NONE', #18155 ) ;
#24913=CARTESIAN_POINT ( 'NONE',  ( 61.99999662536842493, -51.96152422706639840, -9.999999999999998224 ) ) ;
#24914=EDGE_CURVE ( 'NONE', #32504, #9552, #21510, .T. ) ;
#24915=CARTESIAN_POINT ( 'NONE',  ( -60.00000337463104216, 34.64101615137757051, -5.000000000000000000 ) ) ;
#24917=ORIENTED_EDGE ( 'NONE', *, *, #30070, .T. ) ;
#24920=ADVANCED_FACE ( 'NONE', ( #26975 ), #29579, .F. ) ;
#24922=FACE_OUTER_BOUND ( 'NONE', #30868, .T. ) ;
#24923=ORIENTED_EDGE ( 'NONE', *, *, #13716, .T. ) ;
#24924=AXIS2_PLACEMENT_3D ( 'NONE', #11070, #11268, #19525 ) ;
#24927=CARTESIAN_POINT ( 'NONE',  ( -77.00000337463097821, 25.98076211353318854, 12.50000000000000000 ) ) ;
#24928=AXIS2_PLACEMENT_3D ( 'NONE', #33008, #24756, #7323 ) ;
#24929=CIRCLE ( 'NONE', #23746, 2.000000000000000000 ) ;
#24931=DIRECTION ( 'NONE',  ( 0.000000000000000000, 0.000000000000000000, 1.000000000000000000 ) ) ;
#24932=VECTOR ( 'NONE', #33356, 1000.000000000000000 ) ;
#24933=LINE ( 'NONE', #12919, #10444 ) ;
#24934=DIRECTION ( 'NONE',  ( 1.000000000000000000, 0.000000000000000000, 0.000000000000000000 ) ) ;
#24935=CARTESIAN_POINT ( 'NONE',  ( -18.00000337463124467, 69.28203230275516944, 12.50000000000000000 ) ) ;
#24937=CARTESIAN_POINT ( 'NONE',  ( 81.99999662536833966, -3.469446951953614189E-15, -9.999999999999998224 ) ) ;
#24939=CIRCLE ( 'NONE', #26098, 2.000000000000001776 ) ;
#24941=ADVANCED_FACE ( 'NONE', ( #3907 ), #12135, .F. ) ;
#24942=CARTESIAN_POINT ( 'NONE',  ( -8.000003374631278419, -69.28203230275519786, -9.999999999999998224 ) ) ;
#24943=DIRECTION ( 'NONE',  ( 0.4999999999999922839, -0.8660254037844431485, 0.000000000000000000 ) ) ;
#24944=CARTESIAN_POINT ( 'NONE',  ( -53.00000337463109190, -60.62177826491083010, 17.49999999999999645 ) ) ;
#24945=DIRECTION ( 'NONE',  ( -0.5000000000000101030, -0.8660254037844329345, 0.000000000000000000 ) ) ;
#24946=ORIENTED_EDGE ( 'NONE', *, *, #17656, .T. ) ;
#24948=AXIS2_PLACEMENT_3D ( 'NONE', #52, #7767, #16927 ) ;
#24950=CARTESIAN_POINT ( 'NONE',  ( -73.00000337463100664, -43.30127018922202353, -9.999999999999998224 ) ) ;
#24951=AXIS2_PLACEMENT_3D ( 'NONE', #29242, #35060, #15176 ) ;
#24952=CARTESIAN_POINT ( 'NONE',  ( 56.99999662536844625, 60.62177826491077326, 12.50000000000000000 ) ) ;
#24953=ORIENTED_EDGE ( 'NONE', *, *, #17386, .T. ) ;
#24954=EDGE_CURVE ( 'NONE', #7561, #10165, #30507, .T. ) ;
#24956=CYLINDRICAL_SURFACE ( 'NONE', #33215, 2.000000000000001776 ) ;
#24957=EDGE_LOOP ( 'NONE', ( #33987, #34298 ) ) ;
#24958=CIRCLE ( 'NONE', #8772, 2.000000000000001776 ) ;
#24959=AXIS2_PLACEMENT_3D ( 'NONE', #12997, #30059, #1205 ) ;
#24960=AXIS2_PLACEMENT_3D ( 'NONE', #16260, #35765, #1990 ) ;
#24961=DIRECTION ( 'NONE',  ( 1.000000000000000000, 0.000000000000000000, 0.000000000000000000 ) ) ;
#24963=DIRECTION ( 'NONE',  ( 0.4999999999999919509, -0.8660254037844432595, 0.000000000000000000 ) ) ;
#24964=AXIS2_PLACEMENT_3D ( 'NONE', #1818, #10974, #35956 ) ;
#24965=CARTESIAN_POINT ( 'NONE',  ( -58.88972745734155723, 34.00000000000049027, 12.49999999999999822 ) ) ;
#24968=AXIS2_PLACEMENT_3D ( 'NONE', #14139, #33664, #7968 ) ;
#24969=EDGE_CURVE ( 'NONE', #875, #8614, #9723, .T. ) ;
#24970=ORIENTED_EDGE ( 'NONE', *, *, #29264, .F. ) ;
#24971=CARTESIAN_POINT ( 'NONE',  ( 66.99999662536842493, 43.30127018922200222, 12.50000000000000000 ) ) ;
#24972=CARTESIAN_POINT ( 'NONE',  ( 77.99999662536832545, -17.32050807568879591, -9.999999999999998224 ) ) ;
#24973=CARTESIAN_POINT ( 'NONE',  ( -33.00000337463116296, -60.62177826491080168, -9.999999999999998224 ) ) ;
#24976=ORIENTED_EDGE ( 'NONE', *, *, #21115, .F. ) ;
#24978=FACE_OUTER_BOUND ( 'NONE', #24434, .T. ) ;
#24979=AXIS2_PLACEMENT_3D ( 'NONE', #18572, #29989, #1475 ) ;
#24981=ORIENTED_EDGE ( 'NONE', *, *, #30013, .T. ) ;
#24982=DIRECTION ( 'NONE',  ( 1.000000000000000000, 0.000000000000000000, 0.000000000000000000 ) ) ;
#24983=FACE_OUTER_BOUND ( 'NONE', #17920, .T. ) ;
#24984=ORIENTED_EDGE ( 'NONE', *, *, #29576, .T. ) ;
#24986=VERTEX_POINT ( 'NONE', #23800 ) ;
#24987=AXIS2_PLACEMENT_3D ( 'NONE', #10018, #32336, #6654 ) ;
#24990=CARTESIAN_POINT ( 'NONE',  ( 2.999996625368645198, 77.94228634059957983, -9.999999999999998224 ) ) ;
#24992=ADVANCED_FACE ( 'NONE', ( #17791 ), #12705, .F. ) ;
#24994=ORIENTED_EDGE ( 'NONE', *, *, #15585, .F. ) ;
#24995=ORIENTED_EDGE ( 'NONE', *, *, #6887, .F. ) ;
#24996=AXIS2_PLACEMENT_3D ( 'NONE', #4759, #21438, #27430 ) ;
#24997=EDGE_CURVE ( 'NONE', #29968, #9610, #36486, .T. ) ;
#24998=DIRECTION ( 'NONE',  ( -1.000000000000000000, 0.000000000000000000, 0.000000000000000000 ) ) ;
#24999=VERTEX_POINT ( 'NONE', #25753 ) ;
#25000=EDGE_CURVE ( 'NONE', #32624, #30112, #17341, .T. ) ;
#25001=EDGE_CURVE ( 'NONE', #28672, #32425, #3556, .T. ) ;
#25002=PLANE ( 'NONE',  #11789 ) ;
#25003=ORIENTED_EDGE ( 'NONE', *, *, #34211, .T. ) ;
#25005=CIRCLE ( 'NONE', #36378, 27.00000000000000711 ) ;
#25006=VERTEX_POINT ( 'NONE', #1849 ) ;
#25007=DIRECTION ( 'NONE',  ( 0.000000000000000000, 0.000000000000000000, -1.000000000000000000 ) ) ;
#25008=VECTOR ( 'NONE', #7950, 1000.000000000000000 ) ;
#25011=EDGE_LOOP ( 'NONE', ( #10558, #9720 ) ) ;
#25013=CARTESIAN_POINT ( 'NONE',  ( 73.90204319670435495, -6.988578749851858340, 12.50000000000000000 ) ) ;
#25014=ADVANCED_FACE ( 'NONE', ( #21714 ), #10113, .F. ) ;
#25017=CARTESIAN_POINT ( 'NONE',  ( 9.999996625368618552, 69.28203230275516944, 12.50000000000000000 ) ) ;
#25019=DIRECTION ( 'NONE',  ( 0.000000000000000000, 0.000000000000000000, 1.000000000000000000 ) ) ;
#25021=EDGE_CURVE ( 'NONE', #2623, #22366, #16730, .T. ) ;
#25022=EDGE_LOOP ( 'NONE', ( #33867, #21536 ) ) ;
#25023=DIRECTION ( 'NONE',  ( 1.000000000000000000, 0.000000000000000000, 0.000000000000000000 ) ) ;
#25024=DIRECTION ( 'NONE',  ( 1.000000000000000000, 0.000000000000000000, 0.000000000000000000 ) ) ;
#25025=DIRECTION ( 'NONE',  ( -0.000000000000000000, -0.000000000000000000, -1.000000000000000000 ) ) ;
#25026=CARTESIAN_POINT ( 'NONE',  ( 19.99999662536857770, 86.60254037844397601, 12.50000000000000000 ) ) ;
#25027=AXIS2_PLACEMENT_3D ( 'NONE', #1816, #1253, #23955 ) ;
#25028=DIRECTION ( 'NONE',  ( 1.000000000000000000, 0.000000000000000000, 0.000000000000000000 ) ) ;
#25029=CARTESIAN_POINT ( 'NONE',  ( 74.99999662536835388, -43.30127018922199511, -5.000000000000000000 ) ) ;
#25031=AXIS2_PLACEMENT_3D ( 'NONE', #432, #34223, #17676 ) ;
#25032=CARTESIAN_POINT ( 'NONE',  ( -35.00000337463117717, -77.94228634059963667, -5.000000000000000000 ) ) ;
#25033=VERTEX_POINT ( 'NONE', #13100 ) ;
#25034=CARTESIAN_POINT ( 'NONE',  ( -10.00000337463128197, 86.60254037844397601, -9.999999999999998224 ) ) ;
#25035=CIRCLE ( 'NONE', #18441, 2.000000000000001776 ) ;
#25038=CIRCLE ( 'NONE', #31593, 95.00000000000001421 ) ;
#25039=ORIENTED_EDGE ( 'NONE', *, *, #35009, .T. ) ;
#25040=ORIENTED_EDGE ( 'NONE', *, *, #29359, .T. ) ;
#25041=EDGE_CURVE ( 'NONE', #20586, #11580, #3552, .T. ) ;
#25042=ORIENTED_EDGE ( 'NONE', *, *, #33020, .F. ) ;
#25044=DIRECTION ( 'NONE',  ( 1.000000000000000000, 0.000000000000000000, 0.000000000000000000 ) ) ;
#25045=LINE ( 'NONE', #13945, #29827 ) ;
#25046=ADVANCED_FACE ( 'NONE', ( #12896 ), #13274, .F. ) ;
#25047=EDGE_LOOP ( 'NONE', ( #2910, #7191, #29886, #23337, #6641, #14959, #3597, #12141 ) ) ;
#25048=CARTESIAN_POINT ( 'NONE',  ( -58.00000337463107059, -34.64101615137762025, 12.50000000000000000 ) ) ;
#25049=DIRECTION ( 'NONE',  ( 1.000000000000000000, 0.000000000000000000, 0.000000000000000000 ) ) ;
#25050=EDGE_LOOP ( 'NONE', ( #31208, #12214 ) ) ;
#25052=ORIENTED_EDGE ( 'NONE', *, *, #1794, .T. ) ;
#25053=ADVANCED_FACE ( 'NONE', ( #13447 ), #24725, .F. ) ;
#25054=CARTESIAN_POINT ( 'NONE',  ( -82.00000337463096400, -34.64101615137762025, -9.999999999999998224 ) ) ;
#25055=CIRCLE ( 'NONE', #3467, 2.000000000000001776 ) ;
#25056=CARTESIAN_POINT ( 'NONE',  ( 86.99999662536831124, -8.660254037844397956, -9.999999999999998224 ) ) ;
#25057=CARTESIAN_POINT ( 'NONE',  ( -35.00000337463117717, -77.94228634059963667, 12.50000000000000000 ) ) ;
#25058=CIRCLE ( 'NONE', #8869, 2.000000000000001776 ) ;
#25059=VERTEX_POINT ( 'NONE', #10661 ) ;
#25060=LINE ( 'NONE', #2921, #12877 ) ;
#25061=CIRCLE ( 'NONE', #7086, 2.000000000000001776 ) ;
#25063=EDGE_CURVE ( 'NONE', #27693, #29836, #32314, .T. ) ;
#25064=AXIS2_PLACEMENT_3D ( 'NONE', #6693, #18120, #15308 ) ;
#25065=DIRECTION ( 'NONE',  ( 0.000000000000000000, 0.000000000000000000, 1.000000000000000000 ) ) ;
#25066=EDGE_CURVE ( 'NONE', #30130, #29077, #3580, .T. ) ;
#25068=AXIS2_PLACEMENT_3D ( 'NONE', #28319, #11075, #5636 ) ;
#25069=EDGE_CURVE ( 'NONE', #35055, #32859, #36158, .T. ) ;
#25071=CARTESIAN_POINT ( 'NONE',  ( -62.97617850287781494, -4.279621169095772615, 12.49999999999999822 ) ) ;
#25073=ADVANCED_FACE ( 'NONE', ( #30703 ), #10461, .F. ) ;
#25074=ORIENTED_EDGE ( 'NONE', *, *, #28914, .T. ) ;
#25077=FACE_OUTER_BOUND ( 'NONE', #9898, .T. ) ;
#25079=ORIENTED_EDGE ( 'NONE', *, *, #34940, .T. ) ;
#25082=AXIS2_PLACEMENT_3D ( 'NONE', #35100, #7470, #9909 ) ;
#25085=ORIENTED_EDGE ( 'NONE', *, *, #23576, .T. ) ;
#25086=ORIENTED_EDGE ( 'NONE', *, *, #7808, .F. ) ;
#25088=CARTESIAN_POINT ( 'NONE',  ( 66.99999662536841072, 25.98076211353318854, -9.999999999999998224 ) ) ;
#25089=CARTESIAN_POINT ( 'NONE',  ( -81.86307664143558327, 18.04780306571548820, -5.000000000000000000 ) ) ;
#25090=VECTOR ( 'NONE', #8707, 1000.000000000000000 ) ;
#25092=CARTESIAN_POINT ( 'NONE',  ( -2.000003374631303732, -86.60254037844400443, 17.49999999999999645 ) ) ;
#25093=ADVANCED_FACE ( 'NONE', ( #27145 ), #13654, .F. ) ;
#25094=ORIENTED_EDGE ( 'NONE', *, *, #30701, .F. ) ;
#25095=ORIENTED_EDGE ( 'NONE', *, *, #1405, .F. ) ;
#25096=AXIS2_PLACEMENT_3D ( 'NONE', #8423, #28277, #28457 ) ;
#25098=EDGE_LOOP ( 'NONE', ( #34333, #26821 ) ) ;
#25099=CIRCLE ( 'NONE', #18503, 65.00000000000000000 ) ;
#25100=DIRECTION ( 'NONE',  ( 1.000000000000000000, 0.000000000000000000, 0.000000000000000000 ) ) ;
#25101=ORIENTED_EDGE ( 'NONE', *, *, #29216, .F. ) ;
#25102=FACE_BOUND ( 'NONE', #21626, .T. ) ;
#25103=CIRCLE ( 'NONE', #23916, 1.999999999999998224 ) ;
#25104=AXIS2_PLACEMENT_3D ( 'NONE', #29082, #14651, #21721 ) ;
#25105=DIRECTION ( 'NONE',  ( 0.000000000000000000, 0.000000000000000000, 1.000000000000000000 ) ) ;
#25106=CARTESIAN_POINT ( 'NONE',  ( -10.00000337463127842, -69.28203230275519786, -9.999999999999998224 ) ) ;
#25107=EDGE_LOOP ( 'NONE', ( #1635, #28612 ) ) ;
#25109=CARTESIAN_POINT ( 'NONE',  ( 52.99999662536844625, 60.62177826491077326, 12.50000000000000000 ) ) ;
#25110=CIRCLE ( 'NONE', #4739, 2.000000000000001776 ) ;
#25111=DIRECTION ( 'NONE',  ( 1.000000000000000000, 0.000000000000000000, 0.000000000000000000 ) ) ;
#25112=CARTESIAN_POINT ( 'NONE',  ( 69.99999662536841072, 51.96152422706640550, -9.999999999999998224 ) ) ;
#25113=EDGE_CURVE ( 'NONE', #7675, #22212, #15725, .T. ) ;
#25114=ORIENTED_EDGE ( 'NONE', *, *, #26435, .T. ) ;
#25115=CARTESIAN_POINT ( 'NONE',  ( 44.99999662536851019, -60.62177826491080168, 12.50000000000000000 ) ) ;
#25116=VECTOR ( 'NONE', #34194, 1000.000000000000000 ) ;
#25118=DIRECTION ( 'NONE',  ( 0.000000000000000000, 0.000000000000000000, 1.000000000000000000 ) ) ;
#25119=ORIENTED_EDGE ( 'NONE', *, *, #20778, .F. ) ;
#25121=AXIS2_PLACEMENT_3D ( 'NONE', #22683, #17242, #19011 ) ;
#25122=DIRECTION ( 'NONE',  ( 0.000000000000000000, 0.000000000000000000, 1.000000000000000000 ) ) ;
#25123=ORIENTED_EDGE ( 'NONE', *, *, #26567, .T. ) ;
#25124=CYLINDRICAL_SURFACE ( 'NONE', #22926, 2.000000000000001776 ) ;
#25125=DIRECTION ( 'NONE',  ( 0.000000000000000000, 0.000000000000000000, 1.000000000000000000 ) ) ;
#25126=AXIS2_PLACEMENT_3D ( 'NONE', #28801, #13994, #8747 ) ;
#25127=CARTESIAN_POINT ( 'NONE',  ( 76.99999662536836809, 43.30127018922198801, -5.000000000000000000 ) ) ;
#25128=AXIS2_PLACEMENT_3D ( 'NONE', #16107, #30534, #10103 ) ;
#25129=CARTESIAN_POINT ( 'NONE',  ( 66.99999662536839651, -60.62177826491080168, -9.999999999999998224 ) ) ;
#25130=CIRCLE ( 'NONE', #13738, 2.000000000000000000 ) ;
#25132=DIRECTION ( 'NONE',  ( 0.000000000000000000, 0.000000000000000000, 1.000000000000000000 ) ) ;
#25134=EDGE_CURVE ( 'NONE', #34700, #36279, #24553, .T. ) ;
#25135=CARTESIAN_POINT ( 'NONE',  ( -27.00000337463121625, -77.94228634059963667, -5.000000000000000000 ) ) ;
#25136=ORIENTED_EDGE ( 'NONE', *, *, #6005, .T. ) ;
#25137=ORIENTED_EDGE ( 'NONE', *, *, #35695, .F. ) ;
#25138=CIRCLE ( 'NONE', #13742, 2.000000000000001776 ) ;
#25139=DIRECTION ( 'NONE',  ( 0.000000000000000000, 0.000000000000000000, 1.000000000000000000 ) ) ;
#25140=LINE ( 'NONE', #36570, #36701 ) ;
#25143=EDGE_CURVE ( 'NONE', #1110, #36232, #10282, .T. ) ;
#25144=ORIENTED_EDGE ( 'NONE', *, *, #15845, .F. ) ;
#25145=AXIS2_PLACEMENT_3D ( 'NONE', #37092, #36893, #16657 ) ;
#25146=EDGE_CURVE ( 'NONE', #16685, #33091, #20949, .T. ) ;
#25148=ORIENTED_EDGE ( 'NONE', *, *, #4748, .F. ) ;
#25149=ORIENTED_EDGE ( 'NONE', *, *, #9686, .F. ) ;
#25150=CARTESIAN_POINT ( 'NONE',  ( 17.99999662536858835, 69.28203230275516944, -5.000000000000000000 ) ) ;
#25152=CIRCLE ( 'NONE', #29922, 2.000000000000001776 ) ;
#25153=DIRECTION ( 'NONE',  ( 0.000000000000000000, 0.000000000000000000, 1.000000000000000000 ) ) ;
#25154=DIRECTION ( 'NONE',  ( 0.000000000000000000, 0.000000000000000000, 1.000000000000000000 ) ) ;
#25155=AXIS2_PLACEMENT_3D ( 'NONE', #4056, #17940, #29368 ) ;
#25156=DIRECTION ( 'NONE',  ( -1.000000000000000000, 0.000000000000000000, 0.000000000000000000 ) ) ;
#25158=EDGE_CURVE ( 'NONE', #16300, #27851, #8378, .T. ) ;
#25159=ORIENTED_EDGE ( 'NONE', *, *, #29905, .F. ) ;
#25160=VERTEX_POINT ( 'NONE', #17010 ) ;
#25161=VECTOR ( 'NONE', #25328, 1000.000000000000000 ) ;
#25162=ORIENTED_EDGE ( 'NONE', *, *, #19451, .T. ) ;
#25163=EDGE_LOOP ( 'NONE', ( #30686, #13062 ) ) ;
#25164=CARTESIAN_POINT ( 'NONE',  ( -65.00000337463104927, -25.98076211353322051, 17.49999999999999645 ) ) ;
#25165=AXIS2_PLACEMENT_3D ( 'NONE', #1899, #13151, #33195 ) ;
#25166=LINE ( 'NONE', #36410, #17966 ) ;
#25167=VECTOR ( 'NONE', #27107, 1000.000000000000000 ) ;
#25168=DIRECTION ( 'NONE',  ( 1.000000000000000000, 0.000000000000000000, 0.000000000000000000 ) ) ;
#25169=FACE_OUTER_BOUND ( 'NONE', #20346, .T. ) ;
#25171=EDGE_LOOP ( 'NONE', ( #16058, #10433, #3748, #3290 ) ) ;
#25172=FACE_OUTER_BOUND ( 'NONE', #26922, .T. ) ;
#25173=EDGE_CURVE ( 'NONE', #16509, #28869, #10170, .T. ) ;
#25174=DIRECTION ( 'NONE',  ( 0.000000000000000000, 0.000000000000000000, -1.000000000000000000 ) ) ;
#25175=ADVANCED_FACE ( 'NONE', ( #13836 ), #22837, .F. ) ;
#25177=VERTEX_POINT ( 'NONE', #3135 ) ;
#25178=PLANE ( 'NONE',  #32204 ) ;
#25179=CARTESIAN_POINT ( 'NONE',  ( 59.99999662536842493, 51.96152422706639129, -9.999999999999998224 ) ) ;
#25180=AXIS2_PLACEMENT_3D ( 'NONE', #25311, #36194, #36576 ) ;
#25181=ORIENTED_EDGE ( 'NONE', *, *, #32520, .F. ) ;
#25183=DIRECTION ( 'NONE',  ( 0.000000000000000000, 0.000000000000000000, 1.000000000000000000 ) ) ;
#25185=AXIS2_PLACEMENT_3D ( 'NONE', #22890, #29043, #34709 ) ;
#25189=ORIENTED_EDGE ( 'NONE', *, *, #8887, .F. ) ;
#25191=LINE ( 'NONE', #10742, #33861 ) ;
#25192=EDGE_CURVE ( 'NONE', #8893, #4052, #11364, .T. ) ;
#25194=FACE_OUTER_BOUND ( 'NONE', #36742, .T. ) ;
#25195=VERTEX_POINT ( 'NONE', #31256 ) ;
#25197=CARTESIAN_POINT ( 'NONE',  ( 66.86787810013036903, -2.778182860042780700, 12.49999999999999645 ) ) ;
#25199=EDGE_LOOP ( 'NONE', ( #29287, #2140, #23365, #10540 ) ) ;
#25200=ORIENTED_EDGE ( 'NONE', *, *, #6232, .F. ) ;
#25201=DIRECTION ( 'NONE',  ( -0.000000000000000000, -0.000000000000000000, 1.000000000000000000 ) ) ;
#25202=DIRECTION ( 'NONE',  ( -1.000000000000000000, 0.000000000000000000, 0.000000000000000000 ) ) ;
#25203=DIRECTION ( 'NONE',  ( 0.000000000000000000, 0.000000000000000000, 1.000000000000000000 ) ) ;
#25204=FACE_OUTER_BOUND ( 'NONE', #13102, .T. ) ;
#25206=ORIENTED_EDGE ( 'NONE', *, *, #3350, .F. ) ;
#25207=FACE_OUTER_BOUND ( 'NONE', #31508, .T. ) ;
#25208=FACE_BOUND ( 'NONE', #3778, .T. ) ;
#25209=CARTESIAN_POINT ( 'NONE',  ( -35.00000337463116296, -60.62177826491080168, -9.999999999999998224 ) ) ;
#25210=DIRECTION ( 'NONE',  ( -0.8660254037844380415, 0.5000000000000009992, 0.000000000000000000 ) ) ;
#25212=DIRECTION ( 'NONE',  ( 1.000000000000000000, 0.000000000000000000, 0.000000000000000000 ) ) ;
#25213=EDGE_CURVE ( 'NONE', #4661, #19051, #13750, .T. ) ;
#25214=CARTESIAN_POINT ( 'NONE',  ( -32.16008401677955675, -61.25926521283091830, 12.49999999999999645 ) ) ;
#25215=EDGE_CURVE ( 'NONE', #18936, #10178, #2966, .T. ) ;
#25216=DIRECTION ( 'NONE',  ( 0.000000000000000000, 0.000000000000000000, 1.000000000000000000 ) ) ;
#25217=ORIENTED_EDGE ( 'NONE', *, *, #29961, .T. ) ;
#25218=DIRECTION ( 'NONE',  ( 0.000000000000000000, 0.000000000000000000, 1.000000000000000000 ) ) ;
#25219=DIRECTION ( 'NONE',  ( -0.8660254037844379305, 0.5000000000000011102, 0.000000000000000000 ) ) ;
#25220=DIRECTION ( 'NONE',  ( 0.000000000000000000, 0.000000000000000000, 1.000000000000000000 ) ) ;
#25221=ORIENTED_EDGE ( 'NONE', *, *, #29549, .T. ) ;
#25222=ORIENTED_EDGE ( 'NONE', *, *, #10515, .F. ) ;
#25223=ORIENTED_EDGE ( 'NONE', *, *, #30016, .T. ) ;
#25224=CARTESIAN_POINT ( 'NONE',  ( -4.220252828340121276, -79.78402168683115292, -5.000000000000000000 ) ) ;
#25226=VERTEX_POINT ( 'NONE', #26002 ) ;
#25227=DIRECTION ( 'NONE',  ( 1.000000000000000000, 0.000000000000000000, 0.000000000000000000 ) ) ;
#25228=EDGE_CURVE ( 'NONE', #7161, #20458, #28120, .T. ) ;
#25229=FACE_OUTER_BOUND ( 'NONE', #6975, .T. ) ;
#25230=ORIENTED_EDGE ( 'NONE', *, *, #3405, .T. ) ;
#25231=DIRECTION ( 'NONE',  ( 0.000000000000000000, 0.000000000000000000, 1.000000000000000000 ) ) ;
#25232=ORIENTED_EDGE ( 'NONE', *, *, #4365, .T. ) ;
#25233=CARTESIAN_POINT ( 'NONE',  ( 43.19957991610432657, 47.04203867989531318, 12.49999999999999822 ) ) ;
#25235=DIRECTION ( 'NONE',  ( 1.000000000000000000, 0.000000000000000000, 0.000000000000000000 ) ) ;
#25236=EDGE_LOOP ( 'NONE', ( #14348, #11325, #11598, #23604 ) ) ;
#25237=CARTESIAN_POINT ( 'NONE',  ( -33.00000337463116296, 77.94228634059957983, -9.999999999999998224 ) ) ;
#25238=CARTESIAN_POINT ( 'NONE',  ( 49.99999662536846756, 69.28203230275516944, -5.000000000000000000 ) ) ;
#25239=DIRECTION ( 'NONE',  ( 0.000000000000000000, 0.000000000000000000, 1.000000000000000000 ) ) ;
#25240=ADVANCED_FACE ( 'NONE', ( #20200 ), #16841, .F. ) ;
#25242=DIRECTION ( 'NONE',  ( 0.000000000000000000, 0.000000000000000000, 1.000000000000000000 ) ) ;
#25244=VERTEX_POINT ( 'NONE', #17393 ) ;
#25245=ADVANCED_FACE ( 'NONE', ( #11743 ), #30884, .F. ) ;
#25247=VECTOR ( 'NONE', #19684, 1000.000000000000000 ) ;
#25248=CARTESIAN_POINT ( 'NONE',  ( -85.00000337463092137, 25.98076211353317433, -5.000000000000000000 ) ) ;
#25249=CARTESIAN_POINT ( 'NONE',  ( 34.60911832077664485, -75.98085468209112037, -5.000000000000000000 ) ) ;
#25250=CARTESIAN_POINT ( 'NONE',  ( 7.999996625368618552, 69.28203230275516944, 12.50000000000000000 ) ) ;
#25251=EDGE_CURVE ( 'NONE', #34636, #13116, #34716, .T. ) ;
#25253=ORIENTED_EDGE ( 'NONE', *, *, #32048, .F. ) ;
#25256=CARTESIAN_POINT ( 'NONE',  ( 64.99999662536841072, 25.98076211353318854, -9.999999999999998224 ) ) ;
#25257=EDGE_CURVE ( 'NONE', #13225, #26423, #35343, .T. ) ;
#25259=ORIENTED_EDGE ( 'NONE', *, *, #9656, .T. ) ;
#25260=DIRECTION ( 'NONE',  ( 0.000000000000000000, 0.000000000000000000, 1.000000000000000000 ) ) ;
#25261=DIRECTION ( 'NONE',  ( -1.000000000000000000, 0.000000000000000000, 0.000000000000000000 ) ) ;
#25263=EDGE_CURVE ( 'NONE', #26293, #19500, #14368, .T. ) ;
#25266=EDGE_LOOP ( 'NONE', ( #1477, #27090, #21613, #47, #27509 ) ) ;
#25267=EDGE_CURVE ( 'NONE', #13323, #26293, #26941, .T. ) ;
#25269=CYLINDRICAL_SURFACE ( 'NONE', #21891, 1.999999999999998224 ) ;
#25271=EDGE_CURVE ( 'NONE', #33506, #32494, #31438, .T. ) ;
#25272=CARTESIAN_POINT ( 'NONE',  ( 34.99999662536855283, -60.62177826491080168, -9.999999999999998224 ) ) ;
#25273=ORIENTED_EDGE ( 'NONE', *, *, #27193, .T. ) ;
#25275=FACE_BOUND ( 'NONE', #30879, .T. ) ;
#25277=ORIENTED_EDGE ( 'NONE', *, *, #5859, .F. ) ;
#25279=DIRECTION ( 'NONE',  ( 0.000000000000000000, 0.000000000000000000, -1.000000000000000000 ) ) ;
#25281=CARTESIAN_POINT ( 'NONE',  ( 79.99999662536833966, 17.32050807568879236, -9.999999999999998224 ) ) ;
#25282=DIRECTION ( 'NONE',  ( 1.000000000000000000, 0.000000000000000000, 0.000000000000000000 ) ) ;
#25283=EDGE_LOOP ( 'NONE', ( #3934, #3680 ) ) ;
#25284=CARTESIAN_POINT ( 'NONE',  ( 64.99999662536839651, -43.30127018922199511, -9.999999999999998224 ) ) ;
#25285=DIRECTION ( 'NONE',  ( 0.000000000000000000, 0.000000000000000000, 1.000000000000000000 ) ) ;
#25286=LINE ( 'NONE', #36716, #14742 ) ;
#25287=ORIENTED_EDGE ( 'NONE', *, *, #2751, .F. ) ;
#25288=ORIENTED_EDGE ( 'NONE', *, *, #33626, .F. ) ;
#25290=DIRECTION ( 'NONE',  ( 1.000000000000000000, 0.000000000000000000, 0.000000000000000000 ) ) ;
#25291=ORIENTED_EDGE ( 'NONE', *, *, #18390, .F. ) ;
#25292=DIRECTION ( 'NONE',  ( -1.000000000000000000, 0.000000000000000000, 0.000000000000000000 ) ) ;
#25293=DIRECTION ( 'NONE',  ( 0.000000000000000000, 0.000000000000000000, -1.000000000000000000 ) ) ;
#25294=FACE_OUTER_BOUND ( 'NONE', #2836, .T. ) ;
#25298=CARTESIAN_POINT ( 'NONE',  ( -10.00000337463127842, -69.28203230275519786, 12.50000000000000000 ) ) ;
#25299=LINE ( 'NONE', #20226, #25658 ) ;
#25300=ORIENTED_EDGE ( 'NONE', *, *, #10347, .F. ) ;
#25301=VERTEX_POINT ( 'NONE', #12282 ) ;
#25303=CIRCLE ( 'NONE', #20487, 3.000000000000007550 ) ;
#25304=DIRECTION ( 'NONE',  ( 0.000000000000000000, 0.000000000000000000, 1.000000000000000000 ) ) ;
#25306=ADVANCED_FACE ( 'NONE', ( #21116 ), #35209, .F. ) ;
#25307=DIRECTION ( 'NONE',  ( 0.000000000000000000, 0.000000000000000000, 1.000000000000000000 ) ) ;
#25308=FACE_OUTER_BOUND ( 'NONE', #31651, .T. ) ;
#25310=PRODUCT_DEFINITION_CONTEXT ( 'detailed design', #8705, 'design' ) ;
#25311=CARTESIAN_POINT ( 'NONE',  ( 34.99999662536855283, -60.62177826491080168, -5.000000000000000000 ) ) ;
#25312=EDGE_LOOP ( 'NONE', ( #30770, #30613, #22392, #1900, #23890 ) ) ;
#25313=AXIS2_PLACEMENT_3D ( 'NONE', #20058, #22513, #5628 ) ;
#25314=ORIENTED_EDGE ( 'NONE', *, *, #6188, .F. ) ;
#25315=DIRECTION ( 'NONE',  ( 1.000000000000000000, 0.000000000000000000, 0.000000000000000000 ) ) ;
#25316=EDGE_LOOP ( 'NONE', ( #34915, #5409, #31026, #31550 ) ) ;
#25317=DIRECTION ( 'NONE',  ( 0.000000000000000000, 0.000000000000000000, 1.000000000000000000 ) ) ;
#25318=LINE ( 'NONE', #31128, #32591 ) ;
#25320=EDGE_LOOP ( 'NONE', ( #24222, #32919 ) ) ;
#25323=ORIENTED_EDGE ( 'NONE', *, *, #29359, .F. ) ;
#25324=EDGE_CURVE ( 'NONE', #17904, #21445, #1788, .T. ) ;
#25325=EDGE_LOOP ( 'NONE', ( #1113, #15066, #32905, #8100 ) ) ;
#25326=VERTEX_POINT ( 'NONE', #18115 ) ;
#25328=DIRECTION ( 'NONE',  ( 0.000000000000000000, 0.000000000000000000, 1.000000000000000000 ) ) ;
#25329=CARTESIAN_POINT ( 'NONE',  ( 74.99999662536836809, 43.30127018922198801, -9.999999999999998224 ) ) ;
#25330=CARTESIAN_POINT ( 'NONE',  ( -77.00000337463097821, 25.98076211353318854, 17.49999999999999645 ) ) ;
#25333=VERTEX_POINT ( 'NONE', #26383 ) ;
#25335=DIRECTION ( 'NONE',  ( -1.000000000000000000, 0.000000000000000000, 0.000000000000000000 ) ) ;
#25336=ADVANCED_FACE ( 'NONE', ( #6129 ), #29732, .F. ) ;
#25337=AXIS2_PLACEMENT_3D ( 'NONE', #6829, #17913, #35171 ) ;
#25338=DIRECTION ( 'NONE',  ( -1.000000000000000000, 0.000000000000000000, 0.000000000000000000 ) ) ;
#25342=EDGE_LOOP ( 'NONE', ( #15139, #730 ) ) ;
#25343=VERTEX_POINT ( 'NONE', #32176 ) ;
#25344=CARTESIAN_POINT ( 'NONE',  ( 58.88972745734226066, 33.99999999999924682, 12.49999999999999822 ) ) ;
#25346=EDGE_CURVE ( 'NONE', #17463, #1110, #572, .T. ) ;
#25347=CARTESIAN_POINT ( 'NONE',  ( 74.99999662536836809, 8.660254037844394404, 17.49999999999999645 ) ) ;
#25350=EDGE_LOOP ( 'NONE', ( #27974, #24568 ) ) ;
#25352=DIRECTION ( 'NONE',  ( 0.000000000000000000, 0.000000000000000000, 1.000000000000000000 ) ) ;
#25354=VERTEX_POINT ( 'NONE', #3863 ) ;
#25355=DIRECTION ( 'NONE',  ( 0.000000000000000000, 0.000000000000000000, 1.000000000000000000 ) ) ;
#25356=EDGE_LOOP ( 'NONE', ( #372, #35399, #33142, #24749, #4932 ) ) ;
#25358=CIRCLE ( 'NONE', #16978, 2.000000000000001776 ) ;
#25359=CARTESIAN_POINT ( 'NONE',  ( 61.25926521283100357, -32.16008401677932227, -4.999999999999997335 ) ) ;
#25361=EDGE_CURVE ( 'NONE', #5647, #21660, #20944, .T. ) ;
#25362=DIRECTION ( 'NONE',  ( 1.000000000000000000, 0.000000000000000000, 0.000000000000000000 ) ) ;
#25364=VERTEX_POINT ( 'NONE', #4067 ) ;
#25366=LINE ( 'NONE', #1933, #5197 ) ;
#25367=EDGE_CURVE ( 'NONE', #36567, #21017, #16167, .T. ) ;
#25368=AXIS2_PLACEMENT_3D ( 'NONE', #25979, #3114, #11366 ) ;
#25369=DIRECTION ( 'NONE',  ( 0.000000000000000000, 0.000000000000000000, 1.000000000000000000 ) ) ;
#25370=DIRECTION ( 'NONE',  ( 0.000000000000000000, 0.000000000000000000, 1.000000000000000000 ) ) ;
#25371=ORIENTED_EDGE ( 'NONE', *, *, #16979, .T. ) ;
#25372=CARTESIAN_POINT ( 'NONE',  ( 44.99999662536849598, 60.62177826491077326, 12.50000000000000000 ) ) ;
#25373=FACE_BOUND ( 'NONE', #17678, .T. ) ;
#25375=DIRECTION ( 'NONE',  ( -1.000000000000000000, 0.000000000000000000, 0.000000000000000000 ) ) ;
#25376=VECTOR ( 'NONE', #21616, 1000.000000000000000 ) ;
#25378=DIRECTION ( 'NONE',  ( 0.000000000000000000, 0.000000000000000000, 1.000000000000000000 ) ) ;
#25379=FACE_OUTER_BOUND ( 'NONE', #9623, .T. ) ;
#25380=DIRECTION ( 'NONE',  ( 0.000000000000000000, 0.000000000000000000, 1.000000000000000000 ) ) ;
#25381=EDGE_CURVE ( 'NONE', #18749, #11572, #17747, .T. ) ;
#25382=DIRECTION ( 'NONE',  ( 0.000000000000000000, 0.000000000000000000, 1.000000000000000000 ) ) ;
#25383=ORIENTED_EDGE ( 'NONE', *, *, #21563, .F. ) ;
#25384=CYLINDRICAL_SURFACE ( 'NONE', #26224, 2.000000000000001776 ) ;
#25386=CARTESIAN_POINT ( 'NONE',  ( 2.778182860043481028, 66.86787810013034061, -49.86348611802629449 ) ) ;
#25387=CIRCLE ( 'NONE', #21788, 2.000000000000001776 ) ;
#25389=ORIENTED_EDGE ( 'NONE', *, *, #1887, .T. ) ;
#25390=ORIENTED_EDGE ( 'NONE', *, *, #1879, .T. ) ;
#25392=LINE ( 'NONE', #20129, #14149 ) ;
#25394=VERTEX_POINT ( 'NONE', #9692 ) ;
#25395=CARTESIAN_POINT ( 'NONE',  ( 27.78182860042856461, 56.67878100130339902, -4.999999999999997335 ) ) ;
#25400=CARTESIAN_POINT ( 'NONE',  ( 56.67878100130369035, -27.78182860042797131, 12.49999999999999822 ) ) ;
#25401=ORIENTED_EDGE ( 'NONE', *, *, #13618, .F. ) ;
#25402=ADVANCED_FACE ( 'NONE', ( #23394 ), #9302, .F. ) ;
#25403=AXIS2_PLACEMENT_3D ( 'NONE', #34429, #26362, #29353 ) ;
#25404=CARTESIAN_POINT ( 'NONE',  ( -37.00000337463117717, -77.94228634059963667, 17.49999999999999645 ) ) ;
#25406=ADVANCED_FACE ( 'NONE', ( #864 ), #29184, .F. ) ;
#25407=ORIENTED_EDGE ( 'NONE', *, *, #10744, .T. ) ;
#25409=VECTOR ( 'NONE', #7158, 1000.000000000000000 ) ;
#25410=CARTESIAN_POINT ( 'NONE',  ( -2.778182860042080815, 69.13212189986968781, -49.86348611802629449 ) ) ;
#25411=DIRECTION ( 'NONE',  ( 0.000000000000000000, 0.000000000000000000, 1.000000000000000000 ) ) ;
#25412=ORIENTED_EDGE ( 'NONE', *, *, #11161, .F. ) ;
#25413=CARTESIAN_POINT ( 'NONE',  ( 82.99999662536832545, 25.98076211353319565, -5.000000000000000000 ) ) ;
#25414=CARTESIAN_POINT ( 'NONE',  ( -82.00000337463094979, -2.404119930384582903E-14, 12.50000000000000000 ) ) ;
#25415=ORIENTED_EDGE ( 'NONE', *, *, #7122, .F. ) ;
#25416=CARTESIAN_POINT ( 'NONE',  ( -45.00000000000000711, 5.510910596163090344E-15, -5.000000000000000000 ) ) ;
#25417=FACE_OUTER_BOUND ( 'NONE', #7734, .T. ) ;
#25419=DIRECTION ( 'NONE',  ( 1.000000000000000000, 0.000000000000000000, 0.000000000000000000 ) ) ;
#25420=ORIENTED_EDGE ( 'NONE', *, *, #13830, .T. ) ;
#25421=EDGE_CURVE ( 'NONE', #8381, #34620, #30562, .T. ) ;
#25423=VECTOR ( 'NONE', #30156, 1000.000000000000000 ) ;
#25424=DIRECTION ( 'NONE',  ( 0.000000000000000000, 0.000000000000000000, 1.000000000000000000 ) ) ;
#25425=DIRECTION ( 'NONE',  ( 0.000000000000000000, 0.000000000000000000, -1.000000000000000000 ) ) ;
#25426=CIRCLE ( 'NONE', #9246, 2.000000000000001776 ) ;
#25428=ORIENTED_EDGE ( 'NONE', *, *, #28365, .T. ) ;
#25429=DIRECTION ( 'NONE',  ( 1.000000000000000000, 0.000000000000000000, 0.000000000000000000 ) ) ;
#25432=VERTEX_POINT ( 'NONE', #15120 ) ;
#25435=ORIENTED_EDGE ( 'NONE', *, *, #1632, .F. ) ;
#25436=ADVANCED_FACE ( 'NONE', ( #26553 ), #7251, .F. ) ;
#25438=DIRECTION ( 'NONE',  ( -1.000000000000000000, 0.000000000000000000, 0.000000000000000000 ) ) ;
#25439=EDGE_LOOP ( 'NONE', ( #19003, #30937 ) ) ;
#25440=EDGE_CURVE ( 'NONE', #2698, #6733, #11388, .T. ) ;
#25441=DIRECTION ( 'NONE',  ( 0.000000000000000000, 0.000000000000000000, 1.000000000000000000 ) ) ;
#25442=EDGE_LOOP ( 'NONE', ( #15731, #17641, #19258, #6742 ) ) ;
#25443=FACE_BOUND ( 'NONE', #11492, .T. ) ;
#25445=CARTESIAN_POINT ( 'NONE',  ( 11.99999662536865763, -69.28203230275519786, -9.999999999999998224 ) ) ;
#25446=AXIS2_PLACEMENT_3D ( 'NONE', #12275, #299, #34646 ) ;
#25447=EDGE_CURVE ( 'NONE', #11341, #7750, #8982, .T. ) ;
#25448=VERTEX_POINT ( 'NONE', #27841 ) ;
#25449=EDGE_CURVE ( 'NONE', #26021, #33148, #4204, .T. ) ;
#25452=CYLINDRICAL_SURFACE ( 'NONE', #33843, 27.00000000000001421 ) ;
#25454=DIRECTION ( 'NONE',  ( 1.000000000000000000, 0.000000000000000000, 0.000000000000000000 ) ) ;
#25455=EDGE_LOOP ( 'NONE', ( #35580, #330, #25821 ) ) ;
#25456=CARTESIAN_POINT ( 'NONE',  ( -3.374631289687624047E-06, -69.28203230275519786, -9.999999999999998224 ) ) ;
#25457=DIRECTION ( 'NONE',  ( -0.000000000000000000, -0.000000000000000000, 1.000000000000000000 ) ) ;
#25458=DIRECTION ( 'NONE',  ( 1.000000000000000000, 0.000000000000000000, 0.000000000000000000 ) ) ;
#25459=EDGE_CURVE ( 'NONE', #21147, #7638, #4983, .T. ) ;
#25461=AXIS2_PLACEMENT_3D ( 'NONE', #28770, #33546, #18904 ) ;
#25462=EDGE_CURVE ( 'NONE', #16077, #26898, #1980, .T. ) ;
#25465=ADVANCED_FACE ( 'NONE', ( #10067 ), #21676, .T. ) ;
#25466=EDGE_LOOP ( 'NONE', ( #16528, #9767 ) ) ;
#25467=EDGE_CURVE ( 'NONE', #12814, #25033, #2408, .T. ) ;
#25468=CARTESIAN_POINT ( 'NONE',  ( 79.99999662536833966, -3.469446951953614189E-15, -9.999999999999998224 ) ) ;
#25469=CARTESIAN_POINT ( 'NONE',  ( 93.60231327712337190, 15.97563234535636134, -4.999999999999997335 ) ) ;
#25470=DIRECTION ( 'NONE',  ( 0.000000000000000000, 0.000000000000000000, 1.000000000000000000 ) ) ;
#25471=AXIS2_PLACEMENT_3D ( 'NONE', #7974, #11149, #10798 ) ;
#25475=VECTOR ( 'NONE', #30249, 1000.000000000000000 ) ;
#25476=CARTESIAN_POINT ( 'NONE',  ( -37.00000337463116296, 77.94228634059957983, -9.999999999999998224 ) ) ;
#25477=CIRCLE ( 'NONE', #23681, 3.000000000000002665 ) ;
#25479=CIRCLE ( 'NONE', #8108, 2.000000000000001776 ) ;
#25481=AXIS2_PLACEMENT_3D ( 'NONE', #4654, #27689, #12875 ) ;
#25482=ORIENTED_EDGE ( 'NONE', *, *, #5032, .F. ) ;
#25484=CARTESIAN_POINT ( 'NONE',  ( 21.99999662536862033, -69.28203230275519786, -9.999999999999998224 ) ) ;
#25485=DIRECTION ( 'NONE',  ( -1.000000000000000000, 0.000000000000000000, 0.000000000000000000 ) ) ;
#25486=CARTESIAN_POINT ( 'NONE',  ( -20.00000337463123756, -69.28203230275522628, -9.999999999999998224 ) ) ;
#25487=ORIENTED_EDGE ( 'NONE', *, *, #32078, .F. ) ;
#25488=CIRCLE ( 'NONE', #27271, 3.499999999999989342 ) ;
#25489=AXIS2_PLACEMENT_3D ( 'NONE', #35017, #21131, #17961 ) ;
#25490=FACE_BOUND ( 'NONE', #19154, .T. ) ;
#25491=EDGE_LOOP ( 'NONE', ( #29429, #19801, #4236, #8045, #2389 ) ) ;
#25492=ORIENTED_EDGE ( 'NONE', *, *, #7815, .F. ) ;
#25496=LINE ( 'NONE', #2261, #23184 ) ;
#25497=CYLINDRICAL_SURFACE ( 'NONE', #20043, 2.000000000000001776 ) ;
#25498=AXIS2_PLACEMENT_3D ( 'NONE', #31004, #11315, #33815 ) ;
#25499=CARTESIAN_POINT ( 'NONE',  ( -73.00000337463097821, 8.660254037844374864, -5.000000000000000000 ) ) ;
#25500=EDGE_LOOP ( 'NONE', ( #9880, #14303 ) ) ;
#25501=AXIS2_PLACEMENT_3D ( 'NONE', #36598, #33968, #27955 ) ;
#25502=VERTEX_POINT ( 'NONE', #30664 ) ;
#25504=AXIS2_PLACEMENT_3D ( 'NONE', #9387, #18019, #29441 ) ;
#25505=ORIENTED_EDGE ( 'NONE', *, *, #29918, .F. ) ;
#25506=AXIS2_PLACEMENT_3D ( 'NONE', #24491, #19400, #5155 ) ;
#25508=ORIENTED_EDGE ( 'NONE', *, *, #21686, .T. ) ;
#25509=AXIS2_PLACEMENT_3D ( 'NONE', #6313, #2774, #8956 ) ;
#25511=EDGE_CURVE ( 'NONE', #1584, #34250, #27494, .T. ) ;
#25512=CARTESIAN_POINT ( 'NONE',  ( -63.00000337463104927, -43.30127018922202353, -9.999999999999998224 ) ) ;
#25513=ADVANCED_FACE ( 'NONE', ( #7813, #10247, #19249, #19069, #16251, #16420, #12669, #9861, #21301 ), #18868, .F. ) ;
#25514=DIRECTION ( 'NONE',  ( 0.000000000000000000, 0.000000000000000000, -1.000000000000000000 ) ) ;
#25515=CARTESIAN_POINT ( 'NONE',  ( 31.99999662536857770, -69.28203230275519786, -9.999999999999998224 ) ) ;
#25516=FACE_OUTER_BOUND ( 'NONE', #17796, .T. ) ;
#25517=ORIENTED_EDGE ( 'NONE', *, *, #3511, .F. ) ;
#25518=DIRECTION ( 'NONE',  ( 0.000000000000000000, 0.000000000000000000, 1.000000000000000000 ) ) ;
#25519=AXIS2_PLACEMENT_3D ( 'NONE', #10239, #35935, #24287 ) ;
#25520=DIRECTION ( 'NONE',  ( 1.000000000000000000, 0.000000000000000000, 0.000000000000000000 ) ) ;
#25521=DIRECTION ( 'NONE',  ( 0.000000000000000000, 0.000000000000000000, 1.000000000000000000 ) ) ;
#25526=AXIS2_PLACEMENT_3D ( 'NONE', #18076, #8907, #9649 ) ;
#25527=ORIENTED_EDGE ( 'NONE', *, *, #27978, .T. ) ;
#25531=DIRECTION ( 'NONE',  ( 0.000000000000000000, 0.000000000000000000, 1.000000000000000000 ) ) ;
#25532=CYLINDRICAL_SURFACE ( 'NONE', #17881, 2.000000000000001776 ) ;
#25535=VERTEX_POINT ( 'NONE', #30495 ) ;
#25536=CIRCLE ( 'NONE', #9353, 1.999999999999998224 ) ;
#25537=CIRCLE ( 'NONE', #30318, 2.000000000000001776 ) ;
#25539=AXIS2_PLACEMENT_3D ( 'NONE', #4182, #35671, #32654 ) ;
#25540=FACE_OUTER_BOUND ( 'NONE', #8265, .T. ) ;
#25541=AXIS2_PLACEMENT_3D ( 'NONE', #23012, #28443, #14399 ) ;
#25542=ORIENTED_EDGE ( 'NONE', *, *, #12613, .T. ) ;
#25546=AXIS2_PLACEMENT_3D ( 'NONE', #10196, #21058, #12614 ) ;
#25548=CARTESIAN_POINT ( 'NONE',  ( 72.99999662536835388, -43.30127018922199511, 17.49999999999999645 ) ) ;
#25549=CARTESIAN_POINT ( 'NONE',  ( 66.99999662536841072, 25.98076211353318854, -5.000000000000000000 ) ) ;
#25550=VERTEX_POINT ( 'NONE', #35754 ) ;
#25551=ORIENTED_EDGE ( 'NONE', *, *, #30701, .T. ) ;
#25552=DIRECTION ( 'NONE',  ( 1.000000000000000000, 0.000000000000000000, 0.000000000000000000 ) ) ;
#25553=CARTESIAN_POINT ( 'NONE',  ( 67.99999662536838230, 34.64101615137758472, -5.000000000000000000 ) ) ;
#25556=CARTESIAN_POINT ( 'NONE',  ( -10.00000337463128730, 69.28203230275516944, -9.999999999999998224 ) ) ;
#25557=AXIS2_PLACEMENT_3D ( 'NONE', #22667, #34800, #22117 ) ;
#25558=EDGE_LOOP ( 'NONE', ( #28126, #2719, #3701, #35761 ) ) ;
#25560=EDGE_CURVE ( 'NONE', #23471, #31151, #4819, .T. ) ;
#25561=FACE_BOUND ( 'NONE', #8312, .T. ) ;
#25564=FACE_OUTER_BOUND ( 'NONE', #28575, .T. ) ;
#25565=CARTESIAN_POINT ( 'NONE',  ( 0.000000000000000000, 0.000000000000000000, -5.000000000000000000 ) ) ;
#25566=AXIS2_PLACEMENT_3D ( 'NONE', #10980, #5187, #103 ) ;
#25567=FACE_OUTER_BOUND ( 'NONE', #19420, .T. ) ;
#25568=AXIS2_PLACEMENT_3D ( 'NONE', #28867, #25887, #20812 ) ;
#25569=AXIS2_PLACEMENT_3D ( 'NONE', #2380, #13411, #16257 ) ;
#25575=DIRECTION ( 'NONE',  ( -0.000000000000000000, -0.000000000000000000, 1.000000000000000000 ) ) ;
#25576=ORIENTED_EDGE ( 'NONE', *, *, #28846, .T. ) ;
#25577=CIRCLE ( 'NONE', #30355, 33.00000000000001421 ) ;
#25578=VERTEX_POINT ( 'NONE', #24509 ) ;
#25579=ORIENTED_EDGE ( 'NONE', *, *, #15861, .F. ) ;
#25580=ADVANCED_FACE ( 'NONE', ( #35950 ), #13608, .F. ) ;
#25581=CARTESIAN_POINT ( 'NONE',  ( -65.00000337463102085, 43.30127018922198801, 17.49999999999999645 ) ) ;
#25583=ORIENTED_EDGE ( 'NONE', *, *, #26774, .F. ) ;
#25584=AXIS2_PLACEMENT_3D ( 'NONE', #24128, #24514, #35955 ) ;
#25586=ADVANCED_FACE ( 'NONE', ( #5542 ), #33675, .F. ) ;
#25587=AXIS2_PLACEMENT_3D ( 'NONE', #33025, #6963, #4729 ) ;
#25589=CIRCLE ( 'NONE', #9407, 2.000000000000000000 ) ;
#25590=ORIENTED_EDGE ( 'NONE', *, *, #25271, .T. ) ;
#25591=DIRECTION ( 'NONE',  ( 0.8660254037844415942, 0.4999999999999949485, 0.000000000000000000 ) ) ;
#25592=EDGE_CURVE ( 'NONE', #15444, #34250, #32345, .T. ) ;
#25593=ORIENTED_EDGE ( 'NONE', *, *, #9041, .F. ) ;
#25594=FACE_OUTER_BOUND ( 'NONE', #30270, .T. ) ;
#25596=ORIENTED_EDGE ( 'NONE', *, *, #30556, .T. ) ;
#25597=CIRCLE ( 'NONE', #22003, 2.000000000000000000 ) ;
#25598=ORIENTED_EDGE ( 'NONE', *, *, #1873, .F. ) ;
#25599=AXIS2_PLACEMENT_3D ( 'NONE', #20609, #35069, #3193 ) ;
#25600=CIRCLE ( 'NONE', #27383, 3.000000000000007994 ) ;
#25602=DIRECTION ( 'NONE',  ( 1.000000000000000000, 0.000000000000000000, 0.000000000000000000 ) ) ;
#25603=CARTESIAN_POINT ( 'NONE',  ( 58.88972745734226066, 33.99999999999924682, -4.999999999999997335 ) ) ;
#25609=CARTESIAN_POINT ( 'NONE',  ( 16.99999662536863454, -77.94228634059960825, -9.999999999999998224 ) ) ;
#25611=DIRECTION ( 'NONE',  ( 0.000000000000000000, 0.000000000000000000, 1.000000000000000000 ) ) ;
#25612=CIRCLE ( 'NONE', #2263, 2.000000000000001776 ) ;
#25613=DIRECTION ( 'NONE',  ( 0.000000000000000000, 0.000000000000000000, 1.000000000000000000 ) ) ;
#25615=ADVANCED_FACE ( 'NONE', ( #19971 ), #36848, .F. ) ;
#25616=CARTESIAN_POINT ( 'NONE',  ( -73.00000337463097821, 25.98076211353318854, -5.000000000000000000 ) ) ;
#25617=AXIS2_PLACEMENT_3D ( 'NONE', #5944, #20177, #31605 ) ;
#25618=VECTOR ( 'NONE', #1769, 1000.000000000000000 ) ;
#25620=DIRECTION ( 'NONE',  ( 1.000000000000000000, 0.000000000000000000, 0.000000000000000000 ) ) ;
#25621=DIRECTION ( 'NONE',  ( 0.000000000000000000, 0.000000000000000000, 1.000000000000000000 ) ) ;
#25622=AXIS2_PLACEMENT_3D ( 'NONE', #5497, #2876, #23296 ) ;
#25623=VERTEX_POINT ( 'NONE', #25413 ) ;
#25624=AXIS2_PLACEMENT_3D ( 'NONE', #24049, #23667, #34926 ) ;
#25625=ORIENTED_EDGE ( 'NONE', *, *, #35966, .F. ) ;
#25627=DIRECTION ( 'NONE',  ( 0.000000000000000000, 0.000000000000000000, 1.000000000000000000 ) ) ;
#25628=EDGE_CURVE ( 'NONE', #25733, #20787, #5408, .T. ) ;
#25630=VECTOR ( 'NONE', #26885, 1000.000000000000000 ) ;
#25632=ORIENTED_EDGE ( 'NONE', *, *, #14156, .T. ) ;
#25633=EDGE_CURVE ( 'NONE', #30803, #14051, #10195, .T. ) ;
#25635=DIRECTION ( 'NONE',  ( 1.000000000000000000, 0.000000000000000000, 0.000000000000000000 ) ) ;
#25636=LINE ( 'NONE', #28415, #17051 ) ;
#25639=ORIENTED_EDGE ( 'NONE', *, *, #31286, .F. ) ;
#25640=CARTESIAN_POINT ( 'NONE',  ( 72.99999662536836809, 25.98076211353319565, -9.999999999999998224 ) ) ;
#25641=CIRCLE ( 'NONE', #9469, 27.00000000000001421 ) ;
#25642=CARTESIAN_POINT ( 'NONE',  ( 47.63139720814418610, 27.49999999999988987, -10.00000000000000000 ) ) ;
#25643=ORIENTED_EDGE ( 'NONE', *, *, #35554, .T. ) ;
#25645=EDGE_CURVE ( 'NONE', #23444, #13165, #35954, .T. ) ;
#25646=ORIENTED_EDGE ( 'NONE', *, *, #7594, .F. ) ;
#25647=CIRCLE ( 'NONE', #5888, 2.000000000000000000 ) ;
#25648=CIRCLE ( 'NONE', #26808, 2.000000000000001776 ) ;
#25649=FACE_BOUND ( 'NONE', #5262, .T. ) ;
#25650=AXIS2_PLACEMENT_3D ( 'NONE', #7256, #36122, #6868 ) ;
#25651=EDGE_CURVE ( 'NONE', #34636, #22817, #34157, .T. ) ;
#25652=AXIS2_PLACEMENT_3D ( 'NONE', #11612, #28507, #36969 ) ;
#25654=CARTESIAN_POINT ( 'NONE',  ( -18.00000337463123046, 86.60254037844397601, -9.999999999999998224 ) ) ;
#25655=ORIENTED_EDGE ( 'NONE', *, *, #121, .F. ) ;
#25657=CARTESIAN_POINT ( 'NONE',  ( -27.78182860042817026, -56.67878100130359087, -49.86348611802629449 ) ) ;
#25658=VECTOR ( 'NONE', #10863, 1000.000000000000000 ) ;
#25659=CARTESIAN_POINT ( 'NONE',  ( 0.000000000000000000, 0.000000000000000000, 12.49999999999999822 ) ) ;
#25660=FACE_OUTER_BOUND ( 'NONE', #11657, .T. ) ;
#25661=ORIENTED_EDGE ( 'NONE', *, *, #36488, .T. ) ;
#25662=CYLINDRICAL_SURFACE ( 'NONE', #20849, 2.000000000000000000 ) ;
#25663=DIRECTION ( 'NONE',  ( 1.000000000000000000, 0.000000000000000000, 0.000000000000000000 ) ) ;
#25664=CARTESIAN_POINT ( 'NONE',  ( 81.99999662536833966, 17.32050807568879236, 17.49999999999999645 ) ) ;
#25665=ORIENTED_EDGE ( 'NONE', *, *, #30818, .F. ) ;
#25666=EDGE_CURVE ( 'NONE', #19051, #17303, #1560, .T. ) ;
#25667=ORIENTED_EDGE ( 'NONE', *, *, #7377, .T. ) ;
#25668=AXIS2_PLACEMENT_3D ( 'NONE', #28299, #22696, #34145 ) ;
#25670=CARTESIAN_POINT ( 'NONE',  ( 51.99999662536847467, -69.28203230275519786, 17.49999999999999645 ) ) ;
#25671=CIRCLE ( 'NONE', #36958, 2.000000000000001776 ) ;
#25673=PLANE ( 'NONE',  #24617 ) ;
#25674=AXIS2_PLACEMENT_3D ( 'NONE', #36562, #8038, #20023 ) ;
#25676=ADVANCED_FACE ( 'NONE', ( #8171 ), #31224, .F. ) ;
#25679=EDGE_CURVE ( 'NONE', #23569, #33068, #20112, .T. ) ;
#25680=CARTESIAN_POINT ( 'NONE',  ( 71.99999662536838230, -51.96152422706639840, -9.999999999999998224 ) ) ;
#25681=DIRECTION ( 'NONE',  ( 3.469446951953612611E-15, 1.000000000000000000, 0.000000000000000000 ) ) ;
#25682=ORIENTED_EDGE ( 'NONE', *, *, #10293, .F. ) ;
#25684=AXIS2_PLACEMENT_3D ( 'NONE', #1563, #4575, #2117 ) ;
#25686=DIRECTION ( 'NONE',  ( -1.000000000000000000, 0.000000000000000000, 0.000000000000000000 ) ) ;
#25687=DIRECTION ( 'NONE',  ( 1.000000000000000000, 0.000000000000000000, 0.000000000000000000 ) ) ;
#25688=DIRECTION ( 'NONE',  ( 0.000000000000000000, 0.000000000000000000, 1.000000000000000000 ) ) ;
#25690=ADVANCED_FACE ( 'NONE', ( #25801 ), #93, .F. ) ;
#25691=FACE_BOUND ( 'NONE', #18912, .T. ) ;
#25692=CIRCLE ( 'NONE', #1753, 2.000000000000001776 ) ;
#25693=EDGE_LOOP ( 'NONE', ( #19289, #13187 ) ) ;
#25694=ORIENTED_EDGE ( 'NONE', *, *, #19768, .T. ) ;
#25695=CARTESIAN_POINT ( 'NONE',  ( 62.19434990244977257, -52.39915983220758022, 12.49999999999999822 ) ) ;
#25696=VERTEX_POINT ( 'NONE', #8368 ) ;
#25697=LINE ( 'NONE', #19325, #5230 ) ;
#25699=CARTESIAN_POINT ( 'NONE',  ( 47.99999662536848177, -51.96152422706640550, -5.000000000000000000 ) ) ;
#25700=AXIS2_PLACEMENT_3D ( 'NONE', #14509, #632, #25947 ) ;
#25701=ORIENTED_EDGE ( 'NONE', *, *, #36244, .T. ) ;
#25703=CIRCLE ( 'NONE', #29269, 33.00000000000001421 ) ;
#25704=ORIENTED_EDGE ( 'NONE', *, *, #25462, .T. ) ;
#25705=VERTEX_POINT ( 'NONE', #16970 ) ;
#25706=CIRCLE ( 'NONE', #9533, 2.000000000000001776 ) ;
#25708=ORIENTED_EDGE ( 'NONE', *, *, #8399, .F. ) ;
#25709=CARTESIAN_POINT ( 'NONE',  ( -35.83991598322101879, -56.52018970185248037, -4.999999999999997335 ) ) ;
#25710=DIRECTION ( 'NONE',  ( 1.000000000000000000, 0.000000000000000000, 0.000000000000000000 ) ) ;
#25711=EDGE_CURVE ( 'NONE', #6793, #14173, #15945, .T. ) ;
#25712=DIRECTION ( 'NONE',  ( 0.000000000000000000, 0.000000000000000000, -1.000000000000000000 ) ) ;
#25713=DIRECTION ( 'NONE',  ( 0.000000000000000000, 0.000000000000000000, 1.000000000000000000 ) ) ;
#25715=ORIENTED_EDGE ( 'NONE', *, *, #5056, .T. ) ;
#25716=CARTESIAN_POINT ( 'NONE',  ( 62.99999662536841072, -25.98076211353320275, -9.999999999999998224 ) ) ;
#25717=EDGE_CURVE ( 'NONE', #8910, #8894, #29679, .T. ) ;
#25718=CARTESIAN_POINT ( 'NONE',  ( -65.00000337463104927, -25.98076211353322051, -5.000000000000000000 ) ) ;
#25719=AXIS2_PLACEMENT_3D ( 'NONE', #24510, #9511, #15688 ) ;
#25720=CYLINDRICAL_SURFACE ( 'NONE', #21176, 2.000000000000001776 ) ;
#25723=ADVANCED_FACE ( 'NONE', ( #457 ), #25965, .F. ) ;
#25724=DIRECTION ( 'NONE',  ( 1.000000000000000000, 0.000000000000000000, 0.000000000000000000 ) ) ;
#25725=ADVANCED_FACE ( 'NONE', ( #3821 ), #32128, .F. ) ;
#25726=ORIENTED_EDGE ( 'NONE', *, *, #13044, .T. ) ;
#25727=EDGE_LOOP ( 'NONE', ( #11375, #27872 ) ) ;
#25728=DIRECTION ( 'NONE',  ( 1.000000000000000000, 0.000000000000000000, 0.000000000000000000 ) ) ;
#25729=DIRECTION ( 'NONE',  ( 0.000000000000000000, 0.000000000000000000, -1.000000000000000000 ) ) ;
#25730=DIRECTION ( 'NONE',  ( -1.000000000000000000, 0.000000000000000000, 0.000000000000000000 ) ) ;
#25731=FACE_OUTER_BOUND ( 'NONE', #5118, .T. ) ;
#25732=ORIENTED_EDGE ( 'NONE', *, *, #22714, .F. ) ;
#25733=VERTEX_POINT ( 'NONE', #266 ) ;
#25734=AXIS2_PLACEMENT_3D ( 'NONE', #35392, #9498, #26181 ) ;
#25735=EDGE_CURVE ( 'NONE', #25705, #11344, #28510, .T. ) ;
#25736=CYLINDRICAL_SURFACE ( 'NONE', #35665, 2.000000000000001776 ) ;
#25737=ADVANCED_FACE ( 'NONE', ( #9467 ), #6267, .F. ) ;
#25740=EDGE_CURVE ( 'NONE', #25696, #5023, #3100, .T. ) ;
#25741=VERTEX_POINT ( 'NONE', #34606 ) ;
#25742=EDGE_CURVE ( 'NONE', #13541, #12539, #2776, .T. ) ;
#25744=CIRCLE ( 'NONE', #14969, 95.00000000000000000 ) ;
#25745=ORIENTED_EDGE ( 'NONE', *, *, #8694, .F. ) ;
#25747=DIRECTION ( 'NONE',  ( -1.000000000000000000, 0.000000000000000000, 0.000000000000000000 ) ) ;
#25748=CYLINDRICAL_SURFACE ( 'NONE', #5290, 33.00000000000001421 ) ;
#25750=CARTESIAN_POINT ( 'NONE',  ( 0.000000000000000000, 0.000000000000000000, 12.49999999999999822 ) ) ;
#25751=VERTEX_POINT ( 'NONE', #20344 ) ;
#25752=ORIENTED_EDGE ( 'NONE', *, *, #35928, .F. ) ;
#25753=CARTESIAN_POINT ( 'NONE',  ( 71.99999662536839651, 17.32050807568879236, 17.49999999999999645 ) ) ;
#25754=VECTOR ( 'NONE', #27889, 1000.000000000000000 ) ;
#25755=CARTESIAN_POINT ( 'NONE',  ( 0.000000000000000000, 0.000000000000000000, -5.000000000000000000 ) ) ;
#25756=FACE_OUTER_BOUND ( 'NONE', #26887, .T. ) ;
#25757=LINE ( 'NONE', #2499, #32874 ) ;
#25758=ORIENTED_EDGE ( 'NONE', *, *, #14371, .T. ) ;
#25759=CARTESIAN_POINT ( 'NONE',  ( -89.42901512340354486, 31.83425564451495404, -49.86348611802629449 ) ) ;
#25760=FACE_BOUND ( 'NONE', #7723, .T. ) ;
#25762=CARTESIAN_POINT ( 'NONE',  ( 54.99999662536844625, 60.62177826491077326, 17.49999999999999645 ) ) ;
#25763=PLANE ( 'NONE',  #28483 ) ;
#25765=EDGE_CURVE ( 'NONE', #6989, #10733, #6345, .T. ) ;
#25767=DIRECTION ( 'NONE',  ( 0.000000000000000000, 0.000000000000000000, 1.000000000000000000 ) ) ;
#25768=AXIS2_PLACEMENT_3D ( 'NONE', #30801, #10578, #16576 ) ;
#25769=CYLINDRICAL_SURFACE ( 'NONE', #10393, 2.000000000000001776 ) ;
#25770=VERTEX_POINT ( 'NONE', #21072 ) ;
#25772=LINE ( 'NONE', #30805, #32060 ) ;
#25773=AXIS2_PLACEMENT_3D ( 'NONE', #20991, #7121, #18568 ) ;
#25774=DIRECTION ( 'NONE',  ( 0.000000000000000000, 0.000000000000000000, 1.000000000000000000 ) ) ;
#25779=DIRECTION ( 'NONE',  ( 0.000000000000000000, 0.000000000000000000, 1.000000000000000000 ) ) ;
#25780=DIRECTION ( 'NONE',  ( 0.000000000000000000, 0.000000000000000000, 1.000000000000000000 ) ) ;
#25781=ORIENTED_EDGE ( 'NONE', *, *, #1219, .F. ) ;
#25782=CARTESIAN_POINT ( 'NONE',  ( -35.00000337463116296, 77.94228634059957983, 12.50000000000000000 ) ) ;
#25783=ORIENTED_EDGE ( 'NONE', *, *, #2128, .T. ) ;
#25784=EDGE_CURVE ( 'NONE', #17257, #695, #12323, .T. ) ;
#25785=AXIS2_PLACEMENT_3D ( 'NONE', #14667, #11661, #22774 ) ;
#25788=CARTESIAN_POINT ( 'NONE',  ( -85.00000337463092137, 8.660254037844389075, -5.000000000000000000 ) ) ;
#25790=ORIENTED_EDGE ( 'NONE', *, *, #30676, .F. ) ;
#25791=CARTESIAN_POINT ( 'NONE',  ( -23.00000337463121980, -77.94228634059963667, -9.999999999999998224 ) ) ;
#25792=CARTESIAN_POINT ( 'NONE',  ( 64.99999662536839651, -60.62177826491080168, -9.999999999999998224 ) ) ;
#25793=CIRCLE ( 'NONE', #9614, 2.000000000000001776 ) ;
#25794=ORIENTED_EDGE ( 'NONE', *, *, #29752, .F. ) ;
#25796=AXIS2_PLACEMENT_3D ( 'NONE', #13209, #10383, #27633 ) ;
#25798=CARTESIAN_POINT ( 'NONE',  ( 64.99999662536839651, -60.62177826491080168, -9.999999999999998224 ) ) ;
#25800=ORIENTED_EDGE ( 'NONE', *, *, #9684, .T. ) ;
#25801=FACE_OUTER_BOUND ( 'NONE', #798, .T. ) ;
#25802=CARTESIAN_POINT ( 'NONE',  ( -13.00000337463126066, 77.94228634059957983, -5.000000000000000000 ) ) ;
#25803=ORIENTED_EDGE ( 'NONE', *, *, #16747, .F. ) ;
#25804=CARTESIAN_POINT ( 'NONE',  ( -15.00000337463125710, -77.94228634059960825, -9.999999999999998224 ) ) ;
#25805=DIRECTION ( 'NONE',  ( 0.000000000000000000, 0.000000000000000000, 1.000000000000000000 ) ) ;
#25806=FACE_OUTER_BOUND ( 'NONE', #22816, .T. ) ;
#25807=ADVANCED_FACE ( 'NONE', ( #28778 ), #17518, .F. ) ;
#25808=EDGE_CURVE ( 'NONE', #126, #2266, #33316, .T. ) ;
#25809=LINE ( 'NONE', #3109, #36240 ) ;
#25810=VERTEX_POINT ( 'NONE', #35162 ) ;
#25811=EDGE_CURVE ( 'NONE', #520, #10163, #20901, .T. ) ;
#25814=EDGE_CURVE ( 'NONE', #21946, #32590, #23735, .T. ) ;
#25815=ORIENTED_EDGE ( 'NONE', *, *, #6707, .T. ) ;
#25816=ORIENTED_EDGE ( 'NONE', *, *, #20194, .F. ) ;
#25818=CARTESIAN_POINT ( 'NONE',  ( 89.99999662536828282, 0.000000000000000000, -9.999999999999998224 ) ) ;
#25819=CARTESIAN_POINT ( 'NONE',  ( -57.00000337463109901, -60.62177826491083010, -9.999999999999998224 ) ) ;
#25820=CARTESIAN_POINT ( 'NONE',  ( -87.00000337463093558, -8.660254037844422825, -9.999999999999998224 ) ) ;
#25821=ORIENTED_EDGE ( 'NONE', *, *, #18758, .T. ) ;
#25822=DIRECTION ( 'NONE',  ( 0.000000000000000000, 0.000000000000000000, 1.000000000000000000 ) ) ;
#25823=VERTEX_POINT ( 'NONE', #9079 ) ;
#25824=ADVANCED_FACE ( 'NONE', ( #20503 ), #31927, .F. ) ;
#25826=VERTEX_POINT ( 'NONE', #34962 ) ;
#25827=FACE_OUTER_BOUND ( 'NONE', #13270, .T. ) ;
#25828=DIRECTION ( 'NONE',  ( 0.000000000000000000, 0.000000000000000000, -1.000000000000000000 ) ) ;
#25829=DIRECTION ( 'NONE',  ( 0.000000000000000000, 0.000000000000000000, 1.000000000000000000 ) ) ;
#25830=AXIS2_PLACEMENT_3D ( 'NONE', #10868, #33004, #7142 ) ;
#25836=EDGE_CURVE ( 'NONE', #12353, #9125, #36320, .T. ) ;
#25838=DIRECTION ( 'NONE',  ( 0.000000000000000000, 0.000000000000000000, 1.000000000000000000 ) ) ;
#25840=CARTESIAN_POINT ( 'NONE',  ( -27.78182860042817026, -56.67878100130359087, -4.999999999999997335 ) ) ;
#25841=ORIENTED_EDGE ( 'NONE', *, *, #3045, .F. ) ;
#25842=VERTEX_POINT ( 'NONE', #1210 ) ;
#25843=ORIENTED_EDGE ( 'NONE', *, *, #9624, .F. ) ;
#25844=EDGE_CURVE ( 'NONE', #35809, #34083, #10562, .T. ) ;
#25845=DIRECTION ( 'NONE',  ( 0.000000000000000000, 0.000000000000000000, -1.000000000000000000 ) ) ;
#25846=ADVANCED_FACE ( 'NONE', ( #18463 ), #4218, .F. ) ;
#25850=VECTOR ( 'NONE', #25531, 1000.000000000000000 ) ;
#25851=CARTESIAN_POINT ( 'NONE',  ( -68.17080498304596858, 51.15280100851584422, -5.000000000000000000 ) ) ;
#25852=CARTESIAN_POINT ( 'NONE',  ( 7.122621931239992550E-13, 68.00000000000000000, 12.49999999999999822 ) ) ;
#25853=VERTEX_POINT ( 'NONE', #27445 ) ;
#25854=ORIENTED_EDGE ( 'NONE', *, *, #10709, .T. ) ;
#25859=EDGE_LOOP ( 'NONE', ( #9845, #21092, #32104, #17167 ) ) ;
#25861=FACE_BOUND ( 'NONE', #22879, .T. ) ;
#25863=ORIENTED_EDGE ( 'NONE', *, *, #24, .F. ) ;
#25864=LINE ( 'NONE', #157, #20044 ) ;
#25865=ORIENTED_EDGE ( 'NONE', *, *, #12245, .F. ) ;
#25866=EDGE_CURVE ( 'NONE', #34263, #3095, #32685, .T. ) ;
#25869=EDGE_CURVE ( 'NONE', #14264, #34734, #32081, .T. ) ;
#25870=ORIENTED_EDGE ( 'NONE', *, *, #11161, .T. ) ;
#25871=EDGE_LOOP ( 'NONE', ( #28611, #30011, #19296, #35014 ) ) ;
#25872=ORIENTED_EDGE ( 'NONE', *, *, #26757, .F. ) ;
#25873=ORIENTED_EDGE ( 'NONE', *, *, #19186, .T. ) ;
#25874=EDGE_LOOP ( 'NONE', ( #16001, #35193 ) ) ;
#25875=DIRECTION ( 'NONE',  ( 1.000000000000000000, 0.000000000000000000, 0.000000000000000000 ) ) ;
#25876=DIRECTION ( 'NONE',  ( 1.000000000000000000, 0.000000000000000000, 0.000000000000000000 ) ) ;
#25877=CARTESIAN_POINT ( 'NONE',  ( 84.99999662536831124, -8.660254037844397956, 17.49999999999999645 ) ) ;
#25878=FACE_OUTER_BOUND ( 'NONE', #36699, .T. ) ;
#25879=CARTESIAN_POINT ( 'NONE',  ( 44.99999662536849598, -77.94228634059960825, -9.999999999999998224 ) ) ;
#25880=VERTEX_POINT ( 'NONE', #12631 ) ;
#25881=CYLINDRICAL_SURFACE ( 'NONE', #33886, 2.000000000000000000 ) ;
#25883=EDGE_CURVE ( 'NONE', #14204, #5735, #30446, .T. ) ;
#25885=ORIENTED_EDGE ( 'NONE', *, *, #19299, .T. ) ;
#25886=DIRECTION ( 'NONE',  ( 1.000000000000000000, 0.000000000000000000, 0.000000000000000000 ) ) ;
#25887=DIRECTION ( 'NONE',  ( 0.000000000000000000, 0.000000000000000000, 1.000000000000000000 ) ) ;
#25888=VERTEX_POINT ( 'NONE', #1765 ) ;
#25889=VERTEX_POINT ( 'NONE', #21253 ) ;
#25890=DIRECTION ( 'NONE',  ( 0.000000000000000000, 0.000000000000000000, 1.000000000000000000 ) ) ;
#25891=AXIS2_PLACEMENT_3D ( 'NONE', #33562, #7483, #30351 ) ;
#25892=CARTESIAN_POINT ( 'NONE',  ( 29.99999662536857770, -69.28203230275519786, -5.000000000000000000 ) ) ;
#25895=DIRECTION ( 'NONE',  ( 0.000000000000000000, 0.000000000000000000, 1.000000000000000000 ) ) ;
#25896=VERTEX_POINT ( 'NONE', #4774 ) ;
#25897=ORIENTED_EDGE ( 'NONE', *, *, #14936, .T. ) ;
#25898=DIRECTION ( 'NONE',  ( 1.000000000000000000, 0.000000000000000000, 0.000000000000000000 ) ) ;
#25900=DIRECTION ( 'NONE',  ( 0.000000000000000000, 0.000000000000000000, -1.000000000000000000 ) ) ;
#25902=VERTEX_POINT ( 'NONE', #13199 ) ;
#25903=EDGE_CURVE ( 'NONE', #23009, #8155, #30890, .T. ) ;
#25904=CARTESIAN_POINT ( 'NONE',  ( -37.00000337463116296, -60.62177826491080168, -9.999999999999998224 ) ) ;
#25905=ORIENTED_EDGE ( 'NONE', *, *, #35057, .F. ) ;
#25906=ORIENTED_EDGE ( 'NONE', *, *, #6174, .T. ) ;
#25907=EDGE_CURVE ( 'NONE', #26162, #36358, #35524, .T. ) ;
#25908=AXIS2_PLACEMENT_3D ( 'NONE', #14283, #25729, #29435 ) ;
#25911=ORIENTED_EDGE ( 'NONE', *, *, #18665, .F. ) ;
#25912=ORIENTED_EDGE ( 'NONE', *, *, #22241, .F. ) ;
#25913=ADVANCED_FACE ( 'NONE', ( #27244 ), #4019, .F. ) ;
#25914=DIRECTION ( 'NONE',  ( 1.000000000000000000, 0.000000000000000000, 0.000000000000000000 ) ) ;
#25915=EDGE_CURVE ( 'NONE', #36497, #10851, #21313, .T. ) ;
#25917=ORIENTED_EDGE ( 'NONE', *, *, #31134, .F. ) ;
#25918=CARTESIAN_POINT ( 'NONE',  ( -3.499999999999991562, -55.00000000000000000, -5.000000000000000000 ) ) ;
#25919=AXIS2_PLACEMENT_3D ( 'NONE', #2231, #13669, #16673 ) ;
#25920=FACE_BOUND ( 'NONE', #25466, .T. ) ;
#25921=AXIS2_PLACEMENT_3D ( 'NONE', #8135, #19038, #2340 ) ;
#25922=CARTESIAN_POINT ( 'NONE',  ( -27.00000337463120914, 77.94228634059957983, 12.50000000000000000 ) ) ;
#25923=PLANE ( 'NONE',  #18078 ) ;
#25924=FACE_OUTER_BOUND ( 'NONE', #24822, .T. ) ;
#25925=ADVANCED_FACE ( 'NONE', ( #21809 ), #32691, .F. ) ;
#25926=CYLINDRICAL_SURFACE ( 'NONE', #32660, 2.000000000000000000 ) ;
#25927=EDGE_CURVE ( 'NONE', #27221, #31238, #29091, .T. ) ;
#25931=ADVANCED_FACE ( 'NONE', ( #15818 ), #24461, .F. ) ;
#25932=CARTESIAN_POINT ( 'NONE',  ( 64.99999662536841072, 25.98076211353318854, 12.50000000000000000 ) ) ;
#25934=EDGE_CURVE ( 'NONE', #20212, #32853, #29124, .T. ) ;
#25935=DIRECTION ( 'NONE',  ( 0.000000000000000000, 0.000000000000000000, -1.000000000000000000 ) ) ;
#25936=CARTESIAN_POINT ( 'NONE',  ( 6.999996625368676284, -77.94228634059960825, 17.49999999999999645 ) ) ;
#25937=AXIS2_PLACEMENT_3D ( 'NONE', #6242, #34036, #2901 ) ;
#25939=ORIENTED_EDGE ( 'NONE', *, *, #26399, .F. ) ;
#25940=VECTOR ( 'NONE', #9750, 1000.000000000000000 ) ;
#25941=EDGE_LOOP ( 'NONE', ( #784, #24460, #19921, #20916 ) ) ;
#25942=EDGE_LOOP ( 'NONE', ( #36693, #3719, #18005, #10150 ) ) ;
#25944=DIRECTION ( 'NONE',  ( 0.000000000000000000, 0.000000000000000000, 1.000000000000000000 ) ) ;
#25946=ORIENTED_EDGE ( 'NONE', *, *, #25814, .F. ) ;
#25947=DIRECTION ( 'NONE',  ( 1.000000000000000000, 0.000000000000000000, 0.000000000000000000 ) ) ;
#25948=AXIS2_PLACEMENT_3D ( 'NONE', #25932, #11491, #11852 ) ;
#25952=FACE_OUTER_BOUND ( 'NONE', #22845, .T. ) ;
#25953=ORIENTED_EDGE ( 'NONE', *, *, #30883, .F. ) ;
#25954=EDGE_LOOP ( 'NONE', ( #26424, #369 ) ) ;
#25955=CYLINDRICAL_SURFACE ( 'NONE', #17217, 2.000000000000001776 ) ;
#25956=LINE ( 'NONE', #25791, #36389 ) ;
#25959=ORIENTED_EDGE ( 'NONE', *, *, #1683, .F. ) ;
#25960=CARTESIAN_POINT ( 'NONE',  ( 7.999996625368625658, 86.60254037844397601, 17.49999999999999645 ) ) ;
#25961=AXIS2_PLACEMENT_3D ( 'NONE', #9626, #29655, #794 ) ;
#25962=LINE ( 'NONE', #6089, #12062 ) ;
#25963=DIRECTION ( 'NONE',  ( 0.000000000000000000, 0.000000000000000000, -1.000000000000000000 ) ) ;
#25965=CYLINDRICAL_SURFACE ( 'NONE', #17149, 2.000000000000001776 ) ;
#25966=CARTESIAN_POINT ( 'NONE',  ( 61.99999662536842493, 51.96152422706639129, -5.000000000000000000 ) ) ;
#25967=EDGE_LOOP ( 'NONE', ( #33205, #36167, #2383, #1279 ) ) ;
#25968=FACE_OUTER_BOUND ( 'NONE', #34478, .T. ) ;
#25969=DIRECTION ( 'NONE',  ( 1.000000000000000000, 0.000000000000000000, 0.000000000000000000 ) ) ;
#25970=DIRECTION ( 'NONE',  ( 0.000000000000000000, 0.000000000000000000, 1.000000000000000000 ) ) ;
#25972=CIRCLE ( 'NONE', #9796, 2.000000000000001776 ) ;
#25973=EDGE_CURVE ( 'NONE', #5915, #23282, #34013, .T. ) ;
#25974=DIRECTION ( 'NONE',  ( 0.000000000000000000, 0.000000000000000000, -1.000000000000000000 ) ) ;
#25975=AXIS2_PLACEMENT_3D ( 'NONE', #11271, #5292, #19718 ) ;
#25976=EDGE_CURVE ( 'NONE', #4621, #30710, #14309, .T. ) ;
#25977=ORIENTED_EDGE ( 'NONE', *, *, #23838, .F. ) ;
#25979=CARTESIAN_POINT ( 'NONE',  ( -55.00000337463109901, -60.62177826491083010, 17.49999999999999645 ) ) ;
#25980=CIRCLE ( 'NONE', #30761, 2.000000000000001776 ) ;
#25981=ORIENTED_EDGE ( 'NONE', *, *, #23524, .T. ) ;
#25982=EDGE_LOOP ( 'NONE', ( #7282, #16500, #1049, #28182 ) ) ;
#25983=ORIENTED_EDGE ( 'NONE', *, *, #6613, .F. ) ;
#25985=DIRECTION ( 'NONE',  ( 0.000000000000000000, 0.000000000000000000, 1.000000000000000000 ) ) ;
#25986=DIRECTION ( 'NONE',  ( 0.000000000000000000, 0.000000000000000000, 1.000000000000000000 ) ) ;
#25988=DIRECTION ( 'NONE',  ( 0.000000000000000000, 0.000000000000000000, 1.000000000000000000 ) ) ;
#25989=ORIENTED_EDGE ( 'NONE', *, *, #23229, .T. ) ;
#25990=CARTESIAN_POINT ( 'NONE',  ( 43.19957991610432657, 47.04203867989531318, 12.49999999999999822 ) ) ;
#25991=EDGE_LOOP ( 'NONE', ( #20681, #19471 ) ) ;
#25992=FACE_BOUND ( 'NONE', #34911, .T. ) ;
#25993=ADVANCED_FACE ( 'NONE', ( #22925 ), #8123, .T. ) ;
#25994=CIRCLE ( 'NONE', #9824, 27.00000000000001421 ) ;
#25995=FACE_OUTER_BOUND ( 'NONE', #21614, .T. ) ;
#25996=CIRCLE ( 'NONE', #22408, 2.000000000000001776 ) ;
#25997=DIRECTION ( 'NONE',  ( 1.000000000000000000, 0.000000000000000000, -0.000000000000000000 ) ) ;
#25998=DIRECTION ( 'NONE',  ( 0.000000000000000000, 0.000000000000000000, -1.000000000000000000 ) ) ;
#26000=DIRECTION ( 'NONE',  ( 0.000000000000000000, 0.000000000000000000, 1.000000000000000000 ) ) ;
#26002=CARTESIAN_POINT ( 'NONE',  ( -12.00000337463128908, 69.28203230275516944, -5.000000000000000000 ) ) ;
#26003=CARTESIAN_POINT ( 'NONE',  ( 44.99999662536849598, 60.62177826491077326, -5.000000000000000000 ) ) ;
#26004=ORIENTED_EDGE ( 'NONE', *, *, #19186, .F. ) ;
#26005=LINE ( 'NONE', #11746, #35195 ) ;
#26006=CARTESIAN_POINT ( 'NONE',  ( -75.00000337463099243, -25.98076211353322051, -5.000000000000000000 ) ) ;
#26007=DIRECTION ( 'NONE',  ( 0.000000000000000000, 0.000000000000000000, 1.000000000000000000 ) ) ;
#26011=EDGE_CURVE ( 'NONE', #32397, #27172, #29711, .T. ) ;
#26012=EDGE_LOOP ( 'NONE', ( #17414, #12104 ) ) ;
#26016=VECTOR ( 'NONE', #30297, 1000.000000000000000 ) ;
#26017=CARTESIAN_POINT ( 'NONE',  ( 0.000000000000000000, 0.000000000000000000, -5.000000000000000000 ) ) ;
#26018=CARTESIAN_POINT ( 'NONE',  ( 11.99999662536865763, -86.60254037844400443, 17.49999999999999645 ) ) ;
#26019=DIRECTION ( 'NONE',  ( 0.000000000000000000, 0.000000000000000000, 1.000000000000000000 ) ) ;
#26020=CYLINDRICAL_SURFACE ( 'NONE', #7811, 2.000000000000001776 ) ;
#26021=VERTEX_POINT ( 'NONE', #19922 ) ;
#26022=ORIENTED_EDGE ( 'NONE', *, *, #5743, .F. ) ;
#26023=CARTESIAN_POINT ( 'NONE',  ( -58.48108235278846934, -36.97203788309006711, -49.86561046011506448 ) ) ;
#26025=ADVANCED_FACE ( 'NONE', ( #8495 ), #19566, .F. ) ;
#26026=DIRECTION ( 'NONE',  ( -1.000000000000000000, 0.000000000000000000, -0.000000000000000000 ) ) ;
#26027=AXIS2_PLACEMENT_3D ( 'NONE', #35443, #9730, #1470 ) ;
#26028=DIRECTION ( 'NONE',  ( 0.000000000000000000, 0.000000000000000000, 1.000000000000000000 ) ) ;
#26029=ORIENTED_EDGE ( 'NONE', *, *, #30332, .F. ) ;
#26031=CIRCLE ( 'NONE', #19458, 2.000000000000001776 ) ;
#26032=FACE_BOUND ( 'NONE', #7631, .T. ) ;
#26033=ORIENTED_EDGE ( 'NONE', *, *, #31808, .F. ) ;
#26034=EDGE_LOOP ( 'NONE', ( #4324, #27766, #33691, #8850, #19558, #20520, #33744, #34425, #16226, #24407, #17613, #29622 ) ) ;
#26035=ADVANCED_FACE ( 'NONE', ( #25207 ), #19373, .F. ) ;
#26036=CARTESIAN_POINT ( 'NONE',  ( 79.99999662536832545, -34.64101615137759183, -9.999999999999998224 ) ) ;
#26037=ORIENTED_EDGE ( 'NONE', *, *, #22365, .F. ) ;
#26038=AXIS2_PLACEMENT_3D ( 'NONE', #12280, #20737, #862 ) ;
#26039=AXIS2_PLACEMENT_3D ( 'NONE', #25106, #27883, #2919 ) ;
#26041=ADVANCED_FACE ( 'NONE', ( #10763 ), #36452, .F. ) ;
#26042=DIRECTION ( 'NONE',  ( 0.000000000000000000, 0.000000000000000000, 1.000000000000000000 ) ) ;
#26044=ORIENTED_EDGE ( 'NONE', *, *, #30402, .F. ) ;
#26045=EDGE_LOOP ( 'NONE', ( #34348, #20052 ) ) ;
#26047=ORIENTED_EDGE ( 'NONE', *, *, #15628, .F. ) ;
#26048=AXIS2_PLACEMENT_3D ( 'NONE', #5167, #8361, #16606 ) ;
#26049=DIRECTION ( 'NONE',  ( 0.000000000000000000, 0.000000000000000000, 1.000000000000000000 ) ) ;
#26050=ADVANCED_FACE ( 'NONE', ( #22367 ), #19210, .F. ) ;
#26052=CIRCLE ( 'NONE', #6892, 2.000000000000001776 ) ;
#26053=DIRECTION ( 'NONE',  ( 0.000000000000000000, 0.000000000000000000, 1.000000000000000000 ) ) ;
#26054=DIRECTION ( 'NONE',  ( 0.000000000000000000, 0.000000000000000000, 1.000000000000000000 ) ) ;
#26055=DIRECTION ( 'NONE',  ( -1.000000000000000000, 0.000000000000000000, 0.000000000000000000 ) ) ;
#26057=AXIS2_PLACEMENT_3D ( 'NONE', #20367, #25988, #6115 ) ;
#26058=CARTESIAN_POINT ( 'NONE',  ( 24.99999662536859546, -77.94228634059960825, -9.999999999999998224 ) ) ;
#26059=VECTOR ( 'NONE', #21141, 1000.000000000000000 ) ;
#26060=ADVANCED_FACE ( 'NONE', ( #30624 ), #33810, .F. ) ;
#26061=CARTESIAN_POINT ( 'NONE',  ( 76.99999662536836809, -8.660254037844401509, 17.49999999999999645 ) ) ;
#26062=CARTESIAN_POINT ( 'NONE',  ( 62.33939050065184517, -13.89091430021398565, 12.49999999999999822 ) ) ;
#26063=ORIENTED_EDGE ( 'NONE', *, *, #35009, .F. ) ;
#26064=CARTESIAN_POINT ( 'NONE',  ( -80.00000337463094979, -2.428612866367529932E-14, 17.49999999999999645 ) ) ;
#26065=CARTESIAN_POINT ( 'NONE',  ( 83.47442710120355969, -31.09745072740822991, -49.86348611802629449 ) ) ;
#26066=AXIS2_PLACEMENT_3D ( 'NONE', #12080, #23734, #6670 ) ;
#26067=CIRCLE ( 'NONE', #9903, 2.000000000000001776 ) ;
#26068=ORIENTED_EDGE ( 'NONE', *, *, #1618, .F. ) ;
#26069=EDGE_CURVE ( 'NONE', #34910, #32311, #23140, .T. ) ;
#26072=CARTESIAN_POINT ( 'NONE',  ( -15.00000337463125710, -77.94228634059960825, -9.999999999999998224 ) ) ;
#26073=EDGE_CURVE ( 'NONE', #9400, #18535, #11749, .T. ) ;
#26074=CARTESIAN_POINT ( 'NONE',  ( 52.99999662536844625, -60.62177826491080168, 12.50000000000000000 ) ) ;
#26075=CARTESIAN_POINT ( 'NONE',  ( 11.99999662536862566, 86.60254037844397601, 12.50000000000000000 ) ) ;
#26076=FACE_OUTER_BOUND ( 'NONE', #31466, .T. ) ;
#26077=EDGE_LOOP ( 'NONE', ( #35179, #16914, #29028, #14286 ) ) ;
#26079=LINE ( 'NONE', #3590, #27908 ) ;
#26081=AXIS2_PLACEMENT_3D ( 'NONE', #33072, #16026, #36083 ) ;
#26082=VERTEX_POINT ( 'NONE', #28183 ) ;
#26083=CIRCLE ( 'NONE', #33264, 3.000000000000006661 ) ;
#26085=ORIENTED_EDGE ( 'NONE', *, *, #28453, .T. ) ;
#26086=AXIS2_PLACEMENT_3D ( 'NONE', #28825, #3150, #14578 ) ;
#26089=CARTESIAN_POINT ( 'NONE',  ( 52.99999662536844625, -60.62177826491080168, 17.49999999999999645 ) ) ;
#26090=AXIS2_PLACEMENT_3D ( 'NONE', #36527, #13991, #33533 ) ;
#26091=CARTESIAN_POINT ( 'NONE',  ( -87.00000337463093558, 8.660254037844389075, -9.999999999999998224 ) ) ;
#26092=EDGE_CURVE ( 'NONE', #200, #21374, #30336, .T. ) ;
#26093=DIRECTION ( 'NONE',  ( -1.000000000000000000, 0.000000000000000000, 0.000000000000000000 ) ) ;
#26094=ORIENTED_EDGE ( 'NONE', *, *, #5333, .T. ) ;
#26095=EDGE_LOOP ( 'NONE', ( #4283, #17732 ) ) ;
#26096=CARTESIAN_POINT ( 'NONE',  ( 22.99999662536859901, -77.94228634059960825, -9.999999999999998224 ) ) ;
#26097=DIRECTION ( 'NONE',  ( -1.000000000000000000, 0.000000000000000000, 0.000000000000000000 ) ) ;
#26098=AXIS2_PLACEMENT_3D ( 'NONE', #27480, #10601, #4248 ) ;
#26099=CARTESIAN_POINT ( 'NONE',  ( -20.00000337463123756, -86.60254037844400443, -9.999999999999998224 ) ) ;
#26100=ORIENTED_EDGE ( 'NONE', *, *, #5786, .F. ) ;
#26101=CARTESIAN_POINT ( 'NONE',  ( -70.00000337463099243, 17.32050807568877460, -9.999999999999998224 ) ) ;
#26102=FACE_BOUND ( 'NONE', #1967, .T. ) ;
#26103=CARTESIAN_POINT ( 'NONE',  ( 21.99999662536857770, 86.60254037844397601, -9.999999999999998224 ) ) ;
#26104=DIRECTION ( 'NONE',  ( 0.000000000000000000, 0.000000000000000000, 1.000000000000000000 ) ) ;
#26105=CARTESIAN_POINT ( 'NONE',  ( -75.00000337463097821, 8.660254037844374864, 12.50000000000000000 ) ) ;
#26106=FACE_OUTER_BOUND ( 'NONE', #34593, .T. ) ;
#26107=EDGE_CURVE ( 'NONE', #15570, #13632, #27338, .T. ) ;
#26108=CYLINDRICAL_SURFACE ( 'NONE', #12572, 2.000000000000001776 ) ;
#26109=CARTESIAN_POINT ( 'NONE',  ( 62.99999662536839651, 60.62177826491078747, 12.50000000000000000 ) ) ;
#26110=VERTEX_POINT ( 'NONE', #5500 ) ;
#26111=ADVANCED_FACE ( 'NONE', ( #14107 ), #37003, .F. ) ;
#26112=DIRECTION ( 'NONE',  ( 0.000000000000000000, 0.000000000000000000, -1.000000000000000000 ) ) ;
#26114=DIRECTION ( 'NONE',  ( 1.000000000000000000, 0.000000000000000000, 0.000000000000000000 ) ) ;
#26115=AXIS2_PLACEMENT_3D ( 'NONE', #26448, #15023, #23639 ) ;
#26117=EDGE_CURVE ( 'NONE', #18742, #27467, #8858, .T. ) ;
#26118=CIRCLE ( 'NONE', #28491, 1.999999999999998224 ) ;
#26119=VERTEX_POINT ( 'NONE', #771 ) ;
#26120=AXIS2_PLACEMENT_3D ( 'NONE', #22842, #34278, #28987 ) ;
#26122=EDGE_CURVE ( 'NONE', #21182, #17038, #20170, .T. ) ;
#26123=DIRECTION ( 'NONE',  ( 0.000000000000000000, 0.000000000000000000, 1.000000000000000000 ) ) ;
#26124=CARTESIAN_POINT ( 'NONE',  ( -50.00000337463109190, 51.96152422706637708, 12.50000000000000000 ) ) ;
#26125=EDGE_CURVE ( 'NONE', #21598, #14210, #1003, .T. ) ;
#26126=DIRECTION ( 'NONE',  ( 0.000000000000000000, 0.000000000000000000, -1.000000000000000000 ) ) ;
#26128=CIRCLE ( 'NONE', #5797, 2.000000000000001776 ) ;
#26129=DIRECTION ( 'NONE',  ( 0.000000000000000000, 0.000000000000000000, 1.000000000000000000 ) ) ;
#26130=ORIENTED_EDGE ( 'NONE', *, *, #27457, .F. ) ;
#26131=DIRECTION ( 'NONE',  ( -1.000000000000000000, 0.000000000000000000, 0.000000000000000000 ) ) ;
#26132=ORIENTED_EDGE ( 'NONE', *, *, #14774, .F. ) ;
#26133=CARTESIAN_POINT ( 'NONE',  ( 81.99999662536832545, -34.64101615137759183, -9.999999999999998224 ) ) ;
#26134=ORIENTED_EDGE ( 'NONE', *, *, #32921, .T. ) ;
#26135=EDGE_CURVE ( 'NONE', #31600, #1195, #19562, .T. ) ;
#26136=AXIS2_PLACEMENT_3D ( 'NONE', #407, #26651, #11842 ) ;
#26137=VERTEX_POINT ( 'NONE', #23657 ) ;
#26140=EDGE_CURVE ( 'NONE', #35478, #5493, #22551, .T. ) ;
#26141=AXIS2_PLACEMENT_3D ( 'NONE', #35269, #32237, #23443 ) ;
#26142=CARTESIAN_POINT ( 'NONE',  ( -47.00000337463111322, 77.94228634059959404, -9.999999999999998224 ) ) ;
#26145=CIRCLE ( 'NONE', #29132, 2.000000000000000000 ) ;
#26147=AXIS2_PLACEMENT_3D ( 'NONE', #36050, #33212, #24050 ) ;
#26151=EDGE_LOOP ( 'NONE', ( #10266, #25983, #17263, #28095 ) ) ;
#26152=DIRECTION ( 'NONE',  ( 1.000000000000000000, 0.000000000000000000, 0.000000000000000000 ) ) ;
#26153=DIRECTION ( 'NONE',  ( 0.000000000000000000, 0.000000000000000000, 1.000000000000000000 ) ) ;
#26154=ORIENTED_EDGE ( 'NONE', *, *, #30932, .T. ) ;
#26155=DIRECTION ( 'NONE',  ( 0.000000000000000000, 0.000000000000000000, 1.000000000000000000 ) ) ;
#26156=DIRECTION ( 'NONE',  ( 0.000000000000000000, 0.000000000000000000, -1.000000000000000000 ) ) ;
#26158=DIRECTION ( 'NONE',  ( 1.000000000000000000, 0.000000000000000000, 0.000000000000000000 ) ) ;
#26160=ADVANCED_FACE ( 'NONE', ( #8666 ), #17651, .F. ) ;
#26161=CARTESIAN_POINT ( 'NONE',  ( 77.99999662536832545, -17.32050807568879591, 12.50000000000000000 ) ) ;
#26162=VERTEX_POINT ( 'NONE', #18032 ) ;
#26164=DIRECTION ( 'NONE',  ( 1.000000000000000000, 0.000000000000000000, 0.000000000000000000 ) ) ;
#26168=ORIENTED_EDGE ( 'NONE', *, *, #32768, .T. ) ;
#26169=ORIENTED_EDGE ( 'NONE', *, *, #34773, .F. ) ;
#26170=VERTEX_POINT ( 'NONE', #25918 ) ;
#26171=AXIS2_PLACEMENT_3D ( 'NONE', #7778, #21468, #1581 ) ;
#26172=PLANE ( 'NONE',  #463 ) ;
#26173=ADVANCED_FACE ( 'NONE', ( #17309 ), #32278, .F. ) ;
#26175=CIRCLE ( 'NONE', #5839, 2.000000000000001776 ) ;
#26176=VECTOR ( 'NONE', #15934, 1000.000000000000000 ) ;
#26177=CIRCLE ( 'NONE', #416, 2.000000000000001776 ) ;
#26178=AXIS2_PLACEMENT_3D ( 'NONE', #27630, #33458, #7771 ) ;
#26179=CARTESIAN_POINT ( 'NONE',  ( -15.00000337463126066, 77.94228634059957983, 17.49999999999999645 ) ) ;
#26180=EDGE_LOOP ( 'NONE', ( #33954, #27741, #18669, #3721, #21270, #20421 ) ) ;
#26181=DIRECTION ( 'NONE',  ( 1.000000000000000000, 0.000000000000000000, 0.000000000000000000 ) ) ;
#26182=ORIENTED_EDGE ( 'NONE', *, *, #8787, .T. ) ;
#26183=FACE_BOUND ( 'NONE', #32715, .T. ) ;
#26184=CIRCLE ( 'NONE', #12404, 3.000000000000002665 ) ;
#26185=ADVANCED_FACE ( 'NONE', ( #34553 ), #3609, .F. ) ;
#26187=EDGE_CURVE ( 'NONE', #26782, #18020, #10593, .T. ) ;
#26189=EDGE_CURVE ( 'NONE', #30229, #33896, #15379, .T. ) ;
#26191=FACE_OUTER_BOUND ( 'NONE', #314, .T. ) ;
#26192=ORIENTED_EDGE ( 'NONE', *, *, #35996, .T. ) ;
#26193=DIRECTION ( 'NONE',  ( 0.000000000000000000, 0.000000000000000000, 1.000000000000000000 ) ) ;
#26194=AXIS2_PLACEMENT_3D ( 'NONE', #26702, #6822, #29891 ) ;
#26195=VECTOR ( 'NONE', #34913, 1000.000000000000000 ) ;
#26197=VECTOR ( 'NONE', #24656, 1000.000000000000000 ) ;
#26198=DIRECTION ( 'NONE',  ( 1.000000000000000000, 0.000000000000000000, 0.000000000000000000 ) ) ;
#26201=CARTESIAN_POINT ( 'NONE',  ( -35.00000337463116296, -60.62177826491080168, -9.999999999999998224 ) ) ;
#26202=CARTESIAN_POINT ( 'NONE',  ( 12.99999662536863632, -77.94228634059960825, -9.999999999999998224 ) ) ;
#26203=CARTESIAN_POINT ( 'NONE',  ( 32.16008401677996886, 61.25926521283068382, -4.999999999999997335 ) ) ;
#26207=ORIENTED_EDGE ( 'NONE', *, *, #7435, .F. ) ;
#26208=ORIENTED_EDGE ( 'NONE', *, *, #26474, .T. ) ;
#26210=VECTOR ( 'NONE', #29145, 1000.000000000000000 ) ;
#26211=EDGE_CURVE ( 'NONE', #8583, #13323, #3386, .T. ) ;
#26213=AXIS2_PLACEMENT_3D ( 'NONE', #32661, #6791, #9628 ) ;
#26214=DIRECTION ( 'NONE',  ( 0.000000000000000000, 0.000000000000000000, -1.000000000000000000 ) ) ;
#26215=LINE ( 'NONE', #2986, #8136 ) ;
#26216=DIRECTION ( 'NONE',  ( 1.000000000000000000, 0.000000000000000000, 0.000000000000000000 ) ) ;
#26217=CIRCLE ( 'NONE', #22023, 65.00000000000000000 ) ;
#26218=CIRCLE ( 'NONE', #23221, 2.000000000000001776 ) ;
#26219=DIRECTION ( 'NONE',  ( 1.000000000000000000, 0.000000000000000000, 0.000000000000000000 ) ) ;
#26220=EDGE_LOOP ( 'NONE', ( #13538, #36933 ) ) ;
#26221=CIRCLE ( 'NONE', #25064, 2.000000000000001776 ) ;
#26222=ORIENTED_EDGE ( 'NONE', *, *, #1553, .T. ) ;
#26223=CARTESIAN_POINT ( 'NONE',  ( 84.99999662536831124, -25.98076211353319565, -9.999999999999998224 ) ) ;
#26224=AXIS2_PLACEMENT_3D ( 'NONE', #227, #34375, #37015 ) ;
#26227=DIRECTION ( 'NONE',  ( 0.000000000000000000, 0.000000000000000000, 1.000000000000000000 ) ) ;
#26228=EDGE_LOOP ( 'NONE', ( #25323, #15851, #35681, #25841 ) ) ;
#26229=VECTOR ( 'NONE', #4883, 1000.000000000000000 ) ;
#26230=FACE_BOUND ( 'NONE', #1921, .T. ) ;
#26231=ORIENTED_EDGE ( 'NONE', *, *, #31637, .T. ) ;
#26232=ORIENTED_EDGE ( 'NONE', *, *, #20583, .T. ) ;
#26233=EDGE_CURVE ( 'NONE', #34990, #20996, #8185, .T. ) ;
#26234=LINE ( 'NONE', #28675, #3853 ) ;
#26235=ORIENTED_EDGE ( 'NONE', *, *, #27990, .T. ) ;
#26236=AXIS2_PLACEMENT_3D ( 'NONE', #19119, #35805, #30541 ) ;
#26237=CARTESIAN_POINT ( 'NONE',  ( 14.99999662536863632, -77.94228634059960825, -9.999999999999998224 ) ) ;
#26238=LINE ( 'NONE', #23599, #35252 ) ;
#26239=ORIENTED_EDGE ( 'NONE', *, *, #11005, .F. ) ;
#26240=VERTEX_POINT ( 'NONE', #14855 ) ;
#26241=EDGE_LOOP ( 'NONE', ( #33473, #17298, #3540, #31947, #27322 ) ) ;
#26242=AXIS2_PLACEMENT_3D ( 'NONE', #31589, #3105, #6271 ) ;
#26243=ORIENTED_EDGE ( 'NONE', *, *, #18531, .T. ) ;
#26244=VECTOR ( 'NONE', #19530, 1000.000000000000000 ) ;
#26245=VERTEX_POINT ( 'NONE', #968 ) ;
#26249=CARTESIAN_POINT ( 'NONE',  ( 9.999996625368655856, -69.28203230275519786, -9.999999999999998224 ) ) ;
#26251=DIRECTION ( 'NONE',  ( 1.000000000000000000, 0.000000000000000000, 0.000000000000000000 ) ) ;
#26252=EDGE_CURVE ( 'NONE', #14264, #29027, #26294, .T. ) ;
#26253=AXIS2_PLACEMENT_3D ( 'NONE', #34176, #11083, #33986 ) ;
#26254=VERTEX_POINT ( 'NONE', #34916 ) ;
#26256=VECTOR ( 'NONE', #34787, 1000.000000000000000 ) ;
#26257=CARTESIAN_POINT ( 'NONE',  ( 31.09745072740910388, 83.47442710120324705, -5.000000000000011546 ) ) ;
#26259=ORIENTED_EDGE ( 'NONE', *, *, #20342, .T. ) ;
#26262=DIRECTION ( 'NONE',  ( 0.000000000000000000, 0.000000000000000000, 1.000000000000000000 ) ) ;
#26263=AXIS2_PLACEMENT_3D ( 'NONE', #308, #28814, #35213 ) ;
#26264=ORIENTED_EDGE ( 'NONE', *, *, #32534, .F. ) ;
#26266=EDGE_CURVE ( 'NONE', #6635, #7505, #6404, .T. ) ;
#26268=AXIS2_PLACEMENT_3D ( 'NONE', #27189, #1506, #30192 ) ;
#26269=DIRECTION ( 'NONE',  ( 0.8660254037844337116, -0.5000000000000084377, 0.000000000000000000 ) ) ;
#26270=CARTESIAN_POINT ( 'NONE',  ( 52.39915983220795681, 35.19434990244919703, -4.999999999999997335 ) ) ;
#26271=DIRECTION ( 'NONE',  ( 1.000000000000000000, 0.000000000000000000, 0.000000000000000000 ) ) ;
#26273=VECTOR ( 'NONE', #15640, 1000.000000000000000 ) ;
#26274=FACE_OUTER_BOUND ( 'NONE', #17003, .T. ) ;
#26275=FACE_OUTER_BOUND ( 'NONE', #33794, .T. ) ;
#26276=DIRECTION ( 'NONE',  ( 0.000000000000000000, 0.000000000000000000, 1.000000000000000000 ) ) ;
#26277=ORIENTED_EDGE ( 'NONE', *, *, #12263, .F. ) ;
#26280=CARTESIAN_POINT ( 'NONE',  ( -60.00000337463108480, -51.96152422706641971, 17.49999999999999645 ) ) ;
#26281=ORIENTED_EDGE ( 'NONE', *, *, #14400, .T. ) ;
#26283=DIRECTION ( 'NONE',  ( 0.000000000000000000, 0.000000000000000000, 1.000000000000000000 ) ) ;
#26285=CIRCLE ( 'NONE', #28081, 2.000000000000001776 ) ;
#26287=ORIENTED_EDGE ( 'NONE', *, *, #29972, .T. ) ;
#26288=EDGE_LOOP ( 'NONE', ( #14006, #12676, #7598, #21467 ) ) ;
#26290=EDGE_CURVE ( 'NONE', #26576, #9227, #7166, .T. ) ;
#26291=DIRECTION ( 'NONE',  ( 0.000000000000000000, 0.000000000000000000, 1.000000000000000000 ) ) ;
#26292=DIRECTION ( 'NONE',  ( 1.000000000000000000, 0.000000000000000000, 0.000000000000000000 ) ) ;
#26293=VERTEX_POINT ( 'NONE', #23857 ) ;
#26294=LINE ( 'NONE', #12019, #33936 ) ;
#26295=CIRCLE ( 'NONE', #24517, 2.000000000000001776 ) ;
#26297=FACE_BOUND ( 'NONE', #8985, .T. ) ;
#26299=DIRECTION ( 'NONE',  ( 1.000000000000000000, 0.000000000000000000, 0.000000000000000000 ) ) ;
#26300=FACE_OUTER_BOUND ( 'NONE', #30414, .T. ) ;
#26301=CARTESIAN_POINT ( 'NONE',  ( 44.99999662536851019, 77.94228634059959404, -5.000000000000000000 ) ) ;
#26302=ORIENTED_EDGE ( 'NONE', *, *, #25267, .T. ) ;
#26303=DIRECTION ( 'NONE',  ( -1.000000000000000000, 0.000000000000000000, 0.000000000000000000 ) ) ;
#26304=CARTESIAN_POINT ( 'NONE',  ( 76.99999662536836809, -8.660254037844401509, -9.999999999999998224 ) ) ;
#26305=DIRECTION ( 'NONE',  ( 0.000000000000000000, 0.000000000000000000, 1.000000000000000000 ) ) ;
#26306=ORIENTED_EDGE ( 'NONE', *, *, #21242, .T. ) ;
#26307=LINE ( 'NONE', #619, #28605 ) ;
#26308=EDGE_CURVE ( 'NONE', #29824, #26391, #2838, .T. ) ;
#26310=CARTESIAN_POINT ( 'NONE',  ( -8.000003374631278419, -69.28203230275519786, -5.000000000000000000 ) ) ;
#26312=EDGE_LOOP ( 'NONE', ( #5549, #18455, #3024, #12736 ) ) ;
#26313=ORIENTED_EDGE ( 'NONE', *, *, #16201, .T. ) ;
#26315=EDGE_LOOP ( 'NONE', ( #18484, #28517, #12205, #948 ) ) ;
#26317=CARTESIAN_POINT ( 'NONE',  ( -73.00000337463097821, -8.660254037844422825, -9.999999999999998224 ) ) ;
#26319=CIRCLE ( 'NONE', #31105, 2.000000000000001776 ) ;
#26320=CARTESIAN_POINT ( 'NONE',  ( -92.00000337463090716, -1.016341149603137227E-14, 17.49999999999999645 ) ) ;
#26321=ORIENTED_EDGE ( 'NONE', *, *, #32534, .T. ) ;
#26322=VERTEX_POINT ( 'NONE', #21765 ) ;
#26323=DIRECTION ( 'NONE',  ( -1.000000000000000000, 0.000000000000000000, 0.000000000000000000 ) ) ;
#26324=CIRCLE ( 'NONE', #23331, 2.000000000000001776 ) ;
#26325=EDGE_LOOP ( 'NONE', ( #36234, #31365, #27243, #18254 ) ) ;
#26326=CYLINDRICAL_SURFACE ( 'NONE', #6001, 2.000000000000000000 ) ;
#26327=ORIENTED_EDGE ( 'NONE', *, *, #29661, .F. ) ;
#26329=VERTEX_POINT ( 'NONE', #26848 ) ;
#26330=ORIENTED_EDGE ( 'NONE', *, *, #25173, .F. ) ;
#26331=EDGE_CURVE ( 'NONE', #29105, #29077, #35760, .T. ) ;
#26332=DIRECTION ( 'NONE',  ( 1.000000000000000000, 0.000000000000000000, 0.000000000000000000 ) ) ;
#26334=DIRECTION ( 'NONE',  ( 0.000000000000000000, 0.000000000000000000, 1.000000000000000000 ) ) ;
#26335=ORIENTED_EDGE ( 'NONE', *, *, #26338, .T. ) ;
#26336=FACE_OUTER_BOUND ( 'NONE', #2643, .T. ) ;
#26337=CIRCLE ( 'NONE', #14963, 2.000000000000001776 ) ;
#26338=EDGE_CURVE ( 'NONE', #8840, #30504, #19590, .T. ) ;
#26339=LINE ( 'NONE', #11346, #22849 ) ;
#26340=DIRECTION ( 'NONE',  ( 0.000000000000000000, 0.000000000000000000, 1.000000000000000000 ) ) ;
#26342=EDGE_LOOP ( 'NONE', ( #31706, #26420 ) ) ;
#26343=DIRECTION ( 'NONE',  ( 0.000000000000000000, 0.000000000000000000, 1.000000000000000000 ) ) ;
#26344=CARTESIAN_POINT ( 'NONE',  ( 67.99999662536836809, -51.96152422706639840, 17.49999999999999645 ) ) ;
#26346=ORIENTED_EDGE ( 'NONE', *, *, #31640, .T. ) ;
#26347=CARTESIAN_POINT ( 'NONE',  ( -47.00000337463112743, -60.62177826491080168, 17.49999999999999645 ) ) ;
#26349=CARTESIAN_POINT ( 'NONE',  ( -83.00000337463092137, 8.660254037844389075, -9.999999999999998224 ) ) ;
#26350=DIRECTION ( 'NONE',  ( -1.000000000000000000, 0.000000000000000000, 0.000000000000000000 ) ) ;
#26351=CARTESIAN_POINT ( 'NONE',  ( 2.778182860042563540, -69.13212189986967360, -49.86348611802629449 ) ) ;
#26352=DIRECTION ( 'NONE',  ( 1.000000000000000000, 0.000000000000000000, 0.000000000000000000 ) ) ;
#26353=ORIENTED_EDGE ( 'NONE', *, *, #20843, .T. ) ;
#26354=DIRECTION ( 'NONE',  ( -1.000000000000000000, 0.000000000000000000, 0.000000000000000000 ) ) ;
#26355=AXIS2_PLACEMENT_3D ( 'NONE', #2541, #31582, #30837 ) ;
#26356=DIRECTION ( 'NONE',  ( -1.000000000000000000, 0.000000000000000000, 0.000000000000000000 ) ) ;
#26357=DIRECTION ( 'NONE',  ( 1.000000000000000000, 0.000000000000000000, 0.000000000000000000 ) ) ;
#26359=ORIENTED_EDGE ( 'NONE', *, *, #30184, .F. ) ;
#26360=ORIENTED_EDGE ( 'NONE', *, *, #9239, .F. ) ;
#26361=ADVANCED_FACE ( 'NONE', ( #7522 ), #10167, .F. ) ;
#26362=DIRECTION ( 'NONE',  ( 0.000000000000000000, 0.000000000000000000, 1.000000000000000000 ) ) ;
#26363=FACE_OUTER_BOUND ( 'NONE', #715, .T. ) ;
#26364=AXIS2_PLACEMENT_3D ( 'NONE', #29468, #24745, #3788 ) ;
#26365=FACE_OUTER_BOUND ( 'NONE', #21549, .T. ) ;
#26366=AXIS2_PLACEMENT_3D ( 'NONE', #19498, #23233, #19864 ) ;
#26367=DIRECTION ( 'NONE',  ( 0.000000000000000000, 0.000000000000000000, -1.000000000000000000 ) ) ;
#26369=AXIS2_PLACEMENT_3D ( 'NONE', #36769, #33776, #22332 ) ;
#26370=CARTESIAN_POINT ( 'NONE',  ( 24.99999662536859546, -77.94228634059960825, 17.49999999999999645 ) ) ;
#26372=FACE_BOUND ( 'NONE', #30032, .T. ) ;
#26373=AXIS2_PLACEMENT_3D ( 'NONE', #15001, #26426, #35054 ) ;
#26375=LINE ( 'NONE', #3302, #32299 ) ;
#26376=LINE ( 'NONE', #3096, #20277 ) ;
#26377=EDGE_CURVE ( 'NONE', #911, #10350, #25005, .T. ) ;
#26381=ADVANCED_FACE ( 'NONE', ( #15774 ), #35655, .F. ) ;
#26382=DIRECTION ( 'NONE',  ( 1.000000000000000000, 0.000000000000000000, 0.000000000000000000 ) ) ;
#26383=CARTESIAN_POINT ( 'NONE',  ( 21.99999662536859191, 69.28203230275516944, -9.999999999999998224 ) ) ;
#26385=EDGE_LOOP ( 'NONE', ( #1741, #33403, #22952, #1616 ) ) ;
#26386=CARTESIAN_POINT ( 'NONE',  ( 16.99999662536863454, -77.94228634059960825, -9.999999999999998224 ) ) ;
#26388=LINE ( 'NONE', #26202, #5279 ) ;
#26389=FACE_OUTER_BOUND ( 'NONE', #1834, .T. ) ;
#26390=EDGE_CURVE ( 'NONE', #3002, #1135, #12382, .T. ) ;
#26391=VERTEX_POINT ( 'NONE', #32639 ) ;
#26392=EDGE_LOOP ( 'NONE', ( #35420, #14146, #14182, #17220, #9714 ) ) ;
#26393=VECTOR ( 'NONE', #28648, 1000.000000000000000 ) ;
#26397=EDGE_CURVE ( 'NONE', #3085, #6951, #19333, .T. ) ;
#26399=EDGE_CURVE ( 'NONE', #5530, #35823, #24382, .T. ) ;
#26400=EDGE_CURVE ( 'NONE', #28159, #27693, #33969, .T. ) ;
#26401=CARTESIAN_POINT ( 'NONE',  ( -75.00000337463097821, -8.660254037844422825, 17.49999999999999645 ) ) ;
#26402=CARTESIAN_POINT ( 'NONE',  ( 6.999996625368676284, -77.94228634059960825, -9.999999999999998224 ) ) ;
#26403=DIRECTION ( 'NONE',  ( 0.000000000000000000, 0.000000000000000000, 1.000000000000000000 ) ) ;
#26404=CYLINDRICAL_SURFACE ( 'NONE', #11386, 2.000000000000000000 ) ;
#26406=VERTEX_POINT ( 'NONE', #2274 ) ;
#26408=DIRECTION ( 'NONE',  ( 1.000000000000000000, 0.000000000000000000, 0.000000000000000000 ) ) ;
#26409=DIRECTION ( 'NONE',  ( 1.000000000000000000, 0.000000000000000000, 0.000000000000000000 ) ) ;
#26411=FACE_BOUND ( 'NONE', #28424, .T. ) ;
#26412=ORIENTED_EDGE ( 'NONE', *, *, #11014, .F. ) ;
#26413=EDGE_LOOP ( 'NONE', ( #36901, #34057 ) ) ;
#26414=DIRECTION ( 'NONE',  ( 0.000000000000000000, 0.000000000000000000, -1.000000000000000000 ) ) ;
#26415=VERTEX_POINT ( 'NONE', #33404 ) ;
#26417=DIRECTION ( 'NONE',  ( 0.000000000000000000, 0.000000000000000000, -1.000000000000000000 ) ) ;
#26418=CARTESIAN_POINT ( 'NONE',  ( -55.00000337463107059, 60.62177826491078747, -9.999999999999998224 ) ) ;
#26420=ORIENTED_EDGE ( 'NONE', *, *, #1683, .T. ) ;
#26421=ORIENTED_EDGE ( 'NONE', *, *, #21004, .T. ) ;
#26422=VERTEX_POINT ( 'NONE', #5283 ) ;
#26423=VERTEX_POINT ( 'NONE', #30587 ) ;
#26424=ORIENTED_EDGE ( 'NONE', *, *, #34442, .T. ) ;
#26426=DIRECTION ( 'NONE',  ( 0.000000000000000000, 0.000000000000000000, 1.000000000000000000 ) ) ;
#26427=ORIENTED_EDGE ( 'NONE', *, *, #23362, .T. ) ;
#26428=CIRCLE ( 'NONE', #16255, 2.000000000000001776 ) ;
#26429=DIRECTION ( 'NONE',  ( 0.000000000000000000, 0.000000000000000000, 1.000000000000000000 ) ) ;
#26432=EDGE_LOOP ( 'NONE', ( #36981, #26868, #14615, #11403 ) ) ;
#26433=CARTESIAN_POINT ( 'NONE',  ( -22.00000337463124112, -86.60254037844400443, -9.999999999999998224 ) ) ;
#26434=DIRECTION ( 'NONE',  ( 1.000000000000000000, 0.000000000000000000, 0.000000000000000000 ) ) ;
#26435=EDGE_CURVE ( 'NONE', #1584, #23264, #30364, .T. ) ;
#26436=CARTESIAN_POINT ( 'NONE',  ( 69.99999662536839651, 34.64101615137758472, -9.999999999999998224 ) ) ;
#26437=VERTEX_POINT ( 'NONE', #19518 ) ;
#26438=DIRECTION ( 'NONE',  ( 0.000000000000000000, 0.000000000000000000, 1.000000000000000000 ) ) ;
#26439=DIRECTION ( 'NONE',  ( 1.000000000000000000, 0.000000000000000000, 0.000000000000000000 ) ) ;
#26441=ORIENTED_EDGE ( 'NONE', *, *, #1313, .T. ) ;
#26442=CARTESIAN_POINT ( 'NONE',  ( 62.97617850287784336, 4.279621169095339184, -4.999999999999997335 ) ) ;
#26443=DIRECTION ( 'NONE',  ( 0.000000000000000000, 0.000000000000000000, -1.000000000000000000 ) ) ;
#26444=DIRECTION ( 'NONE',  ( -0.000000000000000000, 0.000000000000000000, -1.000000000000000000 ) ) ;
#26446=ORIENTED_EDGE ( 'NONE', *, *, #31527, .T. ) ;
#26447=DIRECTION ( 'NONE',  ( 0.000000000000000000, 0.000000000000000000, 1.000000000000000000 ) ) ;
#26448=CARTESIAN_POINT ( 'NONE',  ( 74.99999662536836809, -8.660254037844401509, -9.999999999999998224 ) ) ;
#26449=ORIENTED_EDGE ( 'NONE', *, *, #15537, .F. ) ;
#26450=VECTOR ( 'NONE', #18645, 1000.000000000000000 ) ;
#26453=EDGE_CURVE ( 'NONE', #28884, #7742, #29766, .T. ) ;
#26454=EDGE_CURVE ( 'NONE', #32590, #35393, #28569, .T. ) ;
#26455=LINE ( 'NONE', #6395, #22302 ) ;
#26456=DIRECTION ( 'NONE',  ( 0.000000000000000000, 0.000000000000000000, 1.000000000000000000 ) ) ;
#26457=DIRECTION ( 'NONE',  ( -0.000000000000000000, -0.000000000000000000, 1.000000000000000000 ) ) ;
#26458=VERTEX_POINT ( 'NONE', #33767 ) ;
#26459=ORIENTED_EDGE ( 'NONE', *, *, #4433, .T. ) ;
#26460=CARTESIAN_POINT ( 'NONE',  ( -57.00000337463107059, 60.62177826491078747, 12.50000000000000000 ) ) ;
#26462=DIRECTION ( 'NONE',  ( 0.000000000000000000, 0.000000000000000000, -1.000000000000000000 ) ) ;
#26464=ORIENTED_EDGE ( 'NONE', *, *, #11445, .F. ) ;
#26465=DIRECTION ( 'NONE',  ( 0.000000000000000000, 0.000000000000000000, 1.000000000000000000 ) ) ;
#26466=FACE_BOUND ( 'NONE', #32703, .T. ) ;
#26468=CARTESIAN_POINT ( 'NONE',  ( 51.13139720814417899, 27.49999999999988987, -10.00000000000000178 ) ) ;
#26469=LINE ( 'NONE', #3777, #36296 ) ;
#26472=CYLINDRICAL_SURFACE ( 'NONE', #9589, 2.000000000000001776 ) ;
#26473=VECTOR ( 'NONE', #28548, 1000.000000000000000 ) ;
#26474=EDGE_CURVE ( 'NONE', #27967, #5647, #29738, .T. ) ;
#26477=DIRECTION ( 'NONE',  ( 0.000000000000000000, 0.000000000000000000, 1.000000000000000000 ) ) ;
#26478=CARTESIAN_POINT ( 'NONE',  ( -90.60231327712325822, -15.97563234535699017, -4.999999999999997335 ) ) ;
#26479=CARTESIAN_POINT ( 'NONE',  ( -62.33939050065184517, 13.89091430021398565, 12.49999999999999822 ) ) ;
#26480=ORIENTED_EDGE ( 'NONE', *, *, #24863, .F. ) ;
#26484=DIRECTION ( 'NONE',  ( 1.000000000000000000, 0.000000000000000000, 0.000000000000000000 ) ) ;
#26485=DIRECTION ( 'NONE',  ( 1.000000000000000000, 0.000000000000000000, 0.000000000000000000 ) ) ;
#26486=ORIENTED_EDGE ( 'NONE', *, *, #13539, .F. ) ;
#26487=ORIENTED_EDGE ( 'NONE', *, *, #28214, .F. ) ;
#26488=EDGE_LOOP ( 'NONE', ( #7857, #19123, #19623, #10276 ) ) ;
#26490=AXIS2_PLACEMENT_3D ( 'NONE', #3080, #9056, #32099 ) ;
#26492=EDGE_CURVE ( 'NONE', #4407, #24647, #15408, .T. ) ;
#26494=VERTEX_POINT ( 'NONE', #8276 ) ;
#26496=ORIENTED_EDGE ( 'NONE', *, *, #36239, .F. ) ;
#26498=ORIENTED_EDGE ( 'NONE', *, *, #6322, .T. ) ;
#26499=DIRECTION ( 'NONE',  ( 1.000000000000000000, 0.000000000000000000, 0.000000000000000000 ) ) ;
#26500=FACE_BOUND ( 'NONE', #6610, .T. ) ;
#26501=AXIS2_PLACEMENT_3D ( 'NONE', #35449, #6366, #23442 ) ;
#26502=DIRECTION ( 'NONE',  ( -1.000000000000000000, 0.000000000000000000, 0.000000000000000000 ) ) ;
#26503=ORIENTED_EDGE ( 'NONE', *, *, #1109, .T. ) ;
#26504=VECTOR ( 'NONE', #25220, 1000.000000000000000 ) ;
#26506=EDGE_LOOP ( 'NONE', ( #504, #1525 ) ) ;
#26510=LINE ( 'NONE', #9256, #26256 ) ;
#26511=EDGE_CURVE ( 'NONE', #22230, #7750, #18382, .T. ) ;
#26512=ORIENTED_EDGE ( 'NONE', *, *, #25228, .T. ) ;
#26514=CARTESIAN_POINT ( 'NONE',  ( 0.000000000000000000, 0.000000000000000000, -10.00000000000000000 ) ) ;
#26515=VERTEX_POINT ( 'NONE', #14057 ) ;
#26516=DIRECTION ( 'NONE',  ( 0.000000000000000000, 0.000000000000000000, 1.000000000000000000 ) ) ;
#26517=CARTESIAN_POINT ( 'NONE',  ( 74.99999662536836809, 43.30127018922198801, -9.999999999999998224 ) ) ;
#26519=DIRECTION ( 'NONE',  ( 0.000000000000000000, 0.000000000000000000, -1.000000000000000000 ) ) ;
#26520=CIRCLE ( 'NONE', #27106, 2.000000000000001776 ) ;
#26521=DIRECTION ( 'NONE',  ( 0.000000000000000000, 0.000000000000000000, 1.000000000000000000 ) ) ;
#26523=EDGE_LOOP ( 'NONE', ( #19748, #34937 ) ) ;
#26527=VERTEX_POINT ( 'NONE', #8452 ) ;
#26529=VERTEX_POINT ( 'NONE', #24971 ) ;
#26530=VERTEX_POINT ( 'NONE', #11062 ) ;
#26531=AXIS2_PLACEMENT_3D ( 'NONE', #32341, #24089, #32702 ) ;
#26533=DIRECTION ( 'NONE',  ( 1.000000000000000000, 0.000000000000000000, 0.000000000000000000 ) ) ;
#26534=LINE ( 'NONE', #34985, #27855 ) ;
#26535=EDGE_CURVE ( 'NONE', #15669, #30855, #22581, .T. ) ;
#26536=CARTESIAN_POINT ( 'NONE',  ( -13.00000337463125710, -77.94228634059960825, -9.999999999999998224 ) ) ;
#26537=DIRECTION ( 'NONE',  ( 0.000000000000000000, 0.000000000000000000, 1.000000000000000000 ) ) ;
#26538=ORIENTED_EDGE ( 'NONE', *, *, #879, .T. ) ;
#26539=EDGE_CURVE ( 'NONE', #22136, #25902, #23788, .T. ) ;
#26540=DIRECTION ( 'NONE',  ( 1.000000000000000000, 0.000000000000000000, 0.000000000000000000 ) ) ;
#26541=EDGE_LOOP ( 'NONE', ( #4207, #24630 ) ) ;
#26542=FACE_BOUND ( 'NONE', #30234, .T. ) ;
#26543=VECTOR ( 'NONE', #12603, 1000.000000000000000 ) ;
#26545=DIRECTION ( 'NONE',  ( 1.000000000000000000, 0.000000000000000000, 0.000000000000000000 ) ) ;
#26547=ORIENTED_EDGE ( 'NONE', *, *, #1951, .T. ) ;
#26548=CARTESIAN_POINT ( 'NONE',  ( -77.00000337463099243, -25.98076211353322051, -9.999999999999998224 ) ) ;
#26550=VECTOR ( 'NONE', #23020, 1000.000000000000000 ) ;
#26551=CYLINDRICAL_SURFACE ( 'NONE', #17077, 2.000000000000001776 ) ;
#26552=EDGE_CURVE ( 'NONE', #34764, #12419, #9404, .T. ) ;
#26553=FACE_OUTER_BOUND ( 'NONE', #1341, .T. ) ;
#26554=DIRECTION ( 'NONE',  ( 1.000000000000000000, 0.000000000000000000, 0.000000000000000000 ) ) ;
#26555=VERTEX_POINT ( 'NONE', #20593 ) ;
#26556=CARTESIAN_POINT ( 'NONE',  ( 69.99999662536839651, 34.64101615137758472, -9.999999999999998224 ) ) ;
#26558=DIRECTION ( 'NONE',  ( 1.000000000000000000, 0.000000000000000000, 0.000000000000000000 ) ) ;
#26559=CIRCLE ( 'NONE', #9181, 33.00000000000002132 ) ;
#26560=ORIENTED_EDGE ( 'NONE', *, *, #36802, .F. ) ;
#26561=ORIENTED_EDGE ( 'NONE', *, *, #24704, .F. ) ;
#26563=LINE ( 'NONE', #12503, #6357 ) ;
#26564=FACE_OUTER_BOUND ( 'NONE', #4281, .T. ) ;
#26565=AXIS2_PLACEMENT_3D ( 'NONE', #2391, #19264, #19632 ) ;
#26566=DIRECTION ( 'NONE',  ( -0.000000000000000000, 0.000000000000000000, -1.000000000000000000 ) ) ;
#26567=EDGE_CURVE ( 'NONE', #32112, #27460, #33376, .T. ) ;
#26568=ORIENTED_EDGE ( 'NONE', *, *, #26593, .T. ) ;
#26569=CARTESIAN_POINT ( 'NONE',  ( -52.00000337463109190, 51.96152422706637708, -5.000000000000000000 ) ) ;
#26570=CARTESIAN_POINT ( 'NONE',  ( -35.00000337463116296, 60.62177826491077326, -5.000000000000000000 ) ) ;
#26571=EDGE_CURVE ( 'NONE', #25853, #2100, #1034, .T. ) ;
#26572=DIRECTION ( 'NONE',  ( 0.000000000000000000, 0.000000000000000000, 1.000000000000000000 ) ) ;
#26573=ORIENTED_EDGE ( 'NONE', *, *, #19299, .F. ) ;
#26575=ADVANCED_FACE ( 'NONE', ( #11792 ), #29032, .F. ) ;
#26576=VERTEX_POINT ( 'NONE', #20054 ) ;
#26577=CARTESIAN_POINT ( 'NONE',  ( 82.99999662536831124, -8.660254037844397956, -5.000000000000000000 ) ) ;
#26579=ORIENTED_EDGE ( 'NONE', *, *, #25447, .F. ) ;
#26583=EDGE_CURVE ( 'NONE', #4105, #23009, #14265, .T. ) ;
#26584=FACE_BOUND ( 'NONE', #32794, .T. ) ;
#26585=ORIENTED_EDGE ( 'NONE', *, *, #3508, .F. ) ;
#26586=ORIENTED_EDGE ( 'NONE', *, *, #26069, .F. ) ;
#26587=DIRECTION ( 'NONE',  ( 0.000000000000000000, 0.000000000000000000, 1.000000000000000000 ) ) ;
#26588=ORIENTED_EDGE ( 'NONE', *, *, #22761, .T. ) ;
#26589=EDGE_CURVE ( 'NONE', #32244, #538, #14609, .T. ) ;
#26591=ADVANCED_FACE ( 'NONE', ( #5824 ), #11436, .T. ) ;
#26593=EDGE_CURVE ( 'NONE', #10050, #34413, #23032, .T. ) ;
#26596=EDGE_LOOP ( 'NONE', ( #29575, #20844 ) ) ;
#26598=EDGE_LOOP ( 'NONE', ( #4374, #36165, #25989, #26877 ) ) ;
#26599=ORIENTED_EDGE ( 'NONE', *, *, #14653, .F. ) ;
#26600=ORIENTED_EDGE ( 'NONE', *, *, #34929, .T. ) ;
#26601=ORIENTED_EDGE ( 'NONE', *, *, #1024, .F. ) ;
#26602=DIRECTION ( 'NONE',  ( 0.000000000000000000, 0.000000000000000000, 1.000000000000000000 ) ) ;
#26604=CARTESIAN_POINT ( 'NONE',  ( 37.99999662536853151, -69.28203230275519786, -5.000000000000000000 ) ) ;
#26606=DIRECTION ( 'NONE',  ( 1.000000000000000000, 0.000000000000000000, 0.000000000000000000 ) ) ;
#26607=DIRECTION ( 'NONE',  ( 0.000000000000000000, 0.000000000000000000, 1.000000000000000000 ) ) ;
#26611=DIRECTION ( 'NONE',  ( -0.000000000000000000, -0.000000000000000000, 1.000000000000000000 ) ) ;
#26612=EDGE_CURVE ( 'NONE', #12595, #29485, #34422, .T. ) ;
#26614=DIRECTION ( 'NONE',  ( 1.000000000000000000, 0.000000000000000000, 0.000000000000000000 ) ) ;
#26615=ORIENTED_EDGE ( 'NONE', *, *, #28174, .F. ) ;
#26616=CARTESIAN_POINT ( 'NONE',  ( 34.99999662536855283, -77.94228634059960825, 17.49999999999999645 ) ) ;
#26617=AXIS2_PLACEMENT_3D ( 'NONE', #19619, #28051, #14363 ) ;
#26618=LINE ( 'NONE', #9574, #29748 ) ;
#26620=AXIS2_PLACEMENT_3D ( 'NONE', #10690, #1312, #9936 ) ;
#26621=EDGE_LOOP ( 'NONE', ( #6284, #30115 ) ) ;
#26622=DIRECTION ( 'NONE',  ( 1.000000000000000000, 0.000000000000000000, 0.000000000000000000 ) ) ;
#26623=FACE_OUTER_BOUND ( 'NONE', #28113, .T. ) ;
#26624=DIRECTION ( 'NONE',  ( -1.000000000000000000, 0.000000000000000000, 0.000000000000000000 ) ) ;
#26625=DIRECTION ( 'NONE',  ( 0.000000000000000000, 0.000000000000000000, -1.000000000000000000 ) ) ;
#26626=EDGE_CURVE ( 'NONE', #6836, #23569, #17036, .T. ) ;
#26628=VECTOR ( 'NONE', #35041, 1000.000000000000000 ) ;
#26630=CIRCLE ( 'NONE', #8065, 2.000000000000001776 ) ;
#26631=DIRECTION ( 'NONE',  ( 0.000000000000000000, 0.000000000000000000, 1.000000000000000000 ) ) ;
#26632=CIRCLE ( 'NONE', #6879, 2.000000000000001776 ) ;
#26634=ORIENTED_EDGE ( 'NONE', *, *, #15630, .F. ) ;
#26635=LINE ( 'NONE', #1325, #18997 ) ;
#26637=CARTESIAN_POINT ( 'NONE',  ( -30.00000337463118427, 69.28203230275516944, -5.000000000000000000 ) ) ;
#26638=ADVANCED_FACE ( 'NONE', ( #34873 ), #6014, .F. ) ;
#26639=DIRECTION ( 'NONE',  ( 1.000000000000000000, 0.000000000000000000, 0.000000000000000000 ) ) ;
#26640=EDGE_CURVE ( 'NONE', #4245, #25195, #12825, .T. ) ;
#26642=CARTESIAN_POINT ( 'NONE',  ( 64.99999662536839651, -43.30127018922199511, -9.999999999999998224 ) ) ;
#26643=EDGE_CURVE ( 'NONE', #29480, #33530, #3867, .T. ) ;
#26645=AXIS2_PLACEMENT_3D ( 'NONE', #15267, #14717, #23360 ) ;
#26647=AXIS2_PLACEMENT_3D ( 'NONE', #15892, #29959, #21527 ) ;
#26648=DIRECTION ( 'NONE',  ( 0.000000000000000000, 0.000000000000000000, 1.000000000000000000 ) ) ;
#26651=DIRECTION ( 'NONE',  ( 0.000000000000000000, 0.000000000000000000, -1.000000000000000000 ) ) ;
#26652=DIRECTION ( 'NONE',  ( 0.000000000000000000, 0.000000000000000000, 1.000000000000000000 ) ) ;
#26653=DIRECTION ( 'NONE',  ( 0.000000000000000000, 0.000000000000000000, 1.000000000000000000 ) ) ;
#26654=CARTESIAN_POINT ( 'NONE',  ( 76.99999662536835388, -43.30127018922199511, 12.50000000000000000 ) ) ;
#26656=EDGE_LOOP ( 'NONE', ( #20930, #9449, #1551, #6081, #22260, #24130 ) ) ;
#26657=DIRECTION ( 'NONE',  ( 0.000000000000000000, 0.000000000000000000, -1.000000000000000000 ) ) ;
#26658=CIRCLE ( 'NONE', #26038, 2.000000000000001776 ) ;
#26659=VECTOR ( 'NONE', #13271, 1000.000000000000000 ) ;
#26662=DIRECTION ( 'NONE',  ( 0.000000000000000000, 0.000000000000000000, 1.000000000000000000 ) ) ;
#26665=FACE_BOUND ( 'NONE', #29230, .T. ) ;
#26666=CARTESIAN_POINT ( 'NONE',  ( -65.00000337463106348, -60.62177826491083010, -9.999999999999998224 ) ) ;
#26667=EDGE_CURVE ( 'NONE', #807, #21781, #28406, .T. ) ;
#26669=ORIENTED_EDGE ( 'NONE', *, *, #35368, .F. ) ;
#26671=CARTESIAN_POINT ( 'NONE',  ( -33.00000337463116296, 60.62177826491077326, -9.999999999999998224 ) ) ;
#26672=FACE_OUTER_BOUND ( 'NONE', #34342, .T. ) ;
#26673=DIRECTION ( 'NONE',  ( 1.000000000000000000, 0.000000000000000000, 0.000000000000000000 ) ) ;
#26675=ORIENTED_EDGE ( 'NONE', *, *, #9061, .F. ) ;
#26676=VERTEX_POINT ( 'NONE', #25709 ) ;
#26678=VECTOR ( 'NONE', #30819, 1000.000000000000000 ) ;
#26679=AXIS2_PLACEMENT_3D ( 'NONE', #3113, #3834, #3666 ) ;
#26680=AXIS2_PLACEMENT_3D ( 'NONE', #14844, #12373, #14642 ) ;
#26681=ORIENTED_EDGE ( 'NONE', *, *, #34659, .F. ) ;
#26682=CARTESIAN_POINT ( 'NONE',  ( -70.00000337463100664, -17.32050807568882078, -5.000000000000000000 ) ) ;
#26683=EDGE_LOOP ( 'NONE', ( #24594, #31110 ) ) ;
#26684=DIRECTION ( 'NONE',  ( 0.000000000000000000, 0.000000000000000000, -1.000000000000000000 ) ) ;
#26686=ORIENTED_EDGE ( 'NONE', *, *, #23643, .T. ) ;
#26687=CYLINDRICAL_SURFACE ( 'NONE', #9454, 2.000000000000001776 ) ;
#26689=EDGE_CURVE ( 'NONE', #34742, #18010, #6363, .T. ) ;
#26690=EDGE_LOOP ( 'NONE', ( #11242, #5401 ) ) ;
#26691=ORIENTED_EDGE ( 'NONE', *, *, #26689, .T. ) ;
#26692=DIRECTION ( 'NONE',  ( 0.000000000000000000, 0.000000000000000000, 1.000000000000000000 ) ) ;
#26696=VERTEX_POINT ( 'NONE', #20795 ) ;
#26697=DIRECTION ( 'NONE',  ( 0.000000000000000000, 0.000000000000000000, 1.000000000000000000 ) ) ;
#26698=DIRECTION ( 'NONE',  ( 0.000000000000000000, 0.000000000000000000, -1.000000000000000000 ) ) ;
#26699=ORIENTED_EDGE ( 'NONE', *, *, #28441, .T. ) ;
#26700=CYLINDRICAL_SURFACE ( 'NONE', #22631, 2.000000000000001776 ) ;
#26701=CIRCLE ( 'NONE', #32052, 1.999999999999998224 ) ;
#26702=CARTESIAN_POINT ( 'NONE',  ( -70.00000337463099243, 51.96152422706637708, 17.49999999999999645 ) ) ;
#26703=CARTESIAN_POINT ( 'NONE',  ( 29.99999662536857770, -69.28203230275519786, -9.999999999999998224 ) ) ;
#26704=CIRCLE ( 'NONE', #23121, 1.999999999999998224 ) ;
#26707=AXIS2_PLACEMENT_3D ( 'NONE', #36646, #10940, #22380 ) ;
#26708=CIRCLE ( 'NONE', #6360, 2.000000000000001776 ) ;
#26709=DIRECTION ( 'NONE',  ( -1.000000000000000000, 0.000000000000000000, 0.000000000000000000 ) ) ;
#26711=VERTEX_POINT ( 'NONE', #32231 ) ;
#26712=CARTESIAN_POINT ( 'NONE',  ( 76.99999662536836809, -8.660254037844401509, 12.50000000000000000 ) ) ;
#26713=CARTESIAN_POINT ( 'NONE',  ( 54.99999662536844625, -60.62177826491080168, -9.999999999999998224 ) ) ;
#26714=DIRECTION ( 'NONE',  ( 0.000000000000000000, 0.000000000000000000, 1.000000000000000000 ) ) ;
#26715=EDGE_CURVE ( 'NONE', #36483, #32323, #2828, .T. ) ;
#26716=EDGE_LOOP ( 'NONE', ( #1404, #32652, #3942, #6768 ) ) ;
#26717=AXIS2_PLACEMENT_3D ( 'NONE', #16051, #1968, #24497 ) ;
#26718=ORIENTED_EDGE ( 'NONE', *, *, #6209, .T. ) ;
#26720=DIRECTION ( 'NONE',  ( 0.000000000000000000, 0.000000000000000000, -1.000000000000000000 ) ) ;
#26721=CARTESIAN_POINT ( 'NONE',  ( -10.00000337463128197, 86.60254037844397601, -5.000000000000000000 ) ) ;
#26722=ADVANCED_FACE ( 'NONE', ( #12906 ), #35998, .T. ) ;
#26723=DIRECTION ( 'NONE',  ( 1.000000000000000000, 0.000000000000000000, 0.000000000000000000 ) ) ;
#26724=AXIS2_PLACEMENT_3D ( 'NONE', #29501, #15260, #29887 ) ;
#26725=DIRECTION ( 'NONE',  ( 0.000000000000000000, 0.000000000000000000, 1.000000000000000000 ) ) ;
#26726=EDGE_CURVE ( 'NONE', #7613, #1450, #36212, .T. ) ;
#26727=AXIS2_PLACEMENT_3D ( 'NONE', #12392, #4347, #1725 ) ;
#26728=LINE ( 'NONE', #36482, #33892 ) ;
#26729=ORIENTED_EDGE ( 'NONE', *, *, #7083, .F. ) ;
#26733=FACE_BOUND ( 'NONE', #18975, .T. ) ;
#26734=AXIS2_PLACEMENT_3D ( 'NONE', #16041, #27818, #18846 ) ;
#26735=CIRCLE ( 'NONE', #22534, 2.000000000000001776 ) ;
#26736=AXIS2_PLACEMENT_3D ( 'NONE', #8963, #23213, #14962 ) ;
#26737=AXIS2_PLACEMENT_3D ( 'NONE', #14870, #3786, #8680 ) ;
#26738=CIRCLE ( 'NONE', #20155, 2.000000000000000000 ) ;
#26739=CARTESIAN_POINT ( 'NONE',  ( -55.00000337463107059, 43.30127018922197379, 12.50000000000000000 ) ) ;
#26740=CARTESIAN_POINT ( 'NONE',  ( -75.00000337463097821, 8.660254037844374864, 12.50000000000000000 ) ) ;
#26741=EDGE_CURVE ( 'NONE', #19312, #2698, #12543, .T. ) ;
#26742=ORIENTED_EDGE ( 'NONE', *, *, #34852, .F. ) ;
#26747=DIRECTION ( 'NONE',  ( 0.000000000000000000, 0.000000000000000000, -1.000000000000000000 ) ) ;
#26748=LINE ( 'NONE', #7252, #16142 ) ;
#26750=DIRECTION ( 'NONE',  ( 0.000000000000000000, 0.000000000000000000, -1.000000000000000000 ) ) ;
#26752=CARTESIAN_POINT ( 'NONE',  ( -60.00000337463108480, -51.96152422706641971, 17.49999999999999645 ) ) ;
#26753=EDGE_CURVE ( 'NONE', #29492, #2026, #21834, .T. ) ;
#26756=AXIS2_PLACEMENT_3D ( 'NONE', #4691, #1680, #15366 ) ;
#26757=EDGE_CURVE ( 'NONE', #34308, #24231, #24365, .T. ) ;
#26758=EDGE_LOOP ( 'NONE', ( #992, #9399, #15166, #10356, #32014 ) ) ;
#26760=DIRECTION ( 'NONE',  ( 1.000000000000000000, 0.000000000000000000, 0.000000000000000000 ) ) ;
#26764=CIRCLE ( 'NONE', #10603, 2.000000000000000000 ) ;
#26766=DIRECTION ( 'NONE',  ( 1.000000000000000000, 0.000000000000000000, 0.000000000000000000 ) ) ;
#26767=DIRECTION ( 'NONE',  ( -0.5000000000000101030, -0.8660254037844329345, 0.000000000000000000 ) ) ;
#26768=EDGE_CURVE ( 'NONE', #19268, #28791, #35006, .T. ) ;
#26769=CARTESIAN_POINT ( 'NONE',  ( -5.000003374631307729, 77.94228634059957983, -9.999999999999998224 ) ) ;
#26771=SHAPE_REPRESENTATION ( 'ventilated rotor', ( #21385 ), #23118 ) ;
#26772=ORIENTED_EDGE ( 'NONE', *, *, #1387, .F. ) ;
#26773=LINE ( 'NONE', #32395, #23655 ) ;
#26774=EDGE_CURVE ( 'NONE', #545, #29294, #6249, .T. ) ;
#26776=ORIENTED_EDGE ( 'NONE', *, *, #28385, .F. ) ;
#26777=CYLINDRICAL_SURFACE ( 'NONE', #7744, 27.00000000000001066 ) ;
#26778=VERTEX_POINT ( 'NONE', #32416 ) ;
#26780=VECTOR ( 'NONE', #30634, 1000.000000000000000 ) ;
#26782=VERTEX_POINT ( 'NONE', #7119 ) ;
#26785=ORIENTED_EDGE ( 'NONE', *, *, #11619, .F. ) ;
#26788=DIRECTION ( 'NONE',  ( 0.000000000000000000, 0.000000000000000000, 1.000000000000000000 ) ) ;
#26789=VECTOR ( 'NONE', #21241, 1000.000000000000000 ) ;
#26790=ADVANCED_FACE ( 'NONE', ( #32595 ), #4122, .F. ) ;
#26791=CARTESIAN_POINT ( 'NONE',  ( -58.00000337463108480, -51.96152422706641971, -9.999999999999998224 ) ) ;
#26792=DIRECTION ( 'NONE',  ( 1.000000000000000000, 0.000000000000000000, 0.000000000000000000 ) ) ;
#26793=ORIENTED_EDGE ( 'NONE', *, *, #23024, .T. ) ;
#26795=AXIS2_PLACEMENT_3D ( 'NONE', #20548, #18118, #29544 ) ;
#26796=ORIENTED_EDGE ( 'NONE', *, *, #9758, .F. ) ;
#26799=ORIENTED_EDGE ( 'NONE', *, *, #306, .F. ) ;
#26800=CARTESIAN_POINT ( 'NONE',  ( -45.00000337463112743, -60.62177826491080168, 12.50000000000000000 ) ) ;
#26801=AXIS2_PLACEMENT_3D ( 'NONE', #30683, #21878, #16093 ) ;
#26803=DIRECTION ( 'NONE',  ( 0.000000000000000000, 0.000000000000000000, 1.000000000000000000 ) ) ;
#26805=EDGE_CURVE ( 'NONE', #10468, #23471, #20608, .T. ) ;
#26806=VECTOR ( 'NONE', #33525, 1000.000000000000000 ) ;
#26807=DIRECTION ( 'NONE',  ( -0.000000000000000000, -0.000000000000000000, 1.000000000000000000 ) ) ;
#26808=AXIS2_PLACEMENT_3D ( 'NONE', #15969, #26653, #9963 ) ;
#26809=CARTESIAN_POINT ( 'NONE',  ( 21.99999662536862033, -69.28203230275519786, 17.49999999999999645 ) ) ;
#26810=LINE ( 'NONE', #32805, #23767 ) ;
#26812=CARTESIAN_POINT ( 'NONE',  ( 58.88972745734179171, -34.00000000000007105, -49.22241343995298024 ) ) ;
#26813=AXIS2_PLACEMENT_3D ( 'NONE', #11476, #22921, #14650 ) ;
#26814=DIRECTION ( 'NONE',  ( 0.000000000000000000, 0.000000000000000000, 1.000000000000000000 ) ) ;
#26815=AXIS2_PLACEMENT_3D ( 'NONE', #1178, #9050, #21041 ) ;
#26816=FACE_OUTER_BOUND ( 'NONE', #186, .T. ) ;
#26817=EDGE_LOOP ( 'NONE', ( #9989, #24442, #24635, #23751 ) ) ;
#26818=DIRECTION ( 'NONE',  ( 1.000000000000000000, 0.000000000000000000, 0.000000000000000000 ) ) ;
#26820=EDGE_LOOP ( 'NONE', ( #3179, #13585, #4885, #11614 ) ) ;
#26821=ORIENTED_EDGE ( 'NONE', *, *, #14229, .T. ) ;
#26822=AXIS2_PLACEMENT_3D ( 'NONE', #35159, #15643, #27064 ) ;
#26823=LINE ( 'NONE', #9017, #30816 ) ;
#26824=EDGE_CURVE ( 'NONE', #3385, #32894, #14647, .T. ) ;
#26826=CARTESIAN_POINT ( 'NONE',  ( -72.00000337463102085, -34.64101615137762025, -9.999999999999998224 ) ) ;
#26827=CARTESIAN_POINT ( 'NONE',  ( 69.99999662536839651, -17.32050807568879947, -9.999999999999998224 ) ) ;
#26828=ORIENTED_EDGE ( 'NONE', *, *, #25213, .F. ) ;
#26829=CIRCLE ( 'NONE', #19635, 2.000000000000001776 ) ;
#26830=DIRECTION ( 'NONE',  ( 1.000000000000000000, 0.000000000000000000, 0.000000000000000000 ) ) ;
#26831=DIRECTION ( 'NONE',  ( -0.4999999999999980571, 0.8660254037844399289, 0.000000000000000000 ) ) ;
#26832=CIRCLE ( 'NONE', #10672, 2.000000000000000000 ) ;
#26833=VERTEX_POINT ( 'NONE', #18737 ) ;
#26834=AXIS2_PLACEMENT_3D ( 'NONE', #14267, #34704, #34321 ) ;
#26836=VERTEX_POINT ( 'NONE', #6731 ) ;
#26837=CARTESIAN_POINT ( 'NONE',  ( -85.00000337463092137, 25.98076211353317433, 12.50000000000000000 ) ) ;
#26838=CARTESIAN_POINT ( 'NONE',  ( -53.00000337463106348, 43.30127018922197379, -5.000000000000000000 ) ) ;
#26839=EDGE_CURVE ( 'NONE', #35776, #1755, #3284, .T. ) ;
#26840=AXIS2_PLACEMENT_3D ( 'NONE', #12965, #10728, #36049 ) ;
#26841=DIRECTION ( 'NONE',  ( 0.000000000000000000, 0.000000000000000000, 1.000000000000000000 ) ) ;
#26842=VERTEX_POINT ( 'NONE', #4303 ) ;
#26845=EDGE_CURVE ( 'NONE', #13964, #16940, #15842, .T. ) ;
#26846=CIRCLE ( 'NONE', #5318, 2.000000000000001776 ) ;
#26847=ORIENTED_EDGE ( 'NONE', *, *, #26757, .T. ) ;
#26848=CARTESIAN_POINT ( 'NONE',  ( -7.000003374631307729, 77.94228634059957983, -9.999999999999998224 ) ) ;
#26849=CARTESIAN_POINT ( 'NONE',  ( -68.00000337463102085, -34.64101615137762025, 12.50000000000000000 ) ) ;
#26850=EDGE_CURVE ( 'NONE', #7710, #8936, #2664, .T. ) ;
#26851=DIRECTION ( 'NONE',  ( -1.000000000000000000, 0.000000000000000000, 0.000000000000000000 ) ) ;
#26852=CARTESIAN_POINT ( 'NONE',  ( -5.000003374631307729, 77.94228634059957983, 12.50000000000000000 ) ) ;
#26853=AXIS2_PLACEMENT_3D ( 'NONE', #14205, #17013, #14397 ) ;
#26854=CARTESIAN_POINT ( 'NONE',  ( -48.00000337463112032, -51.96152422706641971, -9.999999999999998224 ) ) ;
#26855=EDGE_CURVE ( 'NONE', #10938, #33601, #7460, .T. ) ;
#26856=ORIENTED_EDGE ( 'NONE', *, *, #14187, .T. ) ;
#26858=CARTESIAN_POINT ( 'NONE',  ( -20.00000337463123756, -69.28203230275522628, -9.999999999999998224 ) ) ;
#26860=CARTESIAN_POINT ( 'NONE',  ( -63.00000337463106348, -60.62177826491083010, -5.000000000000000000 ) ) ;
#26862=CARTESIAN_POINT ( 'NONE',  ( 42.99999662536848888, -77.94228634059960825, -9.999999999999998224 ) ) ;
#26863=CIRCLE ( 'NONE', #10702, 2.000000000000001776 ) ;
#26864=FACE_BOUND ( 'NONE', #35296, .T. ) ;
#26866=ADVANCED_FACE ( 'NONE', ( #11708 ), #19808, .F. ) ;
#26867=AXIS2_PLACEMENT_3D ( 'NONE', #33111, #26942, #33309 ) ;
#26868=ORIENTED_EDGE ( 'NONE', *, *, #32065, .T. ) ;
#26871=EDGE_CURVE ( 'NONE', #7462, #34182, #5931, .T. ) ;
#26872=EDGE_CURVE ( 'NONE', #8683, #15938, #15240, .T. ) ;
#26873=DIRECTION ( 'NONE',  ( 0.000000000000000000, 0.000000000000000000, 1.000000000000000000 ) ) ;
#26877=ORIENTED_EDGE ( 'NONE', *, *, #897, .T. ) ;
#26879=CARTESIAN_POINT ( 'NONE',  ( -3.374631327851540519E-06, 86.60254037844397601, 17.49999999999999645 ) ) ;
#26880=ORIENTED_EDGE ( 'NONE', *, *, #6664, .F. ) ;
#26881=ORIENTED_EDGE ( 'NONE', *, *, #36239, .T. ) ;
#26882=CARTESIAN_POINT ( 'NONE',  ( 37.99999662536853151, -69.28203230275519786, -9.999999999999998224 ) ) ;
#26883=EDGE_LOOP ( 'NONE', ( #29629, #18672, #21085, #23520 ) ) ;
#26884=ORIENTED_EDGE ( 'NONE', *, *, #34804, .F. ) ;
#26885=DIRECTION ( 'NONE',  ( 0.000000000000000000, 0.000000000000000000, 1.000000000000000000 ) ) ;
#26886=DIRECTION ( 'NONE',  ( 0.000000000000000000, 0.000000000000000000, 1.000000000000000000 ) ) ;
#26887=EDGE_LOOP ( 'NONE', ( #3004, #14940 ) ) ;
#26888=VERTEX_POINT ( 'NONE', #8546 ) ;
#26889=DIRECTION ( 'NONE',  ( 0.000000000000000000, 0.000000000000000000, 1.000000000000000000 ) ) ;
#26892=CARTESIAN_POINT ( 'NONE',  ( -82.00000337463094979, 34.64101615137757051, 17.49999999999999645 ) ) ;
#26894=EDGE_LOOP ( 'NONE', ( #3636, #31642 ) ) ;
#26895=CARTESIAN_POINT ( 'NONE',  ( -70.00000337463102085, -51.96152422706641971, -9.999999999999998224 ) ) ;
#26896=CARTESIAN_POINT ( 'NONE',  ( -28.00000337463119493, -69.28203230275522628, -9.999999999999998224 ) ) ;
#26897=AXIS2_PLACEMENT_3D ( 'NONE', #2524, #36480, #19785 ) ;
#26898=VERTEX_POINT ( 'NONE', #34417 ) ;
#26902=DIRECTION ( 'NONE',  ( -0.8660254037844383745, 0.5000000000000005551, 0.000000000000000000 ) ) ;
#26904=DIRECTION ( 'NONE',  ( -1.000000000000000000, 0.000000000000000000, 0.000000000000000000 ) ) ;
#26906=LINE ( 'NONE', #9827, #10366 ) ;
#26907=ORIENTED_EDGE ( 'NONE', *, *, #4073, .F. ) ;
#26909=DIRECTION ( 'NONE',  ( 0.000000000000000000, 0.000000000000000000, 1.000000000000000000 ) ) ;
#26911=ORIENTED_EDGE ( 'NONE', *, *, #30205, .T. ) ;
#26912=VERTEX_POINT ( 'NONE', #2935 ) ;
#26913=AXIS2_PLACEMENT_3D ( 'NONE', #36397, #6954, #18768 ) ;
#26914=ORIENTED_EDGE ( 'NONE', *, *, #3706, .F. ) ;
#26916=ADVANCED_FACE ( 'NONE', ( #31398 ), #34248, .F. ) ;
#26919=FACE_OUTER_BOUND ( 'NONE', #5234, .T. ) ;
#26920=CARTESIAN_POINT ( 'NONE',  ( -30.00000337463118427, 69.28203230275516944, -9.999999999999998224 ) ) ;
#26921=CARTESIAN_POINT ( 'NONE',  ( 41.99999662536853151, 69.28203230275518365, 12.50000000000000000 ) ) ;
#26922=EDGE_LOOP ( 'NONE', ( #29404, #29219, #33420, #17650, #27437 ) ) ;
#26923=CARTESIAN_POINT ( 'NONE',  ( -80.00000337463094979, 17.32050807568878525, 17.49999999999999645 ) ) ;
#26924=ORIENTED_EDGE ( 'NONE', *, *, #34868, .T. ) ;
#26925=FACE_OUTER_BOUND ( 'NONE', #31185, .T. ) ;
#26926=AXIS2_PLACEMENT_3D ( 'NONE', #25057, #30483, #15679 ) ;
#26928=DIRECTION ( 'NONE',  ( 0.000000000000000000, 0.000000000000000000, 1.000000000000000000 ) ) ;
#26930=ORIENTED_EDGE ( 'NONE', *, *, #1561, .T. ) ;
#26933=ADVANCED_FACE ( 'NONE', ( #31232 ), #10975, .F. ) ;
#26934=EDGE_CURVE ( 'NONE', #22366, #14606, #12854, .T. ) ;
#26935=CARTESIAN_POINT ( 'NONE',  ( -33.00000337463116296, 60.62177826491077326, 17.49999999999999645 ) ) ;
#26936=CIRCLE ( 'NONE', #7786, 2.000000000000001776 ) ;
#26937=CARTESIAN_POINT ( 'NONE',  ( -18.00000337463123756, -86.60254037844400443, -9.999999999999998224 ) ) ;
#26938=DIRECTION ( 'NONE',  ( 0.000000000000000000, 0.000000000000000000, 1.000000000000000000 ) ) ;
#26939=ORIENTED_EDGE ( 'NONE', *, *, #15153, .F. ) ;
#26940=DIRECTION ( 'NONE',  ( 0.000000000000000000, 0.000000000000000000, 1.000000000000000000 ) ) ;
#26941=CIRCLE ( 'NONE', #12557, 3.000000000000002665 ) ;
#26942=DIRECTION ( 'NONE',  ( -0.000000000000000000, -0.000000000000000000, 1.000000000000000000 ) ) ;
#26943=CYLINDRICAL_SURFACE ( 'NONE', #9981, 2.000000000000001776 ) ;
#26946=ORIENTED_EDGE ( 'NONE', *, *, #28654, .T. ) ;
#26947=EDGE_LOOP ( 'NONE', ( #6787, #33344 ) ) ;
#26948=DIRECTION ( 'NONE',  ( -0.000000000000000000, -0.000000000000000000, 1.000000000000000000 ) ) ;
#26949=DIRECTION ( 'NONE',  ( 1.000000000000000000, 0.000000000000000000, 0.000000000000000000 ) ) ;
#26950=VECTOR ( 'NONE', #1597, 1000.000000000000000 ) ;
#26951=CARTESIAN_POINT ( 'NONE',  ( 59.99999662536842493, 51.96152422706639129, -9.999999999999998224 ) ) ;
#26952=AXIS2_PLACEMENT_3D ( 'NONE', #20305, #224, #28744 ) ;
#26954=DIRECTION ( 'NONE',  ( 1.000000000000000000, 0.000000000000000000, 0.000000000000000000 ) ) ;
#26956=CIRCLE ( 'NONE', #14995, 2.000000000000000000 ) ;
#26957=CARTESIAN_POINT ( 'NONE',  ( 91.99999662536828282, 0.000000000000000000, -5.000000000000000000 ) ) ;
#26958=ORIENTED_EDGE ( 'NONE', *, *, #16234, .F. ) ;
#26959=ORIENTED_EDGE ( 'NONE', *, *, #35404, .F. ) ;
#26961=AXIS2_PLACEMENT_3D ( 'NONE', #29003, #26572, #328 ) ;
#26962=DIRECTION ( 'NONE',  ( 0.000000000000000000, 0.000000000000000000, -1.000000000000000000 ) ) ;
#26963=ORIENTED_EDGE ( 'NONE', *, *, #6688, .T. ) ;
#26964=CARTESIAN_POINT ( 'NONE',  ( -50.00000337463109190, 69.28203230275518365, -9.999999999999998224 ) ) ;
#26966=DIRECTION ( 'NONE',  ( 1.000000000000000000, 0.000000000000000000, 0.000000000000000000 ) ) ;
#26967=CARTESIAN_POINT ( 'NONE',  ( 71.99999662536839651, -3.469446951953614189E-15, 12.50000000000000000 ) ) ;
#26969=ORIENTED_EDGE ( 'NONE', *, *, #27274, .F. ) ;
#26970=EDGE_CURVE ( 'NONE', #14832, #25364, #20056, .T. ) ;
#26971=VECTOR ( 'NONE', #25575, 1000.000000000000000 ) ;
#26972=DIRECTION ( 'NONE',  ( 0.000000000000000000, 0.000000000000000000, 1.000000000000000000 ) ) ;
#26973=VERTEX_POINT ( 'NONE', #25250 ) ;
#26975=FACE_OUTER_BOUND ( 'NONE', #23421, .T. ) ;
#26976=CARTESIAN_POINT ( 'NONE',  ( -3.000003374631269981, -77.94228634059960825, -5.000000000000000000 ) ) ;
#26978=ORIENTED_EDGE ( 'NONE', *, *, #34311, .F. ) ;
#26979=EDGE_CURVE ( 'NONE', #21341, #11639, #25809, .T. ) ;
#26980=ORIENTED_EDGE ( 'NONE', *, *, #36892, .F. ) ;
#26981=ORIENTED_EDGE ( 'NONE', *, *, #18812, .F. ) ;
#26983=ORIENTED_EDGE ( 'NONE', *, *, #9391, .F. ) ;
#26985=DIRECTION ( 'NONE',  ( 1.000000000000000000, 0.000000000000000000, 0.000000000000000000 ) ) ;
#26986=ORIENTED_EDGE ( 'NONE', *, *, #11000, .F. ) ;
#26987=FACE_OUTER_BOUND ( 'NONE', #32781, .T. ) ;
#26989=DIRECTION ( 'NONE',  ( -0.4999999999999980571, 0.8660254037844399289, 0.000000000000000000 ) ) ;
#26994=DIRECTION ( 'NONE',  ( 1.000000000000000000, 0.000000000000000000, 0.000000000000000000 ) ) ;
#26996=CARTESIAN_POINT ( 'NONE',  ( 81.99999662536833966, 34.64101615137759183, 12.50000000000000000 ) ) ;
#26997=DIRECTION ( 'NONE',  ( 1.000000000000000000, 0.000000000000000000, 0.000000000000000000 ) ) ;
#26998=ORIENTED_EDGE ( 'NONE', *, *, #7290, .T. ) ;
#26999=ORIENTED_EDGE ( 'NONE', *, *, #26453, .T. ) ;
#27002=CARTESIAN_POINT ( 'NONE',  ( -85.00000337463092137, 25.98076211353317433, 17.49999999999999645 ) ) ;
#27003=CIRCLE ( 'NONE', #3646, 27.00000000000001066 ) ;
#27005=DIRECTION ( 'NONE',  ( 0.000000000000000000, 0.000000000000000000, 1.000000000000000000 ) ) ;
#27006=EDGE_LOOP ( 'NONE', ( #9757, #6170 ) ) ;
#27007=ADVANCED_FACE ( 'NONE', ( #33863 ), #31050, .T. ) ;
#27008=DIRECTION ( 'NONE',  ( 1.000000000000000000, 0.000000000000000000, 0.000000000000000000 ) ) ;
#27009=DIRECTION ( 'NONE',  ( 0.000000000000000000, 0.000000000000000000, 1.000000000000000000 ) ) ;
#27010=ORIENTED_EDGE ( 'NONE', *, *, #26187, .F. ) ;
#27011=EDGE_CURVE ( 'NONE', #22792, #14280, #28403, .T. ) ;
#27012=DIRECTION ( 'NONE',  ( 0.000000000000000000, 0.000000000000000000, -1.000000000000000000 ) ) ;
#27015=CARTESIAN_POINT ( 'NONE',  ( -56.67878100130369035, 27.78182860042797131, 12.49999999999999822 ) ) ;
#27016=DIRECTION ( 'NONE',  ( -1.000000000000000000, 0.000000000000000000, 0.000000000000000000 ) ) ;
#27018=VERTEX_POINT ( 'NONE', #11359 ) ;
#27019=VECTOR ( 'NONE', #34130, 1000.000000000000000 ) ;
#27021=ORIENTED_EDGE ( 'NONE', *, *, #18408, .T. ) ;
#27023=FACE_OUTER_BOUND ( 'NONE', #10434, .T. ) ;
#27024=DIRECTION ( 'NONE',  ( 1.000000000000000000, 0.000000000000000000, 0.000000000000000000 ) ) ;
#27025=DIRECTION ( 'NONE',  ( 0.000000000000000000, 0.000000000000000000, 1.000000000000000000 ) ) ;
#27026=CARTESIAN_POINT ( 'NONE',  ( 72.99999662536836809, 43.30127018922198801, -9.999999999999998224 ) ) ;
#27027=ORIENTED_EDGE ( 'NONE', *, *, #24056, .T. ) ;
#27028=CARTESIAN_POINT ( 'NONE',  ( -45.00000337463111322, -77.94228634059960825, -9.999999999999998224 ) ) ;
#27031=ORIENTED_EDGE ( 'NONE', *, *, #30960, .F. ) ;
#27032=DIRECTION ( 'NONE',  ( 0.000000000000000000, 0.000000000000000000, 1.000000000000000000 ) ) ;
#27033=DIRECTION ( 'NONE',  ( 1.000000000000000000, 0.000000000000000000, -0.000000000000000000 ) ) ;
#27034=ORIENTED_EDGE ( 'NONE', *, *, #26753, .F. ) ;
#27035=ORIENTED_EDGE ( 'NONE', *, *, #20218, .F. ) ;
#27036=EDGE_CURVE ( 'NONE', #245, #20452, #26052, .T. ) ;
#27040=EDGE_CURVE ( 'NONE', #19680, #13964, #29508, .T. ) ;
#27041=CYLINDRICAL_SURFACE ( 'NONE', #13015, 2.000000000000001776 ) ;
#27042=ORIENTED_EDGE ( 'NONE', *, *, #30807, .T. ) ;
#27043=AXIS2_PLACEMENT_3D ( 'NONE', #17454, #31323, #14078 ) ;
#27044=ORIENTED_EDGE ( 'NONE', *, *, #35489, .T. ) ;
#27045=ORIENTED_EDGE ( 'NONE', *, *, #14136, .T. ) ;
#27046=EDGE_CURVE ( 'NONE', #21830, #19005, #3891, .T. ) ;
#27047=CARTESIAN_POINT ( 'NONE',  ( -35.00000337463117717, -77.94228634059963667, -5.000000000000000000 ) ) ;
#27049=VERTEX_POINT ( 'NONE', #23718 ) ;
#27051=CARTESIAN_POINT ( 'NONE',  ( 34.99999662536853862, 77.94228634059959404, -5.000000000000000000 ) ) ;
#27052=VERTEX_POINT ( 'NONE', #32509 ) ;
#27053=EDGE_CURVE ( 'NONE', #22919, #4653, #22443, .T. ) ;
#27054=ORIENTED_EDGE ( 'NONE', *, *, #26979, .T. ) ;
#27055=CARTESIAN_POINT ( 'NONE',  ( -80.00000337463096400, -34.64101615137762025, -5.000000000000000000 ) ) ;
#27056=CARTESIAN_POINT ( 'NONE',  ( 89.99999662536828282, 0.000000000000000000, -9.999999999999998224 ) ) ;
#27058=ORIENTED_EDGE ( 'NONE', *, *, #26117, .F. ) ;
#27059=FACE_OUTER_BOUND ( 'NONE', #2435, .T. ) ;
#27060=LINE ( 'NONE', #21247, #6355 ) ;
#27063=EDGE_CURVE ( 'NONE', #27148, #16244, #29630, .T. ) ;
#27064=DIRECTION ( 'NONE',  ( 1.000000000000000000, 0.000000000000000000, 0.000000000000000000 ) ) ;
#27065=EDGE_CURVE ( 'NONE', #10178, #7273, #8080, .T. ) ;
#27066=VERTEX_POINT ( 'NONE', #12638 ) ;
#27067=DIRECTION ( 'NONE',  ( 0.000000000000000000, 0.000000000000000000, 1.000000000000000000 ) ) ;
#27068=AXIS2_PLACEMENT_3D ( 'NONE', #5503, #31724, #14658 ) ;
#27070=VERTEX_POINT ( 'NONE', #3277 ) ;
#27071=CARTESIAN_POINT ( 'NONE',  ( -4.279621169095561228, 62.97617850287782915, -4.999999999999997335 ) ) ;
#27072=EDGE_CURVE ( 'NONE', #18793, #18742, #8688, .T. ) ;
#27073=CYLINDRICAL_SURFACE ( 'NONE', #10622, 2.000000000000001776 ) ;
#27074=FACE_OUTER_BOUND ( 'NONE', #26716, .T. ) ;
#27075=DIRECTION ( 'NONE',  ( 0.000000000000000000, 0.000000000000000000, -1.000000000000000000 ) ) ;
#27077=CARTESIAN_POINT ( 'NONE',  ( -47.00000337463111322, 77.94228634059959404, -5.000000000000000000 ) ) ;
#27079=ORIENTED_EDGE ( 'NONE', *, *, #29524, .T. ) ;
#27080=DIRECTION ( 'NONE',  ( 0.000000000000000000, 0.000000000000000000, -1.000000000000000000 ) ) ;
#27081=DIRECTION ( 'NONE',  ( -0.000000000000000000, -0.000000000000000000, -1.000000000000000000 ) ) ;
#27082=DIRECTION ( 'NONE',  ( 1.000000000000000000, 0.000000000000000000, 0.000000000000000000 ) ) ;
#27083=ORIENTED_EDGE ( 'NONE', *, *, #20715, .F. ) ;
#27085=EDGE_LOOP ( 'NONE', ( #32348, #3897 ) ) ;
#27086=ORIENTED_EDGE ( 'NONE', *, *, #35281, .T. ) ;
#27088=CARTESIAN_POINT ( 'NONE',  ( 86.45172111230354517, -31.46585318596159553, -4.999999999999997335 ) ) ;
#27090=ORIENTED_EDGE ( 'NONE', *, *, #29576, .F. ) ;
#27091=CARTESIAN_POINT ( 'NONE',  ( 51.99999662536847467, -69.28203230275519786, -9.999999999999998224 ) ) ;
#27092=VECTOR ( 'NONE', #15778, 1000.000000000000000 ) ;
#27093=CYLINDRICAL_SURFACE ( 'NONE', #21920, 2.000000000000001776 ) ;
#27097=CARTESIAN_POINT ( 'NONE',  ( 62.99999662536841072, -25.98076211353320275, -5.000000000000000000 ) ) ;
#27098=FACE_OUTER_BOUND ( 'NONE', #23928, .T. ) ;
#27099=DIRECTION ( 'NONE',  ( 0.000000000000000000, 0.000000000000000000, 1.000000000000000000 ) ) ;
#27100=FACE_OUTER_BOUND ( 'NONE', #31568, .T. ) ;
#27101=EDGE_LOOP ( 'NONE', ( #35324, #29308, #13338, #17281 ) ) ;
#27102=CYLINDRICAL_SURFACE ( 'NONE', #27870, 2.000000000000001776 ) ;
#27104=DIRECTION ( 'NONE',  ( 0.000000000000000000, 0.000000000000000000, 1.000000000000000000 ) ) ;
#27106=AXIS2_PLACEMENT_3D ( 'NONE', #18940, #27174, #24187 ) ;
#27107=DIRECTION ( 'NONE',  ( 0.000000000000000000, 0.000000000000000000, 1.000000000000000000 ) ) ;
#27108=CARTESIAN_POINT ( 'NONE',  ( -78.38502691089041718, -33.46124879229190441, 12.50000000000000000 ) ) ;
#27109=EDGE_CURVE ( 'NONE', #24647, #8725, #298, .T. ) ;
#27110=ORIENTED_EDGE ( 'NONE', *, *, #26593, .F. ) ;
#27111=CARTESIAN_POINT ( 'NONE',  ( 9.999996625368625658, 86.60254037844397601, -9.999999999999998224 ) ) ;
#27113=CARTESIAN_POINT ( 'NONE',  ( -75.00000337463099243, -25.98076211353322051, 17.49999999999999645 ) ) ;
#27116=ORIENTED_EDGE ( 'NONE', *, *, #35459, .T. ) ;
#27117=AXIS2_PLACEMENT_3D ( 'NONE', #10583, #30637, #18842 ) ;
#27118=LINE ( 'NONE', #27305, #27350 ) ;
#27119=LINE ( 'NONE', #4269, #34496 ) ;
#27120=DIRECTION ( 'NONE',  ( 0.000000000000000000, 0.000000000000000000, -1.000000000000000000 ) ) ;
#27121=ORIENTED_EDGE ( 'NONE', *, *, #729, .T. ) ;
#27122=DIRECTION ( 'NONE',  ( 1.000000000000000000, 0.000000000000000000, 0.000000000000000000 ) ) ;
#27124=CARTESIAN_POINT ( 'NONE',  ( 7.999996625368618552, 69.28203230275516944, -5.000000000000000000 ) ) ;
#27125=AXIS2_PLACEMENT_3D ( 'NONE', #5151, #16786, #2348 ) ;
#27127=EDGE_CURVE ( 'NONE', #36648, #31059, #12067, .T. ) ;
#27128=ORIENTED_EDGE ( 'NONE', *, *, #35788, .F. ) ;
#27129=EDGE_LOOP ( 'NONE', ( #28724, #30728 ) ) ;
#27130=AXIS2_PLACEMENT_3D ( 'NONE', #12515, #35976, #3718 ) ;
#27134=DIRECTION ( 'NONE',  ( 1.000000000000000000, 0.000000000000000000, 0.000000000000000000 ) ) ;
#27135=ORIENTED_EDGE ( 'NONE', *, *, #3837, .T. ) ;
#27136=CARTESIAN_POINT ( 'NONE',  ( 0.000000000000000000, 0.000000000000000000, 12.49999999999999822 ) ) ;
#27137=EDGE_CURVE ( 'NONE', #35523, #30112, #23650, .T. ) ;
#27138=FACE_BOUND ( 'NONE', #13575, .T. ) ;
#27140=ORIENTED_EDGE ( 'NONE', *, *, #19948, .F. ) ;
#27141=CARTESIAN_POINT ( 'NONE',  ( -3.374631289687624047E-06, -69.28203230275519786, 12.50000000000000000 ) ) ;
#27142=VERTEX_POINT ( 'NONE', #3661 ) ;
#27144=DIRECTION ( 'NONE',  ( 1.000000000000000000, 0.000000000000000000, 0.000000000000000000 ) ) ;
#27145=FACE_OUTER_BOUND ( 'NONE', #11209, .T. ) ;
#27146=LINE ( 'NONE', #24353, #19717 ) ;
#27147=EDGE_CURVE ( 'NONE', #20281, #35451, #33231, .T. ) ;
#27148=VERTEX_POINT ( 'NONE', #830 ) ;
#27149=DIRECTION ( 'NONE',  ( 0.000000000000000000, 0.000000000000000000, -1.000000000000000000 ) ) ;
#27150=CIRCLE ( 'NONE', #12168, 2.000000000000000000 ) ;
#27151=CARTESIAN_POINT ( 'NONE',  ( 67.99999662536838230, 17.32050807568879236, -9.999999999999998224 ) ) ;
#27152=VERTEX_POINT ( 'NONE', #1025 ) ;
#27153=ORIENTED_EDGE ( 'NONE', *, *, #10819, .T. ) ;
#27154=ORIENTED_EDGE ( 'NONE', *, *, #14862, .T. ) ;
#27156=DIRECTION ( 'NONE',  ( 0.000000000000000000, 0.000000000000000000, 1.000000000000000000 ) ) ;
#27157=VERTEX_POINT ( 'NONE', #30629 ) ;
#27158=DIRECTION ( 'NONE',  ( -1.000000000000000000, 0.000000000000000000, 0.000000000000000000 ) ) ;
#27159=DIRECTION ( 'NONE',  ( 1.000000000000000000, 0.000000000000000000, 0.000000000000000000 ) ) ;
#27160=ORIENTED_EDGE ( 'NONE', *, *, #15790, .T. ) ;
#27161=DIRECTION ( 'NONE',  ( 0.000000000000000000, 0.000000000000000000, 1.000000000000000000 ) ) ;
#27163=DIRECTION ( 'NONE',  ( 1.000000000000000000, 0.000000000000000000, 0.000000000000000000 ) ) ;
#27165=ADVANCED_FACE ( 'NONE', ( #21462 ), #21816, .F. ) ;
#27166=DIRECTION ( 'NONE',  ( -0.8660254037844379305, 0.5000000000000011102, 0.000000000000000000 ) ) ;
#27167=CYLINDRICAL_SURFACE ( 'NONE', #22670, 2.000000000000001776 ) ;
#27169=EDGE_CURVE ( 'NONE', #36755, #31731, #21266, .T. ) ;
#27170=CARTESIAN_POINT ( 'NONE',  ( 0.000000000000000000, 0.000000000000000000, -5.000000000000000000 ) ) ;
#27171=ORIENTED_EDGE ( 'NONE', *, *, #14432, .T. ) ;
#27172=VERTEX_POINT ( 'NONE', #16383 ) ;
#27174=DIRECTION ( 'NONE',  ( 0.000000000000000000, 0.000000000000000000, 1.000000000000000000 ) ) ;
#27175=CARTESIAN_POINT ( 'NONE',  ( -50.00000337463109190, 51.96152422706637708, 12.50000000000000000 ) ) ;
#27176=DIRECTION ( 'NONE',  ( 0.000000000000000000, 0.000000000000000000, 1.000000000000000000 ) ) ;
#27177=ADVANCED_FACE ( 'NONE', ( #10021 ), #19026, .F. ) ;
#27179=CARTESIAN_POINT ( 'NONE',  ( -93.55673653615987462, -16.49657687835775377, 12.49999999999999822 ) ) ;
#27183=DIRECTION ( 'NONE',  ( 0.000000000000000000, 0.000000000000000000, 1.000000000000000000 ) ) ;
#27185=DIRECTION ( 'NONE',  ( 1.000000000000000000, 0.000000000000000000, 0.000000000000000000 ) ) ;
#27186=AXIS2_PLACEMENT_3D ( 'NONE', #23468, #6208, #11831 ) ;
#27187=CARTESIAN_POINT ( 'NONE',  ( -20.00000337463123756, -86.60254037844400443, 12.50000000000000000 ) ) ;
#27188=CIRCLE ( 'NONE', #5039, 2.000000000000001776 ) ;
#27189=CARTESIAN_POINT ( 'NONE',  ( 62.97617850287784336, 4.279621169095339184, 12.49999999999999822 ) ) ;
#27191=ORIENTED_EDGE ( 'NONE', *, *, #21355, .F. ) ;
#27193=EDGE_CURVE ( 'NONE', #719, #29785, #16027, .T. ) ;
#27194=VERTEX_POINT ( 'NONE', #7774 ) ;
#27196=FACE_BOUND ( 'NONE', #5376, .T. ) ;
#27198=CARTESIAN_POINT ( 'NONE',  ( -2.374207310413330682E-13, -68.00000000000000000, -49.86348611802629449 ) ) ;
#27199=CARTESIAN_POINT ( 'NONE',  ( -52.00000337463109190, 51.96152422706637708, 12.50000000000000000 ) ) ;
#27200=CARTESIAN_POINT ( 'NONE',  ( 26.99999662536859546, -77.94228634059960825, -9.999999999999998224 ) ) ;
#27201=ORIENTED_EDGE ( 'NONE', *, *, #24493, .F. ) ;
#27202=DIRECTION ( 'NONE',  ( 1.000000000000000000, 0.000000000000000000, 0.000000000000000000 ) ) ;
#27203=EDGE_CURVE ( 'NONE', #34980, #14875, #5697, .T. ) ;
#27204=AXIS2_PLACEMENT_3D ( 'NONE', #28709, #5643, #17081 ) ;
#27205=LINE ( 'NONE', #13163, #32931 ) ;
#27206=EDGE_CURVE ( 'NONE', #35276, #34186, #30841, .T. ) ;
#27208=ORIENTED_EDGE ( 'NONE', *, *, #15512, .F. ) ;
#27209=DIRECTION ( 'NONE',  ( 0.000000000000000000, 0.000000000000000000, 1.000000000000000000 ) ) ;
#27211=AXIS2_PLACEMENT_3D ( 'NONE', #32974, #7465, #16457 ) ;
#27212=ORIENTED_EDGE ( 'NONE', *, *, #20527, .T. ) ;
#27213=EDGE_CURVE ( 'NONE', #15428, #25705, #31432, .T. ) ;
#27215=EDGE_LOOP ( 'NONE', ( #27925, #21932 ) ) ;
#27216=AXIS2_PLACEMENT_3D ( 'NONE', #14155, #3268, #28392 ) ;
#27217=CYLINDRICAL_SURFACE ( 'NONE', #24716, 2.000000000000001776 ) ;
#27219=DIRECTION ( 'NONE',  ( 0.000000000000000000, 0.000000000000000000, 1.000000000000000000 ) ) ;
#27220=ADVANCED_FACE ( 'NONE', ( #29896 ), #18654, .F. ) ;
#27221=VERTEX_POINT ( 'NONE', #15824 ) ;
#27223=ORIENTED_EDGE ( 'NONE', *, *, #9869, .T. ) ;
#27224=DIRECTION ( 'NONE',  ( 1.000000000000000000, 0.000000000000000000, 0.000000000000000000 ) ) ;
#27225=EDGE_CURVE ( 'NONE', #2344, #10755, #4495, .T. ) ;
#27227=ORIENTED_EDGE ( 'NONE', *, *, #29247, .T. ) ;
#27229=DIRECTION ( 'NONE',  ( 1.000000000000000000, 0.000000000000000000, 0.000000000000000000 ) ) ;
#27230=ORIENTED_EDGE ( 'NONE', *, *, #16666, .T. ) ;
#27231=ORIENTED_EDGE ( 'NONE', *, *, #2301, .T. ) ;
#27232=DIRECTION ( 'NONE',  ( 1.000000000000000000, 0.000000000000000000, 0.000000000000000000 ) ) ;
#27233=CARTESIAN_POINT ( 'NONE',  ( -77.00000337463097821, 43.30127018922197379, 17.49999999999999645 ) ) ;
#27234=ORIENTED_EDGE ( 'NONE', *, *, #20870, .T. ) ;
#27235=EDGE_LOOP ( 'NONE', ( #14999, #28323, #19517, #32656 ) ) ;
#27236=FACE_OUTER_BOUND ( 'NONE', #9438, .T. ) ;
#27237=CARTESIAN_POINT ( 'NONE',  ( 56.67878100130369035, -27.78182860042797131, 12.49999999999999822 ) ) ;
#27240=AXIS2_PLACEMENT_3D ( 'NONE', #9073, #17894, #11691 ) ;
#27241=CARTESIAN_POINT ( 'NONE',  ( -85.00000337463092137, 25.98076211353317433, 12.50000000000000000 ) ) ;
#27242=EDGE_CURVE ( 'NONE', #11718, #5095, #27632, .T. ) ;
#27243=ORIENTED_EDGE ( 'NONE', *, *, #11667, .T. ) ;
#27244=FACE_OUTER_BOUND ( 'NONE', #18772, .T. ) ;
#27245=ORIENTED_EDGE ( 'NONE', *, *, #14044, .T. ) ;
#27246=DIRECTION ( 'NONE',  ( 1.000000000000000000, 0.000000000000000000, 0.000000000000000000 ) ) ;
#27249=DIRECTION ( 'NONE',  ( 0.000000000000000000, 0.000000000000000000, 1.000000000000000000 ) ) ;
#27250=CARTESIAN_POINT ( 'NONE',  ( -55.00000337463110611, -43.30127018922202353, -9.999999999999998224 ) ) ;
#27252=FACE_OUTER_BOUND ( 'NONE', #35181, .T. ) ;
#27253=CIRCLE ( 'NONE', #32018, 2.000000000000001776 ) ;
#27254=EDGE_CURVE ( 'NONE', #24009, #13023, #17675, .T. ) ;
#27256=ORIENTED_EDGE ( 'NONE', *, *, #16020, .T. ) ;
#27257=CYLINDRICAL_SURFACE ( 'NONE', #1625, 2.000000000000001776 ) ;
#27258=CIRCLE ( 'NONE', #21293, 2.000000000000000000 ) ;
#27259=EDGE_CURVE ( 'NONE', #20619, #21307, #21885, .T. ) ;
#27260=DIRECTION ( 'NONE',  ( -1.000000000000000000, 0.000000000000000000, 0.000000000000000000 ) ) ;
#27261=LINE ( 'NONE', #10224, #26504 ) ;
#27262=CIRCLE ( 'NONE', #28461, 33.00000000000001421 ) ;
#27263=CIRCLE ( 'NONE', #16483, 2.000000000000000000 ) ;
#27265=VECTOR ( 'NONE', #8200, 1000.000000000000000 ) ;
#27266=ORIENTED_EDGE ( 'NONE', *, *, #20040, .F. ) ;
#27267=VERTEX_POINT ( 'NONE', #21646 ) ;
#27268=DIRECTION ( 'NONE',  ( 0.000000000000000000, 0.000000000000000000, 1.000000000000000000 ) ) ;
#27269=CARTESIAN_POINT ( 'NONE',  ( -75.00000337463097821, -8.660254037844422825, -9.999999999999998224 ) ) ;
#27271=AXIS2_PLACEMENT_3D ( 'NONE', #21674, #21113, #36114 ) ;
#27272=AXIS2_PLACEMENT_3D ( 'NONE', #21689, #33689, #15882 ) ;
#27274=EDGE_CURVE ( 'NONE', #35191, #15953, #27454, .T. ) ;
#27275=CARTESIAN_POINT ( 'NONE',  ( -63.00000337463102085, 60.62177826491077326, 12.50000000000000000 ) ) ;
#27276=ORIENTED_EDGE ( 'NONE', *, *, #25213, .T. ) ;
#27277=DIRECTION ( 'NONE',  ( 0.000000000000000000, 0.000000000000000000, -1.000000000000000000 ) ) ;
#27278=EDGE_LOOP ( 'NONE', ( #9055, #26281, #7114 ) ) ;
#27279=CYLINDRICAL_SURFACE ( 'NONE', #2767, 2.000000000000000000 ) ;
#27280=DIRECTION ( 'NONE',  ( 1.000000000000000000, 0.000000000000000000, 0.000000000000000000 ) ) ;
#27282=CIRCLE ( 'NONE', #27900, 3.000000000000002665 ) ;
#27283=PLANE ( 'NONE',  #7424 ) ;
#27285=ORIENTED_EDGE ( 'NONE', *, *, #36428, .T. ) ;
#27286=CYLINDRICAL_SURFACE ( 'NONE', #912, 3.000000000000002665 ) ;
#27287=AXIS2_PLACEMENT_3D ( 'NONE', #24136, #21130, #7078 ) ;
#27289=CIRCLE ( 'NONE', #25506, 2.000000000000001776 ) ;
#27290=LINE ( 'NONE', #16065, #30238 ) ;
#27291=DIRECTION ( 'NONE',  ( 0.000000000000000000, 0.000000000000000000, 1.000000000000000000 ) ) ;
#27293=DIRECTION ( 'NONE',  ( 0.000000000000000000, 0.000000000000000000, 1.000000000000000000 ) ) ;
#27294=CARTESIAN_POINT ( 'NONE',  ( 19.99999662536858835, 69.28203230275516944, -9.999999999999998224 ) ) ;
#27295=EDGE_LOOP ( 'NONE', ( #12834, #23568, #1111, #13706 ) ) ;
#27296=ADVANCED_FACE ( 'NONE', ( #16770 ), #59, .F. ) ;
#27297=DIRECTION ( 'NONE',  ( 0.000000000000000000, 0.000000000000000000, 1.000000000000000000 ) ) ;
#27298=CIRCLE ( 'NONE', #1549, 2.000000000000001776 ) ;
#27299=DIRECTION ( 'NONE',  ( 0.000000000000000000, 0.000000000000000000, 1.000000000000000000 ) ) ;
#27300=CARTESIAN_POINT ( 'NONE',  ( 54.99999662536844625, 60.62177826491077326, -5.000000000000000000 ) ) ;
#27302=EDGE_LOOP ( 'NONE', ( #9015, #16582, #23470, #5487 ) ) ;
#27303=ORIENTED_EDGE ( 'NONE', *, *, #2455, .T. ) ;
#27304=ADVANCED_FACE ( 'NONE', ( #2680 ), #36639, .F. ) ;
#27305=CARTESIAN_POINT ( 'NONE',  ( 52.99999662536844625, 60.62177826491077326, -9.999999999999998224 ) ) ;
#27306=CARTESIAN_POINT ( 'NONE',  ( 82.99999662536831124, -25.98076211353319565, 17.49999999999999645 ) ) ;
#27308=LINE ( 'NONE', #24522, #35072 ) ;
#27309=ORIENTED_EDGE ( 'NONE', *, *, #21506, .T. ) ;
#27311=DIRECTION ( 'NONE',  ( 0.000000000000000000, 0.000000000000000000, -1.000000000000000000 ) ) ;
#27312=DIRECTION ( 'NONE',  ( -1.000000000000000000, -8.994862468027883963E-15, 0.000000000000000000 ) ) ;
#27313=CARTESIAN_POINT ( 'NONE',  ( 73.47608876694671665, 59.13646009116074964, 12.49999999999999822 ) ) ;
#27314=VECTOR ( 'NONE', #14673, 1000.000000000000000 ) ;
#27315=AXIS2_PLACEMENT_3D ( 'NONE', #22002, #13360, #27622 ) ;
#27316=CYLINDRICAL_SURFACE ( 'NONE', #3472, 2.000000000000001776 ) ;
#27317=EDGE_CURVE ( 'NONE', #20745, #7037, #1508, .T. ) ;
#27319=EDGE_LOOP ( 'NONE', ( #15281, #707 ) ) ;
#27320=VECTOR ( 'NONE', #34572, 1000.000000000000000 ) ;
#27322=ORIENTED_EDGE ( 'NONE', *, *, #20563, .T. ) ;
#27323=DIRECTION ( 'NONE',  ( 1.000000000000000000, 0.000000000000000000, 0.000000000000000000 ) ) ;
#27324=AXIS2_PLACEMENT_3D ( 'NONE', #5582, #6134, #20550 ) ;
#27325=ADVANCED_FACE ( 'NONE', ( #25379 ), #2507, .T. ) ;
#27326=DIRECTION ( 'NONE',  ( 0.000000000000000000, 0.000000000000000000, 1.000000000000000000 ) ) ;
#27328=EDGE_CURVE ( 'NONE', #7638, #23807, #16508, .T. ) ;
#27330=EDGE_LOOP ( 'NONE', ( #28330, #35818, #26847, #11889 ) ) ;
#27331=DIRECTION ( 'NONE',  ( 1.000000000000000000, 0.000000000000000000, 0.000000000000000000 ) ) ;
#27333=DIRECTION ( 'NONE',  ( 0.000000000000000000, 0.000000000000000000, 1.000000000000000000 ) ) ;
#27334=VERTEX_POINT ( 'NONE', #34369 ) ;
#27335=ORIENTED_EDGE ( 'NONE', *, *, #16844, .T. ) ;
#27337=ORIENTED_EDGE ( 'NONE', *, *, #17072, .F. ) ;
#27338=CIRCLE ( 'NONE', #30920, 2.000000000000001776 ) ;
#27339=DIRECTION ( 'NONE',  ( 0.000000000000000000, 0.000000000000000000, 1.000000000000000000 ) ) ;
#27340=CIRCLE ( 'NONE', #32749, 2.000000000000001776 ) ;
#27341=DIRECTION ( 'NONE',  ( 0.000000000000000000, 0.000000000000000000, 1.000000000000000000 ) ) ;
#27342=CARTESIAN_POINT ( 'NONE',  ( 57.99999662536842493, 51.96152422706639129, 12.50000000000000000 ) ) ;
#27344=FACE_OUTER_BOUND ( 'NONE', #9367, .T. ) ;
#27346=LINE ( 'NONE', #27151, #29800 ) ;
#27347=CYLINDRICAL_SURFACE ( 'NONE', #8916, 27.00000000000001066 ) ;
#27348=VECTOR ( 'NONE', #3414, 1000.000000000000000 ) ;
#27349=ORIENTED_EDGE ( 'NONE', *, *, #20843, .F. ) ;
#27350=VECTOR ( 'NONE', #1433, 1000.000000000000000 ) ;
#27351=EDGE_CURVE ( 'NONE', #18465, #30617, #6922, .T. ) ;
#27352=CIRCLE ( 'NONE', #18362, 2.000000000000001776 ) ;
#27355=ORIENTED_EDGE ( 'NONE', *, *, #24493, .T. ) ;
#27356=DIRECTION ( 'NONE',  ( -1.000000000000000000, 0.000000000000000000, 0.000000000000000000 ) ) ;
#27357=FACE_OUTER_BOUND ( 'NONE', #13248, .T. ) ;
#27358=ORIENTED_EDGE ( 'NONE', *, *, #21793, .F. ) ;
#27359=DIRECTION ( 'NONE',  ( 0.000000000000000000, 0.000000000000000000, 1.000000000000000000 ) ) ;
#27360=DIRECTION ( 'NONE',  ( 0.000000000000000000, 0.000000000000000000, -1.000000000000000000 ) ) ;
#27361=CARTESIAN_POINT ( 'NONE',  ( -87.00000337463093558, -8.660254037844422825, 12.50000000000000000 ) ) ;
#27362=VECTOR ( 'NONE', #3406, 1000.000000000000000 ) ;
#27368=CYLINDRICAL_SURFACE ( 'NONE', #17847, 2.000000000000001776 ) ;
#27369=EDGE_LOOP ( 'NONE', ( #35887, #36989 ) ) ;
#27372=DIRECTION ( 'NONE',  ( 1.000000000000000000, 0.000000000000000000, 0.000000000000000000 ) ) ;
#27373=VECTOR ( 'NONE', #33077, 1000.000000000000000 ) ;
#27374=DIRECTION ( 'NONE',  ( 0.000000000000000000, 0.000000000000000000, 1.000000000000000000 ) ) ;
#27375=EDGE_CURVE ( 'NONE', #985, #30974, #27258, .T. ) ;
#27376=CARTESIAN_POINT ( 'NONE',  ( -32.49191361593891259, -89.27079897466116165, 12.49999999999999822 ) ) ;
#27377=DIRECTION ( 'NONE',  ( 0.000000000000000000, 0.000000000000000000, 1.000000000000000000 ) ) ;
#27378=LINE ( 'NONE', #33930, #34452 ) ;
#27379=ORIENTED_EDGE ( 'NONE', *, *, #30719, .T. ) ;
#27380=CARTESIAN_POINT ( 'NONE',  ( -53.00000337463106348, 60.62177826491078747, -5.000000000000000000 ) ) ;
#27381=VECTOR ( 'NONE', #36915, 1000.000000000000000 ) ;
#27383=AXIS2_PLACEMENT_3D ( 'NONE', #5547, #466, #11704 ) ;
#27385=EDGE_LOOP ( 'NONE', ( #5692, #15706 ) ) ;
#27387=EDGE_LOOP ( 'NONE', ( #17150, #9802, #16969, #34552 ) ) ;
#27388=AXIS2_PLACEMENT_3D ( 'NONE', #18514, #21503, #29937 ) ;
#27389=( NAMED_UNIT ( * ) PLANE_ANGLE_UNIT ( ) SI_UNIT ( $, .RADIAN. ) );
#27391=AXIS2_PLACEMENT_3D ( 'NONE', #7328, #3761, #15199 ) ;
#27392=CARTESIAN_POINT ( 'NONE',  ( 81.99999662536833966, 34.64101615137759183, -9.999999999999998224 ) ) ;
#27393=CIRCLE ( 'NONE', #1647, 2.000000000000001776 ) ;
#27395=ORIENTED_EDGE ( 'NONE', *, *, #34850, .F. ) ;
#27398=ADVANCED_FACE ( 'NONE', ( #25567 ), #28006, .T. ) ;
#27399=CIRCLE ( 'NONE', #35789, 2.000000000000001776 ) ;
#27400=ORIENTED_EDGE ( 'NONE', *, *, #18566, .T. ) ;
#27401=DIRECTION ( 'NONE',  ( -0.000000000000000000, -0.000000000000000000, 1.000000000000000000 ) ) ;
#27402=CARTESIAN_POINT ( 'NONE',  ( -82.00000337463094979, -17.32050807568882078, 12.50000000000000000 ) ) ;
#27403=EDGE_CURVE ( 'NONE', #12539, #12117, #26083, .T. ) ;
#27404=DIRECTION ( 'NONE',  ( 0.000000000000000000, 0.000000000000000000, 1.000000000000000000 ) ) ;
#27405=CARTESIAN_POINT ( 'NONE',  ( 11.99999662536865763, -69.28203230275519786, 12.50000000000000000 ) ) ;
#27407=ORIENTED_EDGE ( 'NONE', *, *, #3405, .F. ) ;
#27410=DIRECTION ( 'NONE',  ( -1.000000000000000000, 0.000000000000000000, 0.000000000000000000 ) ) ;
#27411=EDGE_CURVE ( 'NONE', #5750, #33336, #30869, .T. ) ;
#27413=VERTEX_POINT ( 'NONE', #30798 ) ;
#27414=CARTESIAN_POINT ( 'NONE',  ( 76.99999662536836809, 25.98076211353319565, -9.999999999999998224 ) ) ;
#27415=DIRECTION ( 'NONE',  ( 0.000000000000000000, 0.000000000000000000, 1.000000000000000000 ) ) ;
#27417=ORIENTED_EDGE ( 'NONE', *, *, #13867, .F. ) ;
#27418=ORIENTED_EDGE ( 'NONE', *, *, #27317, .T. ) ;
#27419=DIRECTION ( 'NONE',  ( 1.000000000000000000, 0.000000000000000000, 0.000000000000000000 ) ) ;
#27420=EDGE_CURVE ( 'NONE', #10442, #20675, #30257, .T. ) ;
#27421=CARTESIAN_POINT ( 'NONE',  ( -52.39915983220772233, -35.19434990244957362, -4.999999999999997335 ) ) ;
#27423=ORIENTED_EDGE ( 'NONE', *, *, #6843, .T. ) ;
#27424=ORIENTED_EDGE ( 'NONE', *, *, #5728, .F. ) ;
#27427=CIRCLE ( 'NONE', #23224, 2.000000000000001776 ) ;
#27428=FACE_OUTER_BOUND ( 'NONE', #19825, .T. ) ;
#27429=EDGE_LOOP ( 'NONE', ( #34032, #5394, #22085, #29866, #33552, #19042 ) ) ;
#27430=DIRECTION ( 'NONE',  ( -1.000000000000000000, 0.000000000000000000, 0.000000000000000000 ) ) ;
#27431=VERTEX_POINT ( 'NONE', #16574 ) ;
#27432=VERTEX_POINT ( 'NONE', #2332 ) ;
#27433=CIRCLE ( 'NONE', #2281, 2.000000000000000000 ) ;
#27434=DIRECTION ( 'NONE',  ( 0.000000000000000000, 0.000000000000000000, 1.000000000000000000 ) ) ;
#27435=EDGE_CURVE ( 'NONE', #4953, #1362, #10510, .T. ) ;
#27437=ORIENTED_EDGE ( 'NONE', *, *, #27403, .T. ) ;
#27438=ORIENTED_EDGE ( 'NONE', *, *, #32320, .F. ) ;
#27439=CARTESIAN_POINT ( 'NONE',  ( 84.99999662536832545, 8.660254037844394404, -9.999999999999998224 ) ) ;
#27441=DIRECTION ( 'NONE',  ( 0.000000000000000000, 0.000000000000000000, 1.000000000000000000 ) ) ;
#27442=CARTESIAN_POINT ( 'NONE',  ( 36.99999662536855283, -77.94228634059960825, -5.000000000000000000 ) ) ;
#27443=FACE_OUTER_BOUND ( 'NONE', #2889, .T. ) ;
#27444=ORIENTED_EDGE ( 'NONE', *, *, #29791, .T. ) ;
#27445=CARTESIAN_POINT ( 'NONE',  ( 61.99999662536842493, -51.96152422706639840, 12.50000000000000000 ) ) ;
#27446=CIRCLE ( 'NONE', #3527, 2.000000000000001776 ) ;
#27448=CARTESIAN_POINT ( 'NONE',  ( 68.19434990244977257, -52.39915983220758022, -4.999999999999997335 ) ) ;
#27449=ADVANCED_FACE ( 'NONE', ( #5505 ), #11317, .T. ) ;
#27450=CIRCLE ( 'NONE', #11286, 1.999999999999998224 ) ;
#27451=CYLINDRICAL_SURFACE ( 'NONE', #18411, 3.000000000000002665 ) ;
#27453=DIRECTION ( 'NONE',  ( 0.000000000000000000, 0.000000000000000000, 1.000000000000000000 ) ) ;
#27454=LINE ( 'NONE', #1773, #7515 ) ;
#27455=CIRCLE ( 'NONE', #500, 3.000000000000002665 ) ;
#27456=CARTESIAN_POINT ( 'NONE',  ( -63.00000337463102085, 25.98076211353317433, 12.50000000000000000 ) ) ;
#27457=EDGE_CURVE ( 'NONE', #34186, #19449, #3616, .T. ) ;
#27458=CIRCLE ( 'NONE', #12479, 2.000000000000001776 ) ;
#27459=DIRECTION ( 'NONE',  ( 1.000000000000000000, 0.000000000000000000, 0.000000000000000000 ) ) ;
#27460=VERTEX_POINT ( 'NONE', #14861 ) ;
#27461=DIRECTION ( 'NONE',  ( 0.000000000000000000, 0.000000000000000000, 1.000000000000000000 ) ) ;
#27462=DIRECTION ( 'NONE',  ( 0.000000000000000000, 0.000000000000000000, 1.000000000000000000 ) ) ;
#27463=CARTESIAN_POINT ( 'NONE',  ( 64.99999662536839651, 60.62177826491078747, 12.50000000000000000 ) ) ;
#27465=VERTEX_POINT ( 'NONE', #6058 ) ;
#27466=CIRCLE ( 'NONE', #8315, 2.000000000000001776 ) ;
#27467=VERTEX_POINT ( 'NONE', #29288 ) ;
#27470=DIRECTION ( 'NONE',  ( 0.000000000000000000, 0.000000000000000000, 1.000000000000000000 ) ) ;
#27471=ORIENTED_EDGE ( 'NONE', *, *, #23989, .F. ) ;
#27472=LINE ( 'NONE', #18851, #32289 ) ;
#27473=EDGE_CURVE ( 'NONE', #25535, #691, #9295, .T. ) ;
#27476=ORIENTED_EDGE ( 'NONE', *, *, #12359, .T. ) ;
#27477=LINE ( 'NONE', #4967, #26950 ) ;
#27479=VECTOR ( 'NONE', #9252, 1000.000000000000000 ) ;
#27480=CARTESIAN_POINT ( 'NONE',  ( -35.00000337463116296, 60.62177826491077326, -5.000000000000000000 ) ) ;
#27483=FACE_OUTER_BOUND ( 'NONE', #18426, .T. ) ;
#27484=CIRCLE ( 'NONE', #1146, 1.999999999999998224 ) ;
#27485=ADVANCED_FACE ( 'NONE', ( #26106 ), #32463, .T. ) ;
#27486=LINE ( 'NONE', #33494, #12780 ) ;
#27487=ORIENTED_EDGE ( 'NONE', *, *, #21432, .T. ) ;
#27488=CARTESIAN_POINT ( 'NONE',  ( 0.000000000000000000, 0.000000000000000000, 17.49999999999999645 ) ) ;
#27489=AXIS2_PLACEMENT_3D ( 'NONE', #20573, #26227, #26409 ) ;
#27491=CARTESIAN_POINT ( 'NONE',  ( -3.374631327851540519E-06, 86.60254037844397601, -9.999999999999998224 ) ) ;
#27492=CIRCLE ( 'NONE', #8940, 2.000000000000001776 ) ;
#27494=LINE ( 'NONE', #7428, #4823 ) ;
#27495=CARTESIAN_POINT ( 'NONE',  ( -75.00000337463099243, -25.98076211353322051, -9.999999999999998224 ) ) ;
#27496=ORIENTED_EDGE ( 'NONE', *, *, #2072, .T. ) ;
#27497=AXIS2_PLACEMENT_3D ( 'NONE', #4872, #36170, #16125 ) ;
#27498=DIRECTION ( 'NONE',  ( 0.000000000000000000, 0.000000000000000000, 1.000000000000000000 ) ) ;
#27499=CYLINDRICAL_SURFACE ( 'NONE', #26867, 33.00000000000001421 ) ;
#27500=CARTESIAN_POINT ( 'NONE',  ( 76.71706219562628348, -9.685771384082237034, -5.000000000000000000 ) ) ;
#27501=ORIENTED_EDGE ( 'NONE', *, *, #21690, .F. ) ;
#27502=EDGE_CURVE ( 'NONE', #21745, #8482, #11849, .T. ) ;
#27503=CIRCLE ( 'NONE', #5358, 2.000000000000001776 ) ;
#27504=ORIENTED_EDGE ( 'NONE', *, *, #11175, .T. ) ;
#27505=AXIS2_PLACEMENT_3D ( 'NONE', #4768, #19012, #35699 ) ;
#27508=DIRECTION ( 'NONE',  ( 0.000000000000000000, 0.000000000000000000, 1.000000000000000000 ) ) ;
#27509=ORIENTED_EDGE ( 'NONE', *, *, #32427, .T. ) ;
#27510=AXIS2_PLACEMENT_3D ( 'NONE', #15847, #23937, #21661 ) ;
#27511=FACE_OUTER_BOUND ( 'NONE', #21515, .T. ) ;
#27512=DIRECTION ( 'NONE',  ( -1.000000000000000000, 0.000000000000000000, 0.000000000000000000 ) ) ;
#27514=CIRCLE ( 'NONE', #25734, 2.000000000000001776 ) ;
#27515=CARTESIAN_POINT ( 'NONE',  ( 54.99999662536844625, 43.30127018922198801, 17.49999999999999645 ) ) ;
#27516=VERTEX_POINT ( 'NONE', #780 ) ;
#27517=VERTEX_POINT ( 'NONE', #9046 ) ;
#27521=DIRECTION ( 'NONE',  ( 0.000000000000000000, 0.000000000000000000, 1.000000000000000000 ) ) ;
#27522=ORIENTED_EDGE ( 'NONE', *, *, #12992, .T. ) ;
#27523=ADVANCED_FACE ( 'NONE', ( #12193 ), #23663, .T. ) ;
#27525=EDGE_LOOP ( 'NONE', ( #8076, #18649, #10137, #30765 ) ) ;
#27526=EDGE_CURVE ( 'NONE', #36755, #20745, #15217, .T. ) ;
#27527=DIRECTION ( 'NONE',  ( 0.000000000000000000, 0.000000000000000000, 1.000000000000000000 ) ) ;
#27528=EDGE_CURVE ( 'NONE', #2589, #14801, #27874, .T. ) ;
#27529=LINE ( 'NONE', #21534, #534 ) ;
#27530=AXIS2_PLACEMENT_3D ( 'NONE', #17394, #37093, #28812 ) ;
#27531=EDGE_LOOP ( 'NONE', ( #6937, #14258 ) ) ;
#27532=EDGE_CURVE ( 'NONE', #36216, #33068, #32022, .T. ) ;
#27533=VECTOR ( 'NONE', #23560, 1000.000000000000000 ) ;
#27534=CYLINDRICAL_SURFACE ( 'NONE', #26039, 2.000000000000000000 ) ;
#27535=EDGE_LOOP ( 'NONE', ( #25912, #11284, #5434, #34889 ) ) ;
#27536=ADVANCED_FACE ( 'NONE', ( #35316 ), #414, .F. ) ;
#27538=DIRECTION ( 'NONE',  ( -1.000000000000000000, 0.000000000000000000, 0.000000000000000000 ) ) ;
#27539=DIRECTION ( 'NONE',  ( -1.000000000000000000, 0.000000000000000000, -0.000000000000000000 ) ) ;
#27540=VERTEX_POINT ( 'NONE', #3232 ) ;
#27541=CARTESIAN_POINT ( 'NONE',  ( -75.00000337463099243, -25.98076211353322051, -9.999999999999998224 ) ) ;
#27542=DIRECTION ( 'NONE',  ( -1.000000000000000000, 0.000000000000000000, 0.000000000000000000 ) ) ;
#27544=AXIS2_PLACEMENT_3D ( 'NONE', #1048, #12473, #26540 ) ;
#27545=EDGE_CURVE ( 'NONE', #31097, #5072, #21035, .T. ) ;
#27546=ORIENTED_EDGE ( 'NONE', *, *, #21291, .F. ) ;
#27548=ADVANCED_FACE ( 'NONE', ( #31891 ), #25926, .F. ) ;
#27549=ORIENTED_EDGE ( 'NONE', *, *, #31420, .T. ) ;
#27550=EDGE_LOOP ( 'NONE', ( #35332, #2158, #3913, #2629, #13692, #11791 ) ) ;
#27551=EDGE_CURVE ( 'NONE', #32323, #36578, #24896, .T. ) ;
#27553=VECTOR ( 'NONE', #31006, 1000.000000000000000 ) ;
#27554=DIRECTION ( 'NONE',  ( 0.000000000000000000, 0.000000000000000000, 1.000000000000000000 ) ) ;
#27558=AXIS2_PLACEMENT_3D ( 'NONE', #16340, #36211, #27756 ) ;
#27559=CARTESIAN_POINT ( 'NONE',  ( -28.00000337463118427, 69.28203230275516944, 17.49999999999999645 ) ) ;
#27561=VECTOR ( 'NONE', #28946, 1000.000000000000000 ) ;
#27562=DIRECTION ( 'NONE',  ( 1.000000000000000000, 0.000000000000000000, 0.000000000000000000 ) ) ;
#27564=DIRECTION ( 'NONE',  ( 1.000000000000000000, -0.000000000000000000, 0.000000000000000000 ) ) ;
#27566=DIRECTION ( 'NONE',  ( 1.000000000000000000, 0.000000000000000000, 0.000000000000000000 ) ) ;
#27567=DIRECTION ( 'NONE',  ( 0.000000000000000000, 0.000000000000000000, 1.000000000000000000 ) ) ;
#27568=VERTEX_POINT ( 'NONE', #35488 ) ;
#27569=ORIENTED_EDGE ( 'NONE', *, *, #7395, .F. ) ;
#27570=CARTESIAN_POINT ( 'NONE',  ( -30.99999999999944933, 58.88972745734214698, -49.86561046011506448 ) ) ;
#27571=CARTESIAN_POINT ( 'NONE',  ( 49.99999662536846756, -69.28203230275519786, -9.999999999999998224 ) ) ;
#27572=VECTOR ( 'NONE', #15618, 1000.000000000000000 ) ;
#27573=CARTESIAN_POINT ( 'NONE',  ( 11.64412580323855018, 85.46375187899521109, 12.50000000000000000 ) ) ;
#27574=ORIENTED_EDGE ( 'NONE', *, *, #12008, .T. ) ;
#27576=CARTESIAN_POINT ( 'NONE',  ( -52.00000337463109190, 51.96152422706637708, 17.49999999999999645 ) ) ;
#27579=AXIS2_PLACEMENT_3D ( 'NONE', #567, #11444, #3028 ) ;
#27583=CARTESIAN_POINT ( 'NONE',  ( -63.00000337463104927, -43.30127018922202353, -9.999999999999998224 ) ) ;
#27584=DIRECTION ( 'NONE',  ( 1.000000000000000000, 0.000000000000000000, 0.000000000000000000 ) ) ;
#27587=ORIENTED_EDGE ( 'NONE', *, *, #34306, .T. ) ;
#27588=LINE ( 'NONE', #23910, #24576 ) ;
#27589=ORIENTED_EDGE ( 'NONE', *, *, #14044, .F. ) ;
#27590=DIRECTION ( 'NONE',  ( 0.000000000000000000, 0.000000000000000000, 1.000000000000000000 ) ) ;
#27591=ADVANCED_FACE ( 'NONE', ( #18976 ), #33410, .F. ) ;
#27592=DIRECTION ( 'NONE',  ( 0.000000000000000000, 0.000000000000000000, 1.000000000000000000 ) ) ;
#27593=DIRECTION ( 'NONE',  ( 0.000000000000000000, 0.000000000000000000, -1.000000000000000000 ) ) ;
#27594=CARTESIAN_POINT ( 'NONE',  ( -82.00000337463094979, 34.64101615137757051, -9.999999999999998224 ) ) ;
#27596=ORIENTED_EDGE ( 'NONE', *, *, #22780, .F. ) ;
#27598=DIRECTION ( 'NONE',  ( 0.000000000000000000, 0.000000000000000000, 1.000000000000000000 ) ) ;
#27599=CIRCLE ( 'NONE', #28794, 33.00000000000002132 ) ;
#27600=ORIENTED_EDGE ( 'NONE', *, *, #33713, .T. ) ;
#27601=CARTESIAN_POINT ( 'NONE',  ( -80.00000337463094979, 17.32050807568878525, -9.999999999999998224 ) ) ;
#27602=CARTESIAN_POINT ( 'NONE',  ( 7.999996625368656744, -69.28203230275519786, 12.50000000000000000 ) ) ;
#27603=ORIENTED_EDGE ( 'NONE', *, *, #9736, .F. ) ;
#27604=EDGE_LOOP ( 'NONE', ( #34765, #13813, #24133, #32161, #32224, #36555 ) ) ;
#27605=FACE_OUTER_BOUND ( 'NONE', #11884, .T. ) ;
#27607=DIRECTION ( 'NONE',  ( 0.000000000000000000, 0.000000000000000000, 1.000000000000000000 ) ) ;
#27609=ORIENTED_EDGE ( 'NONE', *, *, #19094, .F. ) ;
#27611=EDGE_CURVE ( 'NONE', #20763, #25354, #1536, .T. ) ;
#27612=DIRECTION ( 'NONE',  ( 0.000000000000000000, 0.000000000000000000, 1.000000000000000000 ) ) ;
#27613=ORIENTED_EDGE ( 'NONE', *, *, #17926, .T. ) ;
#27614=DIRECTION ( 'NONE',  ( 1.000000000000000000, 0.000000000000000000, 0.000000000000000000 ) ) ;
#27615=ORIENTED_EDGE ( 'NONE', *, *, #35657, .T. ) ;
#27616=ORIENTED_EDGE ( 'NONE', *, *, #150, .F. ) ;
#27617=CYLINDRICAL_SURFACE ( 'NONE', #10044, 2.000000000000001776 ) ;
#27618=CYLINDRICAL_SURFACE ( 'NONE', #15286, 2.000000000000001776 ) ;
#27620=ORIENTED_EDGE ( 'NONE', *, *, #15312, .T. ) ;
#27622=DIRECTION ( 'NONE',  ( 1.000000000000000000, 0.000000000000000000, 0.000000000000000000 ) ) ;
#27624=DIRECTION ( 'NONE',  ( 0.8660254037844344888, -0.5000000000000071054, 0.000000000000000000 ) ) ;
#27625=ORIENTED_EDGE ( 'NONE', *, *, #27053, .F. ) ;
#27626=CARTESIAN_POINT ( 'NONE',  ( 69.99999662536841072, 51.96152422706640550, 17.49999999999999645 ) ) ;
#27627=ADVANCED_FACE ( 'NONE', ( #10523 ), #18421, .F. ) ;
#27628=FACE_BOUND ( 'NONE', #29718, .T. ) ;
#27629=CARTESIAN_POINT ( 'NONE',  ( 76.99999662536836809, 25.98076211353319565, -5.000000000000000000 ) ) ;
#27630=CARTESIAN_POINT ( 'NONE',  ( 0.000000000000000000, 0.000000000000000000, -5.000000000000000000 ) ) ;
#27632=LINE ( 'NONE', #1575, #25475 ) ;
#27633=DIRECTION ( 'NONE',  ( -1.000000000000000000, 0.000000000000000000, 0.000000000000000000 ) ) ;
#27637=CARTESIAN_POINT ( 'NONE',  ( -50.00000337463110611, -69.28203230275519786, -5.000000000000000000 ) ) ;
#27638=CIRCLE ( 'NONE', #30020, 33.00000000000001421 ) ;
#27639=CARTESIAN_POINT ( 'NONE',  ( -83.00000337463092137, 8.660254037844389075, 17.49999999999999645 ) ) ;
#27640=CARTESIAN_POINT ( 'NONE',  ( -62.00000337463108480, -51.96152422706641971, -9.999999999999998224 ) ) ;
#27641=ORIENTED_EDGE ( 'NONE', *, *, #23189, .F. ) ;
#27642=ORIENTED_EDGE ( 'NONE', *, *, #21556, .T. ) ;
#27643=EDGE_LOOP ( 'NONE', ( #8487, #32050 ) ) ;
#27644=EDGE_CURVE ( 'NONE', #7812, #11869, #9967, .T. ) ;
#27645=CARTESIAN_POINT ( 'NONE',  ( -67.00000337463102085, 60.62177826491077326, 12.50000000000000000 ) ) ;
#27647=ORIENTED_EDGE ( 'NONE', *, *, #11736, .T. ) ;
#27648=EDGE_CURVE ( 'NONE', #745, #27432, #31401, .T. ) ;
#27649=LINE ( 'NONE', #27823, #22113 ) ;
#27650=CARTESIAN_POINT ( 'NONE',  ( -70.00000337463100664, -17.32050807568882078, 12.50000000000000000 ) ) ;
#27653=EDGE_CURVE ( 'NONE', #7366, #32947, #29689, .T. ) ;
#27654=ORIENTED_EDGE ( 'NONE', *, *, #16174, .F. ) ;
#27655=FACE_BOUND ( 'NONE', #25693, .T. ) ;
#27657=DIRECTION ( 'NONE',  ( 0.000000000000000000, 0.000000000000000000, 1.000000000000000000 ) ) ;
#27659=DIRECTION ( 'NONE',  ( 0.000000000000000000, 0.000000000000000000, 1.000000000000000000 ) ) ;
#27660=ORIENTED_EDGE ( 'NONE', *, *, #10867, .F. ) ;
#27661=DIRECTION ( 'NONE',  ( 0.000000000000000000, 0.000000000000000000, 1.000000000000000000 ) ) ;
#27665=VERTEX_POINT ( 'NONE', #12958 ) ;
#27666=DIRECTION ( 'NONE',  ( 0.000000000000000000, 0.000000000000000000, -1.000000000000000000 ) ) ;
#27668=VERTEX_POINT ( 'NONE', #21773 ) ;
#27669=CARTESIAN_POINT ( 'NONE',  ( 19.99999662536857770, 86.60254037844397601, 12.50000000000000000 ) ) ;
#27670=CARTESIAN_POINT ( 'NONE',  ( 72.77422209630367433, 61.06482292022032965, 12.49999999999999822 ) ) ;
#27671=DIRECTION ( 'NONE',  ( 0.000000000000000000, 0.000000000000000000, 1.000000000000000000 ) ) ;
#27672=EDGE_CURVE ( 'NONE', #1110, #17463, #5660, .T. ) ;
#27673=ORIENTED_EDGE ( 'NONE', *, *, #13793, .F. ) ;
#27674=VERTEX_POINT ( 'NONE', #24043 ) ;
#27676=DIRECTION ( 'NONE',  ( 0.000000000000000000, 0.000000000000000000, 1.000000000000000000 ) ) ;
#27678=LINE ( 'NONE', #19261, #36286 ) ;
#27679=ORIENTED_EDGE ( 'NONE', *, *, #10131, .F. ) ;
#27680=EDGE_LOOP ( 'NONE', ( #5906, #7346, #36058, #19231, #9054, #35352, #16197, #4529, #15721, #7105, #18739, #27417, #18647, #26464, #18170, #21422 ) ) ;
#27683=DIRECTION ( 'NONE',  ( 0.000000000000000000, 0.000000000000000000, -1.000000000000000000 ) ) ;
#27684=DIRECTION ( 'NONE',  ( 0.000000000000000000, 0.000000000000000000, -1.000000000000000000 ) ) ;
#27687=ORIENTED_EDGE ( 'NONE', *, *, #25440, .T. ) ;
#27688=ORIENTED_EDGE ( 'NONE', *, *, #29017, .F. ) ;
#27689=DIRECTION ( 'NONE',  ( 0.000000000000000000, 0.000000000000000000, 1.000000000000000000 ) ) ;
#27690=CARTESIAN_POINT ( 'NONE',  ( -34.00000000000027711, -58.88972745734168512, -49.22241343995298024 ) ) ;
#27691=ORIENTED_EDGE ( 'NONE', *, *, #30353, .T. ) ;
#27692=FACE_OUTER_BOUND ( 'NONE', #11125, .T. ) ;
#27693=VERTEX_POINT ( 'NONE', #18613 ) ;
#27694=DIRECTION ( 'NONE',  ( 0.000000000000000000, 0.000000000000000000, 1.000000000000000000 ) ) ;
#27697=DIRECTION ( 'NONE',  ( 1.000000000000000000, 0.000000000000000000, 0.000000000000000000 ) ) ;
#27698=FACE_OUTER_BOUND ( 'NONE', #34947, .T. ) ;
#27699=ORIENTED_EDGE ( 'NONE', *, *, #20218, .T. ) ;
#27700=CYLINDRICAL_SURFACE ( 'NONE', #27830, 2.000000000000000000 ) ;
#27701=CIRCLE ( 'NONE', #25919, 2.000000000000001776 ) ;
#27702=DIRECTION ( 'NONE',  ( 1.000000000000000000, 0.000000000000000000, 0.000000000000000000 ) ) ;
#27704=ORIENTED_EDGE ( 'NONE', *, *, #11756, .F. ) ;
#27705=CIRCLE ( 'NONE', #36105, 2.000000000000001776 ) ;
#27707=CARTESIAN_POINT ( 'NONE',  ( -70.00000337463102085, -34.64101615137762025, -9.999999999999998224 ) ) ;
#27708=DIRECTION ( 'NONE',  ( 1.000000000000000000, 0.000000000000000000, 0.000000000000000000 ) ) ;
#27709=EDGE_LOOP ( 'NONE', ( #21159, #5721, #11863, #2415 ) ) ;
#27710=ORIENTED_EDGE ( 'NONE', *, *, #8262, .T. ) ;
#27711=EDGE_CURVE ( 'NONE', #33896, #10442, #8656, .T. ) ;
#27713=CARTESIAN_POINT ( 'NONE',  ( 59.99999662536842493, -51.96152422706639840, -9.999999999999998224 ) ) ;
#27714=EDGE_CURVE ( 'NONE', #26973, #3118, #20699, .T. ) ;
#27717=CARTESIAN_POINT ( 'NONE',  ( -75.00000337463097821, 43.30127018922197379, 12.50000000000000000 ) ) ;
#27718=EDGE_CURVE ( 'NONE', #31778, #12006, #15237, .T. ) ;
#27719=CIRCLE ( 'NONE', #20511, 2.000000000000001776 ) ;
#27721=DIRECTION ( 'NONE',  ( 0.000000000000000000, 0.000000000000000000, 1.000000000000000000 ) ) ;
#27725=DIRECTION ( 'NONE',  ( 0.000000000000000000, 0.000000000000000000, 1.000000000000000000 ) ) ;
#27727=CARTESIAN_POINT ( 'NONE',  ( -28.00000337463119493, -69.28203230275522628, -9.999999999999998224 ) ) ;
#27731=VECTOR ( 'NONE', #33075, 1000.000000000000000 ) ;
#27732=CARTESIAN_POINT ( 'NONE',  ( 62.99999662536842493, 43.30127018922200222, -5.000000000000000000 ) ) ;
#27733=DIRECTION ( 'NONE',  ( 1.000000000000000000, 0.000000000000000000, 0.000000000000000000 ) ) ;
#27734=LINE ( 'NONE', #33579, #5930 ) ;
#27736=EDGE_CURVE ( 'NONE', #20758, #27194, #8458, .T. ) ;
#27737=EDGE_CURVE ( 'NONE', #35393, #12539, #951, .T. ) ;
#27738=DIRECTION ( 'NONE',  ( 0.000000000000000000, 0.000000000000000000, -1.000000000000000000 ) ) ;
#27740=DIRECTION ( 'NONE',  ( 0.000000000000000000, 0.000000000000000000, 1.000000000000000000 ) ) ;
#27741=ORIENTED_EDGE ( 'NONE', *, *, #1514, .T. ) ;
#27742=CYLINDRICAL_SURFACE ( 'NONE', #3877, 3.000000000000002665 ) ;
#27744=EDGE_LOOP ( 'NONE', ( #10227, #11773, #18540, #29982, #18181, #22178 ) ) ;
#27745=CARTESIAN_POINT ( 'NONE',  ( 4.279621169095998212, -62.97617850287780072, 12.49999999999999822 ) ) ;
#27746=AXIS2_PLACEMENT_3D ( 'NONE', #14032, #36739, #8248 ) ;
#27747=PLANE ( 'NONE',  #11597 ) ;
#27750=ORIENTED_EDGE ( 'NONE', *, *, #32164, .F. ) ;
#27751=CIRCLE ( 'NONE', #24176, 3.000000000000007550 ) ;
#27752=ADVANCED_FACE ( 'NONE', ( #28149 ), #8627, .F. ) ;
#27755=AXIS2_PLACEMENT_3D ( 'NONE', #10937, #22377, #13210 ) ;
#27756=DIRECTION ( 'NONE',  ( -1.000000000000000000, 0.000000000000000000, 0.000000000000000000 ) ) ;
#27757=EDGE_CURVE ( 'NONE', #25195, #4245, #2752, .T. ) ;
#27758=CARTESIAN_POINT ( 'NONE',  ( 0.000000000000000000, 0.000000000000000000, -5.000000000000000000 ) ) ;
#27761=ORIENTED_EDGE ( 'NONE', *, *, #12008, .F. ) ;
#27762=CIRCLE ( 'NONE', #22986, 2.000000000000001776 ) ;
#27764=CARTESIAN_POINT ( 'NONE',  ( 68.00000000000000000, 0.000000000000000000, 12.49999999999999822 ) ) ;
#27765=FACE_OUTER_BOUND ( 'NONE', #7261, .T. ) ;
#27766=ORIENTED_EDGE ( 'NONE', *, *, #21797, .T. ) ;
#27767=DIRECTION ( 'NONE',  ( 1.000000000000000000, 0.000000000000000000, 0.000000000000000000 ) ) ;
#27768=EDGE_CURVE ( 'NONE', #23390, #16038, #30762, .T. ) ;
#27769=CARTESIAN_POINT ( 'NONE',  ( -22.00000337463124112, -86.60254037844400443, -9.999999999999998224 ) ) ;
#27770=ORIENTED_EDGE ( 'NONE', *, *, #19979, .F. ) ;
#27771=AXIS2_PLACEMENT_3D ( 'NONE', #26401, #9320, #3880 ) ;
#27772=ORIENTED_EDGE ( 'NONE', *, *, #26377, .T. ) ;
#27773=DIRECTION ( 'NONE',  ( 3.491481338843133355E-15, 1.000000000000000000, 0.000000000000000000 ) ) ;
#27774=CARTESIAN_POINT ( 'NONE',  ( -80.00000337463094979, -17.32050807568882078, 17.49999999999999645 ) ) ;
#27775=DIRECTION ( 'NONE',  ( 1.000000000000000000, 0.000000000000000000, 0.000000000000000000 ) ) ;
#27777=ORIENTED_EDGE ( 'NONE', *, *, #4607, .T. ) ;
#27778=ORIENTED_EDGE ( 'NONE', *, *, #22872, .F. ) ;
#27779=ADVANCED_FACE ( 'NONE', ( #25172 ), #17069, .T. ) ;
#27780=AXIS2_PLACEMENT_3D ( 'NONE', #27015, #24601, #27584 ) ;
#27781=EDGE_CURVE ( 'NONE', #26973, #12879, #10721, .T. ) ;
#27782=DIRECTION ( 'NONE',  ( 0.000000000000000000, 0.000000000000000000, 1.000000000000000000 ) ) ;
#27783=EDGE_CURVE ( 'NONE', #31670, #18483, #36963, .T. ) ;
#27785=VERTEX_POINT ( 'NONE', #22889 ) ;
#27787=DIRECTION ( 'NONE',  ( 1.000000000000000000, 0.000000000000000000, 0.000000000000000000 ) ) ;
#27788=EDGE_LOOP ( 'NONE', ( #14186, #30862, #36588, #28215 ) ) ;
#27790=LINE ( 'NONE', #24070, #26789 ) ;
#27792=ORIENTED_EDGE ( 'NONE', *, *, #10995, .F. ) ;
#27794=DIRECTION ( 'NONE',  ( 1.000000000000000000, 0.000000000000000000, 0.000000000000000000 ) ) ;
#27795=FACE_OUTER_BOUND ( 'NONE', #28068, .T. ) ;
#27796=DIRECTION ( 'NONE',  ( 0.000000000000000000, 0.000000000000000000, 1.000000000000000000 ) ) ;
#27797=DIRECTION ( 'NONE',  ( 0.000000000000000000, 0.000000000000000000, 1.000000000000000000 ) ) ;
#27798=AXIS2_PLACEMENT_3D ( 'NONE', #5943, #2946, #9100 ) ;
#27799=ORIENTED_EDGE ( 'NONE', *, *, #18999, .F. ) ;
#27800=DIRECTION ( 'NONE',  ( -0.000000000000000000, -0.000000000000000000, 1.000000000000000000 ) ) ;
#27801=FACE_BOUND ( 'NONE', #16638, .T. ) ;
#27802=DIRECTION ( 'NONE',  ( 0.000000000000000000, 0.000000000000000000, -1.000000000000000000 ) ) ;
#27803=FACE_BOUND ( 'NONE', #22322, .T. ) ;
#27804=DIRECTION ( 'NONE',  ( 0.000000000000000000, 0.000000000000000000, -1.000000000000000000 ) ) ;
#27805=ADVANCED_FACE ( 'NONE', ( #34325 ), #4911, .F. ) ;
#27807=AXIS2_PLACEMENT_3D ( 'NONE', #14989, #26417, #23597 ) ;
#27809=AXIS2_PLACEMENT_3D ( 'NONE', #35826, #16135, #18577 ) ;
#27810=CARTESIAN_POINT ( 'NONE',  ( -17.00000337463126243, 77.94228634059957983, -9.999999999999998224 ) ) ;
#27811=ORIENTED_EDGE ( 'NONE', *, *, #9640, .T. ) ;
#27812=DIRECTION ( 'NONE',  ( 0.000000000000000000, 0.000000000000000000, -1.000000000000000000 ) ) ;
#27814=CARTESIAN_POINT ( 'NONE',  ( -60.00000337463104216, 34.64101615137757051, -5.000000000000000000 ) ) ;
#27815=VERTEX_POINT ( 'NONE', #16893 ) ;
#27816=ORIENTED_EDGE ( 'NONE', *, *, #14392, .F. ) ;
#27818=DIRECTION ( 'NONE',  ( 0.000000000000000000, 0.000000000000000000, 1.000000000000000000 ) ) ;
#27819=CYLINDRICAL_SURFACE ( 'NONE', #166, 2.000000000000001776 ) ;
#27820=AXIS2_PLACEMENT_3D ( 'NONE', #29788, #26602, #33681 ) ;
#27822=CIRCLE ( 'NONE', #11645, 2.000000000000000000 ) ;
#27823=CARTESIAN_POINT ( 'NONE',  ( -43.00000337463112743, -60.62177826491080168, -9.999999999999998224 ) ) ;
#27824=CARTESIAN_POINT ( 'NONE',  ( -50.00000337463109190, 51.96152422706637708, -9.999999999999998224 ) ) ;
#27826=EDGE_CURVE ( 'NONE', #33506, #29268, #2157, .T. ) ;
#27827=CARTESIAN_POINT ( 'NONE',  ( 80.69570903995992239, -15.44541228182035475, 12.50000000000000000 ) ) ;
#27828=ORIENTED_EDGE ( 'NONE', *, *, #35813, .T. ) ;
#27829=CARTESIAN_POINT ( 'NONE',  ( -68.00000337463099243, -2.428612866367529932E-14, -5.000000000000000000 ) ) ;
#27830=AXIS2_PLACEMENT_3D ( 'NONE', #34272, #4857, #19286 ) ;
#27831=VECTOR ( 'NONE', #13356, 1000.000000000000000 ) ;
#27832=AXIS2_PLACEMENT_3D ( 'NONE', #31413, #22427, #14546 ) ;
#27833=CARTESIAN_POINT ( 'NONE',  ( 67.99999662536836809, -51.96152422706639840, -9.999999999999998224 ) ) ;
#27834=DIRECTION ( 'NONE',  ( 1.000000000000000000, 0.000000000000000000, 0.000000000000000000 ) ) ;
#27835=ORIENTED_EDGE ( 'NONE', *, *, #36424, .T. ) ;
#27836=DIRECTION ( 'NONE',  ( 0.000000000000000000, 0.000000000000000000, 1.000000000000000000 ) ) ;
#27837=CARTESIAN_POINT ( 'NONE',  ( -50.00000337463109190, 69.28203230275518365, -5.000000000000000000 ) ) ;
#27839=CIRCLE ( 'NONE', #25471, 3.000000000000002665 ) ;
#27841=CARTESIAN_POINT ( 'NONE',  ( 71.99999662536838230, -34.64101615137759183, 12.50000000000000000 ) ) ;
#27842=DIRECTION ( 'NONE',  ( 0.000000000000000000, 0.000000000000000000, 1.000000000000000000 ) ) ;
#27844=CARTESIAN_POINT ( 'NONE',  ( 51.13139720814417899, 27.49999999999988987, -5.000000000000000000 ) ) ;
#27845=AXIS2_PLACEMENT_3D ( 'NONE', #2124, #13371, #32900 ) ;
#27846=DIRECTION ( 'NONE',  ( -1.000000000000000000, 0.000000000000000000, 0.000000000000000000 ) ) ;
#27847=DIRECTION ( 'NONE',  ( 0.000000000000000000, 0.000000000000000000, 1.000000000000000000 ) ) ;
#27848=EDGE_CURVE ( 'NONE', #20167, #8353, #26701, .T. ) ;
#27849=CIRCLE ( 'NONE', #26647, 2.000000000000001776 ) ;
#27850=AXIS2_PLACEMENT_3D ( 'NONE', #16689, #36737, #17031 ) ;
#27851=VERTEX_POINT ( 'NONE', #28314 ) ;
#27853=EDGE_CURVE ( 'NONE', #8974, #5583, #33291, .T. ) ;
#27854=CARTESIAN_POINT ( 'NONE',  ( 66.99999662536839651, 60.62177826491078747, 12.50000000000000000 ) ) ;
#27855=VECTOR ( 'NONE', #3293, 1000.000000000000000 ) ;
#27856=CARTESIAN_POINT ( 'NONE',  ( 46.99999662536849598, -77.94228634059960825, -9.999999999999998224 ) ) ;
#27858=CIRCLE ( 'NONE', #4538, 3.000000000000005773 ) ;
#27859=CARTESIAN_POINT ( 'NONE',  ( -72.00000337463102085, -51.96152422706641971, 12.50000000000000000 ) ) ;
#27862=ORIENTED_EDGE ( 'NONE', *, *, #24288, .T. ) ;
#27863=CARTESIAN_POINT ( 'NONE',  ( 76.99999662536836809, 8.660254037844394404, -9.999999999999998224 ) ) ;
#27865=CARTESIAN_POINT ( 'NONE',  ( 62.99999662536842493, 43.30127018922200222, -9.999999999999998224 ) ) ;
#27867=ORIENTED_EDGE ( 'NONE', *, *, #18213, .T. ) ;
#27869=CARTESIAN_POINT ( 'NONE',  ( 58.88972745734179171, -34.00000000000007105, 12.49999999999999822 ) ) ;
#27870=AXIS2_PLACEMENT_3D ( 'NONE', #36113, #27661, #15864 ) ;
#27871=DIRECTION ( 'NONE',  ( 0.000000000000000000, 0.000000000000000000, 1.000000000000000000 ) ) ;
#27872=ORIENTED_EDGE ( 'NONE', *, *, #31138, .T. ) ;
#27873=EDGE_CURVE ( 'NONE', #34867, #24850, #3862, .T. ) ;
#27874=CIRCLE ( 'NONE', #29035, 2.000000000000001776 ) ;
#27876=ORIENTED_EDGE ( 'NONE', *, *, #25192, .T. ) ;
#27877=CARTESIAN_POINT ( 'NONE',  ( -77.00000337463100664, -43.30127018922202353, -9.999999999999998224 ) ) ;
#27879=AXIS2_PLACEMENT_3D ( 'NONE', #1743, #33619, #36615 ) ;
#27881=AXIS2_PLACEMENT_3D ( 'NONE', #16640, #10991, #5396 ) ;
#27883=DIRECTION ( 'NONE',  ( 0.000000000000000000, 0.000000000000000000, 1.000000000000000000 ) ) ;
#27886=EDGE_CURVE ( 'NONE', #24245, #28829, #13440, .T. ) ;
#27887=CIRCLE ( 'NONE', #11135, 3.499999999999989342 ) ;
#27888=CYLINDRICAL_SURFACE ( 'NONE', #10469, 2.000000000000001776 ) ;
#27889=DIRECTION ( 'NONE',  ( 0.000000000000000000, 0.000000000000000000, 1.000000000000000000 ) ) ;
#27890=DIRECTION ( 'NONE',  ( 0.000000000000000000, 0.000000000000000000, 1.000000000000000000 ) ) ;
#27891=EDGE_CURVE ( 'NONE', #24391, #34954, #3377, .T. ) ;
#27892=EDGE_LOOP ( 'NONE', ( #4206, #7600 ) ) ;
#27894=CARTESIAN_POINT ( 'NONE',  ( 9.999996625368625658, 86.60254037844397601, -5.000000000000000000 ) ) ;
#27895=DIRECTION ( 'NONE',  ( 0.000000000000000000, 0.000000000000000000, 1.000000000000000000 ) ) ;
#27896=AXIS2_PLACEMENT_3D ( 'NONE', #17700, #14903, #23521 ) ;
#27897=ADVANCED_FACE ( 'NONE', ( #924 ), #25881, .F. ) ;
#27898=ORIENTED_EDGE ( 'NONE', *, *, #2290, .F. ) ;
#27900=AXIS2_PLACEMENT_3D ( 'NONE', #34018, #16573, #13930 ) ;
#27901=CYLINDRICAL_SURFACE ( 'NONE', #27497, 2.000000000000001776 ) ;
#27902=EDGE_LOOP ( 'NONE', ( #4247, #8560, #3870, #32575, #1742, #16250 ) ) ;
#27903=AXIS2_PLACEMENT_3D ( 'NONE', #30028, #4349, #7347 ) ;
#27906=DIRECTION ( 'NONE',  ( 0.000000000000000000, 0.000000000000000000, 1.000000000000000000 ) ) ;
#27908=VECTOR ( 'NONE', #11821, 1000.000000000000000 ) ;
#27909=VECTOR ( 'NONE', #2132, 1000.000000000000000 ) ;
#27911=VECTOR ( 'NONE', #26007, 1000.000000000000000 ) ;
#27913=LINE ( 'NONE', #21566, #30191 ) ;
#27914=CYLINDRICAL_SURFACE ( 'NONE', #31646, 3.499999999999996003 ) ;
#27916=CARTESIAN_POINT ( 'NONE',  ( -70.00000337463102085, -34.64101615137762025, 17.49999999999999645 ) ) ;
#27917=CARTESIAN_POINT ( 'NONE',  ( -83.00000337463092137, -25.98076211353322051, 12.50000000000000000 ) ) ;
#27922=DIRECTION ( 'NONE',  ( 0.000000000000000000, 0.000000000000000000, -1.000000000000000000 ) ) ;
#27923=DIRECTION ( 'NONE',  ( 1.000000000000000000, 0.000000000000000000, 0.000000000000000000 ) ) ;
#27924=DIRECTION ( 'NONE',  ( 0.000000000000000000, 0.000000000000000000, 1.000000000000000000 ) ) ;
#27925=ORIENTED_EDGE ( 'NONE', *, *, #1776, .F. ) ;
#27926=AXIS2_PLACEMENT_3D ( 'NONE', #34200, #11479, #8325 ) ;
#27928=CIRCLE ( 'NONE', #33909, 2.000000000000001776 ) ;
#27929=DIRECTION ( 'NONE',  ( 1.000000000000000000, 0.000000000000000000, 0.000000000000000000 ) ) ;
#27931=ORIENTED_EDGE ( 'NONE', *, *, #4989, .T. ) ;
#27933=DIRECTION ( 'NONE',  ( -1.000000000000000000, 0.000000000000000000, 0.000000000000000000 ) ) ;
#27934=ORIENTED_EDGE ( 'NONE', *, *, #36392, .T. ) ;
#27935=AXIS2_PLACEMENT_3D ( 'NONE', #10560, #16759, #13195 ) ;
#27936=CIRCLE ( 'NONE', #11755, 2.000000000000001776 ) ;
#27938=ADVANCED_FACE ( 'NONE', ( #9171 ), #32029, .F. ) ;
#27939=CIRCLE ( 'NONE', #4589, 2.000000000000000000 ) ;
#27941=CIRCLE ( 'NONE', #25569, 2.000000000000000000 ) ;
#27942=DIRECTION ( 'NONE',  ( -1.000000000000000000, 1.130782710266362465E-14, 0.000000000000000000 ) ) ;
#27943=EDGE_CURVE ( 'NONE', #3582, #23793, #18263, .T. ) ;
#27944=ORIENTED_EDGE ( 'NONE', *, *, #20159, .F. ) ;
#27945=ORIENTED_EDGE ( 'NONE', *, *, #27711, .T. ) ;
#27946=VERTEX_POINT ( 'NONE', #17609 ) ;
#27947=VECTOR ( 'NONE', #12005, 1000.000000000000000 ) ;
#27948=ORIENTED_EDGE ( 'NONE', *, *, #27826, .F. ) ;
#27950=CARTESIAN_POINT ( 'NONE',  ( -87.00000337463093558, 25.98076211353317433, -9.999999999999998224 ) ) ;
#27951=CARTESIAN_POINT ( 'NONE',  ( -68.00000337463102085, -51.96152422706641971, -9.999999999999998224 ) ) ;
#27952=DIRECTION ( 'NONE',  ( 0.000000000000000000, 0.000000000000000000, -1.000000000000000000 ) ) ;
#27954=EDGE_LOOP ( 'NONE', ( #23626, #29706 ) ) ;
#27955=DIRECTION ( 'NONE',  ( 1.000000000000000000, 0.000000000000000000, 0.000000000000000000 ) ) ;
#27956=VECTOR ( 'NONE', #10331, 1000.000000000000000 ) ;
#27957=CARTESIAN_POINT ( 'NONE',  ( -3.374631327851540519E-06, 86.60254037844397601, -9.999999999999998224 ) ) ;
#27958=ADVANCED_FACE ( 'NONE', ( #6369 ), #17809, .F. ) ;
#27959=CIRCLE ( 'NONE', #30921, 2.000000000000000000 ) ;
#27960=CIRCLE ( 'NONE', #29161, 33.00000000000001421 ) ;
#27962=FACE_OUTER_BOUND ( 'NONE', #1693, .T. ) ;
#27965=ORIENTED_EDGE ( 'NONE', *, *, #28873, .T. ) ;
#27966=CIRCLE ( 'NONE', #32756, 2.000000000000001776 ) ;
#27967=VERTEX_POINT ( 'NONE', #26433 ) ;
#27968=AXIS2_PLACEMENT_3D ( 'NONE', #16024, #33256, #22203 ) ;
#27969=DIRECTION ( 'NONE',  ( -0.5000000000000101030, -0.8660254037844328234, 0.000000000000000000 ) ) ;
#27970=CYLINDRICAL_SURFACE ( 'NONE', #6128, 1.999999999999998224 ) ;
#27973=ORIENTED_EDGE ( 'NONE', *, *, #6713, .T. ) ;
#27974=ORIENTED_EDGE ( 'NONE', *, *, #2949, .F. ) ;
#27975=CIRCLE ( 'NONE', #36395, 2.000000000000000000 ) ;
#27976=AXIS2_PLACEMENT_3D ( 'NONE', #16750, #7749, #22540 ) ;
#27977=CARTESIAN_POINT ( 'NONE',  ( 19.99999662536857770, 86.60254037844397601, -5.000000000000000000 ) ) ;
#27978=EDGE_CURVE ( 'NONE', #8893, #29771, #9368, .T. ) ;
#27980=EDGE_CURVE ( 'NONE', #9828, #19877, #15007, .T. ) ;
#27981=AXIS2_PLACEMENT_3D ( 'NONE', #33255, #16570, #1940 ) ;
#27983=VERTEX_POINT ( 'NONE', #20260 ) ;
#27984=ORIENTED_EDGE ( 'NONE', *, *, #23567, .T. ) ;
#27985=EDGE_CURVE ( 'NONE', #31670, #8095, #2694, .T. ) ;
#27986=CARTESIAN_POINT ( 'NONE',  ( -72.00000337463100664, -2.404119930384582903E-14, -9.999999999999998224 ) ) ;
#27988=ORIENTED_EDGE ( 'NONE', *, *, #24016, .F. ) ;
#27989=ORIENTED_EDGE ( 'NONE', *, *, #35094, .T. ) ;
#27990=EDGE_CURVE ( 'NONE', #34413, #666, #31430, .T. ) ;
#27992=FACE_OUTER_BOUND ( 'NONE', #22028, .T. ) ;
#27996=DIRECTION ( 'NONE',  ( 0.000000000000000000, 0.000000000000000000, 1.000000000000000000 ) ) ;
#27997=AXIS2_PLACEMENT_3D ( 'NONE', #19006, #24636, #33057 ) ;
#27999=CARTESIAN_POINT ( 'NONE',  ( -62.97617850287781494, -4.279621169095772615, 12.49999999999999822 ) ) ;
#28000=FACE_BOUND ( 'NONE', #10804, .T. ) ;
#28002=DIRECTION ( 'NONE',  ( -1.000000000000000000, 0.000000000000000000, 0.000000000000000000 ) ) ;
#28003=CIRCLE ( 'NONE', #17827, 95.00000000000000000 ) ;
#28004=DIRECTION ( 'NONE',  ( -1.000000000000000000, 0.000000000000000000, -0.000000000000000000 ) ) ;
#28005=EDGE_CURVE ( 'NONE', #10047, #29027, #2099, .T. ) ;
#28006=PLANE ( 'NONE',  #5140 ) ;
#28007=ADVANCED_FACE ( 'NONE', ( #20433 ), #6181, .F. ) ;
#28008=CARTESIAN_POINT ( 'NONE',  ( -67.00000337463104927, -43.30127018922202353, -9.999999999999998224 ) ) ;
#28009=ADVANCED_FACE ( 'NONE', ( #5830 ), #6738, .T. ) ;
#28010=CIRCLE ( 'NONE', #11823, 2.000000000000001776 ) ;
#28011=EDGE_CURVE ( 'NONE', #20792, #22677, #32603, .T. ) ;
#28012=CARTESIAN_POINT ( 'NONE',  ( -56.74224907228983028, 68.66839587347264739, -49.22241343995295892 ) ) ;
#28013=ORIENTED_EDGE ( 'NONE', *, *, #8040, .T. ) ;
#28015=AXIS2_PLACEMENT_3D ( 'NONE', #10888, #27593, #10334 ) ;
#28016=CYLINDRICAL_SURFACE ( 'NONE', #26707, 2.000000000000001776 ) ;
#28017=LINE ( 'NONE', #33471, #16348 ) ;
#28019=ORIENTED_EDGE ( 'NONE', *, *, #17202, .F. ) ;
#28022=PLANE ( 'NONE',  #20149 ) ;
#28023=CARTESIAN_POINT ( 'NONE',  ( -65.00000337463102085, 25.98076211353317433, -9.999999999999998224 ) ) ;
#28025=VECTOR ( 'NONE', #34002, 1000.000000000000000 ) ;
#28026=DIRECTION ( 'NONE',  ( 0.000000000000000000, 0.000000000000000000, -1.000000000000000000 ) ) ;
#28027=DIRECTION ( 'NONE',  ( 1.000000000000000000, 0.000000000000000000, 0.000000000000000000 ) ) ;
#28028=ORIENTED_EDGE ( 'NONE', *, *, #16249, .T. ) ;
#28030=ORIENTED_EDGE ( 'NONE', *, *, #9403, .F. ) ;
#28031=DIRECTION ( 'NONE',  ( 1.000000000000000000, 0.000000000000000000, 0.000000000000000000 ) ) ;
#28032=CIRCLE ( 'NONE', #1102, 2.000000000000001776 ) ;
#28033=CARTESIAN_POINT ( 'NONE',  ( 68.19171716056558807, -52.81599796988855644, -5.000000000000000000 ) ) ;
#28034=LINE ( 'NONE', #8703, #4046 ) ;
#28035=VECTOR ( 'NONE', #12377, 1000.000000000000000 ) ;
#28036=ORIENTED_EDGE ( 'NONE', *, *, #5531, .T. ) ;
#28037=LINE ( 'NONE', #16963, #6298 ) ;
#28038=AXIS2_PLACEMENT_3D ( 'NONE', #28856, #25712, #22711 ) ;
#28039=AXIS2_PLACEMENT_3D ( 'NONE', #22610, #16424, #34062 ) ;
#28040=DIRECTION ( 'NONE',  ( -1.000000000000000000, 0.000000000000000000, 0.000000000000000000 ) ) ;
#28041=DIRECTION ( 'NONE',  ( 1.000000000000000000, 0.000000000000000000, 0.000000000000000000 ) ) ;
#28042=CIRCLE ( 'NONE', #7683, 65.00000000000000000 ) ;
#28045=DIRECTION ( 'NONE',  ( 0.000000000000000000, 0.000000000000000000, 1.000000000000000000 ) ) ;
#28046=ORIENTED_EDGE ( 'NONE', *, *, #12860, .F. ) ;
#28047=CARTESIAN_POINT ( 'NONE',  ( -67.00000337463104927, -25.98076211353322051, -5.000000000000000000 ) ) ;
#28048=DIRECTION ( 'NONE',  ( 0.000000000000000000, 0.000000000000000000, -1.000000000000000000 ) ) ;
#28049=CARTESIAN_POINT ( 'NONE',  ( -27.78182860042817026, -56.67878100130359087, 12.49999999999999822 ) ) ;
#28050=AXIS2_PLACEMENT_3D ( 'NONE', #20618, #24189, #1316 ) ;
#28051=DIRECTION ( 'NONE',  ( 0.000000000000000000, 0.000000000000000000, 1.000000000000000000 ) ) ;
#28052=VECTOR ( 'NONE', #35521, 1000.000000000000000 ) ;
#28053=EDGE_LOOP ( 'NONE', ( #36775, #33523, #26192, #13939, #32306 ) ) ;
#28054=ADVANCED_FACE ( 'NONE', ( #15740 ), #29799, .F. ) ;
#28055=EDGE_LOOP ( 'NONE', ( #20028, #34076 ) ) ;
#28057=CIRCLE ( 'NONE', #26263, 2.000000000000001776 ) ;
#28058=CYLINDRICAL_SURFACE ( 'NONE', #19985, 2.000000000000000000 ) ;
#28059=CARTESIAN_POINT ( 'NONE',  ( -10.00000337463125000, -86.60254037844400443, -9.999999999999998224 ) ) ;
#28061=ORIENTED_EDGE ( 'NONE', *, *, #36460, .T. ) ;
#28062=CIRCLE ( 'NONE', #2918, 2.000000000000001776 ) ;
#28063=LINE ( 'NONE', #13820, #24215 ) ;
#28064=DIRECTION ( 'NONE',  ( 0.000000000000000000, 0.000000000000000000, 1.000000000000000000 ) ) ;
#28065=AXIS2_PLACEMENT_3D ( 'NONE', #29881, #16203, #21447 ) ;
#28066=LINE ( 'NONE', #25820, #28420 ) ;
#28067=ORIENTED_EDGE ( 'NONE', *, *, #25381, .T. ) ;
#28068=EDGE_LOOP ( 'NONE', ( #32110, #26573, #35347, #28393 ) ) ;
#28069=DIRECTION ( 'NONE',  ( 0.000000000000000000, 0.000000000000000000, 1.000000000000000000 ) ) ;
#28070=CIRCLE ( 'NONE', #6502, 33.00000000000001421 ) ;
#28071=CARTESIAN_POINT ( 'NONE',  ( 14.99999662536863632, -77.94228634059960825, 17.49999999999999645 ) ) ;
#28072=VERTEX_POINT ( 'NONE', #18171 ) ;
#28074=DIRECTION ( 'NONE',  ( 0.000000000000000000, 0.000000000000000000, 1.000000000000000000 ) ) ;
#28076=FACE_BOUND ( 'NONE', #33225, .T. ) ;
#28077=EDGE_CURVE ( 'NONE', #24891, #33006, #24006, .T. ) ;
#28078=AXIS2_PLACEMENT_3D ( 'NONE', #18145, #9893, #12692 ) ;
#28079=EDGE_CURVE ( 'NONE', #13800, #68, #6862, .T. ) ;
#28080=CIRCLE ( 'NONE', #18928, 2.000000000000000000 ) ;
#28081=AXIS2_PLACEMENT_3D ( 'NONE', #24544, #30694, #10839 ) ;
#28082=DIRECTION ( 'NONE',  ( 0.000000000000000000, 0.000000000000000000, -1.000000000000000000 ) ) ;
#28085=CYLINDRICAL_SURFACE ( 'NONE', #35639, 2.000000000000001776 ) ;
#28086=EDGE_CURVE ( 'NONE', #30390, #26110, #15867, .T. ) ;
#28087=VECTOR ( 'NONE', #6909, 1000.000000000000000 ) ;
#28090=ORIENTED_EDGE ( 'NONE', *, *, #30468, .F. ) ;
#28093=CARTESIAN_POINT ( 'NONE',  ( 4.279621169095998212, -62.97617850287780072, -49.86561046011506448 ) ) ;
#28094=DIRECTION ( 'NONE',  ( 0.000000000000000000, 0.000000000000000000, -1.000000000000000000 ) ) ;
#28095=ORIENTED_EDGE ( 'NONE', *, *, #16952, .F. ) ;
#28097=VECTOR ( 'NONE', #18670, 1000.000000000000000 ) ;
#28098=EDGE_CURVE ( 'NONE', #35279, #27267, #14644, .T. ) ;
#28099=DIRECTION ( 'NONE',  ( 1.000000000000000000, 0.000000000000000000, 0.000000000000000000 ) ) ;
#28100=ORIENTED_EDGE ( 'NONE', *, *, #6322, .F. ) ;
#28101=LINE ( 'NONE', #9090, #21125 ) ;
#28102=CARTESIAN_POINT ( 'NONE',  ( -10.00000337463125000, -86.60254037844400443, 17.49999999999999645 ) ) ;
#28103=AXIS2_PLACEMENT_3D ( 'NONE', #13436, #5011, #10447 ) ;
#28105=CIRCLE ( 'NONE', #5352, 2.000000000000000000 ) ;
#28106=CARTESIAN_POINT ( 'NONE',  ( -62.97617850287781494, -4.279621169095772615, 12.49999999999999822 ) ) ;
#28109=DIRECTION ( 'NONE',  ( 1.000000000000000000, 0.000000000000000000, 0.000000000000000000 ) ) ;
#28110=CARTESIAN_POINT ( 'NONE',  ( -85.00000337463092137, -8.660254037844422825, 17.49999999999999645 ) ) ;
#28111=CARTESIAN_POINT ( 'NONE',  ( -73.00000337463099243, -25.98076211353322051, 17.49999999999999645 ) ) ;
#28112=EDGE_LOOP ( 'NONE', ( #11978, #15406 ) ) ;
#28113=EDGE_LOOP ( 'NONE', ( #6921, #12799, #31799, #21153, #34228, #4018 ) ) ;
#28114=AXIS2_PLACEMENT_3D ( 'NONE', #23953, #32940, #20739 ) ;
#28116=CARTESIAN_POINT ( 'NONE',  ( 52.39915983220795681, 35.19434990244919703, -4.999999999999997335 ) ) ;
#28117=CARTESIAN_POINT ( 'NONE',  ( 44.99999662536851019, -60.62177826491080168, 17.49999999999999645 ) ) ;
#28118=CARTESIAN_POINT ( 'NONE',  ( -70.00000337463099243, 51.96152422706637708, 17.49999999999999645 ) ) ;
#28119=EDGE_LOOP ( 'NONE', ( #17492, #26914 ) ) ;
#28120=CIRCLE ( 'NONE', #18550, 95.00000000000000000 ) ;
#28121=CARTESIAN_POINT ( 'NONE',  ( 74.99999662536835388, -25.98076211353319565, -9.999999999999998224 ) ) ;
#28123=ORIENTED_EDGE ( 'NONE', *, *, #8414, .T. ) ;
#28125=CARTESIAN_POINT ( 'NONE',  ( -83.00000337463092137, 25.98076211353317433, 12.50000000000000000 ) ) ;
#28126=ORIENTED_EDGE ( 'NONE', *, *, #9309, .F. ) ;
#28127=AXIS2_PLACEMENT_3D ( 'NONE', #28379, #36831, #34392 ) ;
#28129=CARTESIAN_POINT ( 'NONE',  ( 47.63139720814400846, -27.50000000000022737, -10.00000000000000178 ) ) ;
#28130=CARTESIAN_POINT ( 'NONE',  ( -70.00000337463099243, -2.428612866367529932E-14, 12.50000000000000000 ) ) ;
#28132=ADVANCED_FACE ( 'NONE', ( #1478 ), #9738, .F. ) ;
#28133=DIRECTION ( 'NONE',  ( 0.000000000000000000, 0.000000000000000000, 1.000000000000000000 ) ) ;
#28134=CIRCLE ( 'NONE', #17963, 2.000000000000001776 ) ;
#28135=VERTEX_POINT ( 'NONE', #27361 ) ;
#28136=ORIENTED_EDGE ( 'NONE', *, *, #15171, .F. ) ;
#28137=AXIS2_PLACEMENT_3D ( 'NONE', #35107, #12952, #18606 ) ;
#28138=ORIENTED_EDGE ( 'NONE', *, *, #31170, .T. ) ;
#28140=VERTEX_POINT ( 'NONE', #21367 ) ;
#28141=DIRECTION ( 'NONE',  ( 1.000000000000000000, 0.000000000000000000, 0.000000000000000000 ) ) ;
#28142=CIRCLE ( 'NONE', #34155, 2.000000000000001776 ) ;
#28143=DIRECTION ( 'NONE',  ( 0.000000000000000000, 0.000000000000000000, 1.000000000000000000 ) ) ;
#28144=VECTOR ( 'NONE', #32939, 1000.000000000000000 ) ;
#28145=DIRECTION ( 'NONE',  ( 0.000000000000000000, 0.000000000000000000, -1.000000000000000000 ) ) ;
#28148=EDGE_LOOP ( 'NONE', ( #16714, #7127 ) ) ;
#28149=FACE_OUTER_BOUND ( 'NONE', #23633, .T. ) ;
#28151=DIRECTION ( 'NONE',  ( 0.000000000000000000, 0.000000000000000000, 1.000000000000000000 ) ) ;
#28152=CARTESIAN_POINT ( 'NONE',  ( -76.71706625813334313, 9.685775882613420151, 12.50000000000000000 ) ) ;
#28153=ORIENTED_EDGE ( 'NONE', *, *, #21585, .F. ) ;
#28154=CARTESIAN_POINT ( 'NONE',  ( -45.00000337463112743, -60.62177826491080168, -9.999999999999998224 ) ) ;
#28155=DIRECTION ( 'NONE',  ( 1.000000000000000000, 0.000000000000000000, 0.000000000000000000 ) ) ;
#28156=CIRCLE ( 'NONE', #5420, 2.000000000000001776 ) ;
#28157=ORIENTED_EDGE ( 'NONE', *, *, #7828, .F. ) ;
#28159=VERTEX_POINT ( 'NONE', #24572 ) ;
#28160=DIRECTION ( 'NONE',  ( 1.000000000000000000, 0.000000000000000000, 0.000000000000000000 ) ) ;
#28161=EDGE_CURVE ( 'NONE', #34663, #5470, #36004, .T. ) ;
#28162=DIRECTION ( 'NONE',  ( 0.000000000000000000, 0.000000000000000000, -1.000000000000000000 ) ) ;
#28163=AXIS2_PLACEMENT_3D ( 'NONE', #8286, #19341, #19715 ) ;
#28164=CARTESIAN_POINT ( 'NONE',  ( -77.00000337463097821, 8.660254037844374864, -9.999999999999998224 ) ) ;
#28166=VERTEX_POINT ( 'NONE', #9297 ) ;
#28169=DIRECTION ( 'NONE',  ( 1.000000000000000000, 0.000000000000000000, 0.000000000000000000 ) ) ;
#28170=ORIENTED_EDGE ( 'NONE', *, *, #35356, .F. ) ;
#28171=FACE_OUTER_BOUND ( 'NONE', #15116, .T. ) ;
#28174=EDGE_CURVE ( 'NONE', #6836, #34930, #5075, .T. ) ;
#28175=FACE_OUTER_BOUND ( 'NONE', #14135, .T. ) ;
#28177=ORIENTED_EDGE ( 'NONE', *, *, #19763, .F. ) ;
#28179=DIRECTION ( 'NONE',  ( 0.000000000000000000, 0.000000000000000000, 1.000000000000000000 ) ) ;
#28180=CARTESIAN_POINT ( 'NONE',  ( 46.99999662536851019, -60.62177826491080168, -9.999999999999998224 ) ) ;
#28182=ORIENTED_EDGE ( 'NONE', *, *, #415, .T. ) ;
#28183=CARTESIAN_POINT ( 'NONE',  ( 1.999996625368696490, -86.60254037844400443, 12.50000000000000000 ) ) ;
#28184=AXIS2_PLACEMENT_3D ( 'NONE', #18003, #4134, #29427 ) ;
#28185=FACE_BOUND ( 'NONE', #32556, .T. ) ;
#28189=DIRECTION ( 'NONE',  ( 0.000000000000000000, 0.000000000000000000, 1.000000000000000000 ) ) ;
#28191=CARTESIAN_POINT ( 'NONE',  ( -46.74666114985175369, -61.59604035298635694, 12.50000000000000000 ) ) ;
#28192=DIRECTION ( 'NONE',  ( 0.000000000000000000, 0.000000000000000000, 1.000000000000000000 ) ) ;
#28193=ORIENTED_EDGE ( 'NONE', *, *, #3325, .F. ) ;
#28194=ADVANCED_FACE ( 'NONE', ( #3515 ), #15300, .F. ) ;
#28195=DIRECTION ( 'NONE',  ( 0.000000000000000000, 0.000000000000000000, 1.000000000000000000 ) ) ;
#28196=DIRECTION ( 'NONE',  ( -0.8660254037844449249, -0.4999999999999888978, 0.000000000000000000 ) ) ;
#28197=DIRECTION ( 'NONE',  ( 1.000000000000000000, 0.000000000000000000, 0.000000000000000000 ) ) ;
#28198=VERTEX_POINT ( 'NONE', #12483 ) ;
#28199=EDGE_CURVE ( 'NONE', #36258, #35811, #29371, .T. ) ;
#28200=EDGE_LOOP ( 'NONE', ( #36408, #17125, #24732 ) ) ;
#28201=ORIENTED_EDGE ( 'NONE', *, *, #5521, .F. ) ;
#28202=DIRECTION ( 'NONE',  ( -1.000000000000000000, 0.000000000000000000, 0.000000000000000000 ) ) ;
#28203=CARTESIAN_POINT ( 'NONE',  ( -77.00000337463100664, -43.30127018922202353, 17.49999999999999645 ) ) ;
#28204=EDGE_CURVE ( 'NONE', #15127, #36972, #21111, .T. ) ;
#28206=EDGE_CURVE ( 'NONE', #29785, #25826, #33229, .T. ) ;
#28208=CARTESIAN_POINT ( 'NONE',  ( 17.14523346298344109, -93.36492675454773860, -4.999999999999997335 ) ) ;
#28209=ORIENTED_EDGE ( 'NONE', *, *, #26511, .F. ) ;
#28210=AXIS2_PLACEMENT_3D ( 'NONE', #30118, #35415, #32191 ) ;
#28211=FACE_OUTER_BOUND ( 'NONE', #7009, .T. ) ;
#28212=VERTEX_POINT ( 'NONE', #5959 ) ;
#28213=CARTESIAN_POINT ( 'NONE',  ( -77.00000337463097821, 8.660254037844374864, -9.999999999999998224 ) ) ;
#28214=EDGE_CURVE ( 'NONE', #21455, #12472, #11739, .T. ) ;
#28215=ORIENTED_EDGE ( 'NONE', *, *, #18805, .T. ) ;
#28217=DIRECTION ( 'NONE',  ( -1.000000000000000000, 0.000000000000000000, 0.000000000000000000 ) ) ;
#28218=DIRECTION ( 'NONE',  ( 0.000000000000000000, 0.000000000000000000, 1.000000000000000000 ) ) ;
#28219=EDGE_CURVE ( 'NONE', #4119, #26898, #21856, .T. ) ;
#28220=ADVANCED_FACE ( 'NONE', ( #35200 ), #20939, .F. ) ;
#28221=EDGE_CURVE ( 'NONE', #14572, #2310, #17945, .T. ) ;
#28226=DIRECTION ( 'NONE',  ( 0.000000000000000000, 0.000000000000000000, 1.000000000000000000 ) ) ;
#28228=DIRECTION ( 'NONE',  ( 0.000000000000000000, 0.000000000000000000, 1.000000000000000000 ) ) ;
#28229=DIRECTION ( 'NONE',  ( 1.000000000000000000, 0.000000000000000000, 0.000000000000000000 ) ) ;
#28232=AXIS2_PLACEMENT_3D ( 'NONE', #13133, #24753, #19146 ) ;
#28233=DIRECTION ( 'NONE',  ( 0.000000000000000000, 0.000000000000000000, 1.000000000000000000 ) ) ;
#28234=PLANE ( 'NONE',  #33951 ) ;
#28235=DIRECTION ( 'NONE',  ( -1.000000000000000000, 0.000000000000000000, 0.000000000000000000 ) ) ;
#28238=DIRECTION ( 'NONE',  ( 0.000000000000000000, 0.000000000000000000, 1.000000000000000000 ) ) ;
#28239=CARTESIAN_POINT ( 'NONE',  ( -53.00000337463110611, -43.30127018922202353, -5.000000000000000000 ) ) ;
#28240=ORIENTED_EDGE ( 'NONE', *, *, #32607, .F. ) ;
#28242=CARTESIAN_POINT ( 'NONE',  ( 0.000000000000000000, 0.000000000000000000, -5.000000000000000000 ) ) ;
#28244=CARTESIAN_POINT ( 'NONE',  ( -57.00000337463109901, -60.62177826491083010, 12.50000000000000000 ) ) ;
#28245=ORIENTED_EDGE ( 'NONE', *, *, #489, .T. ) ;
#28247=DIRECTION ( 'NONE',  ( 0.000000000000000000, 0.000000000000000000, -1.000000000000000000 ) ) ;
#28248=VECTOR ( 'NONE', #5124, 1000.000000000000000 ) ;
#28249=CARTESIAN_POINT ( 'NONE',  ( 69.99999662536838230, -34.64101615137759183, -5.000000000000000000 ) ) ;
#28250=EDGE_LOOP ( 'NONE', ( #33269, #6203, #34234, #15711 ) ) ;
#28251=DIRECTION ( 'NONE',  ( -0.000000000000000000, -0.000000000000000000, 1.000000000000000000 ) ) ;
#28252=ORIENTED_EDGE ( 'NONE', *, *, #241, .F. ) ;
#28253=AXIS2_PLACEMENT_3D ( 'NONE', #13902, #30, #17286 ) ;
#28254=FACE_BOUND ( 'NONE', #8465, .T. ) ;
#28255=EDGE_CURVE ( 'NONE', #25448, #20697, #8685, .T. ) ;
#28258=EDGE_CURVE ( 'NONE', #12074, #24619, #860, .T. ) ;
#28259=ORIENTED_EDGE ( 'NONE', *, *, #10564, .T. ) ;
#28262=DIRECTION ( 'NONE',  ( 0.000000000000000000, 0.000000000000000000, 1.000000000000000000 ) ) ;
#28263=DIRECTION ( 'NONE',  ( 0.000000000000000000, 0.000000000000000000, -1.000000000000000000 ) ) ;
#28264=ORIENTED_EDGE ( 'NONE', *, *, #35692, .T. ) ;
#28265=CARTESIAN_POINT ( 'NONE',  ( 36.99999662536855283, -77.94228634059960825, 17.49999999999999645 ) ) ;
#28266=CYLINDRICAL_SURFACE ( 'NONE', #20806, 2.000000000000001776 ) ;
#28267=CARTESIAN_POINT ( 'NONE',  ( -55.00000337463107059, 60.62177826491078747, -5.000000000000000000 ) ) ;
#28268=ORIENTED_EDGE ( 'NONE', *, *, #35479, .F. ) ;
#28271=ORIENTED_EDGE ( 'NONE', *, *, #22400, .T. ) ;
#28272=CARTESIAN_POINT ( 'NONE',  ( 58.88972745734179171, -34.00000000000007105, 12.49999999999999822 ) ) ;
#28273=DIRECTION ( 'NONE',  ( 0.000000000000000000, 0.000000000000000000, 1.000000000000000000 ) ) ;
#28274=EDGE_CURVE ( 'NONE', #29492, #31614, #9114, .T. ) ;
#28275=CARTESIAN_POINT ( 'NONE',  ( 4.999996625368676284, -77.94228634059960825, -9.999999999999998224 ) ) ;
#28277=DIRECTION ( 'NONE',  ( 0.000000000000000000, 0.000000000000000000, -1.000000000000000000 ) ) ;
#28279=CARTESIAN_POINT ( 'NONE',  ( 34.99999662536855283, 60.62177826491078747, -9.999999999999998224 ) ) ;
#28281=ORIENTED_EDGE ( 'NONE', *, *, #13286, .F. ) ;
#28282=ORIENTED_EDGE ( 'NONE', *, *, #2668, .T. ) ;
#28283=CIRCLE ( 'NONE', #28861, 2.000000000000001776 ) ;
#28286=DIRECTION ( 'NONE',  ( 0.000000000000000000, 0.000000000000000000, -1.000000000000000000 ) ) ;
#28287=CYLINDRICAL_SURFACE ( 'NONE', #12039, 2.000000000000001776 ) ;
#28288=CYLINDRICAL_SURFACE ( 'NONE', #11898, 2.000000000000001776 ) ;
#28289=ORIENTED_EDGE ( 'NONE', *, *, #22021, .T. ) ;
#28290=DIRECTION ( 'NONE',  ( 1.000000000000000000, 0.000000000000000000, 0.000000000000000000 ) ) ;
#28291=ORIENTED_EDGE ( 'NONE', *, *, #16334, .F. ) ;
#28292=VECTOR ( 'NONE', #21769, 1000.000000000000000 ) ;
#28296=ORIENTED_EDGE ( 'NONE', *, *, #17980, .F. ) ;
#28297=DIRECTION ( 'NONE',  ( 1.000000000000000000, 0.000000000000000000, 0.000000000000000000 ) ) ;
#28299=CARTESIAN_POINT ( 'NONE',  ( 84.99999662536832545, 25.98076211353319565, 17.49999999999999645 ) ) ;
#28300=EDGE_LOOP ( 'NONE', ( #163, #675, #16078, #16849 ) ) ;
#28302=ORIENTED_EDGE ( 'NONE', *, *, #33101, .T. ) ;
#28303=EDGE_LOOP ( 'NONE', ( #20636, #17148, #29416, #3936, #5458, #28703 ) ) ;
#28304=AXIS2_PLACEMENT_3D ( 'NONE', #17285, #9380, #6580 ) ;
#28306=DIRECTION ( 'NONE',  ( 0.000000000000000000, 0.000000000000000000, -1.000000000000000000 ) ) ;
#28307=EDGE_CURVE ( 'NONE', #24720, #18017, #36823, .T. ) ;
#28308=CARTESIAN_POINT ( 'NONE',  ( 69.99999662536838230, -51.96152422706639840, 12.50000000000000000 ) ) ;
#28309=CARTESIAN_POINT ( 'NONE',  ( 0.000000000000000000, 0.000000000000000000, 12.49999999999999822 ) ) ;
#28310=DIRECTION ( 'NONE',  ( 1.000000000000000000, 0.000000000000000000, 0.000000000000000000 ) ) ;
#28311=CARTESIAN_POINT ( 'NONE',  ( 36.99999662536855283, -77.94228634059960825, -9.999999999999998224 ) ) ;
#28313=EDGE_LOOP ( 'NONE', ( #32961, #13774 ) ) ;
#28314=CARTESIAN_POINT ( 'NONE',  ( 51.13139720814399425, -27.50000000000022737, -5.000000000000000000 ) ) ;
#28315=CARTESIAN_POINT ( 'NONE',  ( 46.99999662536849598, 60.62177826491077326, -9.999999999999998224 ) ) ;
#28316=AXIS2_PLACEMENT_3D ( 'NONE', #23531, #34113, #8418 ) ;
#28319=CARTESIAN_POINT ( 'NONE',  ( 0.000000000000000000, 0.000000000000000000, 17.49999999999999645 ) ) ;
#28321=CARTESIAN_POINT ( 'NONE',  ( 34.60911832077664485, -75.98085468209112037, 12.50000000000000000 ) ) ;
#28322=VERTEX_POINT ( 'NONE', #7247 ) ;
#28323=ORIENTED_EDGE ( 'NONE', *, *, #12407, .T. ) ;
#28324=ADVANCED_FACE ( 'NONE', ( #35566 ), #27286, .T. ) ;
#28326=CARTESIAN_POINT ( 'NONE',  ( 66.99999662536841072, 25.98076211353318854, -9.999999999999998224 ) ) ;
#28327=DIRECTION ( 'NONE',  ( 0.000000000000000000, 0.000000000000000000, 1.000000000000000000 ) ) ;
#28329=ORIENTED_EDGE ( 'NONE', *, *, #2301, .F. ) ;
#28330=ORIENTED_EDGE ( 'NONE', *, *, #27736, .F. ) ;
#28331=CIRCLE ( 'NONE', #3787, 2.000000000000001776 ) ;
#28333=CIRCLE ( 'NONE', #18769, 27.00000000000001421 ) ;
#28335=EDGE_CURVE ( 'NONE', #17344, #30803, #11088, .T. ) ;
#28336=CARTESIAN_POINT ( 'NONE',  ( 46.74665512060159500, 61.59603906214631763, -5.000000000000000000 ) ) ;
#28338=DIRECTION ( 'NONE',  ( 0.000000000000000000, 0.000000000000000000, 1.000000000000000000 ) ) ;
#28341=AXIS2_PLACEMENT_3D ( 'NONE', #34758, #225, #17485 ) ;
#28342=CARTESIAN_POINT ( 'NONE',  ( -62.00000337463108480, -51.96152422706641971, -9.999999999999998224 ) ) ;
#28343=VERTEX_POINT ( 'NONE', #21852 ) ;
#28344=ORIENTED_EDGE ( 'NONE', *, *, #14907, .T. ) ;
#28345=DIRECTION ( 'NONE',  ( 1.000000000000000000, 0.000000000000000000, 0.000000000000000000 ) ) ;
#28346=CYLINDRICAL_SURFACE ( 'NONE', #36447, 2.000000000000001776 ) ;
#28347=CIRCLE ( 'NONE', #810, 2.000000000000001776 ) ;
#28350=DIRECTION ( 'NONE',  ( 0.000000000000000000, 0.000000000000000000, -1.000000000000000000 ) ) ;
#28352=DIRECTION ( 'NONE',  ( 0.8660254037844415942, 0.4999999999999949485, 0.000000000000000000 ) ) ;
#28353=ADVANCED_FACE ( 'NONE', ( #10411 ), #24682, .F. ) ;
#28354=FACE_BOUND ( 'NONE', #3143, .T. ) ;
#28355=DIRECTION ( 'NONE',  ( 1.000000000000000000, 0.000000000000000000, 0.000000000000000000 ) ) ;
#28357=CARTESIAN_POINT ( 'NONE',  ( -60.00000337463107059, -34.64101615137762025, 12.50000000000000000 ) ) ;
#28358=DIRECTION ( 'NONE',  ( -1.000000000000000000, 0.000000000000000000, 0.000000000000000000 ) ) ;
#28359=DIRECTION ( 'NONE',  ( -0.000000000000000000, -0.000000000000000000, 1.000000000000000000 ) ) ;
#28360=AXIS2_PLACEMENT_3D ( 'NONE', #24702, #32955, #12683 ) ;
#28363=ORIENTED_EDGE ( 'NONE', *, *, #2482, .F. ) ;
#28364=CARTESIAN_POINT ( 'NONE',  ( 41.99999662536853151, -69.28203230275519786, 12.50000000000000000 ) ) ;
#28365=EDGE_CURVE ( 'NONE', #28166, #13878, #4520, .T. ) ;
#28366=DIRECTION ( 'NONE',  ( -1.000000000000000000, 0.000000000000000000, 0.000000000000000000 ) ) ;
#28367=DIRECTION ( 'NONE',  ( 1.000000000000000000, 0.000000000000000000, 0.000000000000000000 ) ) ;
#28370=EDGE_LOOP ( 'NONE', ( #3668, #2640 ) ) ;
#28374=DIRECTION ( 'NONE',  ( 0.000000000000000000, 0.000000000000000000, 1.000000000000000000 ) ) ;
#28375=DIRECTION ( 'NONE',  ( 0.000000000000000000, 0.000000000000000000, 1.000000000000000000 ) ) ;
#28377=CARTESIAN_POINT ( 'NONE',  ( 22.99999662536857059, 77.94228634059957983, 12.50000000000000000 ) ) ;
#28378=ORIENTED_EDGE ( 'NONE', *, *, #367, .T. ) ;
#28379=CARTESIAN_POINT ( 'NONE',  ( -25.00000337463121980, -77.94228634059963667, -9.999999999999998224 ) ) ;
#28380=VERTEX_POINT ( 'NONE', #21295 ) ;
#28381=CARTESIAN_POINT ( 'NONE',  ( 54.99999662536844625, 60.62177826491077326, 12.50000000000000000 ) ) ;
#28382=ORIENTED_EDGE ( 'NONE', *, *, #20823, .T. ) ;
#28383=ORIENTED_EDGE ( 'NONE', *, *, #11951, .F. ) ;
#28384=CIRCLE ( 'NONE', #20016, 2.000000000000001776 ) ;
#28385=EDGE_CURVE ( 'NONE', #16153, #20325, #3303, .T. ) ;
#28387=CARTESIAN_POINT ( 'NONE',  ( 77.99999662536832545, -17.32050807568879591, -9.999999999999998224 ) ) ;
#28388=ORIENTED_EDGE ( 'NONE', *, *, #24241, .F. ) ;
#28389=DIRECTION ( 'NONE',  ( 0.000000000000000000, 0.000000000000000000, 1.000000000000000000 ) ) ;
#28390=EDGE_CURVE ( 'NONE', #30085, #21337, #3914, .T. ) ;
#28392=DIRECTION ( 'NONE',  ( 1.000000000000000000, 0.000000000000000000, 0.000000000000000000 ) ) ;
#28393=ORIENTED_EDGE ( 'NONE', *, *, #3278, .F. ) ;
#28395=CARTESIAN_POINT ( 'NONE',  ( 0.000000000000000000, 0.000000000000000000, -5.000000000000000000 ) ) ;
#28396=ADVANCED_FACE ( 'NONE', ( #4426 ), #27102, .F. ) ;
#28397=VERTEX_POINT ( 'NONE', #19061 ) ;
#28400=EDGE_CURVE ( 'NONE', #24755, #28819, #17091, .T. ) ;
#28401=DIRECTION ( 'NONE',  ( 3.491481338843135327E-15, 1.000000000000000000, 0.000000000000000000 ) ) ;
#28402=CYLINDRICAL_SURFACE ( 'NONE', #35769, 2.000000000000001776 ) ;
#28403=LINE ( 'NONE', #2729, #9273 ) ;
#28405=ORIENTED_EDGE ( 'NONE', *, *, #29821, .T. ) ;
#28406=CIRCLE ( 'NONE', #2071, 1.999999999999998224 ) ;
#28408=DIRECTION ( 'NONE',  ( -0.000000000000000000, -0.000000000000000000, 1.000000000000000000 ) ) ;
#28410=ORIENTED_EDGE ( 'NONE', *, *, #7868, .T. ) ;
#28411=ORIENTED_EDGE ( 'NONE', *, *, #9951, .F. ) ;
#28412=EDGE_CURVE ( 'NONE', #7932, #30738, #19476, .T. ) ;
#28413=DIRECTION ( 'NONE',  ( 0.000000000000000000, 0.000000000000000000, 1.000000000000000000 ) ) ;
#28414=CARTESIAN_POINT ( 'NONE',  ( -35.00000337463116296, -60.62177826491080168, 12.50000000000000000 ) ) ;
#28415=CARTESIAN_POINT ( 'NONE',  ( -67.00000337463102085, 60.62177826491077326, -9.999999999999998224 ) ) ;
#28416=ORIENTED_EDGE ( 'NONE', *, *, #4809, .F. ) ;
#28417=CIRCLE ( 'NONE', #18880, 27.00000000000001421 ) ;
#28418=AXIS2_PLACEMENT_3D ( 'NONE', #9719, #7284, #32581 ) ;
#28420=VECTOR ( 'NONE', #34081, 1000.000000000000000 ) ;
#28421=CARTESIAN_POINT ( 'NONE',  ( 54.99999662536844625, -60.62177826491080168, 17.49999999999999645 ) ) ;
#28422=CIRCLE ( 'NONE', #33219, 2.000000000000001776 ) ;
#28423=DIRECTION ( 'NONE',  ( -1.000000000000000000, 0.000000000000000000, 0.000000000000000000 ) ) ;
#28424=EDGE_LOOP ( 'NONE', ( #27444, #4003 ) ) ;
#28425=DIRECTION ( 'NONE',  ( 0.000000000000000000, 0.000000000000000000, -1.000000000000000000 ) ) ;
#28426=EDGE_LOOP ( 'NONE', ( #6078, #24783 ) ) ;
#28427=CARTESIAN_POINT ( 'NONE',  ( 54.99999662536844625, 60.62177826491077326, -9.999999999999998224 ) ) ;
#28430=EDGE_CURVE ( 'NONE', #18017, #2273, #18507, .T. ) ;
#28432=ORIENTED_EDGE ( 'NONE', *, *, #27147, .T. ) ;
#28434=EDGE_CURVE ( 'NONE', #2403, #8706, #8102, .T. ) ;
#28436=DIRECTION ( 'NONE',  ( -0.000000000000000000, -0.000000000000000000, 1.000000000000000000 ) ) ;
#28437=CARTESIAN_POINT ( 'NONE',  ( -80.00000337463094979, -17.32050807568882078, -9.999999999999998224 ) ) ;
#28438=CARTESIAN_POINT ( 'NONE',  ( -3.374631334790434423E-06, 69.28203230275516944, -9.999999999999998224 ) ) ;
#28439=ORIENTED_EDGE ( 'NONE', *, *, #7594, .T. ) ;
#28440=CARTESIAN_POINT ( 'NONE',  ( -87.00000337463093558, 25.98076211353317433, -9.999999999999998224 ) ) ;
#28441=EDGE_CURVE ( 'NONE', #33934, #4453, #15296, .T. ) ;
#28442=DIRECTION ( 'NONE',  ( -1.000000000000000000, 0.000000000000000000, 0.000000000000000000 ) ) ;
#28443=DIRECTION ( 'NONE',  ( 0.000000000000000000, 0.000000000000000000, -1.000000000000000000 ) ) ;
#28444=AXIS2_PLACEMENT_3D ( 'NONE', #3691, #34453, #26382 ) ;
#28445=AXIS2_PLACEMENT_3D ( 'NONE', #16284, #10277, #2014 ) ;
#28446=ORIENTED_EDGE ( 'NONE', *, *, #14972, .T. ) ;
#28447=EDGE_LOOP ( 'NONE', ( #5102, #25781, #30089, #4903 ) ) ;
#28448=EDGE_LOOP ( 'NONE', ( #19295, #14502, #15876, #22876 ) ) ;
#28451=EDGE_CURVE ( 'NONE', #26458, #30803, #296, .T. ) ;
#28452=DIRECTION ( 'NONE',  ( -1.000000000000000000, 0.000000000000000000, 0.000000000000000000 ) ) ;
#28453=EDGE_CURVE ( 'NONE', #11641, #34302, #10507, .T. ) ;
#28454=AXIS2_PLACEMENT_3D ( 'NONE', #30290, #6858, #32540 ) ;
#28455=EDGE_CURVE ( 'NONE', #33896, #28909, #25060, .T. ) ;
#28457=DIRECTION ( 'NONE',  ( -1.000000000000000000, 0.000000000000000000, 0.000000000000000000 ) ) ;
#28459=VECTOR ( 'NONE', #8865, 1000.000000000000000 ) ;
#28460=CYLINDRICAL_SURFACE ( 'NONE', #22621, 2.000000000000001776 ) ;
#28461=AXIS2_PLACEMENT_3D ( 'NONE', #6796, #4200, #32310 ) ;
#28462=CARTESIAN_POINT ( 'NONE',  ( -27.78182860042817026, -56.67878100130359087, 12.49999999999999822 ) ) ;
#28463=ORIENTED_EDGE ( 'NONE', *, *, #27317, .F. ) ;
#28465=ORIENTED_EDGE ( 'NONE', *, *, #18350, .T. ) ;
#28466=CARTESIAN_POINT ( 'NONE',  ( 27.99999662536857414, -69.28203230275519786, -9.999999999999998224 ) ) ;
#28467=VECTOR ( 'NONE', #24029, 1000.000000000000000 ) ;
#28470=CARTESIAN_POINT ( 'NONE',  ( 3.499999999999987566, -55.00000000000000000, -10.00000000000000178 ) ) ;
#28471=ORIENTED_EDGE ( 'NONE', *, *, #25907, .F. ) ;
#28472=CIRCLE ( 'NONE', #312, 27.00000000000001421 ) ;
#28473=AXIS2_PLACEMENT_3D ( 'NONE', #12108, #26566, #23574 ) ;
#28474=FACE_BOUND ( 'NONE', #31786, .T. ) ;
#28475=ORIENTED_EDGE ( 'NONE', *, *, #13882, .F. ) ;
#28478=ORIENTED_EDGE ( 'NONE', *, *, #36873, .T. ) ;
#28482=DIRECTION ( 'NONE',  ( 1.000000000000000000, 0.000000000000000000, 0.000000000000000000 ) ) ;
#28483=AXIS2_PLACEMENT_3D ( 'NONE', #25565, #31191, #28004 ) ;
#28484=DIRECTION ( 'NONE',  ( 0.000000000000000000, 0.000000000000000000, 1.000000000000000000 ) ) ;
#28486=ORIENTED_EDGE ( 'NONE', *, *, #32205, .T. ) ;
#28487=AXIS2_PLACEMENT_3D ( 'NONE', #24527, #35772, #6882 ) ;
#28488=AXIS2_PLACEMENT_3D ( 'NONE', #4890, #1702, #30574 ) ;
#28489=ORIENTED_EDGE ( 'NONE', *, *, #36062, .F. ) ;
#28491=AXIS2_PLACEMENT_3D ( 'NONE', #13577, #31361, #5348 ) ;
#28492=EDGE_LOOP ( 'NONE', ( #4668, #5278, #21685, #15575 ) ) ;
#28493=VECTOR ( 'NONE', #14756, 1000.000000000000000 ) ;
#28495=DIRECTION ( 'NONE',  ( 0.000000000000000000, 0.000000000000000000, 1.000000000000000000 ) ) ;
#28496=DIRECTION ( 'NONE',  ( 0.000000000000000000, 0.000000000000000000, 1.000000000000000000 ) ) ;
#28497=CARTESIAN_POINT ( 'NONE',  ( -23.00000337463121980, -77.94228634059963667, -5.000000000000000000 ) ) ;
#28498=AXIS2_PLACEMENT_3D ( 'NONE', #16430, #22420, #8183 ) ;
#28500=CARTESIAN_POINT ( 'NONE',  ( -37.00000337463117717, -77.94228634059963667, 12.50000000000000000 ) ) ;
#28501=EDGE_LOOP ( 'NONE', ( #473, #26498 ) ) ;
#28502=CARTESIAN_POINT ( 'NONE',  ( -34.00000000000027711, -58.88972745734168512, -49.22241343995298024 ) ) ;
#28506=ORIENTED_EDGE ( 'NONE', *, *, #14441, .T. ) ;
#28507=DIRECTION ( 'NONE',  ( 0.000000000000000000, 0.000000000000000000, -1.000000000000000000 ) ) ;
#28510=CIRCLE ( 'NONE', #13523, 27.00000000000001421 ) ;
#28511=ORIENTED_EDGE ( 'NONE', *, *, #14379, .T. ) ;
#28513=CARTESIAN_POINT ( 'NONE',  ( 67.99999662536836809, -34.64101615137759183, -9.999999999999998224 ) ) ;
#28514=DIRECTION ( 'NONE',  ( 1.000000000000000000, 0.000000000000000000, 0.000000000000000000 ) ) ;
#28515=LINE ( 'NONE', #8833, #1717 ) ;
#28517=ORIENTED_EDGE ( 'NONE', *, *, #22172, .F. ) ;
#28518=ORIENTED_EDGE ( 'NONE', *, *, #30448, .T. ) ;
#28519=AXIS2_PLACEMENT_3D ( 'NONE', #14330, #72, #31554 ) ;
#28521=VECTOR ( 'NONE', #29262, 1000.000000000000000 ) ;
#28522=FACE_OUTER_BOUND ( 'NONE', #8151, .T. ) ;
#28523=AXIS2_PLACEMENT_3D ( 'NONE', #25179, #22522, #16731 ) ;
#28525=ORIENTED_EDGE ( 'NONE', *, *, #34940, .F. ) ;
#28526=DIRECTION ( 'NONE',  ( 0.000000000000000000, 0.000000000000000000, -1.000000000000000000 ) ) ;
#28527=ORIENTED_EDGE ( 'NONE', *, *, #35635, .T. ) ;
#28528=ADVANCED_FACE ( 'NONE', ( #30658 ), #36498, .F. ) ;
#28529=EDGE_CURVE ( 'NONE', #28159, #20602, #13958, .T. ) ;
#28530=ORIENTED_EDGE ( 'NONE', *, *, #19696, .T. ) ;
#28531=AXIS2_PLACEMENT_3D ( 'NONE', #25788, #5706, #11508 ) ;
#28532=CARTESIAN_POINT ( 'NONE',  ( 84.88770958243756581, -10.65709945499358824, -5.000000000000000000 ) ) ;
#28533=FACE_OUTER_BOUND ( 'NONE', #18296, .T. ) ;
#28535=ORIENTED_EDGE ( 'NONE', *, *, #8137, .F. ) ;
#28536=ORIENTED_EDGE ( 'NONE', *, *, #800, .T. ) ;
#28537=DIRECTION ( 'NONE',  ( 0.000000000000000000, 0.000000000000000000, 1.000000000000000000 ) ) ;
#28538=DIRECTION ( 'NONE',  ( -0.000000000000000000, -0.000000000000000000, 1.000000000000000000 ) ) ;
#28539=AXIS2_PLACEMENT_3D ( 'NONE', #4578, #16019, #10375 ) ;
#28540=DIRECTION ( 'NONE',  ( 0.000000000000000000, 0.000000000000000000, 1.000000000000000000 ) ) ;
#28541=DIRECTION ( 'NONE',  ( 0.000000000000000000, 0.000000000000000000, -1.000000000000000000 ) ) ;
#28542=EDGE_CURVE ( 'NONE', #13878, #28166, #8711, .T. ) ;
#28543=CIRCLE ( 'NONE', #32115, 2.000000000000001776 ) ;
#28546=FACE_BOUND ( 'NONE', #31969, .T. ) ;
#28547=CYLINDRICAL_SURFACE ( 'NONE', #21990, 2.000000000000001776 ) ;
#28548=DIRECTION ( 'NONE',  ( -0.000000000000000000, -0.000000000000000000, -1.000000000000000000 ) ) ;
#28549=CARTESIAN_POINT ( 'NONE',  ( -82.00000337463094979, -2.404119930384582903E-14, -5.000000000000000000 ) ) ;
#28550=CARTESIAN_POINT ( 'NONE',  ( -34.00000000000027711, -58.88972745734168512, 12.49999999999999822 ) ) ;
#28551=VECTOR ( 'NONE', #14277, 1000.000000000000000 ) ;
#28552=CIRCLE ( 'NONE', #30377, 2.000000000000001776 ) ;
#28553=LINE ( 'NONE', #14113, #22175 ) ;
#28554=EDGE_CURVE ( 'NONE', #32213, #16797, #28587, .T. ) ;
#28555=DIRECTION ( 'NONE',  ( 0.000000000000000000, 0.000000000000000000, 1.000000000000000000 ) ) ;
#28556=VERTEX_POINT ( 'NONE', #33671 ) ;
#28558=CARTESIAN_POINT ( 'NONE',  ( 54.99999662536844625, -60.62177826491080168, -9.999999999999998224 ) ) ;
#28559=CARTESIAN_POINT ( 'NONE',  ( -40.00000337463113453, -69.28203230275519786, -9.999999999999998224 ) ) ;
#28560=ORIENTED_EDGE ( 'NONE', *, *, #5342, .T. ) ;
#28561=CIRCLE ( 'NONE', #27976, 27.00000000000001421 ) ;
#28563=ORIENTED_EDGE ( 'NONE', *, *, #23329, .F. ) ;
#28564=LINE ( 'NONE', #5150, #30317 ) ;
#28565=CARTESIAN_POINT ( 'NONE',  ( -70.00000337463099243, 34.64101615137758472, 17.49999999999999645 ) ) ;
#28566=CARTESIAN_POINT ( 'NONE',  ( -75.00000337463100664, -43.30127018922202353, -9.999999999999998224 ) ) ;
#28568=AXIS2_PLACEMENT_3D ( 'NONE', #30626, #27802, #16766 ) ;
#28569=CIRCLE ( 'NONE', #35178, 65.00000000000000000 ) ;
#28570=DIRECTION ( 'NONE',  ( 0.000000000000000000, 0.000000000000000000, 1.000000000000000000 ) ) ;
#28571=AXIS2_PLACEMENT_3D ( 'NONE', #32514, #35377, #24266 ) ;
#28572=ORIENTED_EDGE ( 'NONE', *, *, #32538, .T. ) ;
#28573=EDGE_CURVE ( 'NONE', #29660, #7478, #27839, .T. ) ;
#28575=EDGE_LOOP ( 'NONE', ( #5566, #16447, #6830, #21071 ) ) ;
#28576=DIRECTION ( 'NONE',  ( 1.000000000000000000, 0.000000000000000000, 0.000000000000000000 ) ) ;
#28577=VERTEX_POINT ( 'NONE', #22055 ) ;
#28578=AXIS2_PLACEMENT_3D ( 'NONE', #2916, #3092, #11880 ) ;
#28580=AXIS2_PLACEMENT_3D ( 'NONE', #9806, #21630, #1752 ) ;
#28581=CARTESIAN_POINT ( 'NONE',  ( -62.00000337463108480, -51.96152422706641971, 12.50000000000000000 ) ) ;
#28582=LINE ( 'NONE', #22960, #3460 ) ;
#28585=EDGE_CURVE ( 'NONE', #7967, #625, #4976, .T. ) ;
#28586=EDGE_LOOP ( 'NONE', ( #36145, #22532 ) ) ;
#28587=LINE ( 'NONE', #31217, #9293 ) ;
#28590=LINE ( 'NONE', #22969, #34939 ) ;
#28592=EDGE_LOOP ( 'NONE', ( #24173, #1735, #36673, #17422 ) ) ;
#28593=DIRECTION ( 'NONE',  ( -1.000000000000000000, 5.268419445559189404E-15, 0.000000000000000000 ) ) ;
#28594=CIRCLE ( 'NONE', #9434, 2.000000000000001776 ) ;
#28595=DIRECTION ( 'NONE',  ( -1.000000000000000000, 0.000000000000000000, 0.000000000000000000 ) ) ;
#28596=ORIENTED_EDGE ( 'NONE', *, *, #7828, .T. ) ;
#28597=DIRECTION ( 'NONE',  ( 0.000000000000000000, 0.000000000000000000, -1.000000000000000000 ) ) ;
#28598=CIRCLE ( 'NONE', #12417, 1.999999999999998224 ) ;
#28599=AXIS2_PLACEMENT_3D ( 'NONE', #34015, #19022, #13561 ) ;
#28600=DIRECTION ( 'NONE',  ( 0.000000000000000000, 0.000000000000000000, 1.000000000000000000 ) ) ;
#28602=DIRECTION ( 'NONE',  ( 0.000000000000000000, 0.000000000000000000, 1.000000000000000000 ) ) ;
#28603=CIRCLE ( 'NONE', #13615, 2.000000000000001776 ) ;
#28604=ORIENTED_EDGE ( 'NONE', *, *, #15853, .F. ) ;
#28605=VECTOR ( 'NONE', #10345, 1000.000000000000000 ) ;
#28606=EDGE_LOOP ( 'NONE', ( #20018, #19194, #618, #18414 ) ) ;
#28608=DIRECTION ( 'NONE',  ( 0.000000000000000000, 0.000000000000000000, -1.000000000000000000 ) ) ;
#28609=AXIS2_PLACEMENT_3D ( 'NONE', #19485, #11412, #34289 ) ;
#28610=EDGE_CURVE ( 'NONE', #4355, #11389, #5107, .T. ) ;
#28611=ORIENTED_EDGE ( 'NONE', *, *, #28810, .F. ) ;
#28612=ORIENTED_EDGE ( 'NONE', *, *, #6917, .F. ) ;
#28613=CYLINDRICAL_SURFACE ( 'NONE', #20829, 2.000000000000000000 ) ;
#28614=LINE ( 'NONE', #2563, #18252 ) ;
#28616=EDGE_CURVE ( 'NONE', #26529, #23686, #28037, .T. ) ;
#28617=ORIENTED_EDGE ( 'NONE', *, *, #22045, .F. ) ;
#28619=CARTESIAN_POINT ( 'NONE',  ( -33.00000337463117006, -77.94228634059963667, 12.50000000000000000 ) ) ;
#28620=ORIENTED_EDGE ( 'NONE', *, *, #24885, .T. ) ;
#28623=ORIENTED_EDGE ( 'NONE', *, *, #29944, .F. ) ;
#28625=CYLINDRICAL_SURFACE ( 'NONE', #31492, 2.000000000000001776 ) ;
#28627=AXIS2_PLACEMENT_3D ( 'NONE', #34887, #11806, #18178 ) ;
#28628=LINE ( 'NONE', #25445, #19134 ) ;
#28629=PLANE ( 'NONE',  #21490 ) ;
#28630=VERTEX_POINT ( 'NONE', #25237 ) ;
#28633=AXIS2_PLACEMENT_3D ( 'NONE', #28462, #8042, #25681 ) ;
#28634=ADVANCED_FACE ( 'NONE', ( #10962 ), #14148, .F. ) ;
#28635=DIRECTION ( 'NONE',  ( 0.000000000000000000, -0.000000000000000000, -1.000000000000000000 ) ) ;
#28637=ORIENTED_EDGE ( 'NONE', *, *, #16743, .T. ) ;
#28638=CARTESIAN_POINT ( 'NONE',  ( -18.00000337463123756, -86.60254037844400443, 12.50000000000000000 ) ) ;
#28639=FACE_OUTER_BOUND ( 'NONE', #33629, .T. ) ;
#28640=CIRCLE ( 'NONE', #8291, 2.000000000000001776 ) ;
#28642=VERTEX_POINT ( 'NONE', #10575 ) ;
#28643=ORIENTED_EDGE ( 'NONE', *, *, #33709, .F. ) ;
#28644=AXIS2_PLACEMENT_3D ( 'NONE', #19507, #36585, #36401 ) ;
#28645=ORIENTED_EDGE ( 'NONE', *, *, #31170, .F. ) ;
#28646=CIRCLE ( 'NONE', #31037, 2.000000000000001776 ) ;
#28647=AXIS2_PLACEMENT_3D ( 'NONE', #10973, #36509, #33509 ) ;
#28648=DIRECTION ( 'NONE',  ( 0.000000000000000000, 0.000000000000000000, 1.000000000000000000 ) ) ;
#28649=EDGE_CURVE ( 'NONE', #24286, #17057, #27253, .T. ) ;
#28650=AXIS2_PLACEMENT_3D ( 'NONE', #20395, #6703, #15321 ) ;
#28651=LINE ( 'NONE', #8237, #18861 ) ;
#28653=LINE ( 'NONE', #23218, #5143 ) ;
#28654=EDGE_CURVE ( 'NONE', #36932, #30829, #18892, .T. ) ;
#28656=CARTESIAN_POINT ( 'NONE',  ( -50.00000337463110611, -69.28203230275519786, -9.999999999999998224 ) ) ;
#28657=AXIS2_PLACEMENT_3D ( 'NONE', #23275, #17287, #3393 ) ;
#28658=ORIENTED_EDGE ( 'NONE', *, *, #27648, .T. ) ;
#28659=EDGE_CURVE ( 'NONE', #2842, #15693, #36458, .T. ) ;
#28660=EDGE_LOOP ( 'NONE', ( #3791, #34465, #13242, #22758 ) ) ;
#28661=AXIS2_PLACEMENT_3D ( 'NONE', #33248, #27797, #1762 ) ;
#28665=CARTESIAN_POINT ( 'NONE',  ( 62.99999662536839651, -60.62177826491080168, -5.000000000000000000 ) ) ;
#28666=EDGE_CURVE ( 'NONE', #22278, #6597, #30252, .T. ) ;
#28667=ORIENTED_EDGE ( 'NONE', *, *, #32722, .T. ) ;
#28669=ADVANCED_FACE ( 'NONE', ( #2123 ), #13207, .F. ) ;
#28670=FACE_BOUND ( 'NONE', #5005, .T. ) ;
#28671=VECTOR ( 'NONE', #33147, 1000.000000000000000 ) ;
#28672=VERTEX_POINT ( 'NONE', #36263 ) ;
#28673=ORIENTED_EDGE ( 'NONE', *, *, #36193, .T. ) ;
#28674=CIRCLE ( 'NONE', #19120, 1.999999999999998224 ) ;
#28675=CARTESIAN_POINT ( 'NONE',  ( -48.00000337463109190, 51.96152422706637708, -9.999999999999998224 ) ) ;
#28676=EDGE_LOOP ( 'NONE', ( #23852, #5359, #34569, #8570 ) ) ;
#28677=EDGE_CURVE ( 'NONE', #24850, #34867, #6321, .T. ) ;
#28678=EDGE_CURVE ( 'NONE', #14243, #2055, #21913, .T. ) ;
#28679=CARTESIAN_POINT ( 'NONE',  ( 84.99999662536832545, 8.660254037844394404, -9.999999999999998224 ) ) ;
#28680=ADVANCED_FACE ( 'NONE', ( #10767 ), #35713, .F. ) ;
#28681=FACE_OUTER_BOUND ( 'NONE', #19690, .T. ) ;
#28682=EDGE_CURVE ( 'NONE', #5583, #8974, #21290, .T. ) ;
#28683=ORIENTED_EDGE ( 'NONE', *, *, #4256, .F. ) ;
#28684=EDGE_CURVE ( 'NONE', #8353, #13437, #30285, .T. ) ;
#28685=ORIENTED_EDGE ( 'NONE', *, *, #1156, .F. ) ;
#28686=AXIS2_PLACEMENT_3D ( 'NONE', #3720, #712, #34849 ) ;
#28688=VERTEX_POINT ( 'NONE', #7772 ) ;
#28690=ORIENTED_EDGE ( 'NONE', *, *, #26092, .T. ) ;
#28691=DIRECTION ( 'NONE',  ( 0.000000000000000000, 0.000000000000000000, 1.000000000000000000 ) ) ;
#28692=CIRCLE ( 'NONE', #11927, 3.000000000000002665 ) ;
#28693=DIRECTION ( 'NONE',  ( 0.000000000000000000, 0.000000000000000000, 1.000000000000000000 ) ) ;
#28694=DIRECTION ( 'NONE',  ( 1.000000000000000000, 0.000000000000000000, 0.000000000000000000 ) ) ;
#28695=CARTESIAN_POINT ( 'NONE',  ( -68.00000337463099243, 51.96152422706637708, -5.000000000000000000 ) ) ;
#28696=DIRECTION ( 'NONE',  ( 0.000000000000000000, 0.000000000000000000, -1.000000000000000000 ) ) ;
#28697=ORIENTED_EDGE ( 'NONE', *, *, #15761, .T. ) ;
#28698=DIRECTION ( 'NONE',  ( -1.000000000000000000, 0.000000000000000000, 0.000000000000000000 ) ) ;
#28700=AXIS2_PLACEMENT_3D ( 'NONE', #24764, #33014, #24961 ) ;
#28701=AXIS2_PLACEMENT_3D ( 'NONE', #31439, #5769, #14751 ) ;
#28702=CARTESIAN_POINT ( 'NONE',  ( 54.99999662536846046, -43.30127018922200222, -9.999999999999998224 ) ) ;
#28703=ORIENTED_EDGE ( 'NONE', *, *, #9371, .F. ) ;
#28704=CARTESIAN_POINT ( 'NONE',  ( 67.99999662536838230, 17.32050807568879236, -9.999999999999998224 ) ) ;
#28705=AXIS2_PLACEMENT_3D ( 'NONE', #31180, #14099, #19560 ) ;
#28706=CARTESIAN_POINT ( 'NONE',  ( -45.00000337463111322, 60.62177826491077326, 17.49999999999999645 ) ) ;
#28707=ORIENTED_EDGE ( 'NONE', *, *, #3713, .T. ) ;
#28708=VERTEX_POINT ( 'NONE', #4779 ) ;
#28709=CARTESIAN_POINT ( 'NONE',  ( 84.99999662536831124, -25.98076211353319565, -9.999999999999998224 ) ) ;
#28710=CARTESIAN_POINT ( 'NONE',  ( -30.00000337463119848, -69.28203230275522628, -9.999999999999998224 ) ) ;
#28712=PLANE ( 'NONE',  #5315 ) ;
#28714=EDGE_LOOP ( 'NONE', ( #28802, #11574 ) ) ;
#28715=CIRCLE ( 'NONE', #14942, 2.000000000000001776 ) ;
#28716=FACE_OUTER_BOUND ( 'NONE', #36033, .T. ) ;
#28719=AXIS2_PLACEMENT_3D ( 'NONE', #19241, #30654, #27834 ) ;
#28720=ORIENTED_EDGE ( 'NONE', *, *, #1873, .T. ) ;
#28721=ADVANCED_FACE ( 'NONE', ( #30628 ), #4945, .F. ) ;
#28722=FACE_OUTER_BOUND ( 'NONE', #3998, .T. ) ;
#28723=CIRCLE ( 'NONE', #7190, 2.000000000000001776 ) ;
#28724=ORIENTED_EDGE ( 'NONE', *, *, #21186, .T. ) ;
#28725=ORIENTED_EDGE ( 'NONE', *, *, #32842, .F. ) ;
#28726=CYLINDRICAL_SURFACE ( 'NONE', #18804, 2.000000000000001776 ) ;
#28728=DIRECTION ( 'NONE',  ( 1.000000000000000000, 0.000000000000000000, 0.000000000000000000 ) ) ;
#28730=ORIENTED_EDGE ( 'NONE', *, *, #24997, .F. ) ;
#28732=VECTOR ( 'NONE', #20009, 1000.000000000000000 ) ;
#28733=LINE ( 'NONE', #22755, #15485 ) ;
#28735=DIRECTION ( 'NONE',  ( 0.000000000000000000, 0.000000000000000000, 1.000000000000000000 ) ) ;
#28736=ORIENTED_EDGE ( 'NONE', *, *, #3430, .T. ) ;
#28737=DIRECTION ( 'NONE',  ( 0.000000000000000000, 0.000000000000000000, 1.000000000000000000 ) ) ;
#28738=FACE_BOUND ( 'NONE', #4554, .T. ) ;
#28739=DIRECTION ( 'NONE',  ( 0.000000000000000000, 0.000000000000000000, 1.000000000000000000 ) ) ;
#28740=CARTESIAN_POINT ( 'NONE',  ( 42.99999662536848888, 60.62177826491077326, -5.000000000000000000 ) ) ;
#28741=CARTESIAN_POINT ( 'NONE',  ( 1.999996625368710257, -69.28203230275519786, 12.50000000000000000 ) ) ;
#28742=AXIS2_PLACEMENT_3D ( 'NONE', #12215, #17503, #15239 ) ;
#28743=DIRECTION ( 'NONE',  ( -1.000000000000000000, 0.000000000000000000, 0.000000000000000000 ) ) ;
#28744=DIRECTION ( 'NONE',  ( 1.000000000000000000, 0.000000000000000000, 0.000000000000000000 ) ) ;
#28745=AXIS2_PLACEMENT_3D ( 'NONE', #22206, #8129, #19577 ) ;
#28747=ORIENTED_EDGE ( 'NONE', *, *, #1281, .T. ) ;
#28748=CARTESIAN_POINT ( 'NONE',  ( 9.999996625368618552, 69.28203230275516944, -5.000000000000000000 ) ) ;
#28750=CIRCLE ( 'NONE', #35971, 45.00000000000000711 ) ;
#28751=CARTESIAN_POINT ( 'NONE',  ( 84.99999662536831124, -8.660254037844397956, 12.50000000000000000 ) ) ;
#28752=ADVANCED_FACE ( 'NONE', ( #22204 ), #16215, .T. ) ;
#28753=EDGE_LOOP ( 'NONE', ( #30321, #23973, #8530, #28463 ) ) ;
#28754=ORIENTED_EDGE ( 'NONE', *, *, #28901, .T. ) ;
#28755=ORIENTED_EDGE ( 'NONE', *, *, #28385, .T. ) ;
#28756=DIRECTION ( 'NONE',  ( 0.000000000000000000, 0.000000000000000000, -1.000000000000000000 ) ) ;
#28757=CARTESIAN_POINT ( 'NONE',  ( -45.00000337463111322, 77.94228634059959404, 17.49999999999999645 ) ) ;
#28758=DIRECTION ( 'NONE',  ( 0.000000000000000000, 0.000000000000000000, -1.000000000000000000 ) ) ;
#28760=DIRECTION ( 'NONE',  ( -0.4999999999999968359, 0.8660254037844404840, 0.000000000000000000 ) ) ;
#28761=ORIENTED_EDGE ( 'NONE', *, *, #11468, .F. ) ;
#28762=VECTOR ( 'NONE', #12598, 1000.000000000000000 ) ;
#28763=DIRECTION ( 'NONE',  ( -1.000000000000000000, 0.000000000000000000, 0.000000000000000000 ) ) ;
#28765=DIRECTION ( 'NONE',  ( 0.000000000000000000, 0.000000000000000000, -1.000000000000000000 ) ) ;
#28767=ORIENTED_EDGE ( 'NONE', *, *, #8246, .F. ) ;
#28768=DIRECTION ( 'NONE',  ( 0.000000000000000000, 0.000000000000000000, 1.000000000000000000 ) ) ;
#28769=FACE_OUTER_BOUND ( 'NONE', #33540, .T. ) ;
#28770=CARTESIAN_POINT ( 'NONE',  ( 34.99999662536855283, 60.62177826491078747, 12.50000000000000000 ) ) ;
#28771=AXIS2_PLACEMENT_3D ( 'NONE', #2469, #13890, #19175 ) ;
#28772=EDGE_CURVE ( 'NONE', #4318, #24271, #35674, .T. ) ;
#28774=CYLINDRICAL_SURFACE ( 'NONE', #8327, 2.000000000000001776 ) ;
#28775=CARTESIAN_POINT ( 'NONE',  ( 82.99999662536831124, -25.98076211353319565, -9.999999999999998224 ) ) ;
#28776=CARTESIAN_POINT ( 'NONE',  ( -33.00000337463116296, -60.62177826491080168, 12.50000000000000000 ) ) ;
#28777=ORIENTED_EDGE ( 'NONE', *, *, #26189, .T. ) ;
#28778=FACE_OUTER_BOUND ( 'NONE', #19202, .T. ) ;
#28780=EDGE_LOOP ( 'NONE', ( #25407, #7544 ) ) ;
#28782=CYLINDRICAL_SURFACE ( 'NONE', #4632, 2.000000000000001776 ) ;
#28783=DIRECTION ( 'NONE',  ( 1.000000000000000000, 0.000000000000000000, 0.000000000000000000 ) ) ;
#28785=CARTESIAN_POINT ( 'NONE',  ( -68.00000000000000000, 0.000000000000000000, 12.49999999999999822 ) ) ;
#28786=ADVANCED_FACE ( 'NONE', ( #15650 ), #24651, .F. ) ;
#28787=EDGE_LOOP ( 'NONE', ( #17018, #30565, #26022, #31301, #7702, #4265, #13975, #15292, #35556, #32925, #22451, #4594, #17178 ) ) ;
#28788=CARTESIAN_POINT ( 'NONE',  ( 52.39915983220795681, 35.19434990244919703, -4.999999999999997335 ) ) ;
#28789=DIRECTION ( 'NONE',  ( 0.000000000000000000, 0.000000000000000000, 1.000000000000000000 ) ) ;
#28790=EDGE_CURVE ( 'NONE', #35117, #13323, #27282, .T. ) ;
#28791=VERTEX_POINT ( 'NONE', #28549 ) ;
#28792=ORIENTED_EDGE ( 'NONE', *, *, #30263, .T. ) ;
#28793=ORIENTED_EDGE ( 'NONE', *, *, #23802, .T. ) ;
#28794=AXIS2_PLACEMENT_3D ( 'NONE', #13672, #2428, #10478 ) ;
#28798=EDGE_CURVE ( 'NONE', #33601, #24245, #22931, .T. ) ;
#28799=DIRECTION ( 'NONE',  ( -0.000000000000000000, -0.000000000000000000, 1.000000000000000000 ) ) ;
#28800=ORIENTED_EDGE ( 'NONE', *, *, #32563, .F. ) ;
#28801=CARTESIAN_POINT ( 'NONE',  ( -45.00000337463111322, 77.94228634059959404, -9.999999999999998224 ) ) ;
#28802=ORIENTED_EDGE ( 'NONE', *, *, #18079, .F. ) ;
#28803=FACE_BOUND ( 'NONE', #9839, .T. ) ;
#28804=CARTESIAN_POINT ( 'NONE',  ( 56.67878100130369035, -27.78182860042797131, -4.999999999999997335 ) ) ;
#28805=CARTESIAN_POINT ( 'NONE',  ( -42.00000337463114164, 69.28203230275516944, -9.999999999999998224 ) ) ;
#28806=CARTESIAN_POINT ( 'NONE',  ( 87.99999662536828282, 2.449293598294706414E-16, -9.999999999999998224 ) ) ;
#28807=AXIS2_PLACEMENT_3D ( 'NONE', #6581, #30003, #30569 ) ;
#28809=DIRECTION ( 'NONE',  ( 0.000000000000000000, 0.000000000000000000, 1.000000000000000000 ) ) ;
#28810=EDGE_CURVE ( 'NONE', #36526, #17340, #32689, .T. ) ;
#28811=CARTESIAN_POINT ( 'NONE',  ( -4.279621169095561228, 62.97617850287782915, 12.49999999999999822 ) ) ;
#28812=DIRECTION ( 'NONE',  ( 1.000000000000000000, 0.000000000000000000, 0.000000000000000000 ) ) ;
#28813=EDGE_LOOP ( 'NONE', ( #25646, #25162, #32419, #16276 ) ) ;
#28814=DIRECTION ( 'NONE',  ( 0.000000000000000000, 0.000000000000000000, 1.000000000000000000 ) ) ;
#28816=DIRECTION ( 'NONE',  ( 0.000000000000000000, 0.000000000000000000, 1.000000000000000000 ) ) ;
#28817=ADVANCED_FACE ( 'NONE', ( #25924 ), #25763, .T. ) ;
#28818=VERTEX_POINT ( 'NONE', #5879 ) ;
#28819=VERTEX_POINT ( 'NONE', #221 ) ;
#28820=EDGE_CURVE ( 'NONE', #26898, #4119, #11696, .T. ) ;
#28821=ORIENTED_EDGE ( 'NONE', *, *, #5191, .T. ) ;
#28823=AXIS2_PLACEMENT_3D ( 'NONE', #7209, #9813, #21068 ) ;
#28825=CARTESIAN_POINT ( 'NONE',  ( 79.99999662536833966, 34.64101615137759183, -9.999999999999998224 ) ) ;
#28826=CIRCLE ( 'NONE', #27043, 2.000000000000001776 ) ;
#28827=DIRECTION ( 'NONE',  ( 1.000000000000000000, 0.000000000000000000, 0.000000000000000000 ) ) ;
#28828=DIRECTION ( 'NONE',  ( 1.000000000000000000, 0.000000000000000000, 0.000000000000000000 ) ) ;
#28829=VERTEX_POINT ( 'NONE', #34368 ) ;
#28831=CARTESIAN_POINT ( 'NONE',  ( -51.13139720814437084, -27.49999999999955591, -10.00000000000000178 ) ) ;
#28832=EDGE_CURVE ( 'NONE', #19362, #13179, #18320, .T. ) ;
#28833=DIRECTION ( 'NONE',  ( 0.000000000000000000, 0.000000000000000000, -1.000000000000000000 ) ) ;
#28834=DIRECTION ( 'NONE',  ( 0.000000000000000000, 0.000000000000000000, 1.000000000000000000 ) ) ;
#28836=FACE_BOUND ( 'NONE', #1832, .T. ) ;
#28837=EDGE_LOOP ( 'NONE', ( #5714, #35750 ) ) ;
#28838=ORIENTED_EDGE ( 'NONE', *, *, #22097, .F. ) ;
#28839=DIRECTION ( 'NONE',  ( 1.000000000000000000, 0.000000000000000000, 0.000000000000000000 ) ) ;
#28840=EDGE_LOOP ( 'NONE', ( #34291, #7585, #2490, #13084, #8471 ) ) ;
#28842=EDGE_CURVE ( 'NONE', #28991, #35130, #9913, .T. ) ;
#28844=DIRECTION ( 'NONE',  ( 0.000000000000000000, 0.000000000000000000, 1.000000000000000000 ) ) ;
#28845=EDGE_LOOP ( 'NONE', ( #12319, #13856, #27710, #6039 ) ) ;
#28846=EDGE_CURVE ( 'NONE', #16912, #15905, #5337, .T. ) ;
#28847=VERTEX_POINT ( 'NONE', #8670 ) ;
#28848=ORIENTED_EDGE ( 'NONE', *, *, #22290, .T. ) ;
#28850=ORIENTED_EDGE ( 'NONE', *, *, #22703, .T. ) ;
#28851=ORIENTED_EDGE ( 'NONE', *, *, #2511, .F. ) ;
#28852=CARTESIAN_POINT ( 'NONE',  ( -30.00000337463118427, 69.28203230275516944, 17.49999999999999645 ) ) ;
#28853=ADVANCED_FACE ( 'NONE', ( #5676 ), #11112, .F. ) ;
#28854=DIRECTION ( 'NONE',  ( -1.000000000000000000, 0.000000000000000000, 0.000000000000000000 ) ) ;
#28855=EDGE_CURVE ( 'NONE', #2567, #12964, #11651, .T. ) ;
#28856=CARTESIAN_POINT ( 'NONE',  ( 62.33939050065184517, -13.89091430021398565, 12.49999999999999822 ) ) ;
#28857=DIRECTION ( 'NONE',  ( 0.000000000000000000, 0.000000000000000000, -1.000000000000000000 ) ) ;
#28861=AXIS2_PLACEMENT_3D ( 'NONE', #15765, #13493, #13316 ) ;
#28862=CIRCLE ( 'NONE', #15119, 2.000000000000001776 ) ;
#28863=DIRECTION ( 'NONE',  ( 0.000000000000000000, 0.000000000000000000, 1.000000000000000000 ) ) ;
#28864=CARTESIAN_POINT ( 'NONE',  ( 47.99999662536846756, 51.96152422706637708, -9.999999999999998224 ) ) ;
#28865=ORIENTED_EDGE ( 'NONE', *, *, #2829, .F. ) ;
#28866=DIRECTION ( 'NONE',  ( 1.000000000000000000, 0.000000000000000000, 0.000000000000000000 ) ) ;
#28867=CARTESIAN_POINT ( 'NONE',  ( 39.99999662536853151, 69.28203230275518365, -9.999999999999998224 ) ) ;
#28869=VERTEX_POINT ( 'NONE', #28741 ) ;
#28870=EDGE_CURVE ( 'NONE', #9726, #36932, #17123, .T. ) ;
#28871=ORIENTED_EDGE ( 'NONE', *, *, #18044, .F. ) ;
#28872=DIRECTION ( 'NONE',  ( 0.000000000000000000, 0.000000000000000000, 1.000000000000000000 ) ) ;
#28873=EDGE_CURVE ( 'NONE', #31910, #21959, #30866, .T. ) ;
#28874=AXIS2_PLACEMENT_3D ( 'NONE', #2277, #16342, #36412 ) ;
#28875=CARTESIAN_POINT ( 'NONE',  ( -35.19434990244938888, 52.39915983220783602, -4.999999999999997335 ) ) ;
#28876=CARTESIAN_POINT ( 'NONE',  ( 19.99999662536861678, -69.28203230275519786, -5.000000000000000000 ) ) ;
#28877=DIRECTION ( 'NONE',  ( -1.000000000000000000, 0.000000000000000000, 0.000000000000000000 ) ) ;
#28879=CARTESIAN_POINT ( 'NONE',  ( -68.00000337463102085, -51.96152422706641971, 12.50000000000000000 ) ) ;
#28881=CARTESIAN_POINT ( 'NONE',  ( -57.00000337463109901, -60.62177826491083010, -9.999999999999998224 ) ) ;
#28883=DIRECTION ( 'NONE',  ( 0.000000000000000000, 0.000000000000000000, 1.000000000000000000 ) ) ;
#28884=VERTEX_POINT ( 'NONE', #2679 ) ;
#28886=CIRCLE ( 'NONE', #9763, 45.00000000000000711 ) ;
#28887=DIRECTION ( 'NONE',  ( 0.000000000000000000, 0.000000000000000000, -1.000000000000000000 ) ) ;
#28889=DIRECTION ( 'NONE',  ( 1.000000000000000000, 0.000000000000000000, 0.000000000000000000 ) ) ;
#28890=ORIENTED_EDGE ( 'NONE', *, *, #2142, .F. ) ;
#28892=ORIENTED_EDGE ( 'NONE', *, *, #1629, .T. ) ;
#28893=DIRECTION ( 'NONE',  ( 0.000000000000000000, 0.000000000000000000, 1.000000000000000000 ) ) ;
#28894=DIRECTION ( 'NONE',  ( 0.000000000000000000, 0.000000000000000000, 1.000000000000000000 ) ) ;
#28895=DIRECTION ( 'NONE',  ( 1.000000000000000000, 0.000000000000000000, 0.000000000000000000 ) ) ;
#28896=ORIENTED_EDGE ( 'NONE', *, *, #4073, .T. ) ;
#28897=DIRECTION ( 'NONE',  ( 0.000000000000000000, 0.000000000000000000, 1.000000000000000000 ) ) ;
#28898=CIRCLE ( 'NONE', #30702, 27.00000000000001421 ) ;
#28899=FACE_BOUND ( 'NONE', #30713, .T. ) ;
#28900=AXIS2_PLACEMENT_3D ( 'NONE', #35540, #36276, #24837 ) ;
#28901=EDGE_CURVE ( 'NONE', #15901, #1755, #9045, .T. ) ;
#28902=CARTESIAN_POINT ( 'NONE',  ( -75.00000337463097821, 25.98076211353318854, -9.999999999999998224 ) ) ;
#28903=CARTESIAN_POINT ( 'NONE',  ( 56.99999662536844625, -60.62177826491080168, -5.000000000000000000 ) ) ;
#28904=DIRECTION ( 'NONE',  ( -1.000000000000000000, 0.000000000000000000, -0.000000000000000000 ) ) ;
#28905=DIRECTION ( 'NONE',  ( 1.000000000000000000, 0.000000000000000000, 0.000000000000000000 ) ) ;
#28906=PRODUCT_DEFINITION_SHAPE ( 'NONE', 'NONE',  #377 ) ;
#28907=DIRECTION ( 'NONE',  ( 1.000000000000000000, 0.000000000000000000, 0.000000000000000000 ) ) ;
#28908=CARTESIAN_POINT ( 'NONE',  ( -80.00000337463094979, 34.64101615137757051, 12.50000000000000000 ) ) ;
#28909=VERTEX_POINT ( 'NONE', #15043 ) ;
#28910=LINE ( 'NONE', #20118, #2840 ) ;
#28911=LINE ( 'NONE', #3434, #11182 ) ;
#28912=CIRCLE ( 'NONE', #16964, 2.000000000000001776 ) ;
#28914=EDGE_CURVE ( 'NONE', #16077, #1955, #2748, .T. ) ;
#28915=EDGE_LOOP ( 'NONE', ( #14499, #12130 ) ) ;
#28916=EDGE_CURVE ( 'NONE', #36648, #8999, #3329, .T. ) ;
#28917=AXIS2_PLACEMENT_3D ( 'NONE', #11578, #6334, #26408 ) ;
#28918=ORIENTED_EDGE ( 'NONE', *, *, #337, .F. ) ;
#28920=EDGE_CURVE ( 'NONE', #36282, #20160, #24291, .T. ) ;
#28921=EDGE_CURVE ( 'NONE', #32452, #7645, #26469, .T. ) ;
#28922=DIRECTION ( 'NONE',  ( 0.000000000000000000, 0.000000000000000000, 1.000000000000000000 ) ) ;
#28923=CARTESIAN_POINT ( 'NONE',  ( 64.99999662536839651, -60.62177826491080168, -9.999999999999998224 ) ) ;
#28925=VERTEX_POINT ( 'NONE', #26854 ) ;
#28926=FACE_OUTER_BOUND ( 'NONE', #21638, .T. ) ;
#28927=AXIS2_PLACEMENT_3D ( 'NONE', #37013, #34212, #11320 ) ;
#28929=DIRECTION ( 'NONE',  ( 1.000000000000000000, 0.000000000000000000, 0.000000000000000000 ) ) ;
#28930=ORIENTED_EDGE ( 'NONE', *, *, #25811, .T. ) ;
#28932=VERTEX_POINT ( 'NONE', #20303 ) ;
#28933=EDGE_LOOP ( 'NONE', ( #30242, #8549, #23908, #4076 ) ) ;
#28936=DIRECTION ( 'NONE',  ( 0.000000000000000000, 0.000000000000000000, 1.000000000000000000 ) ) ;
#28937=ORIENTED_EDGE ( 'NONE', *, *, #26454, .T. ) ;
#28939=AXIS2_PLACEMENT_3D ( 'NONE', #9436, #34935, #21048 ) ;
#28940=ADVANCED_FACE ( 'NONE', ( #23661 ), #12589, .F. ) ;
#28941=DIRECTION ( 'NONE',  ( 1.000000000000000000, 0.000000000000000000, 0.000000000000000000 ) ) ;
#28944=ORIENTED_EDGE ( 'NONE', *, *, #31808, .T. ) ;
#28945=DIRECTION ( 'NONE',  ( -1.000000000000000000, 0.000000000000000000, 0.000000000000000000 ) ) ;
#28946=DIRECTION ( 'NONE',  ( 0.000000000000000000, 0.000000000000000000, 1.000000000000000000 ) ) ;
#28947=ORIENTED_EDGE ( 'NONE', *, *, #8860, .F. ) ;
#28948=FACE_OUTER_BOUND ( 'NONE', #15342, .T. ) ;
#28949=DIRECTION ( 'NONE',  ( 1.000000000000000000, 0.000000000000000000, 0.000000000000000000 ) ) ;
#28950=DIRECTION ( 'NONE',  ( 0.000000000000000000, 0.000000000000000000, -1.000000000000000000 ) ) ;
#28952=AXIS2_PLACEMENT_3D ( 'NONE', #26740, #9687, #33098 ) ;
#28953=CARTESIAN_POINT ( 'NONE',  ( 2.999999999999768630, -68.00000000000000000, -4.999999999999997335 ) ) ;
#28954=AXIS2_PLACEMENT_3D ( 'NONE', #31150, #13891, #17 ) ;
#28955=ORIENTED_EDGE ( 'NONE', *, *, #22469, .F. ) ;
#28957=DIRECTION ( 'NONE',  ( -0.000000000000000000, -0.000000000000000000, 1.000000000000000000 ) ) ;
#28958=DIRECTION ( 'NONE',  ( 0.000000000000000000, 0.000000000000000000, 1.000000000000000000 ) ) ;
#28961=ORIENTED_EDGE ( 'NONE', *, *, #2525, .T. ) ;
#28962=EDGE_CURVE ( 'NONE', #9593, #19500, #18208, .T. ) ;
#28963=DIRECTION ( 'NONE',  ( 1.000000000000000000, 0.000000000000000000, 0.000000000000000000 ) ) ;
#28964=DIRECTION ( 'NONE',  ( 1.000000000000000000, 0.000000000000000000, 0.000000000000000000 ) ) ;
#28966=CIRCLE ( 'NONE', #13990, 33.00000000000001421 ) ;
#28967=FACE_OUTER_BOUND ( 'NONE', #25558, .T. ) ;
#28968=ORIENTED_EDGE ( 'NONE', *, *, #19979, .T. ) ;
#28969=DIRECTION ( 'NONE',  ( 0.000000000000000000, 0.000000000000000000, -1.000000000000000000 ) ) ;
#28971=FACE_BOUND ( 'NONE', #32818, .T. ) ;
#28972=AXIS2_PLACEMENT_3D ( 'NONE', #959, #12375, #23848 ) ;
#28973=DIRECTION ( 'NONE',  ( 0.000000000000000000, 0.000000000000000000, 1.000000000000000000 ) ) ;
#28974=AXIS2_PLACEMENT_3D ( 'NONE', #16305, #7487, #27562 ) ;
#28975=DIRECTION ( 'NONE',  ( 0.000000000000000000, 0.000000000000000000, -1.000000000000000000 ) ) ;
#28977=DIRECTION ( 'NONE',  ( 1.000000000000000000, 0.000000000000000000, 0.000000000000000000 ) ) ;
#28978=EDGE_CURVE ( 'NONE', #12040, #32985, #29064, .T. ) ;
#28981=CARTESIAN_POINT ( 'NONE',  ( -67.00000337463102085, 43.30127018922198801, -9.999999999999998224 ) ) ;
#28982=CARTESIAN_POINT ( 'NONE',  ( -78.00000337463094979, 34.64101615137757051, -9.999999999999998224 ) ) ;
#28983=ORIENTED_EDGE ( 'NONE', *, *, #12252, .T. ) ;
#28985=AXIS2_PLACEMENT_3D ( 'NONE', #20254, #26049, #23607 ) ;
#28986=DIRECTION ( 'NONE',  ( 1.000000000000000000, 0.000000000000000000, 0.000000000000000000 ) ) ;
#28987=DIRECTION ( 'NONE',  ( 1.000000000000000000, 0.000000000000000000, 0.000000000000000000 ) ) ;
#28990=EDGE_CURVE ( 'NONE', #1755, #6989, #33883, .T. ) ;
#28991=VERTEX_POINT ( 'NONE', #3972 ) ;
#28993=CARTESIAN_POINT ( 'NONE',  ( -51.13139720814437084, -27.49999999999955591, -10.00000000000000000 ) ) ;
#28994=CIRCLE ( 'NONE', #2057, 27.00000000000001421 ) ;
#28996=DIRECTION ( 'NONE',  ( 0.000000000000000000, 0.000000000000000000, 1.000000000000000000 ) ) ;
#28997=ORIENTED_EDGE ( 'NONE', *, *, #35762, .F. ) ;
#28999=ADVANCED_FACE ( 'NONE', ( #15415 ), #9215, .T. ) ;
#29001=DIRECTION ( 'NONE',  ( 0.000000000000000000, 0.000000000000000000, 1.000000000000000000 ) ) ;
#29003=CARTESIAN_POINT ( 'NONE',  ( -3.374631289687624047E-06, -69.28203230275519786, -9.999999999999998224 ) ) ;
#29004=ORIENTED_EDGE ( 'NONE', *, *, #33880, .T. ) ;
#29005=ORIENTED_EDGE ( 'NONE', *, *, #33101, .F. ) ;
#29006=DIRECTION ( 'NONE',  ( 1.000000000000000000, 0.000000000000000000, 0.000000000000000000 ) ) ;
#29007=VECTOR ( 'NONE', #12152, 1000.000000000000000 ) ;
#29008=FACE_OUTER_BOUND ( 'NONE', #16775, .T. ) ;
#29009=AXIS2_PLACEMENT_3D ( 'NONE', #6477, #17909, #29338 ) ;
#29010=FACE_OUTER_BOUND ( 'NONE', #34857, .T. ) ;
#29011=ORIENTED_EDGE ( 'NONE', *, *, #13464, .T. ) ;
#29012=ADVANCED_FACE ( 'NONE', ( #3230 ), #35314, .F. ) ;
#29013=VECTOR ( 'NONE', #8467, 1000.000000000000000 ) ;
#29014=FACE_BOUND ( 'NONE', #1844, .T. ) ;
#29015=ORIENTED_EDGE ( 'NONE', *, *, #24622, .F. ) ;
#29017=EDGE_CURVE ( 'NONE', #630, #7909, #27928, .T. ) ;
#29019=EDGE_LOOP ( 'NONE', ( #12938, #21124, #26907, #24718 ) ) ;
#29020=CIRCLE ( 'NONE', #4508, 3.000000000000002665 ) ;
#29021=AXIS2_PLACEMENT_3D ( 'NONE', #17693, #29128, #26502 ) ;
#29022=FACE_OUTER_BOUND ( 'NONE', #31028, .T. ) ;
#29023=CARTESIAN_POINT ( 'NONE',  ( 49.99999662536846756, 69.28203230275516944, -5.000000000000000000 ) ) ;
#29024=ORIENTED_EDGE ( 'NONE', *, *, #28219, .F. ) ;
#29027=VERTEX_POINT ( 'NONE', #29089 ) ;
#29028=ORIENTED_EDGE ( 'NONE', *, *, #25934, .T. ) ;
#29031=AXIS2_PLACEMENT_3D ( 'NONE', #22597, #27836, #7805 ) ;
#29032=CYLINDRICAL_SURFACE ( 'NONE', #4467, 2.000000000000001776 ) ;
#29033=DIRECTION ( 'NONE',  ( 0.000000000000000000, 0.000000000000000000, -1.000000000000000000 ) ) ;
#29034=ORIENTED_EDGE ( 'NONE', *, *, #8493, .T. ) ;
#29035=AXIS2_PLACEMENT_3D ( 'NONE', #29643, #9418, #23865 ) ;
#29036=DIRECTION ( 'NONE',  ( 1.000000000000000000, 0.000000000000000000, 0.000000000000000000 ) ) ;
#29038=DIRECTION ( 'NONE',  ( -1.000000000000000000, 0.000000000000000000, 0.000000000000000000 ) ) ;
#29039=AXIS2_PLACEMENT_3D ( 'NONE', #18444, #21054, #9797 ) ;
#29041=CIRCLE ( 'NONE', #12885, 2.000000000000001776 ) ;
#29042=CARTESIAN_POINT ( 'NONE',  ( 69.99999662536838230, -51.96152422706639840, -9.999999999999998224 ) ) ;
#29043=DIRECTION ( 'NONE',  ( 0.000000000000000000, 0.000000000000000000, 1.000000000000000000 ) ) ;
#29044=CARTESIAN_POINT ( 'NONE',  ( -63.00000337463102085, 25.98076211353317433, -5.000000000000000000 ) ) ;
#29046=CYLINDRICAL_SURFACE ( 'NONE', #5310, 2.000000000000001776 ) ;
#29047=DIRECTION ( 'NONE',  ( 0.000000000000000000, 0.000000000000000000, 1.000000000000000000 ) ) ;
#29048=AXIS2_PLACEMENT_3D ( 'NONE', #29710, #31950, #15484 ) ;
#29049=AXIS2_PLACEMENT_3D ( 'NONE', #16247, #36500, #28040 ) ;
#29050=ORIENTED_EDGE ( 'NONE', *, *, #22045, .T. ) ;
#29052=VERTEX_POINT ( 'NONE', #3614 ) ;
#29053=ADVANCED_FACE ( 'NONE', ( #12191 ), #972, .F. ) ;
#29054=CARTESIAN_POINT ( 'NONE',  ( -3.374631334790434423E-06, 69.28203230275516944, 17.49999999999999645 ) ) ;
#29055=DIRECTION ( 'NONE',  ( 1.000000000000000000, 0.000000000000000000, 0.000000000000000000 ) ) ;
#29056=DIRECTION ( 'NONE',  ( 0.000000000000000000, 0.000000000000000000, -1.000000000000000000 ) ) ;
#29058=CYLINDRICAL_SURFACE ( 'NONE', #28657, 2.000000000000001776 ) ;
#29059=ORIENTED_EDGE ( 'NONE', *, *, #1869, .T. ) ;
#29061=ADVANCED_FACE ( 'NONE', ( #4174 ), #18974, .F. ) ;
#29062=CARTESIAN_POINT ( 'NONE',  ( -18.00000337463124467, 69.28203230275516944, -9.999999999999998224 ) ) ;
#29063=CARTESIAN_POINT ( 'NONE',  ( -70.00000337463102085, -34.64101615137762025, 17.49999999999999645 ) ) ;
#29064=CIRCLE ( 'NONE', #12905, 1.999999999999998224 ) ;
#29068=DIRECTION ( 'NONE',  ( 0.000000000000000000, 0.000000000000000000, 1.000000000000000000 ) ) ;
#29069=ORIENTED_EDGE ( 'NONE', *, *, #35094, .F. ) ;
#29070=AXIS2_PLACEMENT_3D ( 'NONE', #5980, #33977, #22853 ) ;
#29071=CIRCLE ( 'NONE', #15324, 2.000000000000001776 ) ;
#29072=CIRCLE ( 'NONE', #15927, 65.00000000000000000 ) ;
#29074=CIRCLE ( 'NONE', #27881, 3.499999999999989342 ) ;
#29075=CARTESIAN_POINT ( 'NONE',  ( 56.74224907229030634, -68.66839587347224949, -49.22241343995298024 ) ) ;
#29076=CARTESIAN_POINT ( 'NONE',  ( 44.99999662536849598, -77.94228634059960825, 12.50000000000000000 ) ) ;
#29077=VERTEX_POINT ( 'NONE', #1905 ) ;
#29079=LINE ( 'NONE', #3060, #27348 ) ;
#29080=CARTESIAN_POINT ( 'NONE',  ( -70.00000337463099243, -2.428612866367529932E-14, -9.999999999999998224 ) ) ;
#29081=AXIS2_PLACEMENT_3D ( 'NONE', #8836, #17458, #10653 ) ;
#29082=CARTESIAN_POINT ( 'NONE',  ( 0.000000000000000000, 0.000000000000000000, -5.000000000000000000 ) ) ;
#29083=EDGE_CURVE ( 'NONE', #19786, #19362, #31502, .T. ) ;
#29086=FACE_BOUND ( 'NONE', #32094, .T. ) ;
#29089=CARTESIAN_POINT ( 'NONE',  ( 6.999996625368645198, 77.94228634059957983, -5.000000000000000000 ) ) ;
#29090=CARTESIAN_POINT ( 'NONE',  ( 84.99999662536831124, -8.660254037844397956, -5.000000000000000000 ) ) ;
#29091=CIRCLE ( 'NONE', #32716, 33.00000000000001421 ) ;
#29092=FACE_OUTER_BOUND ( 'NONE', #28250, .T. ) ;
#29095=EDGE_LOOP ( 'NONE', ( #35365, #19719 ) ) ;
#29096=DIRECTION ( 'NONE',  ( 0.000000000000000000, 0.000000000000000000, -1.000000000000000000 ) ) ;
#29098=CARTESIAN_POINT ( 'NONE',  ( -56.67878100130369035, 27.78182860042797131, 12.49999999999999822 ) ) ;
#29099=CARTESIAN_POINT ( 'NONE',  ( 42.99999662536850309, -60.62177826491080168, 12.50000000000000000 ) ) ;
#29101=CIRCLE ( 'NONE', #10574, 27.00000000000001421 ) ;
#29102=CIRCLE ( 'NONE', #36301, 33.00000000000001421 ) ;
#29103=ORIENTED_EDGE ( 'NONE', *, *, #29524, .F. ) ;
#29104=CIRCLE ( 'NONE', #1576, 33.00000000000001421 ) ;
#29105=VERTEX_POINT ( 'NONE', #30401 ) ;
#29106=AXIS2_PLACEMENT_3D ( 'NONE', #12185, #35103, #32276 ) ;
#29107=ADVANCED_FACE ( 'NONE', ( #9775 ), #32644, .F. ) ;
#29108=ORIENTED_EDGE ( 'NONE', *, *, #11468, .T. ) ;
#29109=CARTESIAN_POINT ( 'NONE',  ( -65.00000337463104927, -25.98076211353322051, 17.49999999999999645 ) ) ;
#29111=EDGE_CURVE ( 'NONE', #31389, #18535, #21604, .T. ) ;
#29112=DIRECTION ( 'NONE',  ( 1.000000000000000000, 0.000000000000000000, 0.000000000000000000 ) ) ;
#29114=ORIENTED_EDGE ( 'NONE', *, *, #35762, .T. ) ;
#29115=EDGE_CURVE ( 'NONE', #7710, #34867, #36043, .T. ) ;
#29116=CARTESIAN_POINT ( 'NONE',  ( -70.00000337463102085, -34.64101615137762025, -5.000000000000000000 ) ) ;
#29117=ORIENTED_EDGE ( 'NONE', *, *, #26872, .T. ) ;
#29118=FACE_OUTER_BOUND ( 'NONE', #28448, .T. ) ;
#29119=ORIENTED_EDGE ( 'NONE', *, *, #22390, .F. ) ;
#29122=ORIENTED_EDGE ( 'NONE', *, *, #20359, .T. ) ;
#29124=CIRCLE ( 'NONE', #28539, 2.000000000000001776 ) ;
#29125=ORIENTED_EDGE ( 'NONE', *, *, #22942, .F. ) ;
#29128=DIRECTION ( 'NONE',  ( 0.000000000000000000, 0.000000000000000000, -1.000000000000000000 ) ) ;
#29129=ORIENTED_EDGE ( 'NONE', *, *, #1221, .T. ) ;
#29131=CARTESIAN_POINT ( 'NONE',  ( -13.00000337463126066, 77.94228634059957983, 12.50000000000000000 ) ) ;
#29132=AXIS2_PLACEMENT_3D ( 'NONE', #32558, #7264, #9702 ) ;
#29133=ADVANCED_FACE ( 'NONE', ( #30201 ), #15605, .F. ) ;
#29134=CIRCLE ( 'NONE', #33947, 2.000000000000001776 ) ;
#29136=EDGE_CURVE ( 'NONE', #31157, #23602, #18610, .T. ) ;
#29138=CIRCLE ( 'NONE', #30324, 2.000000000000001776 ) ;
#29139=EDGE_CURVE ( 'NONE', #18222, #4910, #4733, .T. ) ;
#29140=VERTEX_POINT ( 'NONE', #27026 ) ;
#29141=DIRECTION ( 'NONE',  ( 0.000000000000000000, 0.000000000000000000, -1.000000000000000000 ) ) ;
#29142=DIRECTION ( 'NONE',  ( 1.000000000000000000, 0.000000000000000000, 0.000000000000000000 ) ) ;
#29143=EDGE_CURVE ( 'NONE', #20167, #20440, #16170, .T. ) ;
#29144=ORIENTED_EDGE ( 'NONE', *, *, #36539, .F. ) ;
#29145=DIRECTION ( 'NONE',  ( 0.000000000000000000, 0.000000000000000000, 1.000000000000000000 ) ) ;
#29147=CYLINDRICAL_SURFACE ( 'NONE', #23185, 2.000000000000001776 ) ;
#29148=CARTESIAN_POINT ( 'NONE',  ( 0.000000000000000000, 0.000000000000000000, -5.000000000000000000 ) ) ;
#29149=AXIS2_PLACEMENT_3D ( 'NONE', #35510, #19002, #4205 ) ;
#29150=DIRECTION ( 'NONE',  ( 1.000000000000000000, 0.000000000000000000, 0.000000000000000000 ) ) ;
#29152=EDGE_LOOP ( 'NONE', ( #2913, #3723 ) ) ;
#29154=CARTESIAN_POINT ( 'NONE',  ( -67.00000337463102085, 25.98076211353317433, -9.999999999999998224 ) ) ;
#29155=DIRECTION ( 'NONE',  ( 0.000000000000000000, 0.000000000000000000, 1.000000000000000000 ) ) ;
#29158=ORIENTED_EDGE ( 'NONE', *, *, #35203, .T. ) ;
#29160=CIRCLE ( 'NONE', #10036, 2.000000000000001776 ) ;
#29161=AXIS2_PLACEMENT_3D ( 'NONE', #35474, #6206, #29625 ) ;
#29163=DIRECTION ( 'NONE',  ( 0.000000000000000000, 0.000000000000000000, 1.000000000000000000 ) ) ;
#29165=DIRECTION ( 'NONE',  ( 0.000000000000000000, 0.000000000000000000, 1.000000000000000000 ) ) ;
#29166=VECTOR ( 'NONE', #34047, 1000.000000000000000 ) ;
#29167=AXIS2_PLACEMENT_3D ( 'NONE', #14821, #17076, #25724 ) ;
#29169=FACE_OUTER_BOUND ( 'NONE', #26758, .T. ) ;
#29170=EDGE_LOOP ( 'NONE', ( #11055, #4219 ) ) ;
#29171=DIRECTION ( 'NONE',  ( 0.000000000000000000, 0.000000000000000000, 1.000000000000000000 ) ) ;
#29173=FACE_BOUND ( 'NONE', #26095, .T. ) ;
#29176=CARTESIAN_POINT ( 'NONE',  ( -40.00000337463113453, 69.28203230275516944, 17.49999999999999645 ) ) ;
#29179=DIRECTION ( 'NONE',  ( 1.000000000000000000, 0.000000000000000000, 0.000000000000000000 ) ) ;
#29180=AXIS2_PLACEMENT_3D ( 'NONE', #4943, #25025, #30795 ) ;
#29182=CIRCLE ( 'NONE', #18412, 2.000000000000000000 ) ;
#29183=CARTESIAN_POINT ( 'NONE',  ( 62.19434990244976547, -52.39915983220758022, -49.22241343995298024 ) ) ;
#29184=CYLINDRICAL_SURFACE ( 'NONE', #19783, 2.000000000000001776 ) ;
#29185=CARTESIAN_POINT ( 'NONE',  ( 62.99999662536841072, -25.98076211353320275, -9.999999999999998224 ) ) ;
#29187=VERTEX_POINT ( 'NONE', #30591 ) ;
#29188=CARTESIAN_POINT ( 'NONE',  ( -56.67878100130369035, 27.78182860042797131, 12.49999999999999822 ) ) ;
#29189=DIRECTION ( 'NONE',  ( 0.000000000000000000, 0.000000000000000000, 1.000000000000000000 ) ) ;
#29190=DIRECTION ( 'NONE',  ( 0.000000000000000000, 0.000000000000000000, 1.000000000000000000 ) ) ;
#29191=AXIS2_PLACEMENT_3D ( 'NONE', #5432, #3151, #1231 ) ;
#29192=EDGE_LOOP ( 'NONE', ( #10119, #4136, #27355, #33873 ) ) ;
#29193=AXIS2_PLACEMENT_3D ( 'NONE', #36068, #21798, #10555 ) ;
#29194=VERTEX_POINT ( 'NONE', #35859 ) ;
#29195=ORIENTED_EDGE ( 'NONE', *, *, #33880, .F. ) ;
#29196=DIRECTION ( 'NONE',  ( 1.000000000000000000, 0.000000000000000000, 0.000000000000000000 ) ) ;
#29197=DIRECTION ( 'NONE',  ( -1.000000000000000000, 0.000000000000000000, 0.000000000000000000 ) ) ;
#29198=CIRCLE ( 'NONE', #26213, 2.000000000000000000 ) ;
#29199=DIRECTION ( 'NONE',  ( 1.000000000000000000, 0.000000000000000000, 0.000000000000000000 ) ) ;
#29200=CARTESIAN_POINT ( 'NONE',  ( 66.50937412064257614, -41.98910420248104458, -5.000000000000000000 ) ) ;
#29202=VECTOR ( 'NONE', #28064, 1000.000000000000000 ) ;
#29203=VECTOR ( 'NONE', #410, 1000.000000000000000 ) ;
#29205=CARTESIAN_POINT ( 'NONE',  ( 9.999996625368655856, -86.60254037844400443, -9.999999999999998224 ) ) ;
#29206=ADVANCED_FACE ( 'NONE', ( #2075 ), #13512, .F. ) ;
#29207=EDGE_LOOP ( 'NONE', ( #23900, #9121 ) ) ;
#29209=ORIENTED_EDGE ( 'NONE', *, *, #3213, .T. ) ;
#29210=CARTESIAN_POINT ( 'NONE',  ( -23.00000337463121980, -77.94228634059963667, 12.50000000000000000 ) ) ;
#29211=VECTOR ( 'NONE', #35068, 1000.000000000000000 ) ;
#29212=CARTESIAN_POINT ( 'NONE',  ( -75.00000337463097821, 8.660254037844374864, -5.000000000000000000 ) ) ;
#29213=DIRECTION ( 'NONE',  ( -1.000000000000000000, 0.000000000000000000, -0.000000000000000000 ) ) ;
#29214=ORIENTED_EDGE ( 'NONE', *, *, #326, .T. ) ;
#29215=VECTOR ( 'NONE', #36565, 1000.000000000000000 ) ;
#29216=EDGE_CURVE ( 'NONE', #34250, #15061, #22527, .T. ) ;
#29217=FACE_BOUND ( 'NONE', #7795, .T. ) ;
#29218=EDGE_LOOP ( 'NONE', ( #15006, #2424, #27031, #27603 ) ) ;
#29219=ORIENTED_EDGE ( 'NONE', *, *, #30269, .F. ) ;
#29221=ORIENTED_EDGE ( 'NONE', *, *, #29463, .F. ) ;
#29222=VECTOR ( 'NONE', #32980, 1000.000000000000000 ) ;
#29224=DIRECTION ( 'NONE',  ( 1.000000000000000000, 0.000000000000000000, 0.000000000000000000 ) ) ;
#29225=AXIS2_PLACEMENT_3D ( 'NONE', #14300, #10918, #5492 ) ;
#29226=DIRECTION ( 'NONE',  ( -1.000000000000000000, 0.000000000000000000, 0.000000000000000000 ) ) ;
#29227=FACE_BOUND ( 'NONE', #32834, .T. ) ;
#29228=EDGE_CURVE ( 'NONE', #2201, #4900, #10890, .T. ) ;
#29230=EDGE_LOOP ( 'NONE', ( #5635, #978 ) ) ;
#29231=CIRCLE ( 'NONE', #34052, 33.00000000000001421 ) ;
#29233=AXIS2_PLACEMENT_3D ( 'NONE', #25248, #28048, #27846 ) ;
#29234=ORIENTED_EDGE ( 'NONE', *, *, #8054, .F. ) ;
#29237=DIRECTION ( 'NONE',  ( 1.000000000000000000, 0.000000000000000000, 0.000000000000000000 ) ) ;
#29238=DIRECTION ( 'NONE',  ( 1.000000000000000000, 0.000000000000000000, 0.000000000000000000 ) ) ;
#29239=ORIENTED_EDGE ( 'NONE', *, *, #7657, .F. ) ;
#29241=CARTESIAN_POINT ( 'NONE',  ( 11.99999662536861855, 69.28203230275516944, -9.999999999999998224 ) ) ;
#29242=CARTESIAN_POINT ( 'NONE',  ( 49.99999662536846756, 69.28203230275516944, -9.999999999999998224 ) ) ;
#29244=DIRECTION ( 'NONE',  ( 0.000000000000000000, 0.000000000000000000, 1.000000000000000000 ) ) ;
#29245=AXIS2_PLACEMENT_3D ( 'NONE', #18461, #15080, #4015 ) ;
#29246=CARTESIAN_POINT ( 'NONE',  ( 27.99999662536855993, 69.28203230275518365, 17.49999999999999645 ) ) ;
#29247=EDGE_CURVE ( 'NONE', #8519, #36949, #24323, .T. ) ;
#29248=CARTESIAN_POINT ( 'NONE',  ( 69.99999662536839651, -17.32050807568879947, -9.999999999999998224 ) ) ;
#29250=CARTESIAN_POINT ( 'NONE',  ( -76.71706625813334313, 9.685775882613420151, -5.000000000000000000 ) ) ;
#29251=FACE_OUTER_BOUND ( 'NONE', #11532, .T. ) ;
#29253=EDGE_LOOP ( 'NONE', ( #17989, #27395, #15349, #28475 ) ) ;
#29255=CARTESIAN_POINT ( 'NONE',  ( 52.99999662536844625, 60.62177826491077326, 17.49999999999999645 ) ) ;
#29256=VECTOR ( 'NONE', #36754, 1000.000000000000000 ) ;
#29257=CARTESIAN_POINT ( 'NONE',  ( -70.00000337463099243, 51.96152422706637708, 12.50000000000000000 ) ) ;
#29259=CARTESIAN_POINT ( 'NONE',  ( -58.48108235278846934, -36.97203788309005290, -4.999999999999997335 ) ) ;
#29260=EDGE_CURVE ( 'NONE', #12727, #35025, #376, .T. ) ;
#29261=VERTEX_POINT ( 'NONE', #28500 ) ;
#29262=DIRECTION ( 'NONE',  ( 0.000000000000000000, 0.000000000000000000, 1.000000000000000000 ) ) ;
#29263=DIRECTION ( 'NONE',  ( 0.000000000000000000, 0.000000000000000000, -1.000000000000000000 ) ) ;
#29264=EDGE_CURVE ( 'NONE', #33654, #14526, #20144, .T. ) ;
#29266=AXIS2_PLACEMENT_3D ( 'NONE', #25395, #4798, #21837 ) ;
#29267=CARTESIAN_POINT ( 'NONE',  ( -3.000003374631308173, 77.94228634059957983, -9.999999999999998224 ) ) ;
#29268=VERTEX_POINT ( 'NONE', #14062 ) ;
#29269=AXIS2_PLACEMENT_3D ( 'NONE', #1494, #12929, #24389 ) ;
#29270=DIRECTION ( 'NONE',  ( 0.000000000000000000, 0.000000000000000000, 1.000000000000000000 ) ) ;
#29273=DIRECTION ( 'NONE',  ( 1.000000000000000000, 0.000000000000000000, 0.000000000000000000 ) ) ;
#29275=AXIS2_PLACEMENT_3D ( 'NONE', #14535, #34970, #832 ) ;
#29276=ORIENTED_EDGE ( 'NONE', *, *, #13487, .T. ) ;
#29277=FACE_OUTER_BOUND ( 'NONE', #30266, .T. ) ;
#29279=DIRECTION ( 'NONE',  ( 0.000000000000000000, 0.000000000000000000, 1.000000000000000000 ) ) ;
#29280=ADVANCED_FACE ( 'NONE', ( #12 ), #22713, .T. ) ;
#29281=VERTEX_POINT ( 'NONE', #8083 ) ;
#29282=DIRECTION ( 'NONE',  ( 0.000000000000000000, 0.000000000000000000, 1.000000000000000000 ) ) ;
#29283=FACE_BOUND ( 'NONE', #13161, .T. ) ;
#29287=ORIENTED_EDGE ( 'NONE', *, *, #26871, .F. ) ;
#29288=CARTESIAN_POINT ( 'NONE',  ( -17.00000337463125533, -77.94228634059960825, -5.000000000000000000 ) ) ;
#29290=CARTESIAN_POINT ( 'NONE',  ( 77.99999662536832545, -17.32050807568879591, -9.999999999999998224 ) ) ;
#29291=AXIS2_PLACEMENT_3D ( 'NONE', #26920, #26725, #1044 ) ;
#29294=VERTEX_POINT ( 'NONE', #2834 ) ;
#29295=DIRECTION ( 'NONE',  ( 1.000000000000000000, 0.000000000000000000, 0.000000000000000000 ) ) ;
#29296=CARTESIAN_POINT ( 'NONE',  ( 0.000000000000000000, 0.000000000000000000, 12.49999999999999822 ) ) ;
#29297=CARTESIAN_POINT ( 'NONE',  ( -48.00000337463112032, -51.96152422706641971, -9.999999999999998224 ) ) ;
#29298=AXIS2_PLACEMENT_3D ( 'NONE', #34815, #3502, #4051 ) ;
#29299=VERTEX_POINT ( 'NONE', #33773 ) ;
#29300=VERTEX_POINT ( 'NONE', #19338 ) ;
#29302=VERTEX_POINT ( 'NONE', #19523 ) ;
#29303=CYLINDRICAL_SURFACE ( 'NONE', #982, 2.000000000000001776 ) ;
#29304=LINE ( 'NONE', #23881, #18765 ) ;
#29305=AXIS2_PLACEMENT_3D ( 'NONE', #4591, #7578, #19028 ) ;
#29306=CARTESIAN_POINT ( 'NONE',  ( 25.30168577890723469, -79.91940132325416357, 12.50000000000000000 ) ) ;
#29308=ORIENTED_EDGE ( 'NONE', *, *, #2088, .F. ) ;
#29309=VERTEX_POINT ( 'NONE', #22887 ) ;
#29310=FACE_OUTER_BOUND ( 'NONE', #4685, .T. ) ;
#29312=ORIENTED_EDGE ( 'NONE', *, *, #26125, .F. ) ;
#29313=CYLINDRICAL_SURFACE ( 'NONE', #17377, 3.499999999999991562 ) ;
#29315=AXIS2_PLACEMENT_3D ( 'NONE', #29974, #7109, #10844 ) ;
#29317=ORIENTED_EDGE ( 'NONE', *, *, #30157, .F. ) ;
#29318=VERTEX_POINT ( 'NONE', #16891 ) ;
#29320=FACE_BOUND ( 'NONE', #19019, .T. ) ;
#29321=DIRECTION ( 'NONE',  ( 1.000000000000000000, 0.000000000000000000, 0.000000000000000000 ) ) ;
#29322=ORIENTED_EDGE ( 'NONE', *, *, #17911, .T. ) ;
#29323=VERTEX_POINT ( 'NONE', #28311 ) ;
#29324=DIRECTION ( 'NONE',  ( 0.000000000000000000, 0.000000000000000000, 1.000000000000000000 ) ) ;
#29325=CARTESIAN_POINT ( 'NONE',  ( 51.67316999614278217, 68.18636315956837279, -5.000000000000000000 ) ) ;
#29327=AXIS2_PLACEMENT_3D ( 'NONE', #6582, #1139, #35637 ) ;
#29328=ADVANCED_FACE ( 'NONE', ( #25516 ), #20995, .F. ) ;
#29330=CARTESIAN_POINT ( 'NONE',  ( 49.99999662536848177, -51.96152422706640550, -9.999999999999998224 ) ) ;
#29331=DIRECTION ( 'NONE',  ( -1.000000000000000000, 0.000000000000000000, 0.000000000000000000 ) ) ;
#29332=EDGE_LOOP ( 'NONE', ( #7629, #31341, #30051, #35770, #29406, #33711 ) ) ;
#29334=EDGE_CURVE ( 'NONE', #14823, #1054, #32025, .T. ) ;
#29335=DIRECTION ( 'NONE',  ( 0.000000000000000000, 0.000000000000000000, 1.000000000000000000 ) ) ;
#29336=LINE ( 'NONE', #3477, #15999 ) ;
#29337=DIRECTION ( 'NONE',  ( 0.000000000000000000, 0.000000000000000000, -1.000000000000000000 ) ) ;
#29338=DIRECTION ( 'NONE',  ( -1.000000000000000000, -5.139921410301647641E-15, 0.000000000000000000 ) ) ;
#29342=CARTESIAN_POINT ( 'NONE',  ( -2.000003374631334818, 69.28203230275516944, -9.999999999999998224 ) ) ;
#29344=CARTESIAN_POINT ( 'NONE',  ( -19.13981058454750794, 60.93295298010998806, 12.49999999999999822 ) ) ;
#29345=EDGE_CURVE ( 'NONE', #30962, #6801, #3741, .T. ) ;
#29346=AXIS2_PLACEMENT_3D ( 'NONE', #11520, #36670, #10969 ) ;
#29347=CARTESIAN_POINT ( 'NONE',  ( 84.99999662536831124, -8.660254037844397956, -5.000000000000000000 ) ) ;
#29348=PLANE ( 'NONE',  #11582 ) ;
#29350=ORIENTED_EDGE ( 'NONE', *, *, #2747, .T. ) ;
#29353=DIRECTION ( 'NONE',  ( 1.000000000000000000, 0.000000000000000000, 0.000000000000000000 ) ) ;
#29354=DIRECTION ( 'NONE',  ( 0.000000000000000000, 0.000000000000000000, -1.000000000000000000 ) ) ;
#29358=DIRECTION ( 'NONE',  ( 1.000000000000000000, 0.000000000000000000, 0.000000000000000000 ) ) ;
#29359=EDGE_CURVE ( 'NONE', #21552, #6546, #2781, .T. ) ;
#29362=CIRCLE ( 'NONE', #13798, 2.000000000000001776 ) ;
#29364=CARTESIAN_POINT ( 'NONE',  ( 36.99999662536855283, -77.94228634059960825, 12.50000000000000000 ) ) ;
#29366=FACE_BOUND ( 'NONE', #19359, .T. ) ;
#29368=DIRECTION ( 'NONE',  ( 1.000000000000000000, 0.000000000000000000, 0.000000000000000000 ) ) ;
#29369=DIRECTION ( 'NONE',  ( -1.000000000000000000, 0.000000000000000000, 0.000000000000000000 ) ) ;
#29370=EDGE_LOOP ( 'NONE', ( #30289, #4121, #33874 ) ) ;
#29371=LINE ( 'NONE', #6302, #10479 ) ;
#29373=FACE_OUTER_BOUND ( 'NONE', #23871, .T. ) ;
#29375=DIRECTION ( 'NONE',  ( -1.000000000000000000, 0.000000000000000000, 0.000000000000000000 ) ) ;
#29376=DIRECTION ( 'NONE',  ( 0.000000000000000000, 0.000000000000000000, -1.000000000000000000 ) ) ;
#29377=EDGE_LOOP ( 'NONE', ( #19980, #24655 ) ) ;
#29378=FACE_OUTER_BOUND ( 'NONE', #16472, .T. ) ;
#29379=CARTESIAN_POINT ( 'NONE',  ( -62.00000337463108480, -51.96152422706641971, -9.999999999999998224 ) ) ;
#29381=EDGE_LOOP ( 'NONE', ( #18876, #11034 ) ) ;
#29382=VERTEX_POINT ( 'NONE', #12150 ) ;
#29384=ORIENTED_EDGE ( 'NONE', *, *, #475, .T. ) ;
#29385=EDGE_CURVE ( 'NONE', #24271, #10050, #31531, .T. ) ;
#29387=CARTESIAN_POINT ( 'NONE',  ( 79.99999662536832545, -34.64101615137759183, 17.49999999999999645 ) ) ;
#29389=PLANE ( 'NONE',  #14598 ) ;
#29390=CARTESIAN_POINT ( 'NONE',  ( -75.00000337463100664, -43.30127018922202353, -9.999999999999998224 ) ) ;
#29391=CARTESIAN_POINT ( 'NONE',  ( -10.00000337463128730, 69.28203230275516944, -5.000000000000000000 ) ) ;
#29394=ORIENTED_EDGE ( 'NONE', *, *, #943, .F. ) ;
#29395=DIRECTION ( 'NONE',  ( 1.000000000000000000, 0.000000000000000000, 0.000000000000000000 ) ) ;
#29396=EDGE_CURVE ( 'NONE', #15480, #22341, #28543, .T. ) ;
#29397=CARTESIAN_POINT ( 'NONE',  ( 31.46585318596250502, 86.45172111230321832, 12.49999999999999822 ) ) ;
#29398=ORIENTED_EDGE ( 'NONE', *, *, #8976, .F. ) ;
#29400=DIRECTION ( 'NONE',  ( -1.000000000000000000, 0.000000000000000000, 0.000000000000000000 ) ) ;
#29401=ORIENTED_EDGE ( 'NONE', *, *, #20194, .T. ) ;
#29402=FACE_BOUND ( 'NONE', #31136, .T. ) ;
#29404=ORIENTED_EDGE ( 'NONE', *, *, #461, .F. ) ;
#29405=DIRECTION ( 'NONE',  ( 0.000000000000000000, 0.000000000000000000, 1.000000000000000000 ) ) ;
#29406=ORIENTED_EDGE ( 'NONE', *, *, #3445, .T. ) ;
#29408=CARTESIAN_POINT ( 'NONE',  ( -33.00000337463117006, -77.94228634059963667, -9.999999999999998224 ) ) ;
#29411=ORIENTED_EDGE ( 'NONE', *, *, #11488, .T. ) ;
#29412=ORIENTED_EDGE ( 'NONE', *, *, #27046, .T. ) ;
#29413=EDGE_LOOP ( 'NONE', ( #29445, #5064 ) ) ;
#29414=EDGE_CURVE ( 'NONE', #2651, #8103, #33348, .T. ) ;
#29416=ORIENTED_EDGE ( 'NONE', *, *, #10160, .T. ) ;
#29417=CARTESIAN_POINT ( 'NONE',  ( -20.00000337463123756, -69.28203230275522628, -9.999999999999998224 ) ) ;
#29418=AXIS2_PLACEMENT_3D ( 'NONE', #25798, #34407, #20500 ) ;
#29419=LINE ( 'NONE', #3737, #7806 ) ;
#29420=VERTEX_POINT ( 'NONE', #14445 ) ;
#29421=AXIS2_PLACEMENT_3D ( 'NONE', #2047, #32822, #13481 ) ;
#29422=CARTESIAN_POINT ( 'NONE',  ( 77.99999662536833966, 17.32050807568879236, 17.49999999999999645 ) ) ;
#29423=LINE ( 'NONE', #29241, #4940 ) ;
#29425=ORIENTED_EDGE ( 'NONE', *, *, #32369, .F. ) ;
#29426=DIRECTION ( 'NONE',  ( 1.000000000000000000, 0.000000000000000000, 0.000000000000000000 ) ) ;
#29427=DIRECTION ( 'NONE',  ( 1.000000000000000000, 0.000000000000000000, 0.000000000000000000 ) ) ;
#29428=DIRECTION ( 'NONE',  ( 0.000000000000000000, 0.000000000000000000, 1.000000000000000000 ) ) ;
#29429=ORIENTED_EDGE ( 'NONE', *, *, #18194, .F. ) ;
#29431=LINE ( 'NONE', #32997, #8799 ) ;
#29432=ORIENTED_EDGE ( 'NONE', *, *, #19076, .T. ) ;
#29433=ORIENTED_EDGE ( 'NONE', *, *, #24172, .F. ) ;
#29434=FACE_OUTER_BOUND ( 'NONE', #15810, .T. ) ;
#29435=DIRECTION ( 'NONE',  ( -1.000000000000000000, 0.000000000000000000, 0.000000000000000000 ) ) ;
#29436=ADVANCED_FACE ( 'NONE', ( #17607 ), #11797, .F. ) ;
#29437=DIRECTION ( 'NONE',  ( 0.000000000000000000, 0.000000000000000000, -1.000000000000000000 ) ) ;
#29438=LINE ( 'NONE', #11999, #16684 ) ;
#29439=ORIENTED_EDGE ( 'NONE', *, *, #29083, .F. ) ;
#29441=DIRECTION ( 'NONE',  ( 1.000000000000000000, 0.000000000000000000, 0.000000000000000000 ) ) ;
#29442=EDGE_LOOP ( 'NONE', ( #27770, #7197, #21183, #34741, #33039, #22165, #8695, #4766, #15220, #13600 ) ) ;
#29444=CYLINDRICAL_SURFACE ( 'NONE', #27391, 3.000000000000002665 ) ;
#29445=ORIENTED_EDGE ( 'NONE', *, *, #33976, .T. ) ;
#29446=CARTESIAN_POINT ( 'NONE',  ( 36.99999662536855283, 60.62177826491078747, -9.999999999999998224 ) ) ;
#29447=CARTESIAN_POINT ( 'NONE',  ( 56.67878100130369035, -27.78182860042797131, 12.49999999999999822 ) ) ;
#29448=FACE_OUTER_BOUND ( 'NONE', #25325, .T. ) ;
#29450=ORIENTED_EDGE ( 'NONE', *, *, #24308, .F. ) ;
#29451=EDGE_CURVE ( 'NONE', #8999, #36648, #21969, .T. ) ;
#29453=ORIENTED_EDGE ( 'NONE', *, *, #2433, .T. ) ;
#29454=CARTESIAN_POINT ( 'NONE',  ( -55.00000337463109901, -60.62177826491083010, -5.000000000000000000 ) ) ;
#29455=PLANE ( 'NONE',  #23949 ) ;
#29456=EDGE_CURVE ( 'NONE', #36578, #245, #4608, .T. ) ;
#29458=CARTESIAN_POINT ( 'NONE',  ( 52.99999662536844625, 43.30127018922198801, 17.49999999999999645 ) ) ;
#29459=DIRECTION ( 'NONE',  ( 1.000000000000000000, 0.000000000000000000, 0.000000000000000000 ) ) ;
#29460=VERTEX_POINT ( 'NONE', #36174 ) ;
#29461=DIRECTION ( 'NONE',  ( 0.000000000000000000, 0.000000000000000000, 1.000000000000000000 ) ) ;
#29462=DIRECTION ( 'NONE',  ( -0.000000000000000000, 0.000000000000000000, -1.000000000000000000 ) ) ;
#29463=EDGE_CURVE ( 'NONE', #3619, #6911, #35735, .T. ) ;
#29464=CIRCLE ( 'NONE', #13312, 2.000000000000001776 ) ;
#29466=FACE_OUTER_BOUND ( 'NONE', #9517, .T. ) ;
#29467=CARTESIAN_POINT ( 'NONE',  ( 31.02796211690949235, -59.29837256189548356, 12.49999999999999645 ) ) ;
#29468=CARTESIAN_POINT ( 'NONE',  ( -45.00000337463111322, -77.94228634059960825, 17.49999999999999645 ) ) ;
#29469=VERTEX_POINT ( 'NONE', #12912 ) ;
#29470=ORIENTED_EDGE ( 'NONE', *, *, #3301, .T. ) ;
#29472=ADVANCED_FACE ( 'NONE', ( #36003 ), #15563, .F. ) ;
#29473=DIRECTION ( 'NONE',  ( 0.000000000000000000, 0.000000000000000000, 1.000000000000000000 ) ) ;
#29475=ORIENTED_EDGE ( 'NONE', *, *, #20152, .F. ) ;
#29476=ORIENTED_EDGE ( 'NONE', *, *, #11592, .T. ) ;
#29477=ORIENTED_EDGE ( 'NONE', *, *, #16679, .T. ) ;
#29478=DIRECTION ( 'NONE',  ( 1.000000000000000000, 0.000000000000000000, 0.000000000000000000 ) ) ;
#29479=AXIS2_PLACEMENT_3D ( 'NONE', #24057, #18224, #21225 ) ;
#29480=VERTEX_POINT ( 'NONE', #27559 ) ;
#29482=ORIENTED_EDGE ( 'NONE', *, *, #20401, .T. ) ;
#29483=DIRECTION ( 'NONE',  ( 0.000000000000000000, 0.000000000000000000, 1.000000000000000000 ) ) ;
#29484=ORIENTED_EDGE ( 'NONE', *, *, #5186, .T. ) ;
#29485=VERTEX_POINT ( 'NONE', #13118 ) ;
#29486=ADVANCED_FACE ( 'NONE', ( #33365 ), #9735, .F. ) ;
#29487=FILL_AREA_STYLE ('',( #33393 ) ) ;
#29489=CIRCLE ( 'NONE', #21713, 2.000000000000001776 ) ;
#29490=ADVANCED_FACE ( 'NONE', ( #4488 ), #30161, .F. ) ;
#29492=VERTEX_POINT ( 'NONE', #12549 ) ;
#29493=VECTOR ( 'NONE', #2517, 1000.000000000000000 ) ;
#29494=ORIENTED_EDGE ( 'NONE', *, *, #25063, .T. ) ;
#29496=DIRECTION ( 'NONE',  ( -1.000000000000000000, 0.000000000000000000, 0.000000000000000000 ) ) ;
#29498=CARTESIAN_POINT ( 'NONE',  ( 68.66839587347284635, 56.74224907228958870, -49.22241343995293761 ) ) ;
#29499=CARTESIAN_POINT ( 'NONE',  ( -40.00000337463113453, -69.28203230275519786, -5.000000000000000000 ) ) ;
#29500=ORIENTED_EDGE ( 'NONE', *, *, #3439, .F. ) ;
#29501=CARTESIAN_POINT ( 'NONE',  ( -80.00000337463094979, -2.428612866367529932E-14, 12.50000000000000000 ) ) ;
#29502=CARTESIAN_POINT ( 'NONE',  ( 51.99999662536847467, 51.96152422706637708, 17.49999999999999645 ) ) ;
#29503=VERTEX_POINT ( 'NONE', #19131 ) ;
#29504=FACE_OUTER_BOUND ( 'NONE', #35995, .T. ) ;
#29505=EDGE_CURVE ( 'NONE', #2973, #29420, #405, .T. ) ;
#29506=CARTESIAN_POINT ( 'NONE',  ( -8.000003374631287301, 69.28203230275516944, 12.50000000000000000 ) ) ;
#29507=CARTESIAN_POINT ( 'NONE',  ( 44.99999662536851019, 77.94228634059959404, 12.50000000000000000 ) ) ;
#29508=LINE ( 'NONE', #18261, #35030 ) ;
#29509=CIRCLE ( 'NONE', #34317, 33.00000000000001421 ) ;
#29511=EDGE_CURVE ( 'NONE', #23723, #15799, #33938, .T. ) ;
#29513=EDGE_LOOP ( 'NONE', ( #6631, #6180 ) ) ;
#29514=CARTESIAN_POINT ( 'NONE',  ( 34.99999662536855283, 60.62177826491078747, -5.000000000000000000 ) ) ;
#29517=ORIENTED_EDGE ( 'NONE', *, *, #25628, .T. ) ;
#29518=EDGE_LOOP ( 'NONE', ( #12070, #11507 ) ) ;
#29520=LINE ( 'NONE', #12650, #34399 ) ;
#29521=DIRECTION ( 'NONE',  ( 0.000000000000000000, 0.000000000000000000, 1.000000000000000000 ) ) ;
#29522=CARTESIAN_POINT ( 'NONE',  ( -20.00000337463124112, 69.28203230275516944, 17.49999999999999645 ) ) ;
#29523=CARTESIAN_POINT ( 'NONE',  ( 56.67878100130369035, -27.78182860042797131, 12.49999999999999822 ) ) ;
#29524=EDGE_CURVE ( 'NONE', #2400, #24065, #27959, .T. ) ;
#29525=CARTESIAN_POINT ( 'NONE',  ( 46.99999662536851019, 77.94228634059959404, -9.999999999999998224 ) ) ;
#29526=ORIENTED_EDGE ( 'NONE', *, *, #7262, .T. ) ;
#29528=EDGE_LOOP ( 'NONE', ( #22149, #23173, #2457, #24771 ) ) ;
#29529=FACE_BOUND ( 'NONE', #9250, .T. ) ;
#29530=CIRCLE ( 'NONE', #17548, 2.000000000000001776 ) ;
#29531=EDGE_CURVE ( 'NONE', #9530, #7637, #17755, .T. ) ;
#29532=AXIS2_PLACEMENT_3D ( 'NONE', #20179, #3342, #26026 ) ;
#29534=EDGE_CURVE ( 'NONE', #16822, #27152, #1007, .T. ) ;
#29536=ADVANCED_FACE ( 'NONE', ( #24171 ), #18370, .F. ) ;
#29539=CARTESIAN_POINT ( 'NONE',  ( 29.99999662536857770, -69.28203230275519786, -9.999999999999998224 ) ) ;
#29540=CIRCLE ( 'NONE', #32521, 2.000000000000001776 ) ;
#29541=DIRECTION ( 'NONE',  ( 1.000000000000000000, 0.000000000000000000, 0.000000000000000000 ) ) ;
#29542=CARTESIAN_POINT ( 'NONE',  ( -70.00000337463099243, 17.32050807568877460, 12.50000000000000000 ) ) ;
#29543=EDGE_LOOP ( 'NONE', ( #512, #13733 ) ) ;
#29544=DIRECTION ( 'NONE',  ( 1.000000000000000000, 0.000000000000000000, 0.000000000000000000 ) ) ;
#29545=CARTESIAN_POINT ( 'NONE',  ( -35.00000337463116296, 60.62177826491077326, 12.50000000000000000 ) ) ;
#29546=DIRECTION ( 'NONE',  ( 0.000000000000000000, 0.000000000000000000, 1.000000000000000000 ) ) ;
#29547=ORIENTED_EDGE ( 'NONE', *, *, #8422, .T. ) ;
#29549=EDGE_CURVE ( 'NONE', #4453, #2973, #26810, .T. ) ;
#29550=ORIENTED_EDGE ( 'NONE', *, *, #21076, .F. ) ;
#29552=DIRECTION ( 'NONE',  ( 1.000000000000000000, 0.000000000000000000, 0.000000000000000000 ) ) ;
#29553=CIRCLE ( 'NONE', #30154, 2.000000000000001776 ) ;
#29554=CARTESIAN_POINT ( 'NONE',  ( 61.53067111003264955, -72.28378166041994746, -49.22241343995298024 ) ) ;
#29555=DIRECTION ( 'NONE',  ( 0.000000000000000000, 0.000000000000000000, 1.000000000000000000 ) ) ;
#29558=ORIENTED_EDGE ( 'NONE', *, *, #23082, .F. ) ;
#29559=VECTOR ( 'NONE', #31876, 1000.000000000000000 ) ;
#29560=ORIENTED_EDGE ( 'NONE', *, *, #10829, .F. ) ;
#29561=DIRECTION ( 'NONE',  ( 1.000000000000000000, 0.000000000000000000, 0.000000000000000000 ) ) ;
#29562=EDGE_CURVE ( 'NONE', #6282, #10243, #34551, .T. ) ;
#29563=( GEOMETRIC_REPRESENTATION_CONTEXT ( 3 ) GLOBAL_UNCERTAINTY_ASSIGNED_CONTEXT ( ( #30573 ) ) GLOBAL_UNIT_ASSIGNED_CONTEXT ( ( #33209, #10526, #7728 ) ) REPRESENTATION_CONTEXT ( 'NONE', 'WORKASPACE' ) );
#29565=ORIENTED_EDGE ( 'NONE', *, *, #16696, .F. ) ;
#29566=EDGE_CURVE ( 'NONE', #15386, #14472, #14760, .T. ) ;
#29567=CARTESIAN_POINT ( 'NONE',  ( 0.000000000000000000, 0.000000000000000000, -5.000000000000000000 ) ) ;
#29568=VERTEX_POINT ( 'NONE', #35623 ) ;
#29569=ADVANCED_FACE ( 'NONE', ( #9920 ), #21365, .F. ) ;
#29570=LINE ( 'NONE', #35604, #11923 ) ;
#29572=ORIENTED_EDGE ( 'NONE', *, *, #29111, .F. ) ;
#29573=EDGE_CURVE ( 'NONE', #34610, #17931, #8791, .T. ) ;
#29574=FACE_OUTER_BOUND ( 'NONE', #11253, .T. ) ;
#29575=ORIENTED_EDGE ( 'NONE', *, *, #14603, .T. ) ;
#29576=EDGE_CURVE ( 'NONE', #22308, #11341, #27340, .T. ) ;
#29577=CIRCLE ( 'NONE', #12797, 2.000000000000001776 ) ;
#29578=DIRECTION ( 'NONE',  ( 0.000000000000000000, 0.000000000000000000, 1.000000000000000000 ) ) ;
#29579=CYLINDRICAL_SURFACE ( 'NONE', #9544, 2.000000000000001776 ) ;
#29580=CARTESIAN_POINT ( 'NONE',  ( 69.99999662536841072, 51.96152422706640550, 17.49999999999999645 ) ) ;
#29581=EDGE_LOOP ( 'NONE', ( #10456, #25752, #20505, #17473 ) ) ;
#29585=VERTEX_POINT ( 'NONE', #16674 ) ;
#29587=CIRCLE ( 'NONE', #2058, 27.00000000000001421 ) ;
#29588=EDGE_CURVE ( 'NONE', #33302, #18995, #9379, .T. ) ;
#29589=VERTEX_POINT ( 'NONE', #31268 ) ;
#29590=VERTEX_POINT ( 'NONE', #11905 ) ;
#29591=EDGE_CURVE ( 'NONE', #14042, #12472, #12360, .T. ) ;
#29593=CIRCLE ( 'NONE', #3855, 33.00000000000001421 ) ;
#29600=ORIENTED_EDGE ( 'NONE', *, *, #1913, .F. ) ;
#29601=DIRECTION ( 'NONE',  ( 0.000000000000000000, 0.000000000000000000, 1.000000000000000000 ) ) ;
#29602=CARTESIAN_POINT ( 'NONE',  ( -55.00000337463107059, 60.62177826491078747, 12.50000000000000000 ) ) ;
#29603=VECTOR ( 'NONE', #5632, 1000.000000000000000 ) ;
#29604=DIRECTION ( 'NONE',  ( 1.000000000000000000, 0.000000000000000000, 0.000000000000000000 ) ) ;
#29605=VERTEX_POINT ( 'NONE', #5035 ) ;
#29606=CYLINDRICAL_SURFACE ( 'NONE', #16677, 2.000000000000001776 ) ;
#29607=AXIS2_PLACEMENT_3D ( 'NONE', #8811, #14438, #733 ) ;
#29608=DIRECTION ( 'NONE',  ( 0.000000000000000000, 0.000000000000000000, 1.000000000000000000 ) ) ;
#29609=VERTEX_POINT ( 'NONE', #19847 ) ;
#29611=VERTEX_POINT ( 'NONE', #33915 ) ;
#29612=DIRECTION ( 'NONE',  ( -0.000000000000000000, -0.000000000000000000, -1.000000000000000000 ) ) ;
#29613=DIRECTION ( 'NONE',  ( 1.000000000000000000, 0.000000000000000000, 0.000000000000000000 ) ) ;
#29614=DIRECTION ( 'NONE',  ( -1.000000000000000000, 0.000000000000000000, 0.000000000000000000 ) ) ;
#29616=ORIENTED_EDGE ( 'NONE', *, *, #799, .T. ) ;
#29617=CIRCLE ( 'NONE', #5092, 2.000000000000001776 ) ;
#29618=CARTESIAN_POINT ( 'NONE',  ( -25.00000337463121980, -77.94228634059963667, -5.000000000000000000 ) ) ;
#29620=DIRECTION ( 'NONE',  ( 1.000000000000000000, 0.000000000000000000, 0.000000000000000000 ) ) ;
#29621=VECTOR ( 'NONE', #25986, 1000.000000000000000 ) ;
#29622=ORIENTED_EDGE ( 'NONE', *, *, #4082, .F. ) ;
#29623=DIRECTION ( 'NONE',  ( 0.000000000000000000, 0.000000000000000000, 1.000000000000000000 ) ) ;
#29624=VERTEX_POINT ( 'NONE', #2035 ) ;
#29625=DIRECTION ( 'NONE',  ( -1.051347561198064495E-14, -1.000000000000000000, 0.000000000000000000 ) ) ;
#29626=CARTESIAN_POINT ( 'NONE',  ( 72.99999662536836809, -8.660254037844401509, 17.49999999999999645 ) ) ;
#29629=ORIENTED_EDGE ( 'NONE', *, *, #32909, .F. ) ;
#29630=CIRCLE ( 'NONE', #3305, 2.000000000000000000 ) ;
#29631=VERTEX_POINT ( 'NONE', #24927 ) ;
#29632=CIRCLE ( 'NONE', #923, 2.000000000000001776 ) ;
#29635=ORIENTED_EDGE ( 'NONE', *, *, #17001, .F. ) ;
#29636=DIRECTION ( 'NONE',  ( 1.000000000000000000, 0.000000000000000000, 0.000000000000000000 ) ) ;
#29637=EDGE_CURVE ( 'NONE', #24803, #29568, #10677, .T. ) ;
#29638=DIRECTION ( 'NONE',  ( 0.000000000000000000, 0.000000000000000000, 1.000000000000000000 ) ) ;
#29639=CARTESIAN_POINT ( 'NONE',  ( 90.60231327712337190, 15.97563234535636134, 12.49999999999999822 ) ) ;
#29640=DIRECTION ( 'NONE',  ( 1.000000000000000000, 0.000000000000000000, 0.000000000000000000 ) ) ;
#29641=DIRECTION ( 'NONE',  ( 0.000000000000000000, 0.000000000000000000, -1.000000000000000000 ) ) ;
#29642=ORIENTED_EDGE ( 'NONE', *, *, #16263, .F. ) ;
#29643=CARTESIAN_POINT ( 'NONE',  ( 69.99999662536839651, 34.64101615137758472, 17.49999999999999645 ) ) ;
#29644=CIRCLE ( 'NONE', #17109, 2.000000000000001776 ) ;
#29645=AXIS2_PLACEMENT_3D ( 'NONE', #254, #12052, #9457 ) ;
#29646=CARTESIAN_POINT ( 'NONE',  ( 47.63139720814418610, 27.49999999999988987, -10.00000000000000178 ) ) ;
#29649=LINE ( 'NONE', #4354, #22563 ) ;
#29650=LINE ( 'NONE', #3981, #28762 ) ;
#29652=EDGE_LOOP ( 'NONE', ( #28896, #9980 ) ) ;
#29653=VECTOR ( 'NONE', #35751, 1000.000000000000000 ) ;
#29654=DIRECTION ( 'NONE',  ( 0.000000000000000000, 0.000000000000000000, 1.000000000000000000 ) ) ;
#29655=DIRECTION ( 'NONE',  ( 0.000000000000000000, 0.000000000000000000, 1.000000000000000000 ) ) ;
#29657=FACE_OUTER_BOUND ( 'NONE', #28660, .T. ) ;
#29660=VERTEX_POINT ( 'NONE', #25469 ) ;
#29661=EDGE_CURVE ( 'NONE', #35979, #10417, #22554, .T. ) ;
#29663=AXIS2_PLACEMENT_3D ( 'NONE', #29618, #20621, #32259 ) ;
#29665=CARTESIAN_POINT ( 'NONE',  ( -61.53067111003215217, 72.28378166042038799, -4.999999999999997335 ) ) ;
#29667=EDGE_LOOP ( 'NONE', ( #10620, #35875 ) ) ;
#29668=CARTESIAN_POINT ( 'NONE',  ( -55.00000337463110611, -43.30127018922202353, -5.000000000000000000 ) ) ;
#29669=ORIENTED_EDGE ( 'NONE', *, *, #12629, .T. ) ;
#29672=EDGE_CURVE ( 'NONE', #35319, #20996, #17184, .T. ) ;
#29673=CARTESIAN_POINT ( 'NONE',  ( 64.99999662536839651, 60.62177826491078747, 17.49999999999999645 ) ) ;
#29674=CARTESIAN_POINT ( 'NONE',  ( 70.47608876694671665, 59.13646009116074964, -49.22241343995293761 ) ) ;
#29675=EDGE_LOOP ( 'NONE', ( #26449, #17288, #19041, #5605 ) ) ;
#29676=ORIENTED_EDGE ( 'NONE', *, *, #257, .F. ) ;
#29678=CARTESIAN_POINT ( 'NONE',  ( -35.00000337463116296, -60.62177826491080168, 17.49999999999999645 ) ) ;
#29679=CIRCLE ( 'NONE', #975, 2.000000000000001776 ) ;
#29681=CARTESIAN_POINT ( 'NONE',  ( -73.00000337463097821, 43.30127018922197379, 17.49999999999999645 ) ) ;
#29682=AXIS2_PLACEMENT_3D ( 'NONE', #22014, #19217, #7219 ) ;
#29683=VERTEX_POINT ( 'NONE', #9092 ) ;
#29684=DIRECTION ( 'NONE',  ( 0.000000000000000000, 0.000000000000000000, -1.000000000000000000 ) ) ;
#29686=ORIENTED_EDGE ( 'NONE', *, *, #19421, .T. ) ;
#29687=EDGE_CURVE ( 'NONE', #34734, #14264, #30338, .T. ) ;
#29688=DIRECTION ( 'NONE',  ( 0.000000000000000000, 0.000000000000000000, 1.000000000000000000 ) ) ;
#29689=CIRCLE ( 'NONE', #6325, 3.000000000000005773 ) ;
#29691=DIRECTION ( 'NONE',  ( -0.000000000000000000, -0.000000000000000000, 1.000000000000000000 ) ) ;
#29692=DIRECTION ( 'NONE',  ( -1.000000000000000000, 0.000000000000000000, 0.000000000000000000 ) ) ;
#29694=CARTESIAN_POINT ( 'NONE',  ( -55.00000337463109901, -60.62177826491083010, -9.999999999999998224 ) ) ;
#29695=AXIS2_PLACEMENT_3D ( 'NONE', #31942, #6280, #1582 ) ;
#29696=CIRCLE ( 'NONE', #4590, 33.00000000000001421 ) ;
#29698=CARTESIAN_POINT ( 'NONE',  ( -2.778182860043012958, -66.86787810013035482, -4.999999999999997335 ) ) ;
#29699=ORIENTED_EDGE ( 'NONE', *, *, #25134, .T. ) ;
#29700=CARTESIAN_POINT ( 'NONE',  ( -80.00000337463094979, 34.64101615137757051, -5.000000000000000000 ) ) ;
#29701=CARTESIAN_POINT ( 'NONE',  ( -48.00000337463109190, 51.96152422706637708, -9.999999999999998224 ) ) ;
#29702=DIRECTION ( 'NONE',  ( 0.000000000000000000, 0.000000000000000000, 1.000000000000000000 ) ) ;
#29704=CIRCLE ( 'NONE', #25519, 2.000000000000001776 ) ;
#29706=ORIENTED_EDGE ( 'NONE', *, *, #7833, .F. ) ;
#29707=ADVANCED_FACE ( 'NONE', ( #33735 ), #5237, .F. ) ;
#29709=CARTESIAN_POINT ( 'NONE',  ( 64.99999662536841072, -25.98076211353320275, 17.49999999999999645 ) ) ;
#29710=CARTESIAN_POINT ( 'NONE',  ( 70.47608876694671665, 59.13646009116074964, 12.49999999999999822 ) ) ;
#29711=CIRCLE ( 'NONE', #2181, 2.000000000000001776 ) ;
#29712=CARTESIAN_POINT ( 'NONE',  ( 74.99999662536835388, -43.30127018922199511, -9.999999999999998224 ) ) ;
#29717=ADVANCED_FACE ( 'NONE', ( #36904 ), #33564, .F. ) ;
#29718=EDGE_LOOP ( 'NONE', ( #30021, #5653 ) ) ;
#29719=FACE_BOUND ( 'NONE', #1397, .T. ) ;
#29721=CIRCLE ( 'NONE', #384, 2.000000000000001776 ) ;
#29723=AXIS2_PLACEMENT_3D ( 'NONE', #33609, #8463, #7911 ) ;
#29724=EDGE_CURVE ( 'NONE', #22792, #17282, #29160, .T. ) ;
#29726=DIRECTION ( 'NONE',  ( 0.000000000000000000, 0.000000000000000000, -1.000000000000000000 ) ) ;
#29729=DIRECTION ( 'NONE',  ( -0.000000000000000000, -0.000000000000000000, 1.000000000000000000 ) ) ;
#29731=LINE ( 'NONE', #9691, #18906 ) ;
#29732=CYLINDRICAL_SURFACE ( 'NONE', #36540, 2.000000000000001776 ) ;
#29735=CARTESIAN_POINT ( 'NONE',  ( 44.99999662536851019, -60.62177826491080168, 12.50000000000000000 ) ) ;
#29737=LINE ( 'NONE', #24129, #36945 ) ;
#29738=CIRCLE ( 'NONE', #16591, 2.000000000000001776 ) ;
#29739=ORIENTED_EDGE ( 'NONE', *, *, #17239, .T. ) ;
#29740=ADVANCED_FACE ( 'NONE', ( #8032 ), #16302, .F. ) ;
#29741=ORIENTED_EDGE ( 'NONE', *, *, #23623, .T. ) ;
#29742=AXIS2_PLACEMENT_3D ( 'NONE', #3283, #27906, #8419 ) ;
#29743=ORIENTED_EDGE ( 'NONE', *, *, #16320, .F. ) ;
#29744=CARTESIAN_POINT ( 'NONE',  ( -47.00000337463111322, 60.62177826491077326, 12.50000000000000000 ) ) ;
#29746=CIRCLE ( 'NONE', #23181, 2.000000000000001776 ) ;
#29747=EDGE_CURVE ( 'NONE', #29309, #20458, #21265, .T. ) ;
#29748=VECTOR ( 'NONE', #4315, 1000.000000000000000 ) ;
#29749=CARTESIAN_POINT ( 'NONE',  ( 52.39915983220795681, 35.19434990244919703, -4.999999999999997335 ) ) ;
#29750=CIRCLE ( 'NONE', #16601, 2.000000000000001776 ) ;
#29751=CIRCLE ( 'NONE', #34566, 2.000000000000001776 ) ;
#29752=EDGE_CURVE ( 'NONE', #8095, #32403, #36966, .T. ) ;
#29753=CARTESIAN_POINT ( 'NONE',  ( 56.67878100130369035, -27.78182860042797131, -49.86348611802629449 ) ) ;
#29755=CIRCLE ( 'NONE', #13602, 2.000000000000001776 ) ;
#29759=CYLINDRICAL_SURFACE ( 'NONE', #25481, 2.000000000000001776 ) ;
#29760=CARTESIAN_POINT ( 'NONE',  ( -5.000003374631269537, -77.94228634059960825, 12.50000000000000000 ) ) ;
#29761=ORIENTED_EDGE ( 'NONE', *, *, #37060, .F. ) ;
#29762=CARTESIAN_POINT ( 'NONE',  ( -43.00000337463111322, 77.94228634059959404, 12.50000000000000000 ) ) ;
#29763=ORIENTED_EDGE ( 'NONE', *, *, #17756, .T. ) ;
#29765=CYLINDRICAL_SURFACE ( 'NONE', #5125, 2.000000000000001776 ) ;
#29766=CIRCLE ( 'NONE', #17778, 2.000000000000001776 ) ;
#29767=ADVANCED_FACE ( 'NONE', ( #662 ), #9661, .F. ) ;
#29768=AXIS2_PLACEMENT_3D ( 'NONE', #16221, #4950, #16388 ) ;
#29769=CARTESIAN_POINT ( 'NONE',  ( 0.000000000000000000, 0.000000000000000000, -5.000000000000000000 ) ) ;
#29770=ORIENTED_EDGE ( 'NONE', *, *, #27714, .F. ) ;
#29771=VERTEX_POINT ( 'NONE', #21086 ) ;
#29772=DIRECTION ( 'NONE',  ( 1.000000000000000000, 0.000000000000000000, 0.000000000000000000 ) ) ;
#29773=ORIENTED_EDGE ( 'NONE', *, *, #36728, .T. ) ;
#29776=CIRCLE ( 'NONE', #2253, 2.000000000000001776 ) ;
#29778=VECTOR ( 'NONE', #9072, 1000.000000000000000 ) ;
#29779=CARTESIAN_POINT ( 'NONE',  ( 29.99999662536857770, -69.28203230275519786, -9.999999999999998224 ) ) ;
#29780=CARTESIAN_POINT ( 'NONE',  ( -34.00000000000027711, -58.88972745734168512, -4.999999999999997335 ) ) ;
#29781=ORIENTED_EDGE ( 'NONE', *, *, #4034, .F. ) ;
#29784=EDGE_LOOP ( 'NONE', ( #25074, #10541 ) ) ;
#29785=VERTEX_POINT ( 'NONE', #35537 ) ;
#29786=EDGE_CURVE ( 'NONE', #35919, #29281, #11803, .T. ) ;
#29788=CARTESIAN_POINT ( 'NONE',  ( 89.99999662536828282, 0.000000000000000000, -9.999999999999998224 ) ) ;
#29790=CARTESIAN_POINT ( 'NONE',  ( -12.00000337463125000, -86.60254037844400443, -5.000000000000000000 ) ) ;
#29791=EDGE_CURVE ( 'NONE', #24619, #28688, #13617, .T. ) ;
#29792=EDGE_LOOP ( 'NONE', ( #6910, #1989, #28067, #20553, #26793 ) ) ;
#29793=CIRCLE ( 'NONE', #13640, 2.000000000000001776 ) ;
#29795=AXIS2_PLACEMENT_3D ( 'NONE', #6055, #14857, #9213 ) ;
#29796=DIRECTION ( 'NONE',  ( -1.000000000000000000, 0.000000000000000000, 0.000000000000000000 ) ) ;
#29797=DIRECTION ( 'NONE',  ( -1.000000000000000000, 0.000000000000000000, 0.000000000000000000 ) ) ;
#29798=VERTEX_POINT ( 'NONE', #7030 ) ;
#29799=CYLINDRICAL_SURFACE ( 'NONE', #30223, 2.000000000000001776 ) ;
#29800=VECTOR ( 'NONE', #12900, 1000.000000000000000 ) ;
#29801=EDGE_CURVE ( 'NONE', #25394, #31695, #15409, .T. ) ;
#29802=CYLINDRICAL_SURFACE ( 'NONE', #28184, 27.00000000000001066 ) ;
#29803=CIRCLE ( 'NONE', #14846, 2.000000000000001776 ) ;
#29806=CARTESIAN_POINT ( 'NONE',  ( 87.83969979969882047, 14.80603122773025504, -49.86561046011506448 ) ) ;
#29807=ADVANCED_FACE ( 'NONE', ( #12815 ), #34975, .F. ) ;
#29809=EDGE_CURVE ( 'NONE', #30112, #25842, #8216, .T. ) ;
#29811=ORIENTED_EDGE ( 'NONE', *, *, #20060, .T. ) ;
#29813=DIRECTION ( 'NONE',  ( 1.000000000000000000, 0.000000000000000000, 0.000000000000000000 ) ) ;
#29814=DIRECTION ( 'NONE',  ( -0.000000000000000000, -0.000000000000000000, 1.000000000000000000 ) ) ;
#29815=CARTESIAN_POINT ( 'NONE',  ( -69.61831313460106685, -36.60425647305652319, -5.000000000000000000 ) ) ;
#29817=VERTEX_POINT ( 'NONE', #4030 ) ;
#29819=ADVANCED_FACE ( 'NONE', ( #9272 ), #3665, .T. ) ;
#29820=CARTESIAN_POINT ( 'NONE',  ( 54.99999662536844625, 43.30127018922198801, -9.999999999999998224 ) ) ;
#29821=EDGE_CURVE ( 'NONE', #24381, #7306, #29901, .T. ) ;
#29824=VERTEX_POINT ( 'NONE', #6278 ) ;
#29827=VECTOR ( 'NONE', #24666, 1000.000000000000000 ) ;
#29828=AXIS2_PLACEMENT_3D ( 'NONE', #31487, #5825, #6017 ) ;
#29829=CARTESIAN_POINT ( 'NONE',  ( 19.99999662536858835, 69.28203230275516944, -9.999999999999998224 ) ) ;
#29831=AXIS2_PLACEMENT_3D ( 'NONE', #22841, #33722, #2417 ) ;
#29832=DIRECTION ( 'NONE',  ( -1.000000000000000000, 0.000000000000000000, 0.000000000000000000 ) ) ;
#29833=CARTESIAN_POINT ( 'NONE',  ( -48.00000337463109190, 69.28203230275518365, -9.999999999999998224 ) ) ;
#29835=DIRECTION ( 'NONE',  ( -1.000000000000000000, 0.000000000000000000, 0.000000000000000000 ) ) ;
#29836=VERTEX_POINT ( 'NONE', #26712 ) ;
#29837=ORIENTED_EDGE ( 'NONE', *, *, #11274, .F. ) ;
#29838=VECTOR ( 'NONE', #15815, 1000.000000000000000 ) ;
#29839=ORIENTED_EDGE ( 'NONE', *, *, #12379, .T. ) ;
#29841=CARTESIAN_POINT ( 'NONE',  ( 84.99999662536831124, -8.660254037844397956, 12.50000000000000000 ) ) ;
#29842=FACE_OUTER_BOUND ( 'NONE', #19845, .T. ) ;
#29843=DIRECTION ( 'NONE',  ( 0.000000000000000000, 0.000000000000000000, -1.000000000000000000 ) ) ;
#29844=AXIS2_PLACEMENT_3D ( 'NONE', #23472, #28893, #25914 ) ;
#29845=DIRECTION ( 'NONE',  ( -0.000000000000000000, -0.000000000000000000, 1.000000000000000000 ) ) ;
#29846=ORIENTED_EDGE ( 'NONE', *, *, #32885, .F. ) ;
#29847=DIRECTION ( 'NONE',  ( 0.000000000000000000, 0.000000000000000000, 1.000000000000000000 ) ) ;
#29853=DIRECTION ( 'NONE',  ( 0.000000000000000000, 0.000000000000000000, -1.000000000000000000 ) ) ;
#29854=CIRCLE ( 'NONE', #35288, 2.000000000000001776 ) ;
#29855=FACE_OUTER_BOUND ( 'NONE', #36533, .T. ) ;
#29856=CARTESIAN_POINT ( 'NONE',  ( -8.000003374631287301, 69.28203230275516944, -9.999999999999998224 ) ) ;
#29857=ORIENTED_EDGE ( 'NONE', *, *, #2060, .F. ) ;
#29858=EDGE_LOOP ( 'NONE', ( #18564, #31137, #5836, #20522, #8601, #18363, #8389, #9551, #5207, #35315, #1017, #20172, #13988, #13434, #8022, #26359 ) ) ;
#29859=CIRCLE ( 'NONE', #4120, 2.000000000000001776 ) ;
#29860=AXIS2_PLACEMENT_3D ( 'NONE', #8886, #17335, #28760 ) ;
#29861=CARTESIAN_POINT ( 'NONE',  ( 0.000000000000000000, 0.000000000000000000, -10.00000000000000000 ) ) ;
#29864=ORIENTED_EDGE ( 'NONE', *, *, #7872, .F. ) ;
#29865=EDGE_LOOP ( 'NONE', ( #15663, #11128, #14262, #1115 ) ) ;
#29866=ORIENTED_EDGE ( 'NONE', *, *, #3802, .T. ) ;
#29867=CIRCLE ( 'NONE', #2957, 33.00000000000001421 ) ;
#29868=EDGE_CURVE ( 'NONE', #21598, #7182, #23724, .T. ) ;
#29869=CARTESIAN_POINT ( 'NONE',  ( 9.999996625368625658, 86.60254037844397601, -9.999999999999998224 ) ) ;
#29870=ORIENTED_EDGE ( 'NONE', *, *, #4867, .F. ) ;
#29871=EDGE_CURVE ( 'NONE', #8170, #17344, #4039, .T. ) ;
#29872=ORIENTED_EDGE ( 'NONE', *, *, #15793, .T. ) ;
#29873=DIRECTION ( 'NONE',  ( 0.000000000000000000, 0.000000000000000000, -1.000000000000000000 ) ) ;
#29874=VERTEX_POINT ( 'NONE', #20917 ) ;
#29875=VERTEX_POINT ( 'NONE', #1030 ) ;
#29876=CARTESIAN_POINT ( 'NONE',  ( -67.00000337463104927, -25.98076211353322051, 17.49999999999999645 ) ) ;
#29877=AXIS2_PLACEMENT_3D ( 'NONE', #36353, #8021, #1850 ) ;
#29879=ORIENTED_EDGE ( 'NONE', *, *, #10057, .F. ) ;
#29880=ORIENTED_EDGE ( 'NONE', *, *, #13549, .T. ) ;
#29881=CARTESIAN_POINT ( 'NONE',  ( 19.99999662536861678, -69.28203230275519786, -9.999999999999998224 ) ) ;
#29882=AXIS2_PLACEMENT_3D ( 'NONE', #2666, #36251, #28345 ) ;
#29883=DIRECTION ( 'NONE',  ( -1.000000000000000000, 0.000000000000000000, 0.000000000000000000 ) ) ;
#29886=ORIENTED_EDGE ( 'NONE', *, *, #13552, .T. ) ;
#29887=DIRECTION ( 'NONE',  ( 1.000000000000000000, 0.000000000000000000, 0.000000000000000000 ) ) ;
#29888=AXIS2_PLACEMENT_3D ( 'NONE', #18492, #16046, #29915 ) ;
#29891=DIRECTION ( 'NONE',  ( 1.000000000000000000, 0.000000000000000000, 0.000000000000000000 ) ) ;
#29892=CARTESIAN_POINT ( 'NONE',  ( 59.13646009116148150, -70.47608876694609137, 12.49999999999999822 ) ) ;
#29893=CARTESIAN_POINT ( 'NONE',  ( -52.39915983220772233, -35.19434990244957362, 12.49999999999999822 ) ) ;
#29894=VECTOR ( 'NONE', #25441, 1000.000000000000000 ) ;
#29896=FACE_OUTER_BOUND ( 'NONE', #37061, .T. ) ;
#29897=CARTESIAN_POINT ( 'NONE',  ( 63.10544158860312081, 59.98094972882071829, 12.50000000000000000 ) ) ;
#29898=CARTESIAN_POINT ( 'NONE',  ( 64.99999662536841072, 25.98076211353318854, 12.50000000000000000 ) ) ;
#29899=CIRCLE ( 'NONE', #22708, 3.000000000000002665 ) ;
#29900=VERTEX_POINT ( 'NONE', #10386 ) ;
#29901=LINE ( 'NONE', #20516, #3418 ) ;
#29903=FACE_OUTER_BOUND ( 'NONE', #31210, .T. ) ;
#29904=VERTEX_POINT ( 'NONE', #32906 ) ;
#29905=EDGE_CURVE ( 'NONE', #25059, #16555, #1947, .T. ) ;
#29907=AXIS2_PLACEMENT_3D ( 'NONE', #33757, #22871, #22693 ) ;
#29908=ORIENTED_EDGE ( 'NONE', *, *, #34515, .T. ) ;
#29911=CARTESIAN_POINT ( 'NONE',  ( -13.89091430021420237, -62.33939050065180254, 12.49999999999999822 ) ) ;
#29913=VECTOR ( 'NONE', #36545, 1000.000000000000000 ) ;
#29914=EDGE_LOOP ( 'NONE', ( #4317, #22573, #36403, #32801 ) ) ;
#29915=DIRECTION ( 'NONE',  ( 1.000000000000000000, 0.000000000000000000, 0.000000000000000000 ) ) ;
#29917=ORIENTED_EDGE ( 'NONE', *, *, #33103, .T. ) ;
#29918=EDGE_CURVE ( 'NONE', #6451, #16018, #1038, .T. ) ;
#29919=LINE ( 'NONE', #19236, #13168 ) ;
#29920=ORIENTED_EDGE ( 'NONE', *, *, #5711, .T. ) ;
#29921=FACE_BOUND ( 'NONE', #18938, .T. ) ;
#29922=AXIS2_PLACEMENT_3D ( 'NONE', #9844, #18673, #15674 ) ;
#29923=CIRCLE ( 'NONE', #34117, 3.000000000000002665 ) ;
#29924=DIRECTION ( 'NONE',  ( 0.000000000000000000, 0.000000000000000000, 1.000000000000000000 ) ) ;
#29925=CARTESIAN_POINT ( 'NONE',  ( -7.000003374631269537, -77.94228634059960825, -5.000000000000000000 ) ) ;
#29926=CARTESIAN_POINT ( 'NONE',  ( -47.63139720814380951, 27.50000000000055422, -10.00000000000000178 ) ) ;
#29927=AXIS2_PLACEMENT_3D ( 'NONE', #11114, #29462, #8867 ) ;
#29928=ORIENTED_EDGE ( 'NONE', *, *, #19887, .T. ) ;
#29929=DIRECTION ( 'NONE',  ( -1.000000000000000000, -2.492861883996299315E-14, 0.000000000000000000 ) ) ;
#29932=CIRCLE ( 'NONE', #5407, 2.000000000000001776 ) ;
#29934=FACE_OUTER_BOUND ( 'NONE', #11894, .T. ) ;
#29935=EDGE_CURVE ( 'NONE', #20586, #18237, #8821, .T. ) ;
#29936=VERTEX_POINT ( 'NONE', #13376 ) ;
#29937=DIRECTION ( 'NONE',  ( 1.000000000000000000, 0.000000000000000000, 0.000000000000000000 ) ) ;
#29939=CARTESIAN_POINT ( 'NONE',  ( -12.00000337463125000, -86.60254037844400443, -9.999999999999998224 ) ) ;
#29940=CARTESIAN_POINT ( 'NONE',  ( -3.000003374631308173, 77.94228634059957983, -9.999999999999998224 ) ) ;
#29941=EDGE_CURVE ( 'NONE', #24063, #31658, #1779, .T. ) ;
#29942=ORIENTED_EDGE ( 'NONE', *, *, #26855, .F. ) ;
#29943=ORIENTED_EDGE ( 'NONE', *, *, #14019, .F. ) ;
#29944=EDGE_CURVE ( 'NONE', #32725, #18729, #16007, .T. ) ;
#29946=DIRECTION ( 'NONE',  ( 0.000000000000000000, 0.000000000000000000, 1.000000000000000000 ) ) ;
#29947=CIRCLE ( 'NONE', #16796, 2.000000000000001776 ) ;
#29949=ADVANCED_FACE ( 'NONE', ( #2130 ), #16579, .T. ) ;
#29951=CIRCLE ( 'NONE', #12593, 3.000000000000002665 ) ;
#29952=FACE_OUTER_BOUND ( 'NONE', #33686, .T. ) ;
#29955=DIRECTION ( 'NONE',  ( 0.000000000000000000, 0.000000000000000000, -1.000000000000000000 ) ) ;
#29956=ORIENTED_EDGE ( 'NONE', *, *, #30741, .F. ) ;
#29957=ORIENTED_EDGE ( 'NONE', *, *, #16666, .F. ) ;
#29958=LINE ( 'NONE', #10267, #1544 ) ;
#29959=DIRECTION ( 'NONE',  ( 0.000000000000000000, 0.000000000000000000, -1.000000000000000000 ) ) ;
#29960=ORIENTED_EDGE ( 'NONE', *, *, #15211, .T. ) ;
#29961=EDGE_CURVE ( 'NONE', #26137, #2878, #17779, .T. ) ;
#29962=FACE_OUTER_BOUND ( 'NONE', #11872, .T. ) ;
#29965=EDGE_CURVE ( 'NONE', #20237, #23192, #10627, .T. ) ;
#29966=FACE_BOUND ( 'NONE', #28055, .T. ) ;
#29967=EDGE_LOOP ( 'NONE', ( #6087, #426 ) ) ;
#29968=VERTEX_POINT ( 'NONE', #10775 ) ;
#29969=DIRECTION ( 'NONE',  ( 0.000000000000000000, 0.000000000000000000, -1.000000000000000000 ) ) ;
#29970=ORIENTED_EDGE ( 'NONE', *, *, #31171, .T. ) ;
#29972=EDGE_CURVE ( 'NONE', #32493, #21629, #22209, .T. ) ;
#29974=CARTESIAN_POINT ( 'NONE',  ( 33.99999999999986500, -58.88972745734191250, -4.999999999999997335 ) ) ;
#29978=ORIENTED_EDGE ( 'NONE', *, *, #17980, .T. ) ;
#29979=DIRECTION ( 'NONE',  ( 0.000000000000000000, 0.000000000000000000, 1.000000000000000000 ) ) ;
#29980=CARTESIAN_POINT ( 'NONE',  ( 79.99999662536832545, -17.32050807568879591, 12.50000000000000000 ) ) ;
#29981=VERTEX_POINT ( 'NONE', #30078 ) ;
#29982=ORIENTED_EDGE ( 'NONE', *, *, #23922, .F. ) ;
#29983=ORIENTED_EDGE ( 'NONE', *, *, #1129, .F. ) ;
#29984=CARTESIAN_POINT ( 'NONE',  ( -10.00000337463125000, -86.60254037844400443, -5.000000000000000000 ) ) ;
#29985=CYLINDRICAL_SURFACE ( 'NONE', #13802, 2.000000000000001776 ) ;
#29987=EDGE_CURVE ( 'NONE', #28791, #19268, #16623, .T. ) ;
#29988=LINE ( 'NONE', #36002, #1369 ) ;
#29989=DIRECTION ( 'NONE',  ( 0.000000000000000000, 0.000000000000000000, 1.000000000000000000 ) ) ;
#29990=ORIENTED_EDGE ( 'NONE', *, *, #15312, .F. ) ;
#29991=DIRECTION ( 'NONE',  ( 0.000000000000000000, 0.000000000000000000, 1.000000000000000000 ) ) ;
#29992=DIRECTION ( 'NONE',  ( 1.000000000000000000, 0.000000000000000000, 0.000000000000000000 ) ) ;
#29993=ADVANCED_FACE ( 'NONE', ( #13770 ), #27257, .F. ) ;
#29994=CARTESIAN_POINT ( 'NONE',  ( -60.00000337463104216, 51.96152422706639129, 17.49999999999999645 ) ) ;
#29995=DIRECTION ( 'NONE',  ( 0.000000000000000000, 0.000000000000000000, 1.000000000000000000 ) ) ;
#29996=CARTESIAN_POINT ( 'NONE',  ( -65.00000337463106348, -60.62177826491083010, -5.000000000000000000 ) ) ;
#29997=DIRECTION ( 'NONE',  ( 1.000000000000000000, 0.000000000000000000, 0.000000000000000000 ) ) ;
#29999=ORIENTED_EDGE ( 'NONE', *, *, #25158, .T. ) ;
#30000=CARTESIAN_POINT ( 'NONE',  ( -52.39915983220772233, -35.19434990244957362, 12.49999999999999822 ) ) ;
#30001=DIRECTION ( 'NONE',  ( 0.000000000000000000, 0.000000000000000000, 1.000000000000000000 ) ) ;
#30002=AXIS2_PLACEMENT_3D ( 'NONE', #23018, #34467, #11758 ) ;
#30003=DIRECTION ( 'NONE',  ( 0.000000000000000000, 0.000000000000000000, 1.000000000000000000 ) ) ;
#30005=ORIENTED_EDGE ( 'NONE', *, *, #10772, .F. ) ;
#30006=DIRECTION ( 'NONE',  ( 0.000000000000000000, 0.000000000000000000, 1.000000000000000000 ) ) ;
#30007=CARTESIAN_POINT ( 'NONE',  ( 0.000000000000000000, 0.000000000000000000, -10.00000000000000000 ) ) ;
#30008=EDGE_CURVE ( 'NONE', #23662, #6894, #5251, .T. ) ;
#30010=DIRECTION ( 'NONE',  ( 0.000000000000000000, 0.000000000000000000, 1.000000000000000000 ) ) ;
#30011=ORIENTED_EDGE ( 'NONE', *, *, #32164, .T. ) ;
#30012=DIRECTION ( 'NONE',  ( 0.000000000000000000, 0.000000000000000000, 1.000000000000000000 ) ) ;
#30013=EDGE_CURVE ( 'NONE', #6156, #17794, #9998, .T. ) ;
#30014=CARTESIAN_POINT ( 'NONE',  ( -46.74666114985175369, -61.59604035298635694, -5.000000000000000000 ) ) ;
#30015=DIRECTION ( 'NONE',  ( -1.000000000000000000, 0.000000000000000000, 0.000000000000000000 ) ) ;
#30016=EDGE_CURVE ( 'NONE', #6890, #603, #24476, .T. ) ;
#30020=AXIS2_PLACEMENT_3D ( 'NONE', #15754, #16316, #36017 ) ;
#30021=ORIENTED_EDGE ( 'NONE', *, *, #27072, .T. ) ;
#30023=CARTESIAN_POINT ( 'NONE',  ( 79.99999662536833966, 17.32050807568879236, 17.49999999999999645 ) ) ;
#30024=CARTESIAN_POINT ( 'NONE',  ( 81.99999662536833966, -3.469446951953614189E-15, 17.49999999999999645 ) ) ;
#30025=DIRECTION ( 'NONE',  ( 0.000000000000000000, 0.000000000000000000, 1.000000000000000000 ) ) ;
#30026=DIRECTION ( 'NONE',  ( 0.000000000000000000, 0.000000000000000000, 1.000000000000000000 ) ) ;
#30027=ORIENTED_EDGE ( 'NONE', *, *, #915, .T. ) ;
#30028=CARTESIAN_POINT ( 'NONE',  ( 9.999996625368618552, 69.28203230275516944, 12.50000000000000000 ) ) ;
#30029=DIRECTION ( 'NONE',  ( 0.000000000000000000, 0.000000000000000000, -1.000000000000000000 ) ) ;
#30031=DIRECTION ( 'NONE',  ( 1.000000000000000000, 0.000000000000000000, 0.000000000000000000 ) ) ;
#30032=EDGE_LOOP ( 'NONE', ( #32001, #26958 ) ) ;
#30033=CARTESIAN_POINT ( 'NONE',  ( 69.99999662536839651, -17.32050807568879947, -9.999999999999998224 ) ) ;
#30034=FACE_BOUND ( 'NONE', #9728, .T. ) ;
#30036=EDGE_LOOP ( 'NONE', ( #29957, #481, #36503, #22778 ) ) ;
#30038=CARTESIAN_POINT ( 'NONE',  ( 47.04203867989577503, -43.19957991610382919, 12.49999999999999822 ) ) ;
#30039=CARTESIAN_POINT ( 'NONE',  ( -72.00000337463100664, -17.32050807568882078, -5.000000000000000000 ) ) ;
#30042=AXIS2_PLACEMENT_3D ( 'NONE', #25347, #20078, #28514 ) ;
#30043=ORIENTED_EDGE ( 'NONE', *, *, #16320, .T. ) ;
#30044=ORIENTED_EDGE ( 'NONE', *, *, #9126, .T. ) ;
#30045=CARTESIAN_POINT ( 'NONE',  ( 0.000000000000000000, 0.000000000000000000, 12.49999999999999822 ) ) ;
#30046=EDGE_CURVE ( 'NONE', #598, #32017, #25589, .T. ) ;
#30048=EDGE_CURVE ( 'NONE', #1072, #22136, #8679, .T. ) ;
#30049=ORIENTED_EDGE ( 'NONE', *, *, #14435, .T. ) ;
#30050=FACE_BOUND ( 'NONE', #34397, .T. ) ;
#30051=ORIENTED_EDGE ( 'NONE', *, *, #26492, .F. ) ;
#30052=ORIENTED_EDGE ( 'NONE', *, *, #10293, .T. ) ;
#30053=PLANE ( 'NONE',  #2254 ) ;
#30055=VERTEX_POINT ( 'NONE', #14321 ) ;
#30056=EDGE_LOOP ( 'NONE', ( #11662, #26459, #27811, #15792 ) ) ;
#30057=EDGE_CURVE ( 'NONE', #32725, #29300, #28910, .T. ) ;
#30058=CARTESIAN_POINT ( 'NONE',  ( -61.06482292022059255, 72.77422209630346117, -5.000000000000000000 ) ) ;
#30059=DIRECTION ( 'NONE',  ( 0.000000000000000000, 0.000000000000000000, 1.000000000000000000 ) ) ;
#30061=DIRECTION ( 'NONE',  ( 1.000000000000000000, 0.000000000000000000, 0.000000000000000000 ) ) ;
#30064=AXIS2_PLACEMENT_3D ( 'NONE', #7720, #27952, #19171 ) ;
#30065=ORIENTED_EDGE ( 'NONE', *, *, #36910, .T. ) ;
#30068=CARTESIAN_POINT ( 'NONE',  ( 51.99999662536847467, 51.96152422706637708, 12.50000000000000000 ) ) ;
#30069=CARTESIAN_POINT ( 'NONE',  ( 84.99999662536831124, -25.98076211353319565, -5.000000000000000000 ) ) ;
#30070=EDGE_CURVE ( 'NONE', #3159, #3670, #20231, .T. ) ;
#30071=CARTESIAN_POINT ( 'NONE',  ( -4.279621169095561228, 62.97617850287782915, 12.49999999999999822 ) ) ;
#30072=EDGE_CURVE ( 'NONE', #34695, #12950, #2890, .T. ) ;
#30074=EDGE_CURVE ( 'NONE', #18017, #24720, #3452, .T. ) ;
#30075=EDGE_CURVE ( 'NONE', #36125, #6234, #19935, .T. ) ;
#30076=CARTESIAN_POINT ( 'NONE',  ( -77.00000337463097821, -8.660254037844422825, 12.50000000000000000 ) ) ;
#30078=CARTESIAN_POINT ( 'NONE',  ( -87.00000337463093558, -25.98076211353322051, 12.50000000000000000 ) ) ;
#30079=CARTESIAN_POINT ( 'NONE',  ( 61.99999662536842493, -51.96152422706639840, -5.000000000000000000 ) ) ;
#30080=DIRECTION ( 'NONE',  ( 1.000000000000000000, 0.000000000000000000, 0.000000000000000000 ) ) ;
#30082=CIRCLE ( 'NONE', #12695, 2.000000000000001776 ) ;
#30083=CIRCLE ( 'NONE', #8547, 3.000000000000002665 ) ;
#30084=EDGE_LOOP ( 'NONE', ( #21971, #23131 ) ) ;
#30085=VERTEX_POINT ( 'NONE', #8872 ) ;
#30086=DIRECTION ( 'NONE',  ( 0.000000000000000000, 0.000000000000000000, 1.000000000000000000 ) ) ;
#30087=DIRECTION ( 'NONE',  ( -1.000000000000000000, 0.000000000000000000, 0.000000000000000000 ) ) ;
#30088=DIRECTION ( 'NONE',  ( 1.000000000000000000, 0.000000000000000000, 0.000000000000000000 ) ) ;
#30089=ORIENTED_EDGE ( 'NONE', *, *, #8302, .T. ) ;
#30090=CARTESIAN_POINT ( 'NONE',  ( 41.99999662536853151, 69.28203230275518365, -9.999999999999998224 ) ) ;
#30091=CIRCLE ( 'NONE', #13355, 2.000000000000001776 ) ;
#30092=DIRECTION ( 'NONE',  ( 0.000000000000000000, 0.000000000000000000, 1.000000000000000000 ) ) ;
#30093=EDGE_LOOP ( 'NONE', ( #15340, #4029, #25, #6035 ) ) ;
#30095=ORIENTED_EDGE ( 'NONE', *, *, #31864, .F. ) ;
#30096=DIRECTION ( 'NONE',  ( 0.000000000000000000, 0.000000000000000000, 1.000000000000000000 ) ) ;
#30099=DIRECTION ( 'NONE',  ( -1.000000000000000000, 0.000000000000000000, 0.000000000000000000 ) ) ;
#30101=ORIENTED_EDGE ( 'NONE', *, *, #7868, .F. ) ;
#30103=CARTESIAN_POINT ( 'NONE',  ( 9.999996625368625658, 86.60254037844397601, -5.000000000000000000 ) ) ;
#30104=DIRECTION ( 'NONE',  ( 0.000000000000000000, 0.000000000000000000, 1.000000000000000000 ) ) ;
#30105=CIRCLE ( 'NONE', #36116, 33.00000000000001421 ) ;
#30106=CARTESIAN_POINT ( 'NONE',  ( -85.00000337463092137, 8.660254037844389075, 12.50000000000000000 ) ) ;
#30107=CYLINDRICAL_SURFACE ( 'NONE', #34128, 2.000000000000001776 ) ;
#30108=VERTEX_POINT ( 'NONE', #8505 ) ;
#30109=DIRECTION ( 'NONE',  ( 1.000000000000000000, 0.000000000000000000, 0.000000000000000000 ) ) ;
#30110=CARTESIAN_POINT ( 'NONE',  ( -53.00000337463109190, -60.62177826491083010, -9.999999999999998224 ) ) ;
#30111=DIRECTION ( 'NONE',  ( 1.000000000000000000, 0.000000000000000000, 0.000000000000000000 ) ) ;
#30112=VERTEX_POINT ( 'NONE', #20310 ) ;
#30113=AXIS2_PLACEMENT_3D ( 'NONE', #36721, #20514, #26352 ) ;
#30114=EDGE_CURVE ( 'NONE', #11413, #2754, #29803, .T. ) ;
#30115=ORIENTED_EDGE ( 'NONE', *, *, #32475, .F. ) ;
#30116=CYLINDRICAL_SURFACE ( 'NONE', #19573, 33.00000000000001421 ) ;
#30117=DIRECTION ( 'NONE',  ( 0.000000000000000000, 0.000000000000000000, 1.000000000000000000 ) ) ;
#30118=CARTESIAN_POINT ( 'NONE',  ( 54.99999662536844625, 43.30127018922198801, -9.999999999999998224 ) ) ;
#30120=CARTESIAN_POINT ( 'NONE',  ( -52.39915983220772233, -35.19434990244957362, -4.999999999999997335 ) ) ;
#30121=CARTESIAN_POINT ( 'NONE',  ( -83.00000337463092137, -8.660254037844422825, -9.999999999999998224 ) ) ;
#30122=CARTESIAN_POINT ( 'NONE',  ( -15.00000337463125710, -77.94228634059960825, 17.49999999999999645 ) ) ;
#30123=AXIS2_PLACEMENT_3D ( 'NONE', #28757, #25779, #3081 ) ;
#30124=CARTESIAN_POINT ( 'NONE',  ( 62.97617850287784336, 4.279621169095339184, -4.999999999999997335 ) ) ;
#30126=VERTEX_POINT ( 'NONE', #16941 ) ;
#30127=CIRCLE ( 'NONE', #21164, 3.499999999999989342 ) ;
#30128=DIRECTION ( 'NONE',  ( 0.000000000000000000, 0.000000000000000000, -1.000000000000000000 ) ) ;
#30130=VERTEX_POINT ( 'NONE', #13935 ) ;
#30133=CARTESIAN_POINT ( 'NONE',  ( 14.99999662536863632, -77.94228634059960825, -9.999999999999998224 ) ) ;
#30134=ADVANCED_FACE ( 'NONE', ( #22936 ), #25384, .F. ) ;
#30135=AXIS2_PLACEMENT_3D ( 'NONE', #14702, #19609, #31221 ) ;
#30137=ORIENTED_EDGE ( 'NONE', *, *, #2824, .F. ) ;
#30139=VERTEX_POINT ( 'NONE', #14495 ) ;
#30140=DIRECTION ( 'NONE',  ( 0.000000000000000000, 0.000000000000000000, 1.000000000000000000 ) ) ;
#30141=VERTEX_POINT ( 'NONE', #28364 ) ;
#30143=AXIS2_PLACEMENT_3D ( 'NONE', #8551, #3489, #31406 ) ;
#30145=DIRECTION ( 'NONE',  ( 0.000000000000000000, 0.000000000000000000, 1.000000000000000000 ) ) ;
#30147=DIRECTION ( 'NONE',  ( 0.000000000000000000, 0.000000000000000000, 1.000000000000000000 ) ) ;
#30148=DIRECTION ( 'NONE',  ( 1.000000000000000000, 0.000000000000000000, 0.000000000000000000 ) ) ;
#30150=CARTESIAN_POINT ( 'NONE',  ( 69.99999662536839651, 34.64101615137758472, -5.000000000000000000 ) ) ;
#30151=DIRECTION ( 'NONE',  ( 1.000000000000000000, 0.000000000000000000, 0.000000000000000000 ) ) ;
#30154=AXIS2_PLACEMENT_3D ( 'NONE', #35968, #33122, #7442 ) ;
#30155=ORIENTED_EDGE ( 'NONE', *, *, #1277, .T. ) ;
#30156=DIRECTION ( 'NONE',  ( 0.000000000000000000, 0.000000000000000000, 1.000000000000000000 ) ) ;
#30157=EDGE_CURVE ( 'NONE', #15837, #2273, #7066, .T. ) ;
#30158=FACE_OUTER_BOUND ( 'NONE', #32187, .T. ) ;
#30159=ORIENTED_EDGE ( 'NONE', *, *, #16844, .F. ) ;
#30160=DIRECTION ( 'NONE',  ( -1.000000000000000000, 0.000000000000000000, 0.000000000000000000 ) ) ;
#30161=CYLINDRICAL_SURFACE ( 'NONE', #20175, 2.000000000000001776 ) ;
#30162=ORIENTED_EDGE ( 'NONE', *, *, #18929, .F. ) ;
#30163=CARTESIAN_POINT ( 'NONE',  ( 54.99999662536844625, -60.62177826491080168, 17.49999999999999645 ) ) ;
#30164=AXIS2_PLACEMENT_3D ( 'NONE', #206, #4620, #4810 ) ;
#30165=CARTESIAN_POINT ( 'NONE',  ( -50.00000337463109190, 69.28203230275518365, 17.49999999999999645 ) ) ;
#30166=CARTESIAN_POINT ( 'NONE',  ( -52.39915983220772233, -35.19434990244957362, -4.999999999999997335 ) ) ;
#30168=CARTESIAN_POINT ( 'NONE',  ( 6.999996625368676284, -77.94228634059960825, -9.999999999999998224 ) ) ;
#30169=CARTESIAN_POINT ( 'NONE',  ( -35.00000337463117717, -77.94228634059963667, 17.49999999999999645 ) ) ;
#30171=EDGE_LOOP ( 'NONE', ( #15173, #25583, #15013, #31227 ) ) ;
#30172=CARTESIAN_POINT ( 'NONE',  ( 59.99999662536842493, 51.96152422706639129, -5.000000000000000000 ) ) ;
#30174=DIRECTION ( 'NONE',  ( 0.000000000000000000, 0.000000000000000000, 1.000000000000000000 ) ) ;
#30175=DIRECTION ( 'NONE',  ( 0.000000000000000000, 0.000000000000000000, 1.000000000000000000 ) ) ;
#30176=DIRECTION ( 'NONE',  ( 0.000000000000000000, 0.000000000000000000, 1.000000000000000000 ) ) ;
#30179=DIRECTION ( 'NONE',  ( 0.000000000000000000, 0.000000000000000000, -1.000000000000000000 ) ) ;
#30180=LINE ( 'NONE', #21584, #5754 ) ;
#30181=AXIS2_PLACEMENT_3D ( 'NONE', #21478, #15840, #2090 ) ;
#30182=CARTESIAN_POINT ( 'NONE',  ( -62.97617850287781494, -4.279621169095772615, -49.86561046011506448 ) ) ;
#30184=EDGE_CURVE ( 'NONE', #7360, #25770, #13645, .T. ) ;
#30185=DIRECTION ( 'NONE',  ( 1.000000000000000000, 0.000000000000000000, 0.000000000000000000 ) ) ;
#30186=ORIENTED_EDGE ( 'NONE', *, *, #6698, .T. ) ;
#30187=CARTESIAN_POINT ( 'NONE',  ( 84.99999662536832545, 25.98076211353319565, -9.999999999999998224 ) ) ;
#30188=VECTOR ( 'NONE', #12577, 1000.000000000000000 ) ;
#30189=LINE ( 'NONE', #30582, #15825 ) ;
#30191=VECTOR ( 'NONE', #7310, 1000.000000000000000 ) ;
#30192=DIRECTION ( 'NONE',  ( -0.8660254037844449249, -0.4999999999999888978, 0.000000000000000000 ) ) ;
#30193=ORIENTED_EDGE ( 'NONE', *, *, #4288, .T. ) ;
#30194=ORIENTED_EDGE ( 'NONE', *, *, #9959, .T. ) ;
#30195=EDGE_LOOP ( 'NONE', ( #1302, #36120 ) ) ;
#30197=DIRECTION ( 'NONE',  ( 0.000000000000000000, 0.000000000000000000, 1.000000000000000000 ) ) ;
#30198=AXIS2_PLACEMENT_3D ( 'NONE', #26800, #23809, #24167 ) ;
#30199=FACE_OUTER_BOUND ( 'NONE', #7413, .T. ) ;
#30200=CARTESIAN_POINT ( 'NONE',  ( 0.000000000000000000, 0.000000000000000000, -5.000000000000000000 ) ) ;
#30201=FACE_OUTER_BOUND ( 'NONE', #12144, .T. ) ;
#30202=EDGE_LOOP ( 'NONE', ( #14608, #30379, #19583, #13723 ) ) ;
#30203=DIRECTION ( 'NONE',  ( 0.000000000000000000, 0.000000000000000000, 1.000000000000000000 ) ) ;
#30205=EDGE_CURVE ( 'NONE', #29817, #8784, #8847, .T. ) ;
#30206=DIRECTION ( 'NONE',  ( 1.000000000000000000, 0.000000000000000000, 0.000000000000000000 ) ) ;
#30207=CYLINDRICAL_SURFACE ( 'NONE', #32573, 2.000000000000001776 ) ;
#30209=DIRECTION ( 'NONE',  ( 1.000000000000000000, 0.000000000000000000, 0.000000000000000000 ) ) ;
#30212=EDGE_CURVE ( 'NONE', #30829, #1410, #5281, .T. ) ;
#30213=ORIENTED_EDGE ( 'NONE', *, *, #1024, .T. ) ;
#30214=AXIS2_PLACEMENT_3D ( 'NONE', #28106, #31103, #5429 ) ;
#30215=ADVANCED_FACE ( 'NONE', ( #20858 ), #12401, .F. ) ;
#30216=CARTESIAN_POINT ( 'NONE',  ( -55.00000337463107059, 43.30127018922197379, -9.999999999999998224 ) ) ;
#30220=ORIENTED_EDGE ( 'NONE', *, *, #12616, .T. ) ;
#30221=VERTEX_POINT ( 'NONE', #9427 ) ;
#30222=DIRECTION ( 'NONE',  ( 1.000000000000000000, 0.000000000000000000, 0.000000000000000000 ) ) ;
#30223=AXIS2_PLACEMENT_3D ( 'NONE', #35625, #12916, #6930 ) ;
#30224=ORIENTED_EDGE ( 'NONE', *, *, #2468, .T. ) ;
#30226=ORIENTED_EDGE ( 'NONE', *, *, #17225, .T. ) ;
#30227=PLANE ( 'NONE',  #11192 ) ;
#30228=VERTEX_POINT ( 'NONE', #20655 ) ;
#30229=VERTEX_POINT ( 'NONE', #23314 ) ;
#30231=DIRECTION ( 'NONE',  ( 0.000000000000000000, 0.000000000000000000, 1.000000000000000000 ) ) ;
#30232=ADVANCED_FACE ( 'NONE', ( #29466 ), #23488, .F. ) ;
#30233=DIRECTION ( 'NONE',  ( 0.000000000000000000, 0.000000000000000000, -1.000000000000000000 ) ) ;
#30234=EDGE_LOOP ( 'NONE', ( #7895, #2342 ) ) ;
#30235=EDGE_LOOP ( 'NONE', ( #10539, #24244, #14477, #2628 ) ) ;
#30236=DIRECTION ( 'NONE',  ( 1.000000000000000000, 0.000000000000000000, 0.000000000000000000 ) ) ;
#30238=VECTOR ( 'NONE', #27104, 1000.000000000000000 ) ;
#30240=CIRCLE ( 'NONE', #14662, 2.000000000000001776 ) ;
#30241=FACE_OUTER_BOUND ( 'NONE', #26883, .T. ) ;
#30242=ORIENTED_EDGE ( 'NONE', *, *, #24751, .F. ) ;
#30244=VERTEX_POINT ( 'NONE', #6617 ) ;
#30245=DIRECTION ( 'NONE',  ( 0.000000000000000000, 0.000000000000000000, 1.000000000000000000 ) ) ;
#30246=FACE_OUTER_BOUND ( 'NONE', #23141, .T. ) ;
#30247=DIRECTION ( 'NONE',  ( 0.000000000000000000, 0.000000000000000000, -1.000000000000000000 ) ) ;
#30248=DIRECTION ( 'NONE',  ( 0.5000000000000039968, 0.8660254037844363761, 0.000000000000000000 ) ) ;
#30249=DIRECTION ( 'NONE',  ( 0.000000000000000000, 0.000000000000000000, 1.000000000000000000 ) ) ;
#30250=EDGE_CURVE ( 'NONE', #1539, #36932, #9617, .T. ) ;
#30252=CIRCLE ( 'NONE', #23673, 2.000000000000001776 ) ;
#30253=CARTESIAN_POINT ( 'NONE',  ( -27.78182860042817026, -56.67878100130359087, 12.49999999999999822 ) ) ;
#30254=VERTEX_POINT ( 'NONE', #26862 ) ;
#30257=CIRCLE ( 'NONE', #9917, 95.00000000000001421 ) ;
#30258=CARTESIAN_POINT ( 'NONE',  ( 74.99999662536836809, 8.660254037844394404, -5.000000000000000000 ) ) ;
#30259=CARTESIAN_POINT ( 'NONE',  ( 56.99999662536844625, 43.30127018922198801, 12.50000000000000000 ) ) ;
#30260=AXIS2_PLACEMENT_3D ( 'NONE', #27047, #1545, #9988 ) ;
#30261=AXIS2_PLACEMENT_3D ( 'NONE', #34085, #19638, #22263 ) ;
#30263=EDGE_CURVE ( 'NONE', #20675, #6890, #17240, .T. ) ;
#30265=VERTEX_POINT ( 'NONE', #32469 ) ;
#30266=EDGE_LOOP ( 'NONE', ( #8367, #34964, #21524, #8973 ) ) ;
#30267=DIRECTION ( 'NONE',  ( 0.000000000000000000, 0.000000000000000000, 1.000000000000000000 ) ) ;
#30268=FACE_OUTER_BOUND ( 'NONE', #25942, .T. ) ;
#30269=EDGE_CURVE ( 'NONE', #26676, #15417, #18445, .T. ) ;
#30270=EDGE_LOOP ( 'NONE', ( #2065, #10616, #34109, #35024 ) ) ;
#30271=EDGE_CURVE ( 'NONE', #7029, #3626, #22032, .T. ) ;
#30274=DIRECTION ( 'NONE',  ( 0.000000000000000000, 0.000000000000000000, 1.000000000000000000 ) ) ;
#30275=CARTESIAN_POINT ( 'NONE',  ( -20.00000337463124112, 69.28203230275516944, -9.999999999999998224 ) ) ;
#30276=ORIENTED_EDGE ( 'NONE', *, *, #10882, .T. ) ;
#30277=DIRECTION ( 'NONE',  ( 0.000000000000000000, 0.000000000000000000, -1.000000000000000000 ) ) ;
#30278=ORIENTED_EDGE ( 'NONE', *, *, #36622, .F. ) ;
#30279=FACE_BOUND ( 'NONE', #8653, .T. ) ;
#30280=ADVANCED_FACE ( 'NONE', ( #6229 ), #12596, .F. ) ;
#30281=EDGE_CURVE ( 'NONE', #695, #11751, #3620, .T. ) ;
#30282=DIRECTION ( 'NONE',  ( 0.000000000000000000, 0.000000000000000000, 1.000000000000000000 ) ) ;
#30283=DIRECTION ( 'NONE',  ( 1.000000000000000000, 0.000000000000000000, 0.000000000000000000 ) ) ;
#30285=CIRCLE ( 'NONE', #29682, 1.999999999999998224 ) ;
#30289=ORIENTED_EDGE ( 'NONE', *, *, #27213, .F. ) ;
#30290=CARTESIAN_POINT ( 'NONE',  ( 54.99999662536844625, 60.62177826491077326, 12.50000000000000000 ) ) ;
#30292=CIRCLE ( 'NONE', #25504, 2.000000000000001776 ) ;
#30293=PRODUCT_CONTEXT ( 'NONE', #1266, 'mechanical' ) ;
#30296=CARTESIAN_POINT ( 'NONE',  ( -72.00000337463100664, -2.404119930384582903E-14, 12.50000000000000000 ) ) ;
#30297=DIRECTION ( 'NONE',  ( -0.000000000000000000, -0.000000000000000000, -1.000000000000000000 ) ) ;
#30299=CARTESIAN_POINT ( 'NONE',  ( 4.279621169095998212, -62.97617850287780072, 12.49999999999999822 ) ) ;
#30300=CARTESIAN_POINT ( 'NONE',  ( 49.99999662536846756, 51.96152422706637708, -5.000000000000000000 ) ) ;
#30301=ORIENTED_EDGE ( 'NONE', *, *, #24954, .T. ) ;
#30302=CARTESIAN_POINT ( 'NONE',  ( -5.000003374631307729, 77.94228634059957983, 17.49999999999999645 ) ) ;
#30303=AXIS2_PLACEMENT_3D ( 'NONE', #30310, #24697, #33519 ) ;
#30304=DIRECTION ( 'NONE',  ( 1.000000000000000000, 0.000000000000000000, 0.000000000000000000 ) ) ;
#30305=DIRECTION ( 'NONE',  ( 0.000000000000000000, 0.000000000000000000, 1.000000000000000000 ) ) ;
#30307=EDGE_LOOP ( 'NONE', ( #10236, #34805 ) ) ;
#30309=CARTESIAN_POINT ( 'NONE',  ( 82.99999662536831124, -8.660254037844397956, -9.999999999999998224 ) ) ;
#30310=CARTESIAN_POINT ( 'NONE',  ( 69.99999662536838230, -34.64101615137759183, -5.000000000000000000 ) ) ;
#30311=DIRECTION ( 'NONE',  ( 1.000000000000000000, 0.000000000000000000, 0.000000000000000000 ) ) ;
#30314=DIRECTION ( 'NONE',  ( 0.000000000000000000, 0.000000000000000000, 1.000000000000000000 ) ) ;
#30315=CARTESIAN_POINT ( 'NONE',  ( 64.99999662536839651, -60.62177826491080168, -5.000000000000000000 ) ) ;
#30317=VECTOR ( 'NONE', #2900, 1000.000000000000000 ) ;
#30318=AXIS2_PLACEMENT_3D ( 'NONE', #29678, #27441, #32684 ) ;
#30319=DIRECTION ( 'NONE',  ( 0.000000000000000000, 0.000000000000000000, -1.000000000000000000 ) ) ;
#30320=CIRCLE ( 'NONE', #31511, 1.999999999999998224 ) ;
#30321=ORIENTED_EDGE ( 'NONE', *, *, #27526, .F. ) ;
#30322=ORIENTED_EDGE ( 'NONE', *, *, #16762, .F. ) ;
#30323=CARTESIAN_POINT ( 'NONE',  ( 0.000000000000000000, 0.000000000000000000, -5.000000000000000000 ) ) ;
#30324=AXIS2_PLACEMENT_3D ( 'NONE', #19424, #36312, #10424 ) ;
#30325=DIRECTION ( 'NONE',  ( 1.000000000000000000, 0.000000000000000000, 0.000000000000000000 ) ) ;
#30327=DIRECTION ( 'NONE',  ( -1.000000000000000000, 0.000000000000000000, -0.000000000000000000 ) ) ;
#30330=CARTESIAN_POINT ( 'NONE',  ( 14.99999662536859901, 77.94228634059957983, 12.50000000000000000 ) ) ;
#30332=EDGE_CURVE ( 'NONE', #2053, #34151, #13026, .T. ) ;
#30333=CYLINDRICAL_SURFACE ( 'NONE', #12261, 2.000000000000001776 ) ;
#30334=ORIENTED_EDGE ( 'NONE', *, *, #165, .F. ) ;
#30336=CIRCLE ( 'NONE', #36929, 27.00000000000001421 ) ;
#30337=CARTESIAN_POINT ( 'NONE',  ( 14.99999662536859901, 77.94228634059957983, 17.49999999999999645 ) ) ;
#30338=CIRCLE ( 'NONE', #14174, 2.000000000000000000 ) ;
#30339=DIRECTION ( 'NONE',  ( 0.000000000000000000, 0.000000000000000000, 1.000000000000000000 ) ) ;
#30340=DIRECTION ( 'NONE',  ( -1.000000000000000000, 0.000000000000000000, 0.000000000000000000 ) ) ;
#30341=ORIENTED_EDGE ( 'NONE', *, *, #26492, .T. ) ;
#30343=CARTESIAN_POINT ( 'NONE',  ( 31.46585318596250502, 86.45172111230321832, -49.86348611802629449 ) ) ;
#30345=EDGE_LOOP ( 'NONE', ( #9276, #6336, #18054, #34001 ) ) ;
#30348=VERTEX_POINT ( 'NONE', #3433 ) ;
#30349=DIRECTION ( 'NONE',  ( -1.000000000000000000, 0.000000000000000000, 0.000000000000000000 ) ) ;
#30350=VERTEX_POINT ( 'NONE', #14868 ) ;
#30351=DIRECTION ( 'NONE',  ( -1.000000000000000000, 0.000000000000000000, 0.000000000000000000 ) ) ;
#30352=DIRECTION ( 'NONE',  ( -1.000000000000000000, 0.000000000000000000, 0.000000000000000000 ) ) ;
#30353=EDGE_CURVE ( 'NONE', #28869, #2447, #26307, .T. ) ;
#30354=EDGE_CURVE ( 'NONE', #35698, #30350, #33036, .T. ) ;
#30355=AXIS2_PLACEMENT_3D ( 'NONE', #952, #12371, #1502 ) ;
#30356=CARTESIAN_POINT ( 'NONE',  ( 21.99999662536862033, -69.28203230275519786, -9.999999999999998224 ) ) ;
#30357=CARTESIAN_POINT ( 'NONE',  ( -75.00000337463097821, -8.660254037844422825, -9.999999999999998224 ) ) ;
#30358=DIRECTION ( 'NONE',  ( 0.000000000000000000, 0.000000000000000000, 1.000000000000000000 ) ) ;
#30359=DIRECTION ( 'NONE',  ( 1.000000000000000000, 0.000000000000000000, 0.000000000000000000 ) ) ;
#30360=CIRCLE ( 'NONE', #31644, 2.000000000000001776 ) ;
#30361=AXIS2_PLACEMENT_3D ( 'NONE', #30122, #10086, #4275 ) ;
#30362=CARTESIAN_POINT ( 'NONE',  ( 76.99999662536836809, 25.98076211353319565, -9.999999999999998224 ) ) ;
#30363=VERTEX_POINT ( 'NONE', #32860 ) ;
#30364=CIRCLE ( 'NONE', #14198, 2.000000000000001776 ) ;
#30365=ORIENTED_EDGE ( 'NONE', *, *, #1170, .T. ) ;
#30366=EDGE_CURVE ( 'NONE', #22384, #2691, #12422, .T. ) ;
#30367=DIRECTION ( 'NONE',  ( 0.000000000000000000, 0.000000000000000000, 1.000000000000000000 ) ) ;
#30368=VECTOR ( 'NONE', #34026, 1000.000000000000000 ) ;
#30369=CARTESIAN_POINT ( 'NONE',  ( 56.56138580058825482, 61.87160379013676703, 12.50000000000000000 ) ) ;
#30370=CARTESIAN_POINT ( 'NONE',  ( -77.00000337463097821, 25.98076211353318854, -9.999999999999998224 ) ) ;
#30371=DIRECTION ( 'NONE',  ( 1.000000000000000000, 0.000000000000000000, 0.000000000000000000 ) ) ;
#30373=ORIENTED_EDGE ( 'NONE', *, *, #36938, .F. ) ;
#30374=CYLINDRICAL_SURFACE ( 'NONE', #15326, 3.000000000000002665 ) ;
#30375=AXIS2_PLACEMENT_3D ( 'NONE', #31273, #20025, #140 ) ;
#30377=AXIS2_PLACEMENT_3D ( 'NONE', #3660, #1023, #15266 ) ;
#30378=CARTESIAN_POINT ( 'NONE',  ( 64.99999662536839651, 60.62177826491078747, -9.999999999999998224 ) ) ;
#30379=ORIENTED_EDGE ( 'NONE', *, *, #4941, .T. ) ;
#30380=EDGE_CURVE ( 'NONE', #36171, #27334, #471, .T. ) ;
#30382=ORIENTED_EDGE ( 'NONE', *, *, #21456, .F. ) ;
#30383=VECTOR ( 'NONE', #32379, 1000.000000000000000 ) ;
#30384=DIRECTION ( 'NONE',  ( 0.000000000000000000, 0.000000000000000000, 1.000000000000000000 ) ) ;
#30386=DIRECTION ( 'NONE',  ( 0.000000000000000000, -0.000000000000000000, -1.000000000000000000 ) ) ;
#30388=DIRECTION ( 'NONE',  ( 1.000000000000000000, 0.000000000000000000, 0.000000000000000000 ) ) ;
#30389=ORIENTED_EDGE ( 'NONE', *, *, #30542, .T. ) ;
#30390=VERTEX_POINT ( 'NONE', #1348 ) ;
#30392=AXIS2_PLACEMENT_3D ( 'NONE', #4393, #13008, #22369 ) ;
#30393=CIRCLE ( 'NONE', #34585, 2.000000000000001776 ) ;
#30394=DIRECTION ( 'NONE',  ( 0.000000000000000000, 0.000000000000000000, 1.000000000000000000 ) ) ;
#30397=EDGE_CURVE ( 'NONE', #21619, #19686, #27399, .T. ) ;
#30398=FACE_OUTER_BOUND ( 'NONE', #5909, .T. ) ;
#30400=LINE ( 'NONE', #27594, #27092 ) ;
#30401=CARTESIAN_POINT ( 'NONE',  ( -26.97173872511423198, 77.60723454213314199, -5.000000000000000000 ) ) ;
#30402=EDGE_CURVE ( 'NONE', #33336, #15570, #34003, .T. ) ;
#30404=DIRECTION ( 'NONE',  ( 1.000000000000000000, 0.000000000000000000, 0.000000000000000000 ) ) ;
#30405=CIRCLE ( 'NONE', #34594, 2.000000000000001776 ) ;
#30406=CIRCLE ( 'NONE', #16045, 2.000000000000001776 ) ;
#30407=LINE ( 'NONE', #15976, #1802 ) ;
#30409=ORIENTED_EDGE ( 'NONE', *, *, #30046, .F. ) ;
#30410=DIRECTION ( 'NONE',  ( 0.000000000000000000, 0.000000000000000000, 1.000000000000000000 ) ) ;
#30411=ADVANCED_FACE ( 'NONE', ( #7730 ), #1732, .F. ) ;
#30412=FACE_BOUND ( 'NONE', #25320, .T. ) ;
#30413=AXIS2_PLACEMENT_3D ( 'NONE', #12445, #21457, #12634 ) ;
#30414=EDGE_LOOP ( 'NONE', ( #5280, #17369, #551, #6147 ) ) ;
#30415=EDGE_LOOP ( 'NONE', ( #23078, #23418 ) ) ;
#30416=ADVANCED_FACE ( 'NONE', ( #36420 ), #16177, .F. ) ;
#30422=ORIENTED_EDGE ( 'NONE', *, *, #29747, .F. ) ;
#30423=AXIS2_PLACEMENT_3D ( 'NONE', #32523, #23934, #26533 ) ;
#30424=CIRCLE ( 'NONE', #29795, 2.000000000000001776 ) ;
#30425=ORIENTED_EDGE ( 'NONE', *, *, #27435, .T. ) ;
#30426=AXIS2_PLACEMENT_3D ( 'NONE', #514, #29189, #3523 ) ;
#30427=FACE_BOUND ( 'NONE', #18420, .T. ) ;
#30429=ORIENTED_EDGE ( 'NONE', *, *, #20174, .F. ) ;
#30431=VERTEX_POINT ( 'NONE', #7533 ) ;
#30432=EDGE_LOOP ( 'NONE', ( #7355, #4008 ) ) ;
#30433=CIRCLE ( 'NONE', #14272, 2.000000000000001776 ) ;
#30434=EDGE_CURVE ( 'NONE', #20671, #26912, #35208, .T. ) ;
#30435=CARTESIAN_POINT ( 'NONE',  ( 59.13646009116148150, -70.47608876694609137, -4.999999999999997335 ) ) ;
#30436=DIRECTION ( 'NONE',  ( 1.000000000000000000, 0.000000000000000000, 0.000000000000000000 ) ) ;
#30438=ORIENTED_EDGE ( 'NONE', *, *, #16995, .F. ) ;
#30439=CARTESIAN_POINT ( 'NONE',  ( 72.99999662536835388, -43.30127018922199511, 12.50000000000000000 ) ) ;
#30441=CARTESIAN_POINT ( 'NONE',  ( -17.00000337463126243, 77.94228634059957983, -5.000000000000000000 ) ) ;
#30442=EDGE_CURVE ( 'NONE', #13981, #2623, #5864, .T. ) ;
#30443=DIRECTION ( 'NONE',  ( 0.000000000000000000, 0.000000000000000000, 1.000000000000000000 ) ) ;
#30444=CARTESIAN_POINT ( 'NONE',  ( -35.19434990244938888, 52.39915983220783602, 12.49999999999999822 ) ) ;
#30445=ORIENTED_EDGE ( 'NONE', *, *, #24791, .F. ) ;
#30446=LINE ( 'NONE', #15645, #3943 ) ;
#30447=AXIS2_PLACEMENT_3D ( 'NONE', #20245, #5816, #17255 ) ;
#30448=EDGE_CURVE ( 'NONE', #29302, #550, #31596, .T. ) ;
#30449=FACE_BOUND ( 'NONE', #29381, .T. ) ;
#30450=AXIS2_PLACEMENT_3D ( 'NONE', #11264, #14808, #29036 ) ;
#30452=LINE ( 'NONE', #16571, #16602 ) ;
#30453=DIRECTION ( 'NONE',  ( -1.000000000000000000, 0.000000000000000000, 0.000000000000000000 ) ) ;
#30455=VECTOR ( 'NONE', #8718, 1000.000000000000000 ) ;
#30456=CARTESIAN_POINT ( 'NONE',  ( 81.99999662536832545, -17.32050807568879591, -9.999999999999998224 ) ) ;
#30458=CARTESIAN_POINT ( 'NONE',  ( 62.99999662536842493, 43.30127018922200222, -9.999999999999998224 ) ) ;
#30459=VERTEX_POINT ( 'NONE', #15981 ) ;
#30460=CARTESIAN_POINT ( 'NONE',  ( -62.00000337463104927, 34.64101615137757051, -9.999999999999998224 ) ) ;
#30461=FACE_OUTER_BOUND ( 'NONE', #18663, .T. ) ;
#30462=DIRECTION ( 'NONE',  ( 0.000000000000000000, 0.000000000000000000, -1.000000000000000000 ) ) ;
#30463=AXIS2_PLACEMENT_3D ( 'NONE', #31506, #2854, #2650 ) ;
#30465=CIRCLE ( 'NONE', #28661, 2.000000000000000000 ) ;
#30466=ORIENTED_EDGE ( 'NONE', *, *, #28585, .F. ) ;
#30467=ORIENTED_EDGE ( 'NONE', *, *, #12494, .F. ) ;
#30468=EDGE_CURVE ( 'NONE', #8340, #34827, #10679, .T. ) ;
#30471=ORIENTED_EDGE ( 'NONE', *, *, #14446, .F. ) ;
#30473=AXIS2_PLACEMENT_3D ( 'NONE', #2413, #8406, #10662 ) ;
#30475=ORIENTED_EDGE ( 'NONE', *, *, #23477, .F. ) ;
#30476=DIRECTION ( 'NONE',  ( -1.000000000000000000, 0.000000000000000000, 0.000000000000000000 ) ) ;
#30478=ORIENTED_EDGE ( 'NONE', *, *, #18033, .T. ) ;
#30480=CARTESIAN_POINT ( 'NONE',  ( 0.000000000000000000, 0.000000000000000000, 17.49999999999999645 ) ) ;
#30482=CARTESIAN_POINT ( 'NONE',  ( -50.00000337463110611, -69.28203230275519786, 12.50000000000000000 ) ) ;
#30483=DIRECTION ( 'NONE',  ( 0.000000000000000000, 0.000000000000000000, 1.000000000000000000 ) ) ;
#30484=CARTESIAN_POINT ( 'NONE',  ( -70.00000337463102085, -34.64101615137762025, -5.000000000000000000 ) ) ;
#30485=ADVANCED_FACE ( 'NONE', ( #33608 ), #1527, .F. ) ;
#30487=DIRECTION ( 'NONE',  ( 0.000000000000000000, 0.000000000000000000, 1.000000000000000000 ) ) ;
#30491=DIRECTION ( 'NONE',  ( 1.000000000000000000, 0.000000000000000000, 0.000000000000000000 ) ) ;
#30492=DIRECTION ( 'NONE',  ( 0.000000000000000000, 0.000000000000000000, 1.000000000000000000 ) ) ;
#30493=CIRCLE ( 'NONE', #14328, 2.000000000000000000 ) ;
#30495=CARTESIAN_POINT ( 'NONE',  ( -77.00000337463097821, 25.98076211353318854, -9.999999999999998224 ) ) ;
#30496=DIRECTION ( 'NONE',  ( 0.000000000000000000, 0.000000000000000000, 1.000000000000000000 ) ) ;
#30497=ORIENTED_EDGE ( 'NONE', *, *, #5423, .F. ) ;
#30498=CIRCLE ( 'NONE', #25796, 3.000000000000002665 ) ;
#30499=CARTESIAN_POINT ( 'NONE',  ( -8.000003374631249997, -86.60254037844400443, -9.999999999999998224 ) ) ;
#30502=CARTESIAN_POINT ( 'NONE',  ( 82.99999662536832545, 8.660254037844394404, -9.999999999999998224 ) ) ;
#30503=EDGE_CURVE ( 'NONE', #1195, #23444, #2083, .T. ) ;
#30504=VERTEX_POINT ( 'NONE', #10179 ) ;
#30505=CIRCLE ( 'NONE', #13154, 2.000000000000001776 ) ;
#30507=CIRCLE ( 'NONE', #10146, 2.000000000000001776 ) ;
#30510=EDGE_CURVE ( 'NONE', #2177, #20675, #34642, .T. ) ;
#30511=ADVANCED_FACE ( 'NONE', ( #17075 ), #5471, .F. ) ;
#30512=CARTESIAN_POINT ( 'NONE',  ( 47.63139720814400846, -27.50000000000022737, -5.000000000000000000 ) ) ;
#30515=EDGE_CURVE ( 'NONE', #34980, #1135, #17278, .T. ) ;
#30517=DIRECTION ( 'NONE',  ( -1.000000000000000000, 0.000000000000000000, 0.000000000000000000 ) ) ;
#30519=EDGE_CURVE ( 'NONE', #24412, #2691, #7092, .T. ) ;
#30521=CIRCLE ( 'NONE', #35323, 1.999999999999998224 ) ;
#30523=ORIENTED_EDGE ( 'NONE', *, *, #16075, .F. ) ;
#30524=ORIENTED_EDGE ( 'NONE', *, *, #19451, .F. ) ;
#30526=VECTOR ( 'NONE', #13398, 1000.000000000000000 ) ;
#30527=CARTESIAN_POINT ( 'NONE',  ( 49.99999662536846756, 69.28203230275516944, -5.000000000000000000 ) ) ;
#30530=EDGE_LOOP ( 'NONE', ( #22531, #21942, #21322, #30638 ) ) ;
#30532=AXIS2_PLACEMENT_3D ( 'NONE', #18971, #4730, #22326 ) ;
#30533=ADVANCED_FACE ( 'NONE', ( #27962 ), #25178, .F. ) ;
#30534=DIRECTION ( 'NONE',  ( 0.000000000000000000, 0.000000000000000000, -1.000000000000000000 ) ) ;
#30535=DIRECTION ( 'NONE',  ( 0.000000000000000000, 0.000000000000000000, 1.000000000000000000 ) ) ;
#30536=EDGE_LOOP ( 'NONE', ( #1463, #34497, #21708, #13315, #17934 ) ) ;
#30537=DIRECTION ( 'NONE',  ( -1.000000000000000000, 0.000000000000000000, 0.000000000000000000 ) ) ;
#30538=CARTESIAN_POINT ( 'NONE',  ( -5.000003374631307729, 77.94228634059957983, -9.999999999999998224 ) ) ;
#30541=DIRECTION ( 'NONE',  ( -1.000000000000000000, 0.000000000000000000, -0.000000000000000000 ) ) ;
#30542=EDGE_CURVE ( 'NONE', #12595, #21994, #8632, .T. ) ;
#30545=AXIS2_PLACEMENT_3D ( 'NONE', #15850, #27277, #30476 ) ;
#30546=ORIENTED_EDGE ( 'NONE', *, *, #25449, .T. ) ;
#30550=CARTESIAN_POINT ( 'NONE',  ( 74.99999662536835388, -43.30127018922199511, 17.49999999999999645 ) ) ;
#30551=ORIENTED_EDGE ( 'NONE', *, *, #5728, .T. ) ;
#30552=DIRECTION ( 'NONE',  ( 0.000000000000000000, 0.000000000000000000, -1.000000000000000000 ) ) ;
#30554=EDGE_CURVE ( 'NONE', #10919, #20978, #23067, .T. ) ;
#30556=EDGE_CURVE ( 'NONE', #10919, #8273, #20252, .T. ) ;
#30559=DIRECTION ( 'NONE',  ( -1.000000000000000000, 0.000000000000000000, 0.000000000000000000 ) ) ;
#30561=CARTESIAN_POINT ( 'NONE',  ( -3.374631334790434423E-06, 69.28203230275516944, -5.000000000000000000 ) ) ;
#30562=CIRCLE ( 'NONE', #18579, 2.000000000000001776 ) ;
#30564=CARTESIAN_POINT ( 'NONE',  ( -32.00000337463119848, -69.28203230275522628, -9.999999999999998224 ) ) ;
#30565=ORIENTED_EDGE ( 'NONE', *, *, #35889, .T. ) ;
#30566=ORIENTED_EDGE ( 'NONE', *, *, #4999, .F. ) ;
#30568=DIRECTION ( 'NONE',  ( -1.000000000000000000, 0.000000000000000000, 0.000000000000000000 ) ) ;
#30569=DIRECTION ( 'NONE',  ( 1.000000000000000000, 0.000000000000000000, 0.000000000000000000 ) ) ;
#30570=AXIS2_PLACEMENT_3D ( 'NONE', #8681, #20121, #31549 ) ;
#30571=DIRECTION ( 'NONE',  ( 1.000000000000000000, 0.000000000000000000, 0.000000000000000000 ) ) ;
#30572=ORIENTED_EDGE ( 'NONE', *, *, #34824, .T. ) ;
#30573=UNCERTAINTY_MEASURE_WITH_UNIT (LENGTH_MEASURE( 1.000000000000000082E-05 ), #33209, 'distance_accuracy_value', 'NONE');
#30574=DIRECTION ( 'NONE',  ( 1.000000000000000000, 0.000000000000000000, 0.000000000000000000 ) ) ;
#30575=DIRECTION ( 'NONE',  ( 1.000000000000000000, 0.000000000000000000, 0.000000000000000000 ) ) ;
#30576=ORIENTED_EDGE ( 'NONE', *, *, #7829, .T. ) ;
#30577=CYLINDRICAL_SURFACE ( 'NONE', #21222, 2.000000000000001776 ) ;
#30578=CIRCLE ( 'NONE', #13124, 2.000000000000001776 ) ;
#30579=VERTEX_POINT ( 'NONE', #28704 ) ;
#30582=CARTESIAN_POINT ( 'NONE',  ( 44.13139720814401556, -27.50000000000022737, -10.00000000000000000 ) ) ;
#30583=CARTESIAN_POINT ( 'NONE',  ( -48.00000337463110611, -69.28203230275519786, -5.000000000000000000 ) ) ;
#30584=ORIENTED_EDGE ( 'NONE', *, *, #10425, .F. ) ;
#30585=ORIENTED_EDGE ( 'NONE', *, *, #32068, .T. ) ;
#30586=EDGE_LOOP ( 'NONE', ( #12174, #19679 ) ) ;
#30587=CARTESIAN_POINT ( 'NONE',  ( -82.00000337463094979, -17.32050807568882078, -9.999999999999998224 ) ) ;
#30588=CARTESIAN_POINT ( 'NONE',  ( 41.99999662536853151, 69.28203230275518365, -5.000000000000000000 ) ) ;
#30589=DIRECTION ( 'NONE',  ( -1.000000000000000000, 0.000000000000000000, 0.000000000000000000 ) ) ;
#30590=DIRECTION ( 'NONE',  ( 0.000000000000000000, 0.000000000000000000, 1.000000000000000000 ) ) ;
#30591=CARTESIAN_POINT ( 'NONE',  ( 16.49657687835809128, -93.55673653615983199, -5.000000000000000000 ) ) ;
#30592=ORIENTED_EDGE ( 'NONE', *, *, #32863, .F. ) ;
#30593=CARTESIAN_POINT ( 'NONE',  ( 64.99999662536839651, -60.62177826491080168, 12.50000000000000000 ) ) ;
#30595=ADVANCED_FACE ( 'NONE', ( #5837 ), #3032, .F. ) ;
#30596=LINE ( 'NONE', #18787, #9203 ) ;
#30597=EDGE_LOOP ( 'NONE', ( #3573, #27761, #28511, #7997 ) ) ;
#30602=DIRECTION ( 'NONE',  ( 0.000000000000000000, 0.000000000000000000, -1.000000000000000000 ) ) ;
#30603=DIRECTION ( 'NONE',  ( 1.000000000000000000, 0.000000000000000000, 0.000000000000000000 ) ) ;
#30605=ORIENTED_EDGE ( 'NONE', *, *, #11488, .F. ) ;
#30606=EDGE_LOOP ( 'NONE', ( #10361, #30839 ) ) ;
#30607=CARTESIAN_POINT ( 'NONE',  ( -5.000003374631307729, 77.94228634059957983, -9.999999999999998224 ) ) ;
#30609=CIRCLE ( 'NONE', #36035, 2.000000000000001776 ) ;
#30611=EDGE_LOOP ( 'NONE', ( #19585, #15705, #4826, #18965 ) ) ;
#30612=EDGE_CURVE ( 'NONE', #7366, #17904, #14070, .T. ) ;
#30613=ORIENTED_EDGE ( 'NONE', *, *, #37020, .T. ) ;
#30614=DIRECTION ( 'NONE',  ( -1.000000000000000000, 0.000000000000000000, -0.000000000000000000 ) ) ;
#30615=FACE_BOUND ( 'NONE', #24155, .T. ) ;
#30616=ORIENTED_EDGE ( 'NONE', *, *, #4118, .T. ) ;
#30617=VERTEX_POINT ( 'NONE', #2641 ) ;
#30619=DIRECTION ( 'NONE',  ( 1.000000000000000000, 0.000000000000000000, 0.000000000000000000 ) ) ;
#30620=LINE ( 'NONE', #33806, #28248 ) ;
#30621=DIRECTION ( 'NONE',  ( 0.000000000000000000, 0.000000000000000000, 1.000000000000000000 ) ) ;
#30624=FACE_OUTER_BOUND ( 'NONE', #5987, .T. ) ;
#30625=CARTESIAN_POINT ( 'NONE',  ( -85.00000337463092137, -25.98076211353322051, -9.999999999999998224 ) ) ;
#30626=CARTESIAN_POINT ( 'NONE',  ( 74.99999662536836809, 8.660254037844394404, -5.000000000000000000 ) ) ;
#30627=CARTESIAN_POINT ( 'NONE',  ( 74.99999662536835388, -43.30127018922199511, -9.999999999999998224 ) ) ;
#30628=FACE_OUTER_BOUND ( 'NONE', #3073, .T. ) ;
#30629=CARTESIAN_POINT ( 'NONE',  ( -63.00000337463106348, -60.62177826491083010, 17.49999999999999645 ) ) ;
#30631=ADVANCED_FACE ( 'NONE', ( #2474 ), #5089, .T. ) ;
#30632=LINE ( 'NONE', #30458, #19950 ) ;
#30633=ORIENTED_EDGE ( 'NONE', *, *, #1069, .T. ) ;
#30634=DIRECTION ( 'NONE',  ( 0.000000000000000000, 0.000000000000000000, 1.000000000000000000 ) ) ;
#30635=AXIS2_PLACEMENT_3D ( 'NONE', #31162, #31505, #6033 ) ;
#30636=DIRECTION ( 'NONE',  ( 1.000000000000000000, 0.000000000000000000, 0.000000000000000000 ) ) ;
#30637=DIRECTION ( 'NONE',  ( 0.000000000000000000, 0.000000000000000000, 1.000000000000000000 ) ) ;
#30638=ORIENTED_EDGE ( 'NONE', *, *, #21309, .T. ) ;
#30639=ORIENTED_EDGE ( 'NONE', *, *, #22437, .T. ) ;
#30640=EDGE_LOOP ( 'NONE', ( #19993, #26132, #21986, #30186 ) ) ;
#30643=VERTEX_POINT ( 'NONE', #13720 ) ;
#30644=ADVANCED_FACE ( 'NONE', ( #20 ), #22338, .F. ) ;
#30646=LINE ( 'NONE', #34898, #3924 ) ;
#30647=EDGE_LOOP ( 'NONE', ( #36597, #13949 ) ) ;
#30650=VERTEX_POINT ( 'NONE', #34715 ) ;
#30651=LINE ( 'NONE', #36487, #995 ) ;
#30652=ADVANCED_FACE ( 'NONE', ( #571 ), #29606, .F. ) ;
#30653=CARTESIAN_POINT ( 'NONE',  ( 86.99999662536831124, -25.98076211353319565, -5.000000000000000000 ) ) ;
#30654=DIRECTION ( 'NONE',  ( 0.000000000000000000, 0.000000000000000000, 1.000000000000000000 ) ) ;
#30655=AXIS2_PLACEMENT_3D ( 'NONE', #31351, #31190, #20302 ) ;
#30657=ORIENTED_EDGE ( 'NONE', *, *, #22844, .F. ) ;
#30658=FACE_OUTER_BOUND ( 'NONE', #21028, .T. ) ;
#30662=ADVANCED_FACE ( 'NONE', ( #23265 ), #931, .F. ) ;
#30664=CARTESIAN_POINT ( 'NONE',  ( -87.00000337463093558, 25.98076211353317433, 17.49999999999999645 ) ) ;
#30666=ORIENTED_EDGE ( 'NONE', *, *, #10739, .F. ) ;
#30667=CYLINDRICAL_SURFACE ( 'NONE', #452, 2.000000000000001776 ) ;
#30669=CARTESIAN_POINT ( 'NONE',  ( 69.99999662536838230, -34.64101615137759183, -9.999999999999998224 ) ) ;
#30670=AXIS2_PLACEMENT_3D ( 'NONE', #36229, #12973, #24431 ) ;
#30671=ORIENTED_EDGE ( 'NONE', *, *, #29868, .F. ) ;
#30673=DIRECTION ( 'NONE',  ( 0.000000000000000000, 0.000000000000000000, 1.000000000000000000 ) ) ;
#30674=CARTESIAN_POINT ( 'NONE',  ( -55.00000337463107059, 43.30127018922197379, 17.49999999999999645 ) ) ;
#30675=CARTESIAN_POINT ( 'NONE',  ( 72.28378166042060116, 61.53067111003190348, 12.49999999999999822 ) ) ;
#30676=EDGE_CURVE ( 'NONE', #5735, #9729, #13673, .T. ) ;
#30677=ORIENTED_EDGE ( 'NONE', *, *, #6856, .F. ) ;
#30678=ORIENTED_EDGE ( 'NONE', *, *, #18493, .T. ) ;
#30679=AXIS2_PLACEMENT_3D ( 'NONE', #4875, #30552, #27158 ) ;
#30680=CARTESIAN_POINT ( 'NONE',  ( 44.13139720814420031, 27.49999999999988987, -5.000000000000000000 ) ) ;
#30683=CARTESIAN_POINT ( 'NONE',  ( 34.99999662536853862, 77.94228634059959404, -9.999999999999998224 ) ) ;
#30684=ORIENTED_EDGE ( 'NONE', *, *, #22199, .T. ) ;
#30685=EDGE_CURVE ( 'NONE', #9891, #33338, #21465, .T. ) ;
#30686=ORIENTED_EDGE ( 'NONE', *, *, #24375, .T. ) ;
#30687=DIRECTION ( 'NONE',  ( 1.000000000000000000, 0.000000000000000000, 0.000000000000000000 ) ) ;
#30688=ORIENTED_EDGE ( 'NONE', *, *, #2564, .F. ) ;
#30689=ADVANCED_FACE ( 'NONE', ( #24010 ), #11992, .T. ) ;
#30691=ORIENTED_EDGE ( 'NONE', *, *, #22659, .F. ) ;
#30692=DIRECTION ( 'NONE',  ( 1.000000000000000000, 0.000000000000000000, 0.000000000000000000 ) ) ;
#30693=VECTOR ( 'NONE', #8638, 1000.000000000000000 ) ;
#30694=DIRECTION ( 'NONE',  ( 0.000000000000000000, 0.000000000000000000, 1.000000000000000000 ) ) ;
#30697=VERTEX_POINT ( 'NONE', #29250 ) ;
#30700=CARTESIAN_POINT ( 'NONE',  ( 72.99999662536836809, 25.98076211353319565, 12.50000000000000000 ) ) ;
#30701=EDGE_CURVE ( 'NONE', #12539, #27066, #28042, .T. ) ;
#30702=AXIS2_PLACEMENT_3D ( 'NONE', #11024, #22461, #17020 ) ;
#30703=FACE_OUTER_BOUND ( 'NONE', #15187, .T. ) ;
#30704=FACE_OUTER_BOUND ( 'NONE', #16512, .T. ) ;
#30705=ORIENTED_EDGE ( 'NONE', *, *, #27169, .F. ) ;
#30706=AXIS2_PLACEMENT_3D ( 'NONE', #8876, #34573, #17324 ) ;
#30708=CARTESIAN_POINT ( 'NONE',  ( 86.99999662536832545, 8.660254037844394404, 17.49999999999999645 ) ) ;
#30709=CARTESIAN_POINT ( 'NONE',  ( -48.00000337463110611, -69.28203230275519786, 12.50000000000000000 ) ) ;
#30710=VERTEX_POINT ( 'NONE', #3383 ) ;
#30712=CARTESIAN_POINT ( 'NONE',  ( 79.99999662536832545, -17.32050807568879591, -5.000000000000000000 ) ) ;
#30713=EDGE_LOOP ( 'NONE', ( #6000, #31174 ) ) ;
#30714=DIRECTION ( 'NONE',  ( 0.000000000000000000, 0.000000000000000000, -1.000000000000000000 ) ) ;
#30715=CIRCLE ( 'NONE', #25937, 2.000000000000001776 ) ;
#30716=CARTESIAN_POINT ( 'NONE',  ( 84.99999662536832545, 8.660254037844394404, -9.999999999999998224 ) ) ;
#30718=DIRECTION ( 'NONE',  ( 0.8660254037844344888, -0.5000000000000069944, 0.000000000000000000 ) ) ;
#30719=EDGE_CURVE ( 'NONE', #35067, #36125, #24441, .T. ) ;
#30720=DIRECTION ( 'NONE',  ( 1.000000000000000000, 0.000000000000000000, 0.000000000000000000 ) ) ;
#30721=FACE_OUTER_BOUND ( 'NONE', #6466, .T. ) ;
#30722=CYLINDRICAL_SURFACE ( 'NONE', #4555, 2.000000000000000000 ) ;
#30723=EDGE_CURVE ( 'NONE', #2483, #31393, #4694, .T. ) ;
#30724=DIRECTION ( 'NONE',  ( 1.000000000000000000, 0.000000000000000000, 0.000000000000000000 ) ) ;
#30725=CARTESIAN_POINT ( 'NONE',  ( 74.99999662536836809, 25.98076211353319565, -9.999999999999998224 ) ) ;
#30726=ORIENTED_EDGE ( 'NONE', *, *, #8510, .F. ) ;
#30727=EDGE_CURVE ( 'NONE', #25733, #15477, #6026, .T. ) ;
#30728=ORIENTED_EDGE ( 'NONE', *, *, #3575, .T. ) ;
#30730=CIRCLE ( 'NONE', #6797, 1.999999999999998224 ) ;
#30731=DIRECTION ( 'NONE',  ( 1.000000000000000000, 0.000000000000000000, 0.000000000000000000 ) ) ;
#30732=CYLINDRICAL_SURFACE ( 'NONE', #29421, 2.000000000000001776 ) ;
#30733=LINE ( 'NONE', #21744, #24563 ) ;
#30734=ADVANCED_FACE ( 'NONE', ( #9743 ), #12556, .F. ) ;
#30736=EDGE_CURVE ( 'NONE', #4, #5148, #11865, .T. ) ;
#30738=VERTEX_POINT ( 'NONE', #9177 ) ;
#30739=FACE_OUTER_BOUND ( 'NONE', #26656, .T. ) ;
#30740=EDGE_LOOP ( 'NONE', ( #3702, #17349 ) ) ;
#30741=EDGE_CURVE ( 'NONE', #18729, #19586, #17814, .T. ) ;
#30743=DIRECTION ( 'NONE',  ( 1.000000000000000000, 0.000000000000000000, 0.000000000000000000 ) ) ;
#30744=EDGE_CURVE ( 'NONE', #9425, #15109, #22062, .T. ) ;
#30746=DIRECTION ( 'NONE',  ( 0.000000000000000000, 0.000000000000000000, 1.000000000000000000 ) ) ;
#30747=ADVANCED_FACE ( 'NONE', ( #17614 ), #29046, .F. ) ;
#30748=DIRECTION ( 'NONE',  ( 0.000000000000000000, 0.000000000000000000, -1.000000000000000000 ) ) ;
#30749=EDGE_CURVE ( 'NONE', #10183, #6568, #32245, .T. ) ;
#30750=ORIENTED_EDGE ( 'NONE', *, *, #36193, .F. ) ;
#30751=ORIENTED_EDGE ( 'NONE', *, *, #10829, .T. ) ;
#30752=CIRCLE ( 'NONE', #14582, 2.000000000000001776 ) ;
#30754=DIRECTION ( 'NONE',  ( 1.000000000000000000, 0.000000000000000000, 0.000000000000000000 ) ) ;
#30755=AXIS2_PLACEMENT_3D ( 'NONE', #32651, #4351, #9424 ) ;
#30756=DIRECTION ( 'NONE',  ( 0.000000000000000000, 0.000000000000000000, -1.000000000000000000 ) ) ;
#30757=DIRECTION ( 'NONE',  ( 1.000000000000000000, 0.000000000000000000, 0.000000000000000000 ) ) ;
#30758=CYLINDRICAL_SURFACE ( 'NONE', #10928, 2.000000000000001776 ) ;
#30760=VERTEX_POINT ( 'NONE', #12920 ) ;
#30761=AXIS2_PLACEMENT_3D ( 'NONE', #18661, #21470, #26357 ) ;
#30762=LINE ( 'NONE', #25716, #29603 ) ;
#30764=CARTESIAN_POINT ( 'NONE',  ( -45.00000337463111322, -77.94228634059960825, -5.000000000000000000 ) ) ;
#30765=ORIENTED_EDGE ( 'NONE', *, *, #8716, .T. ) ;
#30766=DIRECTION ( 'NONE',  ( 0.000000000000000000, 0.000000000000000000, -1.000000000000000000 ) ) ;
#30769=CIRCLE ( 'NONE', #6202, 2.000000000000001776 ) ;
#30770=ORIENTED_EDGE ( 'NONE', *, *, #34907, .F. ) ;
#30771=DIRECTION ( 'NONE',  ( 0.000000000000000000, 0.000000000000000000, 1.000000000000000000 ) ) ;
#30775=EDGE_LOOP ( 'NONE', ( #34592, #16585, #34381, #1964 ) ) ;
#30777=LINE ( 'NONE', #13906, #5144 ) ;
#30779=ORIENTED_EDGE ( 'NONE', *, *, #26612, .T. ) ;
#30780=CARTESIAN_POINT ( 'NONE',  ( 0.000000000000000000, 0.000000000000000000, 12.49999999999999822 ) ) ;
#30781=ORIENTED_EDGE ( 'NONE', *, *, #25324, .F. ) ;
#30783=CARTESIAN_POINT ( 'NONE',  ( -56.67878100130369035, 27.78182860042797131, 12.49999999999999822 ) ) ;
#30784=DIRECTION ( 'NONE',  ( 0.000000000000000000, 0.000000000000000000, 1.000000000000000000 ) ) ;
#30786=VERTEX_POINT ( 'NONE', #18931 ) ;
#30787=ORIENTED_EDGE ( 'NONE', *, *, #17122, .T. ) ;
#30789=DIRECTION ( 'NONE',  ( 0.000000000000000000, 0.000000000000000000, -1.000000000000000000 ) ) ;
#30792=ORIENTED_EDGE ( 'NONE', *, *, #8986, .T. ) ;
#30793=DIRECTION ( 'NONE',  ( 1.000000000000000000, 0.000000000000000000, 0.000000000000000000 ) ) ;
#30794=FACE_BOUND ( 'NONE', #28837, .T. ) ;
#30795=DIRECTION ( 'NONE',  ( -1.000000000000000000, 0.000000000000000000, 0.000000000000000000 ) ) ;
#30796=FACE_OUTER_BOUND ( 'NONE', #23371, .T. ) ;
#30797=DIRECTION ( 'NONE',  ( 0.000000000000000000, 0.000000000000000000, -1.000000000000000000 ) ) ;
#30798=CARTESIAN_POINT ( 'NONE',  ( 56.29165124598846859, -32.50000000000006395, 12.49999999999999822 ) ) ;
#30799=CIRCLE ( 'NONE', #11625, 3.000000000000006217 ) ;
#30800=CIRCLE ( 'NONE', #12231, 2.000000000000000000 ) ;
#30801=CARTESIAN_POINT ( 'NONE',  ( 49.99999662536846756, -69.28203230275519786, -9.999999999999998224 ) ) ;
#30802=DIRECTION ( 'NONE',  ( 0.000000000000000000, 0.000000000000000000, 1.000000000000000000 ) ) ;
#30803=VERTEX_POINT ( 'NONE', #18578 ) ;
#30805=CARTESIAN_POINT ( 'NONE',  ( 47.99999662536846756, 69.28203230275516944, -9.999999999999998224 ) ) ;
#30806=CYLINDRICAL_SURFACE ( 'NONE', #25921, 2.000000000000001776 ) ;
#30807=EDGE_CURVE ( 'NONE', #33375, #14832, #4721, .T. ) ;
#30808=EDGE_CURVE ( 'NONE', #1450, #16018, #2039, .T. ) ;
#30809=VERTEX_POINT ( 'NONE', #16306 ) ;
#30810=ORIENTED_EDGE ( 'NONE', *, *, #5884, .F. ) ;
#30812=AXIS2_PLACEMENT_3D ( 'NONE', #12093, #23391, #18110 ) ;
#30814=DIRECTION ( 'NONE',  ( 0.000000000000000000, 0.000000000000000000, 1.000000000000000000 ) ) ;
#30815=ORIENTED_EDGE ( 'NONE', *, *, #8202, .F. ) ;
#30816=VECTOR ( 'NONE', #15576, 1000.000000000000000 ) ;
#30817=DIRECTION ( 'NONE',  ( -0.000000000000000000, -0.000000000000000000, 1.000000000000000000 ) ) ;
#30818=EDGE_CURVE ( 'NONE', #23401, #13703, #17295, .T. ) ;
#30819=DIRECTION ( 'NONE',  ( 0.000000000000000000, 0.000000000000000000, 1.000000000000000000 ) ) ;
#30820=VERTEX_POINT ( 'NONE', #36008 ) ;
#30822=ORIENTED_EDGE ( 'NONE', *, *, #35042, .F. ) ;
#30823=FACE_OUTER_BOUND ( 'NONE', #17224, .T. ) ;
#30824=CIRCLE ( 'NONE', #24248, 2.000000000000001776 ) ;
#30825=CIRCLE ( 'NONE', #14074, 3.000000000000002665 ) ;
#30826=CARTESIAN_POINT ( 'NONE',  ( -5.000003374631269537, -77.94228634059960825, 17.49999999999999645 ) ) ;
#30827=DIRECTION ( 'NONE',  ( -1.000000000000000000, 0.000000000000000000, 0.000000000000000000 ) ) ;
#30828=ADVANCED_FACE ( 'NONE', ( #1867 ), #27167, .F. ) ;
#30829=VERTEX_POINT ( 'NONE', #7685 ) ;
#30833=DIRECTION ( 'NONE',  ( 0.000000000000000000, 0.000000000000000000, 1.000000000000000000 ) ) ;
#30837=DIRECTION ( 'NONE',  ( 1.000000000000000000, 0.000000000000000000, 0.000000000000000000 ) ) ;
#30838=DIRECTION ( 'NONE',  ( 1.000000000000000000, 0.000000000000000000, 0.000000000000000000 ) ) ;
#30839=ORIENTED_EDGE ( 'NONE', *, *, #36702, .F. ) ;
#30840=CARTESIAN_POINT ( 'NONE',  ( 31.46585318596250502, 86.45172111230321832, 12.49999999999999822 ) ) ;
#30841=CIRCLE ( 'NONE', #15872, 2.000000000000001776 ) ;
#30842=DIRECTION ( 'NONE',  ( 0.000000000000000000, 0.000000000000000000, 1.000000000000000000 ) ) ;
#30846=ORIENTED_EDGE ( 'NONE', *, *, #20497, .T. ) ;
#30848=ORIENTED_EDGE ( 'NONE', *, *, #29228, .T. ) ;
#30849=FACE_OUTER_BOUND ( 'NONE', #1332, .T. ) ;
#30850=CIRCLE ( 'NONE', #35660, 2.000000000000001776 ) ;
#30851=DIRECTION ( 'NONE',  ( 1.000000000000000000, 0.000000000000000000, 0.000000000000000000 ) ) ;
#30852=CIRCLE ( 'NONE', #18280, 2.000000000000001776 ) ;
#30853=CIRCLE ( 'NONE', #936, 3.499999999999989342 ) ;
#30855=VERTEX_POINT ( 'NONE', #12724 ) ;
#30856=ORIENTED_EDGE ( 'NONE', *, *, #19242, .T. ) ;
#30858=DIRECTION ( 'NONE',  ( 0.000000000000000000, 0.000000000000000000, 1.000000000000000000 ) ) ;
#30859=FACE_OUTER_BOUND ( 'NONE', #34148, .T. ) ;
#30860=EDGE_CURVE ( 'NONE', #7478, #200, #10481, .T. ) ;
#30861=DIRECTION ( 'NONE',  ( 1.000000000000000000, 0.000000000000000000, 0.000000000000000000 ) ) ;
#30862=ORIENTED_EDGE ( 'NONE', *, *, #19213, .F. ) ;
#30863=ORIENTED_EDGE ( 'NONE', *, *, #30250, .T. ) ;
#30864=LINE ( 'NONE', #33882, #27265 ) ;
#30865=EDGE_CURVE ( 'NONE', #27665, #14128, #4696, .T. ) ;
#30866=CIRCLE ( 'NONE', #36876, 33.00000000000001421 ) ;
#30868=EDGE_LOOP ( 'NONE', ( #12801, #14275 ) ) ;
#30869=CIRCLE ( 'NONE', #18295, 2.000000000000001776 ) ;
#30870=CARTESIAN_POINT ( 'NONE',  ( -8.000003374631278419, -69.28203230275519786, 12.50000000000000000 ) ) ;
#30872=FACE_BOUND ( 'NONE', #28714, .T. ) ;
#30875=CIRCLE ( 'NONE', #8721, 2.000000000000001776 ) ;
#30876=AXIS2_PLACEMENT_3D ( 'NONE', #27869, #16831, #19444 ) ;
#30877=CARTESIAN_POINT ( 'NONE',  ( -57.00000337463111322, -43.30127018922202353, -9.999999999999998224 ) ) ;
#30879=EDGE_LOOP ( 'NONE', ( #14, #32234 ) ) ;
#30881=VECTOR ( 'NONE', #37081, 1000.000000000000000 ) ;
#30882=FACE_OUTER_BOUND ( 'NONE', #14172, .T. ) ;
#30883=EDGE_CURVE ( 'NONE', #8438, #23785, #13293, .T. ) ;
#30884=CYLINDRICAL_SURFACE ( 'NONE', #22156, 2.000000000000001776 ) ;
#30885=CYLINDRICAL_SURFACE ( 'NONE', #3548, 2.000000000000001776 ) ;
#30886=VERTEX_POINT ( 'NONE', #21735 ) ;
#30888=LINE ( 'NONE', #19291, #19063 ) ;
#30890=CIRCLE ( 'NONE', #8738, 2.000000000000001776 ) ;
#30892=ORIENTED_EDGE ( 'NONE', *, *, #26308, .T. ) ;
#30893=ORIENTED_EDGE ( 'NONE', *, *, #26331, .T. ) ;
#30894=VECTOR ( 'NONE', #15779, 1000.000000000000000 ) ;
#30895=ADVANCED_FACE ( 'NONE', ( #1689 ), #21371, .F. ) ;
#30896=CYLINDRICAL_SURFACE ( 'NONE', #9619, 2.000000000000001776 ) ;
#30897=ORIENTED_EDGE ( 'NONE', *, *, #35013, .T. ) ;
#30899=DIRECTION ( 'NONE',  ( 0.000000000000000000, 0.000000000000000000, -1.000000000000000000 ) ) ;
#30900=DIRECTION ( 'NONE',  ( 1.000000000000000000, 0.000000000000000000, 0.000000000000000000 ) ) ;
#30901=AXIS2_PLACEMENT_3D ( 'NONE', #33181, #18948, #10498 ) ;
#30903=AXIS2_PLACEMENT_3D ( 'NONE', #18478, #36090, #6832 ) ;
#30904=DIRECTION ( 'NONE',  ( 0.000000000000000000, 0.000000000000000000, -1.000000000000000000 ) ) ;
#30905=AXIS2_PLACEMENT_3D ( 'NONE', #11942, #29190, #23399 ) ;
#30909=DIRECTION ( 'NONE',  ( 0.000000000000000000, 0.000000000000000000, 1.000000000000000000 ) ) ;
#30910=DIRECTION ( 'NONE',  ( 0.000000000000000000, 0.000000000000000000, 1.000000000000000000 ) ) ;
#30911=ORIENTED_EDGE ( 'NONE', *, *, #21914, .F. ) ;
#30912=ORIENTED_EDGE ( 'NONE', *, *, #22187, .T. ) ;
#30913=FACE_OUTER_BOUND ( 'NONE', #20488, .T. ) ;
#30915=CARTESIAN_POINT ( 'NONE',  ( 11.99999662536865763, -69.28203230275519786, -5.000000000000000000 ) ) ;
#30916=CARTESIAN_POINT ( 'NONE',  ( 72.28378166042060116, 61.53067111003190348, -49.22241343995293761 ) ) ;
#30917=DIRECTION ( 'NONE',  ( 1.000000000000000000, 0.000000000000000000, 0.000000000000000000 ) ) ;
#30918=ORIENTED_EDGE ( 'NONE', *, *, #17858, .F. ) ;
#30920=AXIS2_PLACEMENT_3D ( 'NONE', #25372, #36804, #11107 ) ;
#30921=AXIS2_PLACEMENT_3D ( 'NONE', #3921, #7484, #18741 ) ;
#30924=EDGE_LOOP ( 'NONE', ( #11594, #32519 ) ) ;
#30926=CARTESIAN_POINT ( 'NONE',  ( 56.99999662536844625, 60.62177826491077326, -9.999999999999998224 ) ) ;
#30928=AXIS2_PLACEMENT_3D ( 'NONE', #30482, #35562, #4055 ) ;
#30929=LINE ( 'NONE', #33588, #14794 ) ;
#30931=VECTOR ( 'NONE', #32181, 1000.000000000000000 ) ;
#30932=EDGE_CURVE ( 'NONE', #34151, #29420, #28070, .T. ) ;
#30934=VERTEX_POINT ( 'NONE', #26996 ) ;
#30936=ORIENTED_EDGE ( 'NONE', *, *, #28901, .F. ) ;
#30937=ORIENTED_EDGE ( 'NONE', *, *, #34852, .T. ) ;
#30939=ADVANCED_FACE ( 'NONE', ( #14409 ), #19850, .F. ) ;
#30941=ORIENTED_EDGE ( 'NONE', *, *, #5939, .F. ) ;
#30944=ADVANCED_FACE ( 'NONE', ( #13851 ), #33739, .F. ) ;
#30945=CARTESIAN_POINT ( 'NONE',  ( 93.60231327712337190, 15.97563234535636134, 12.49999999999999822 ) ) ;
#30946=CARTESIAN_POINT ( 'NONE',  ( -22.00000337463124112, 69.28203230275516944, -9.999999999999998224 ) ) ;
#30949=ORIENTED_EDGE ( 'NONE', *, *, #4806, .T. ) ;
#30950=DIRECTION ( 'NONE',  ( -0.000000000000000000, -0.000000000000000000, 1.000000000000000000 ) ) ;
#30952=CARTESIAN_POINT ( 'NONE',  ( -20.00000337463123756, -69.28203230275522628, -9.999999999999998224 ) ) ;
#30957=CARTESIAN_POINT ( 'NONE',  ( 2.999999999999768630, -68.00000000000000000, -49.86348611802629449 ) ) ;
#30958=CARTESIAN_POINT ( 'NONE',  ( 27.78182860042856461, 56.67878100130339902, 12.49999999999999822 ) ) ;
#30960=EDGE_CURVE ( 'NONE', #1861, #3252, #24472, .T. ) ;
#30962=VERTEX_POINT ( 'NONE', #5242 ) ;
#30964=ADVANCED_FACE ( 'NONE', ( #30721 ), #27914, .F. ) ;
#30966=CIRCLE ( 'NONE', #18396, 2.000000000000000000 ) ;
#30968=EDGE_CURVE ( 'NONE', #22847, #12612, #33464, .T. ) ;
#30972=EDGE_CURVE ( 'NONE', #14875, #34980, #27458, .T. ) ;
#30973=DIRECTION ( 'NONE',  ( 1.000000000000000000, 0.000000000000000000, 0.000000000000000000 ) ) ;
#30974=VERTEX_POINT ( 'NONE', #22467 ) ;
#30975=ORIENTED_EDGE ( 'NONE', *, *, #25742, .F. ) ;
#30976=AXIS2_PLACEMENT_3D ( 'NONE', #29188, #7070, #13243 ) ;
#30978=DIRECTION ( 'NONE',  ( 0.000000000000000000, 0.000000000000000000, 1.000000000000000000 ) ) ;
#30980=AXIS2_PLACEMENT_3D ( 'NONE', #33457, #16212, #11110 ) ;
#30981=DIRECTION ( 'NONE',  ( 0.000000000000000000, 0.000000000000000000, -1.000000000000000000 ) ) ;
#30983=AXIS2_PLACEMENT_3D ( 'NONE', #29980, #4298, #15729 ) ;
#30984=CARTESIAN_POINT ( 'NONE',  ( -25.00000337463120914, 77.94228634059957983, 12.50000000000000000 ) ) ;
#30986=CARTESIAN_POINT ( 'NONE',  ( -80.00000337463094979, 34.64101615137757051, -9.999999999999998224 ) ) ;
#30987=DIRECTION ( 'NONE',  ( 0.000000000000000000, 0.000000000000000000, 1.000000000000000000 ) ) ;
#30988=ORIENTED_EDGE ( 'NONE', *, *, #32082, .F. ) ;
#30989=EDGE_LOOP ( 'NONE', ( #6048, #15262, #19705 ) ) ;
#30990=LINE ( 'NONE', #26791, #2358 ) ;
#30991=LINE ( 'NONE', #33805, #21350 ) ;
#30994=CYLINDRICAL_SURFACE ( 'NONE', #3709, 2.000000000000001776 ) ;
#30995=CARTESIAN_POINT ( 'NONE',  ( 34.99999662536853862, 77.94228634059959404, 12.50000000000000000 ) ) ;
#30996=CIRCLE ( 'NONE', #8253, 27.00000000000001421 ) ;
#30997=ORIENTED_EDGE ( 'NONE', *, *, #35127, .F. ) ;
#30998=DIRECTION ( 'NONE',  ( 1.000000000000000000, 0.000000000000000000, 0.000000000000000000 ) ) ;
#31000=FACE_BOUND ( 'NONE', #9393, .T. ) ;
#31001=CARTESIAN_POINT ( 'NONE',  ( -60.00000337463108480, -51.96152422706641971, -5.000000000000000000 ) ) ;
#31002=CARTESIAN_POINT ( 'NONE',  ( 61.53067111003264955, -72.28378166041994746, 12.49999999999999822 ) ) ;
#31003=CIRCLE ( 'NONE', #13659, 2.000000000000001776 ) ;
#31004=CARTESIAN_POINT ( 'NONE',  ( 79.99999662536833966, -3.469446951953614189E-15, -5.000000000000000000 ) ) ;
#31005=DIRECTION ( 'NONE',  ( 0.000000000000000000, 0.000000000000000000, 1.000000000000000000 ) ) ;
#31006=DIRECTION ( 'NONE',  ( 0.000000000000000000, 0.000000000000000000, 1.000000000000000000 ) ) ;
#31007=AXIS2_PLACEMENT_3D ( 'NONE', #15704, #7087, #13258 ) ;
#31008=CARTESIAN_POINT ( 'NONE',  ( 41.99999662536853151, 69.28203230275518365, 17.49999999999999645 ) ) ;
#31010=CIRCLE ( 'NONE', #35819, 2.000000000000001776 ) ;
#31011=AXIS2_PLACEMENT_3D ( 'NONE', #1338, #21031, #27024 ) ;
#31012=CARTESIAN_POINT ( 'NONE',  ( 2.778182860042552438, -69.13212189986967360, -4.999999999999997335 ) ) ;
#31013=FACE_OUTER_BOUND ( 'NONE', #2067, .T. ) ;
#31015=ORIENTED_EDGE ( 'NONE', *, *, #12109, .T. ) ;
#31017=ORIENTED_EDGE ( 'NONE', *, *, #5133, .F. ) ;
#31018=ORIENTED_EDGE ( 'NONE', *, *, #10772, .T. ) ;
#31019=AXIS2_PLACEMENT_3D ( 'NONE', #14118, #28195, #11494 ) ;
#31020=EDGE_CURVE ( 'NONE', #12923, #14280, #29859, .T. ) ;
#31021=CARTESIAN_POINT ( 'NONE',  ( -85.00000337463092137, 25.98076211353317433, -9.999999999999998224 ) ) ;
#31022=DIRECTION ( 'NONE',  ( 0.000000000000000000, 0.000000000000000000, 1.000000000000000000 ) ) ;
#31023=ORIENTED_EDGE ( 'NONE', *, *, #3957, .F. ) ;
#31024=AXIS2_PLACEMENT_3D ( 'NONE', #17412, #30910, #31275 ) ;
#31025=DIRECTION ( 'NONE',  ( 0.000000000000000000, 0.000000000000000000, -1.000000000000000000 ) ) ;
#31026=ORIENTED_EDGE ( 'NONE', *, *, #6316, .T. ) ;
#31028=EDGE_LOOP ( 'NONE', ( #30162, #21502, #35720, #35499 ) ) ;
#31029=LINE ( 'NONE', #25054, #365 ) ;
#31030=CIRCLE ( 'NONE', #26853, 2.000000000000001776 ) ;
#31032=LINE ( 'NONE', #25056, #31567 ) ;
#31033=CARTESIAN_POINT ( 'NONE',  ( 59.99999662536843914, -34.64101615137759893, -9.999999999999998224 ) ) ;
#31034=CIRCLE ( 'NONE', #29225, 2.000000000000000000 ) ;
#31035=ORIENTED_EDGE ( 'NONE', *, *, #28554, .T. ) ;
#31037=AXIS2_PLACEMENT_3D ( 'NONE', #25877, #174, #23056 ) ;
#31039=EDGE_CURVE ( 'NONE', #12699, #23292, #13700, .T. ) ;
#31040=FACE_OUTER_BOUND ( 'NONE', #2304, .T. ) ;
#31042=VERTEX_POINT ( 'NONE', #26569 ) ;
#31043=DIRECTION ( 'NONE',  ( 0.5000000000000038858, 0.8660254037844362651, 0.000000000000000000 ) ) ;
#31044=CARTESIAN_POINT ( 'NONE',  ( -65.00000337463102085, 43.30127018922198801, 12.50000000000000000 ) ) ;
#31046=DIRECTION ( 'NONE',  ( -1.156482317317870344E-14, -1.000000000000000000, 0.000000000000000000 ) ) ;
#31047=DIRECTION ( 'NONE',  ( 0.000000000000000000, 0.000000000000000000, 1.000000000000000000 ) ) ;
#31048=DIRECTION ( 'NONE',  ( 0.000000000000000000, -0.000000000000000000, -1.000000000000000000 ) ) ;
#31049=CIRCLE ( 'NONE', #14882, 33.00000000000001421 ) ;
#31050=PLANE ( 'NONE',  #11670 ) ;
#31052=EDGE_CURVE ( 'NONE', #16962, #14513, #19100, .T. ) ;
#31053=CIRCLE ( 'NONE', #2311, 2.000000000000001776 ) ;
#31054=VERTEX_POINT ( 'NONE', #3330 ) ;
#31055=ORIENTED_EDGE ( 'NONE', *, *, #1833, .T. ) ;
#31057=CIRCLE ( 'NONE', #7106, 2.000000000000001776 ) ;
#31058=DIRECTION ( 'NONE',  ( -1.000000000000000000, 0.000000000000000000, 0.000000000000000000 ) ) ;
#31059=VERTEX_POINT ( 'NONE', #11760 ) ;
#31060=EDGE_LOOP ( 'NONE', ( #36705, #8393 ) ) ;
#31061=CIRCLE ( 'NONE', #30447, 65.00000000000000000 ) ;
#31062=EDGE_CURVE ( 'NONE', #148, #17870, #34056, .T. ) ;
#31063=CARTESIAN_POINT ( 'NONE',  ( 4.999996625368645198, 77.94228634059957983, -5.000000000000000000 ) ) ;
#31064=CARTESIAN_POINT ( 'NONE',  ( -62.00000337463104927, 34.64101615137757051, -9.999999999999998224 ) ) ;
#31065=AXIS2_PLACEMENT_3D ( 'NONE', #37085, #25829, #6121 ) ;
#31066=DIRECTION ( 'NONE',  ( 1.000000000000000000, 0.000000000000000000, 0.000000000000000000 ) ) ;
#31068=ORIENTED_EDGE ( 'NONE', *, *, #5759, .F. ) ;
#31069=CYLINDRICAL_SURFACE ( 'NONE', #26090, 2.000000000000001776 ) ;
#31070=CARTESIAN_POINT ( 'NONE',  ( -17.00000337463125533, -77.94228634059960825, 12.50000000000000000 ) ) ;
#31073=CARTESIAN_POINT ( 'NONE',  ( -8.000003374631249997, -86.60254037844400443, 17.49999999999999645 ) ) ;
#31074=ORIENTED_EDGE ( 'NONE', *, *, #6827, .F. ) ;
#31075=DIRECTION ( 'NONE',  ( -1.000000000000000000, 0.000000000000000000, -0.000000000000000000 ) ) ;
#31076=VECTOR ( 'NONE', #22135, 1000.000000000000000 ) ;
#31078=DIRECTION ( 'NONE',  ( 0.000000000000000000, 0.000000000000000000, 1.000000000000000000 ) ) ;
#31079=EDGE_CURVE ( 'NONE', #8482, #10470, #23281, .T. ) ;
#31081=EDGE_CURVE ( 'NONE', #2089, #4841, #1713, .T. ) ;
#31083=CARTESIAN_POINT ( 'NONE',  ( 93.60231327712337190, 15.97563234535636134, -49.86561046011506448 ) ) ;
#31085=DIRECTION ( 'NONE',  ( 1.000000000000000000, 0.000000000000000000, 0.000000000000000000 ) ) ;
#31086=CARTESIAN_POINT ( 'NONE',  ( -75.00000337463097821, 25.98076211353318854, 12.50000000000000000 ) ) ;
#31088=CARTESIAN_POINT ( 'NONE',  ( 9.999996625368618552, 69.28203230275516944, 17.49999999999999645 ) ) ;
#31089=EDGE_CURVE ( 'NONE', #15962, #32853, #321, .T. ) ;
#31090=AXIS2_PLACEMENT_3D ( 'NONE', #19205, #8320, #19917 ) ;
#31093=ORIENTED_EDGE ( 'NONE', *, *, #13693, .T. ) ;
#31094=EDGE_CURVE ( 'NONE', #35130, #5261, #23577, .T. ) ;
#31095=ORIENTED_EDGE ( 'NONE', *, *, #9858, .T. ) ;
#31097=VERTEX_POINT ( 'NONE', #885 ) ;
#31098=CYLINDRICAL_SURFACE ( 'NONE', #15151, 2.000000000000001776 ) ;
#31100=VECTOR ( 'NONE', #34089, 1000.000000000000000 ) ;
#31101=CYLINDRICAL_SURFACE ( 'NONE', #9019, 2.000000000000000000 ) ;
#31102=CIRCLE ( 'NONE', #32928, 2.000000000000001776 ) ;
#31103=DIRECTION ( 'NONE',  ( 0.000000000000000000, -0.000000000000000000, -1.000000000000000000 ) ) ;
#31105=AXIS2_PLACEMENT_3D ( 'NONE', #36640, #33819, #34022 ) ;
#31106=DIRECTION ( 'NONE',  ( -1.000000000000000000, 0.000000000000000000, 0.000000000000000000 ) ) ;
#31107=CARTESIAN_POINT ( 'NONE',  ( 52.39915983220795681, 35.19434990244919703, 12.49999999999999822 ) ) ;
#31108=CARTESIAN_POINT ( 'NONE',  ( -85.00000337463092137, 8.660254037844389075, -9.999999999999998224 ) ) ;
#31110=ORIENTED_EDGE ( 'NONE', *, *, #26125, .T. ) ;
#31111=ORIENTED_EDGE ( 'NONE', *, *, #33594, .F. ) ;
#31112=CARTESIAN_POINT ( 'NONE',  ( -62.00000337463107769, -34.64101615137762025, 12.50000000000000000 ) ) ;
#31113=AXIS2_PLACEMENT_3D ( 'NONE', #35210, #18116, #9693 ) ;
#31114=DIRECTION ( 'NONE',  ( -0.5000000000000098810, -0.8660254037844328234, 0.000000000000000000 ) ) ;
#31115=FACE_OUTER_BOUND ( 'NONE', #15559, .T. ) ;
#31116=DIRECTION ( 'NONE',  ( -0.000000000000000000, -0.000000000000000000, -1.000000000000000000 ) ) ;
#31117=VERTEX_POINT ( 'NONE', #23775 ) ;
#31119=EDGE_CURVE ( 'NONE', #25823, #22212, #223, .T. ) ;
#31120=DIRECTION ( 'NONE',  ( 0.000000000000000000, 0.000000000000000000, 1.000000000000000000 ) ) ;
#31121=EDGE_LOOP ( 'NONE', ( #20251, #19756, #2938, #9659, #11425 ) ) ;
#31122=ORIENTED_EDGE ( 'NONE', *, *, #23499, .T. ) ;
#31123=EDGE_CURVE ( 'NONE', #34040, #33, #4421, .T. ) ;
#31124=DIRECTION ( 'NONE',  ( -0.000000000000000000, -0.000000000000000000, 1.000000000000000000 ) ) ;
#31125=ORIENTED_EDGE ( 'NONE', *, *, #10394, .T. ) ;
#31127=DIRECTION ( 'NONE',  ( -0.000000000000000000, -0.000000000000000000, -1.000000000000000000 ) ) ;
#31128=CARTESIAN_POINT ( 'NONE',  ( -8.000003374631287301, 69.28203230275516944, -9.999999999999998224 ) ) ;
#31130=DIRECTION ( 'NONE',  ( -0.000000000000000000, 0.000000000000000000, -1.000000000000000000 ) ) ;
#31131=CIRCLE ( 'NONE', #8967, 33.00000000000001421 ) ;
#31133=VERTEX_POINT ( 'NONE', #8778 ) ;
#31134=EDGE_CURVE ( 'NONE', #4152, #36749, #1414, .T. ) ;
#31135=AXIS2_PLACEMENT_3D ( 'NONE', #19335, #30756, #5077 ) ;
#31136=EDGE_LOOP ( 'NONE', ( #26134, #3264 ) ) ;
#31137=ORIENTED_EDGE ( 'NONE', *, *, #6821, .T. ) ;
#31138=EDGE_CURVE ( 'NONE', #7314, #18680, #31925, .T. ) ;
#31139=EDGE_LOOP ( 'NONE', ( #8472, #4299 ) ) ;
#31140=DIRECTION ( 'NONE',  ( -1.000000000000000000, 0.000000000000000000, 0.000000000000000000 ) ) ;
#31141=CIRCLE ( 'NONE', #8977, 45.00000000000000711 ) ;
#31142=FACE_OUTER_BOUND ( 'NONE', #4791, .T. ) ;
#31144=DIRECTION ( 'NONE',  ( 1.000000000000000000, 0.000000000000000000, 0.000000000000000000 ) ) ;
#31145=DIRECTION ( 'NONE',  ( 1.000000000000000000, 0.000000000000000000, 0.000000000000000000 ) ) ;
#31147=VERTEX_POINT ( 'NONE', #6526 ) ;
#31148=DIRECTION ( 'NONE',  ( 1.000000000000000000, 0.000000000000000000, 0.000000000000000000 ) ) ;
#31150=CARTESIAN_POINT ( 'NONE',  ( 19.99999662536861678, -86.60254037844400443, 17.49999999999999645 ) ) ;
#31151=VERTEX_POINT ( 'NONE', #31647 ) ;
#31154=DIRECTION ( 'NONE',  ( 0.000000000000000000, 0.000000000000000000, 1.000000000000000000 ) ) ;
#31155=AXIS2_PLACEMENT_3D ( 'NONE', #30378, #27740, #13488 ) ;
#31156=VERTEX_POINT ( 'NONE', #20760 ) ;
#31157=VERTEX_POINT ( 'NONE', #32194 ) ;
#31158=ADVANCED_FACE ( 'NONE', ( #20561 ), #29389, .T. ) ;
#31159=FACE_OUTER_BOUND ( 'NONE', #570, .T. ) ;
#31162=CARTESIAN_POINT ( 'NONE',  ( -5.000003374631269537, -77.94228634059960825, -5.000000000000000000 ) ) ;
#31163=CARTESIAN_POINT ( 'NONE',  ( 89.27079897466126113, -32.49191361593859284, 12.49999999999999822 ) ) ;
#31165=ORIENTED_EDGE ( 'NONE', *, *, #4357, .T. ) ;
#31166=CIRCLE ( 'NONE', #25773, 2.000000000000001776 ) ;
#31170=EDGE_CURVE ( 'NONE', #21416, #16153, #19994, .T. ) ;
#31171=EDGE_CURVE ( 'NONE', #36953, #29140, #30769, .T. ) ;
#31172=DIRECTION ( 'NONE',  ( 0.000000000000000000, 0.000000000000000000, 1.000000000000000000 ) ) ;
#31174=ORIENTED_EDGE ( 'NONE', *, *, #18774, .T. ) ;
#31175=DIRECTION ( 'NONE',  ( 1.000000000000000000, 0.000000000000000000, 0.000000000000000000 ) ) ;
#31176=CARTESIAN_POINT ( 'NONE',  ( 44.99999662536851019, -60.62177826491080168, -5.000000000000000000 ) ) ;
#31178=EDGE_LOOP ( 'NONE', ( #27654, #6628, #8538, #19209 ) ) ;
#31179=EDGE_LOOP ( 'NONE', ( #15675, #20423, #9795, #29558, #19262 ) ) ;
#31180=CARTESIAN_POINT ( 'NONE',  ( 62.97617850287784336, 4.279621169095339184, 12.49999999999999822 ) ) ;
#31181=PLANE ( 'NONE',  #17160 ) ;
#31182=CARTESIAN_POINT ( 'NONE',  ( -69.13212189986965939, -2.778182860042805125, 12.49999999999999645 ) ) ;
#31184=ADVANCED_FACE ( 'NONE', ( #27511 ), #12867, .T. ) ;
#31185=EDGE_LOOP ( 'NONE', ( #19691, #31759, #7816, #15564, #10357 ) ) ;
#31186=CARTESIAN_POINT ( 'NONE',  ( 62.97617850287784336, 4.279621169095339184, 12.49999999999999822 ) ) ;
#31187=CIRCLE ( 'NONE', #32384, 2.000000000000001776 ) ;
#31188=FACE_BOUND ( 'NONE', #3615, .T. ) ;
#31189=DIRECTION ( 'NONE',  ( 1.000000000000000000, 0.000000000000000000, 0.000000000000000000 ) ) ;
#31190=DIRECTION ( 'NONE',  ( 0.000000000000000000, 0.000000000000000000, -1.000000000000000000 ) ) ;
#31191=DIRECTION ( 'NONE',  ( 0.000000000000000000, 0.000000000000000000, -1.000000000000000000 ) ) ;
#31192=DIRECTION ( 'NONE',  ( 0.000000000000000000, -0.000000000000000000, -1.000000000000000000 ) ) ;
#31195=ORIENTED_EDGE ( 'NONE', *, *, #2139, .T. ) ;
#31196=CARTESIAN_POINT ( 'NONE',  ( 46.99999662536849598, -77.94228634059960825, -9.999999999999998224 ) ) ;
#31198=CYLINDRICAL_SURFACE ( 'NONE', #35960, 2.000000000000000000 ) ;
#31199=EDGE_LOOP ( 'NONE', ( #4928, #35785, #11766, #28685 ) ) ;
#31200=ORIENTED_EDGE ( 'NONE', *, *, #21249, .T. ) ;
#31201=ADVANCED_FACE ( 'NONE', ( #24325 ), #4273, .T. ) ;
#31203=DIRECTION ( 'NONE',  ( 1.000000000000000000, 0.000000000000000000, 0.000000000000000000 ) ) ;
#31205=ADVANCED_FACE ( 'NONE', ( #16088 ), #24526, .F. ) ;
#31206=ORIENTED_EDGE ( 'NONE', *, *, #34811, .F. ) ;
#31207=CARTESIAN_POINT ( 'NONE',  ( 62.99999662536839651, -43.30127018922199511, -9.999999999999998224 ) ) ;
#31208=ORIENTED_EDGE ( 'NONE', *, *, #34596, .F. ) ;
#31209=CARTESIAN_POINT ( 'NONE',  ( -60.93295298010992411, -19.13981058454771755, 12.49999999999999822 ) ) ;
#31210=EDGE_LOOP ( 'NONE', ( #1159, #21640, #22918, #1672 ) ) ;
#31211=ADVANCED_FACE ( 'NONE', ( #1828 ), #21132, .F. ) ;
#31212=CARTESIAN_POINT ( 'NONE',  ( 54.99999662536844625, 60.62177826491077326, -5.000000000000000000 ) ) ;
#31214=CARTESIAN_POINT ( 'NONE',  ( -4.279621169095561228, 62.97617850287782915, 12.49999999999999822 ) ) ;
#31215=CARTESIAN_POINT ( 'NONE',  ( -78.38502691089041718, -33.46124879229190441, -5.000000000000000000 ) ) ;
#31216=ORIENTED_EDGE ( 'NONE', *, *, #268, .F. ) ;
#31217=CARTESIAN_POINT ( 'NONE',  ( -62.00000337463107769, -34.64101615137762025, -9.999999999999998224 ) ) ;
#31218=ADVANCED_FACE ( 'NONE', ( #29952 ), #35771, .F. ) ;
#31219=LINE ( 'NONE', #22233, #35664 ) ;
#31220=EDGE_CURVE ( 'NONE', #1450, #14564, #5028, .T. ) ;
#31221=DIRECTION ( 'NONE',  ( -1.000000000000000000, 0.000000000000000000, 0.000000000000000000 ) ) ;
#31223=VERTEX_POINT ( 'NONE', #18703 ) ;
#31224=CYLINDRICAL_SURFACE ( 'NONE', #18946, 2.000000000000001776 ) ;
#31225=CARTESIAN_POINT ( 'NONE',  ( 59.99999662536843914, -34.64101615137759893, 12.50000000000000000 ) ) ;
#31226=EDGE_CURVE ( 'NONE', #36567, #21017, #10990, .T. ) ;
#31227=ORIENTED_EDGE ( 'NONE', *, *, #28666, .F. ) ;
#31228=DIRECTION ( 'NONE',  ( 0.000000000000000000, 0.000000000000000000, 1.000000000000000000 ) ) ;
#31229=CIRCLE ( 'NONE', #25121, 2.000000000000001776 ) ;
#31230=DIRECTION ( 'NONE',  ( 1.000000000000000000, 0.000000000000000000, 0.000000000000000000 ) ) ;
#31231=CARTESIAN_POINT ( 'NONE',  ( 59.99999662536842493, 51.96152422706639129, -9.999999999999998224 ) ) ;
#31232=FACE_OUTER_BOUND ( 'NONE', #1896, .T. ) ;
#31233=VERTEX_POINT ( 'NONE', #18884 ) ;
#31234=ORIENTED_EDGE ( 'NONE', *, *, #13683, .T. ) ;
#31236=LINE ( 'NONE', #5552, #33144 ) ;
#31237=EDGE_LOOP ( 'NONE', ( #18057, #22428 ) ) ;
#31238=VERTEX_POINT ( 'NONE', #1637 ) ;
#31240=DIRECTION ( 'NONE',  ( 0.000000000000000000, 0.000000000000000000, -1.000000000000000000 ) ) ;
#31242=EDGE_CURVE ( 'NONE', #36088, #8851, #15791, .T. ) ;
#31243=ORIENTED_EDGE ( 'NONE', *, *, #35938, .F. ) ;
#31245=DIRECTION ( 'NONE',  ( 0.000000000000000000, -0.000000000000000000, -1.000000000000000000 ) ) ;
#31246=CIRCLE ( 'NONE', #35444, 2.000000000000001776 ) ;
#31247=DIRECTION ( 'NONE',  ( -1.000000000000000000, 0.000000000000000000, 0.000000000000000000 ) ) ;
#31248=VERTEX_POINT ( 'NONE', #4085 ) ;
#31251=FACE_OUTER_BOUND ( 'NONE', #14596, .T. ) ;
#31252=CARTESIAN_POINT ( 'NONE',  ( 9.999996625368618552, 69.28203230275516944, -5.000000000000000000 ) ) ;
#31255=DIRECTION ( 'NONE',  ( 0.5000000000000039968, 0.8660254037844363761, 0.000000000000000000 ) ) ;
#31256=CARTESIAN_POINT ( 'NONE',  ( 66.99999662536839651, -60.62177826491080168, 12.50000000000000000 ) ) ;
#31257=FACE_OUTER_BOUND ( 'NONE', #4287, .T. ) ;
#31258=EDGE_CURVE ( 'NONE', #603, #13910, #23573, .T. ) ;
#31260=DIRECTION ( 'NONE',  ( 0.000000000000000000, 0.000000000000000000, 1.000000000000000000 ) ) ;
#31261=CARTESIAN_POINT ( 'NONE',  ( -45.00000337463111322, 77.94228634059959404, -5.000000000000000000 ) ) ;
#31262=CARTESIAN_POINT ( 'NONE',  ( 81.99999662536832545, -17.32050807568879591, 12.50000000000000000 ) ) ;
#31263=ORIENTED_EDGE ( 'NONE', *, *, #29961, .F. ) ;
#31265=AXIS2_PLACEMENT_3D ( 'NONE', #5675, #11846, #22930 ) ;
#31266=ORIENTED_EDGE ( 'NONE', *, *, #5273, .T. ) ;
#31267=DIRECTION ( 'NONE',  ( 0.000000000000000000, 0.000000000000000000, -1.000000000000000000 ) ) ;
#31268=CARTESIAN_POINT ( 'NONE',  ( -83.45172111230354517, 31.46585318596159553, -4.999999999999997335 ) ) ;
#31269=DIRECTION ( 'NONE',  ( 0.000000000000000000, -0.000000000000000000, -1.000000000000000000 ) ) ;
#31270=CARTESIAN_POINT ( 'NONE',  ( 32.49191361593954497, 89.27079897466093428, 12.49999999999999822 ) ) ;
#31271=DIRECTION ( 'NONE',  ( 1.000000000000000000, 0.000000000000000000, 0.000000000000000000 ) ) ;
#31273=CARTESIAN_POINT ( 'NONE',  ( 52.39915983220795681, 35.19434990244919703, -4.999999999999997335 ) ) ;
#31274=EDGE_CURVE ( 'NONE', #3592, #281, #29553, .T. ) ;
#31275=DIRECTION ( 'NONE',  ( 1.000000000000000000, 0.000000000000000000, 0.000000000000000000 ) ) ;
#31276=EDGE_CURVE ( 'NONE', #8319, #32142, #2029, .T. ) ;
#31277=ORIENTED_EDGE ( 'NONE', *, *, #18993, .T. ) ;
#31278=VERTEX_POINT ( 'NONE', #4645 ) ;
#31279=CIRCLE ( 'NONE', #1953, 2.000000000000001776 ) ;
#31280=DIRECTION ( 'NONE',  ( 1.000000000000000000, 0.000000000000000000, 0.000000000000000000 ) ) ;
#31283=DIRECTION ( 'NONE',  ( 1.000000000000000000, 0.000000000000000000, 0.000000000000000000 ) ) ;
#31284=ADVANCED_FACE ( 'NONE', ( #33321 ), #7639, .T. ) ;
#31286=EDGE_CURVE ( 'NONE', #35776, #10733, #28966, .T. ) ;
#31287=FACE_BOUND ( 'NONE', #22824, .T. ) ;
#31288=ORIENTED_EDGE ( 'NONE', *, *, #18119, .T. ) ;
#31291=AXIS2_PLACEMENT_3D ( 'NONE', #32347, #9831, #6663 ) ;
#31292=DIRECTION ( 'NONE',  ( 0.000000000000000000, 0.000000000000000000, 1.000000000000000000 ) ) ;
#31293=EDGE_LOOP ( 'NONE', ( #2778, #6108 ) ) ;
#31295=CARTESIAN_POINT ( 'NONE',  ( 7.999996625368625658, 86.60254037844397601, 12.50000000000000000 ) ) ;
#31298=LINE ( 'NONE', #2819, #36453 ) ;
#31299=ADVANCED_FACE ( 'NONE', ( #16634 ), #33693, .T. ) ;
#31300=ORIENTED_EDGE ( 'NONE', *, *, #2094, .T. ) ;
#31301=ORIENTED_EDGE ( 'NONE', *, *, #31527, .F. ) ;
#31302=ORIENTED_EDGE ( 'NONE', *, *, #31123, .F. ) ;
#31304=AXIS2_PLACEMENT_3D ( 'NONE', #35634, #1696, #1492 ) ;
#31306=CARTESIAN_POINT ( 'NONE',  ( -59.13646009116099833, 70.47608876694653190, -4.999999999999997335 ) ) ;
#31310=DIRECTION ( 'NONE',  ( 1.000000000000000000, 0.000000000000000000, 0.000000000000000000 ) ) ;
#31311=ORIENTED_EDGE ( 'NONE', *, *, #3137, .F. ) ;
#31314=EDGE_CURVE ( 'NONE', #19087, #25741, #18794, .T. ) ;
#31315=CARTESIAN_POINT ( 'NONE',  ( 83.67878100130371877, -27.78182860042797131, 12.49999999999999822 ) ) ;
#31317=DIRECTION ( 'NONE',  ( 1.000000000000000000, 0.000000000000000000, 0.000000000000000000 ) ) ;
#31319=ORIENTED_EDGE ( 'NONE', *, *, #3932, .F. ) ;
#31320=ORIENTED_EDGE ( 'NONE', *, *, #13095, .F. ) ;
#31321=CARTESIAN_POINT ( 'NONE',  ( -75.00000337463097821, 8.660254037844374864, -9.999999999999998224 ) ) ;
#31323=DIRECTION ( 'NONE',  ( 0.000000000000000000, 0.000000000000000000, 1.000000000000000000 ) ) ;
#31324=DIRECTION ( 'NONE',  ( -1.000000000000000000, 0.000000000000000000, -0.000000000000000000 ) ) ;
#31327=EDGE_LOOP ( 'NONE', ( #30705, #10994, #2617, #13557 ) ) ;
#31328=CIRCLE ( 'NONE', #33125, 2.000000000000001776 ) ;
#31331=EDGE_CURVE ( 'NONE', #20247, #16338, #7998, .T. ) ;
#31332=ORIENTED_EDGE ( 'NONE', *, *, #18488, .F. ) ;
#31333=FACE_BOUND ( 'NONE', #21474, .T. ) ;
#31334=ORIENTED_EDGE ( 'NONE', *, *, #25903, .F. ) ;
#31335=EDGE_LOOP ( 'NONE', ( #16337, #1117, #26946 ) ) ;
#31336=CARTESIAN_POINT ( 'NONE',  ( -60.00000337463107059, -34.64101615137762025, -9.999999999999998224 ) ) ;
#31337=CARTESIAN_POINT ( 'NONE',  ( -8.000003374631249997, -86.60254037844400443, -9.999999999999998224 ) ) ;
#31339=DIRECTION ( 'NONE',  ( 0.000000000000000000, 0.000000000000000000, 1.000000000000000000 ) ) ;
#31340=EDGE_LOOP ( 'NONE', ( #24197, #30382, #23894, #11167 ) ) ;
#31341=ORIENTED_EDGE ( 'NONE', *, *, #9131, .F. ) ;
#31343=LINE ( 'NONE', #20099, #22560 ) ;
#31344=FACE_OUTER_BOUND ( 'NONE', #2779, .T. ) ;
#31347=ORIENTED_EDGE ( 'NONE', *, *, #3953, .F. ) ;
#31348=CARTESIAN_POINT ( 'NONE',  ( 59.99999662536845335, 34.64101615137759893, -9.999999999999998224 ) ) ;
#31349=FACE_BOUND ( 'NONE', #14308, .T. ) ;
#31350=CARTESIAN_POINT ( 'NONE',  ( 54.99999662536844625, 60.62177826491077326, -9.999999999999998224 ) ) ;
#31351=CARTESIAN_POINT ( 'NONE',  ( 0.000000000000000000, 0.000000000000000000, -5.000000000000000000 ) ) ;
#31352=DIRECTION ( 'NONE',  ( -0.4999999999999980016, 0.8660254037844398178, 0.000000000000000000 ) ) ;
#31353=DIRECTION ( 'NONE',  ( 0.000000000000000000, 0.000000000000000000, -1.000000000000000000 ) ) ;
#31355=AXIS2_PLACEMENT_3D ( 'NONE', #20221, #14966, #29199 ) ;
#31356=DIRECTION ( 'NONE',  ( 1.000000000000000000, 0.000000000000000000, 0.000000000000000000 ) ) ;
#31358=CARTESIAN_POINT ( 'NONE',  ( -52.00000337463112032, -51.96152422706641971, 12.50000000000000000 ) ) ;
#31359=EDGE_LOOP ( 'NONE', ( #36822, #17601, #4707, #30193, #28019, #33184 ) ) ;
#31360=CARTESIAN_POINT ( 'NONE',  ( -75.00000337463100664, -43.30127018922202353, 17.49999999999999645 ) ) ;
#31361=DIRECTION ( 'NONE',  ( 0.000000000000000000, 0.000000000000000000, -1.000000000000000000 ) ) ;
#31362=LINE ( 'NONE', #11121, #26971 ) ;
#31365=ORIENTED_EDGE ( 'NONE', *, *, #3584, .T. ) ;
#31366=EDGE_LOOP ( 'NONE', ( #33908, #32247 ) ) ;
#31367=CIRCLE ( 'NONE', #34383, 2.000000000000001776 ) ;
#31368=CARTESIAN_POINT ( 'NONE',  ( -51.13139720814437084, -27.49999999999955591, -5.000000000000000000 ) ) ;
#31369=DIRECTION ( 'NONE',  ( 0.000000000000000000, 0.000000000000000000, 1.000000000000000000 ) ) ;
#31372=DIRECTION ( 'NONE',  ( 0.000000000000000000, 0.000000000000000000, 1.000000000000000000 ) ) ;
#31373=EDGE_CURVE ( 'NONE', #22617, #1670, #821, .T. ) ;
#31374=VERTEX_POINT ( 'NONE', #30680 ) ;
#31375=DIRECTION ( 'NONE',  ( 0.000000000000000000, 0.000000000000000000, 1.000000000000000000 ) ) ;
#31376=ORIENTED_EDGE ( 'NONE', *, *, #33121, .T. ) ;
#31377=DIRECTION ( 'NONE',  ( 1.000000000000000000, 0.000000000000000000, 0.000000000000000000 ) ) ;
#31379=EDGE_LOOP ( 'NONE', ( #34033, #1716 ) ) ;
#31380=AXIS2_PLACEMENT_3D ( 'NONE', #24101, #10901, #27969 ) ;
#31382=CARTESIAN_POINT ( 'NONE',  ( 74.99999662536836809, 8.660254037844394404, -9.999999999999998224 ) ) ;
#31383=VERTEX_POINT ( 'NONE', #36869 ) ;
#31384=DIRECTION ( 'NONE',  ( 0.000000000000000000, 0.000000000000000000, 1.000000000000000000 ) ) ;
#31386=CARTESIAN_POINT ( 'NONE',  ( -72.00000337463102085, -51.96152422706641971, -5.000000000000000000 ) ) ;
#31387=DIRECTION ( 'NONE',  ( 0.000000000000000000, 0.000000000000000000, -1.000000000000000000 ) ) ;
#31388=EDGE_CURVE ( 'NONE', #393, #5725, #34370, .T. ) ;
#31389=VERTEX_POINT ( 'NONE', #2561 ) ;
#31390=CIRCLE ( 'NONE', #27809, 2.000000000000001776 ) ;
#31391=DIRECTION ( 'NONE',  ( -0.000000000000000000, -0.000000000000000000, 1.000000000000000000 ) ) ;
#31392=CARTESIAN_POINT ( 'NONE',  ( -61.53067111003215217, 72.28378166042038799, 12.49999999999999822 ) ) ;
#31393=VERTEX_POINT ( 'NONE', #34257 ) ;
#31394=EDGE_CURVE ( 'NONE', #14998, #11018, #19988, .T. ) ;
#31395=DIRECTION ( 'NONE',  ( -1.047444401652940795E-14, -1.000000000000000000, 0.000000000000000000 ) ) ;
#31396=DIRECTION ( 'NONE',  ( -1.000000000000000000, 0.000000000000000000, 0.000000000000000000 ) ) ;
#31397=LINE ( 'NONE', #23162, #35129 ) ;
#31398=FACE_OUTER_BOUND ( 'NONE', #13046, .T. ) ;
#31399=EDGE_CURVE ( 'NONE', #4235, #6394, #18190, .T. ) ;
#31400=ORIENTED_EDGE ( 'NONE', *, *, #12325, .T. ) ;
#31401=CIRCLE ( 'NONE', #7542, 95.00000000000001421 ) ;
#31402=ORIENTED_EDGE ( 'NONE', *, *, #28573, .T. ) ;
#31403=VECTOR ( 'NONE', #22980, 1000.000000000000000 ) ;
#31404=EDGE_CURVE ( 'NONE', #35276, #5559, #36325, .T. ) ;
#31405=DIRECTION ( 'NONE',  ( 0.000000000000000000, 0.000000000000000000, 1.000000000000000000 ) ) ;
#31406=DIRECTION ( 'NONE',  ( 1.000000000000000000, 0.000000000000000000, 0.000000000000000000 ) ) ;
#31408=AXIS2_PLACEMENT_3D ( 'NONE', #15015, #6191, #35462 ) ;
#31409=ORIENTED_EDGE ( 'NONE', *, *, #2564, .T. ) ;
#31412=DIRECTION ( 'NONE',  ( -1.000000000000000000, 0.000000000000000000, 0.000000000000000000 ) ) ;
#31413=CARTESIAN_POINT ( 'NONE',  ( -50.00000337463112032, -51.96152422706641971, -9.999999999999998224 ) ) ;
#31414=EDGE_CURVE ( 'NONE', #34083, #35809, #17017, .T. ) ;
#31415=CIRCLE ( 'NONE', #16440, 2.000000000000000000 ) ;
#31416=AXIS2_PLACEMENT_3D ( 'NONE', #14595, #4468, #9545 ) ;
#31418=EDGE_LOOP ( 'NONE', ( #14786, #9948 ) ) ;
#31420=EDGE_CURVE ( 'NONE', #4355, #26422, #22256, .T. ) ;
#31422=CARTESIAN_POINT ( 'NONE',  ( 59.99999662536842493, 51.96152422706639129, 17.49999999999999645 ) ) ;
#31423=ORIENTED_EDGE ( 'NONE', *, *, #17345, .T. ) ;
#31424=EDGE_CURVE ( 'NONE', #29605, #6350, #28063, .T. ) ;
#31425=EDGE_CURVE ( 'NONE', #29624, #29503, #5640, .T. ) ;
#31426=DIRECTION ( 'NONE',  ( 0.000000000000000000, 0.000000000000000000, 1.000000000000000000 ) ) ;
#31427=ORIENTED_EDGE ( 'NONE', *, *, #4989, .F. ) ;
#31428=FACE_BOUND ( 'NONE', #4009, .T. ) ;
#31430=CIRCLE ( 'NONE', #32606, 2.000000000000001776 ) ;
#31431=CARTESIAN_POINT ( 'NONE',  ( 24.99999662536857059, 77.94228634059957983, 12.50000000000000000 ) ) ;
#31432=CIRCLE ( 'NONE', #14676, 27.00000000000001421 ) ;
#31433=ORIENTED_EDGE ( 'NONE', *, *, #30048, .F. ) ;
#31436=CIRCLE ( 'NONE', #9896, 2.000000000000001776 ) ;
#31438=LINE ( 'NONE', #28981, #7169 ) ;
#31439=CARTESIAN_POINT ( 'NONE',  ( -30.00000337463118427, 69.28203230275516944, -5.000000000000000000 ) ) ;
#31441=DIRECTION ( 'NONE',  ( 0.8660254037844347108, -0.5000000000000067724, 0.000000000000000000 ) ) ;
#31442=CARTESIAN_POINT ( 'NONE',  ( 81.99999662536833966, -3.469446951953614189E-15, -9.999999999999998224 ) ) ;
#31443=CARTESIAN_POINT ( 'NONE',  ( -53.00000337463106348, 43.30127018922197379, 17.49999999999999645 ) ) ;
#31446=EDGE_LOOP ( 'NONE', ( #9384, #20804, #33399, #29439, #31562, #24082 ) ) ;
#31448=CARTESIAN_POINT ( 'NONE',  ( 59.99999662536842493, -51.96152422706639840, 17.49999999999999645 ) ) ;
#31450=DIRECTION ( 'NONE',  ( 0.000000000000000000, 0.000000000000000000, 1.000000000000000000 ) ) ;
#31451=DIRECTION ( 'NONE',  ( 0.000000000000000000, 0.000000000000000000, -1.000000000000000000 ) ) ;
#31455=AXIS2_PLACEMENT_3D ( 'NONE', #1792, #16232, #35930 ) ;
#31458=ORIENTED_EDGE ( 'NONE', *, *, #20665, .F. ) ;
#31460=ADVANCED_FACE ( 'NONE', ( #32152 ), #6287, .F. ) ;
#31461=DIRECTION ( 'NONE',  ( -0.000000000000000000, -0.000000000000000000, 1.000000000000000000 ) ) ;
#31462=CYLINDRICAL_SURFACE ( 'NONE', #24504, 1.999999999999998224 ) ;
#31463=ORIENTED_EDGE ( 'NONE', *, *, #8649, .F. ) ;
#31465=FACE_BOUND ( 'NONE', #16980, .T. ) ;
#31466=EDGE_LOOP ( 'NONE', ( #13522, #36902, #2494, #1489 ) ) ;
#31467=ORIENTED_EDGE ( 'NONE', *, *, #27781, .F. ) ;
#31469=ORIENTED_EDGE ( 'NONE', *, *, #26233, .T. ) ;
#31471=DIRECTION ( 'NONE',  ( 0.000000000000000000, 0.000000000000000000, -1.000000000000000000 ) ) ;
#31473=DIRECTION ( 'NONE',  ( 0.000000000000000000, 0.000000000000000000, 1.000000000000000000 ) ) ;
#31474=ORIENTED_EDGE ( 'NONE', *, *, #11427, .F. ) ;
#31475=AXIS2_PLACEMENT_3D ( 'NONE', #30593, #25518, #31148 ) ;
#31476=EDGE_LOOP ( 'NONE', ( #30691, #34832, #9069, #1936 ) ) ;
#31477=VECTOR ( 'NONE', #13065, 1000.000000000000000 ) ;
#31478=ORIENTED_EDGE ( 'NONE', *, *, #8414, .F. ) ;
#31479=AXIS2_PLACEMENT_3D ( 'NONE', #18947, #18759, #21582 ) ;
#31482=ORIENTED_EDGE ( 'NONE', *, *, #3108, .T. ) ;
#31483=CIRCLE ( 'NONE', #27324, 2.000000000000001776 ) ;
#31484=EDGE_LOOP ( 'NONE', ( #9634, #26037 ) ) ;
#31485=DIRECTION ( 'NONE',  ( 0.000000000000000000, 0.000000000000000000, 1.000000000000000000 ) ) ;
#31486=CARTESIAN_POINT ( 'NONE',  ( -10.00000337463125000, -86.60254037844400443, 17.49999999999999645 ) ) ;
#31487=CARTESIAN_POINT ( 'NONE',  ( 0.000000000000000000, 0.000000000000000000, -5.000000000000000000 ) ) ;
#31489=DIRECTION ( 'NONE',  ( 0.000000000000000000, 0.000000000000000000, -1.000000000000000000 ) ) ;
#31490=VERTEX_POINT ( 'NONE', #3494 ) ;
#31491=DIRECTION ( 'NONE',  ( 0.000000000000000000, 0.000000000000000000, 1.000000000000000000 ) ) ;
#31492=AXIS2_PLACEMENT_3D ( 'NONE', #8207, #11545, #36534 ) ;
#31493=LINE ( 'NONE', #14449, #3618 ) ;
#31494=DIRECTION ( 'NONE',  ( 1.000000000000000000, 0.000000000000000000, 0.000000000000000000 ) ) ;
#31495=ORIENTED_EDGE ( 'NONE', *, *, #12325, .F. ) ;
#31496=DIRECTION ( 'NONE',  ( 0.000000000000000000, 0.000000000000000000, 1.000000000000000000 ) ) ;
#31498=ORIENTED_EDGE ( 'NONE', *, *, #16239, .T. ) ;
#31499=AXIS2_PLACEMENT_3D ( 'NONE', #12800, #27067, #10014 ) ;
#31500=ORIENTED_EDGE ( 'NONE', *, *, #6232, .T. ) ;
#31501=DIRECTION ( 'NONE',  ( 1.000000000000000000, 0.000000000000000000, 0.000000000000000000 ) ) ;
#31502=CIRCLE ( 'NONE', #21316, 2.000000000000001776 ) ;
#31503=CARTESIAN_POINT ( 'NONE',  ( -80.00000337463096400, -34.64101615137762025, -9.999999999999998224 ) ) ;
#31505=DIRECTION ( 'NONE',  ( 0.000000000000000000, 0.000000000000000000, -1.000000000000000000 ) ) ;
#31506=CARTESIAN_POINT ( 'NONE',  ( -65.00000337463104927, -25.98076211353322051, -9.999999999999998224 ) ) ;
#31507=ORIENTED_EDGE ( 'NONE', *, *, #34334, .F. ) ;
#31508=EDGE_LOOP ( 'NONE', ( #31546, #25816, #32148, #9780, #33834 ) ) ;
#31510=CIRCLE ( 'NONE', #12332, 2.000000000000001776 ) ;
#31511=AXIS2_PLACEMENT_3D ( 'NONE', #24191, #30006, #27008 ) ;
#31512=DIRECTION ( 'NONE',  ( 0.000000000000000000, 0.000000000000000000, 1.000000000000000000 ) ) ;
#31513=LINE ( 'NONE', #17293, #32667 ) ;
#31514=AXIS2_PLACEMENT_3D ( 'NONE', #1349, #12967, #15425 ) ;
#31516=AXIS2_PLACEMENT_3D ( 'NONE', #4988, #10811, #10252 ) ;
#31517=ORIENTED_EDGE ( 'NONE', *, *, #67, .F. ) ;
#31518=DIRECTION ( 'NONE',  ( 0.000000000000000000, 0.000000000000000000, 1.000000000000000000 ) ) ;
#31519=EDGE_LOOP ( 'NONE', ( #4329, #3768, #26911, #1979, #27688 ) ) ;
#31520=ORIENTED_EDGE ( 'NONE', *, *, #21359, .F. ) ;
#31521=LINE ( 'NONE', #36297, #21174 ) ;
#31522=EDGE_CURVE ( 'NONE', #27267, #35279, #28384, .T. ) ;
#31524=ORIENTED_EDGE ( 'NONE', *, *, #18347, .T. ) ;
#31527=EDGE_CURVE ( 'NONE', #36437, #26422, #8635, .T. ) ;
#31528=AXIS2_PLACEMENT_3D ( 'NONE', #23299, #20464, #9039 ) ;
#31529=DIRECTION ( 'NONE',  ( 0.000000000000000000, 0.000000000000000000, -1.000000000000000000 ) ) ;
#31530=CARTESIAN_POINT ( 'NONE',  ( -15.00000337463125710, -77.94228634059960825, 12.50000000000000000 ) ) ;
#31531=CIRCLE ( 'NONE', #26141, 2.000000000000001776 ) ;
#31534=FACE_BOUND ( 'NONE', #36233, .T. ) ;
#31536=FACE_OUTER_BOUND ( 'NONE', #24073, .T. ) ;
#31537=DIRECTION ( 'NONE',  ( 1.000000000000000000, 0.000000000000000000, 0.000000000000000000 ) ) ;
#31539=AXIS2_PLACEMENT_3D ( 'NONE', #12861, #30673, #19081 ) ;
#31540=DIRECTION ( 'NONE',  ( 1.000000000000000000, 0.000000000000000000, 0.000000000000000000 ) ) ;
#31544=ADVANCED_FACE ( 'NONE', ( #108 ), #6110, .F. ) ;
#31545=DIRECTION ( 'NONE',  ( 0.000000000000000000, 0.000000000000000000, 1.000000000000000000 ) ) ;
#31546=ORIENTED_EDGE ( 'NONE', *, *, #36728, .F. ) ;
#31547=DIRECTION ( 'NONE',  ( 0.000000000000000000, 0.000000000000000000, 1.000000000000000000 ) ) ;
#31549=DIRECTION ( 'NONE',  ( -1.000000000000000000, 0.000000000000000000, 0.000000000000000000 ) ) ;
#31550=ORIENTED_EDGE ( 'NONE', *, *, #28921, .F. ) ;
#31551=CIRCLE ( 'NONE', #21368, 2.000000000000000000 ) ;
#31552=EDGE_LOOP ( 'NONE', ( #13239, #29908 ) ) ;
#31554=DIRECTION ( 'NONE',  ( 1.000000000000000000, 0.000000000000000000, 0.000000000000000000 ) ) ;
#31555=DIRECTION ( 'NONE',  ( 1.000000000000000000, 0.000000000000000000, 0.000000000000000000 ) ) ;
#31556=CARTESIAN_POINT ( 'NONE',  ( -5.000003374631269537, -77.94228634059960825, -5.000000000000000000 ) ) ;
#31557=ORIENTED_EDGE ( 'NONE', *, *, #17999, .F. ) ;
#31558=CIRCLE ( 'NONE', #28568, 2.000000000000001776 ) ;
#31561=AXIS2_PLACEMENT_3D ( 'NONE', #25034, #36466, #36273 ) ;
#31562=ORIENTED_EDGE ( 'NONE', *, *, #24443, .T. ) ;
#31564=EDGE_LOOP ( 'NONE', ( #28983, #30301 ) ) ;
#31565=DIRECTION ( 'NONE',  ( 0.000000000000000000, 0.000000000000000000, 1.000000000000000000 ) ) ;
#31566=ORIENTED_EDGE ( 'NONE', *, *, #8787, .F. ) ;
#31567=VECTOR ( 'NONE', #36490, 1000.000000000000000 ) ;
#31568=EDGE_LOOP ( 'NONE', ( #1731, #13679 ) ) ;
#31569=EDGE_CURVE ( 'NONE', #17870, #148, #23014, .T. ) ;
#31570=AXIS2_PLACEMENT_3D ( 'NONE', #7590, #30267, #13384 ) ;
#31571=AXIS2_PLACEMENT_3D ( 'NONE', #30435, #1554, #35890 ) ;
#31573=DIRECTION ( 'NONE',  ( -1.000000000000000000, 0.000000000000000000, 0.000000000000000000 ) ) ;
#31575=LINE ( 'NONE', #36541, #26659 ) ;
#31576=ORIENTED_EDGE ( 'NONE', *, *, #24885, .F. ) ;
#31578=CIRCLE ( 'NONE', #3436, 2.000000000000000000 ) ;
#31579=CARTESIAN_POINT ( 'NONE',  ( -70.00000337463102085, -34.64101615137762025, 12.50000000000000000 ) ) ;
#31580=CYLINDRICAL_SURFACE ( 'NONE', #831, 2.000000000000000000 ) ;
#31581=EDGE_LOOP ( 'NONE', ( #30572, #11160 ) ) ;
#31582=DIRECTION ( 'NONE',  ( 0.000000000000000000, 0.000000000000000000, 1.000000000000000000 ) ) ;
#31583=AXIS2_PLACEMENT_3D ( 'NONE', #32869, #7187, #795 ) ;
#31584=FACE_OUTER_BOUND ( 'NONE', #8093, .T. ) ;
#31586=DIRECTION ( 'NONE',  ( 1.000000000000000000, 0.000000000000000000, 0.000000000000000000 ) ) ;
#31588=AXIS2_PLACEMENT_3D ( 'NONE', #16520, #5462, #25168 ) ;
#31589=CARTESIAN_POINT ( 'NONE',  ( -35.00000337463117717, -77.94228634059963667, -9.999999999999998224 ) ) ;
#31592=DIRECTION ( 'NONE',  ( -1.000000000000000000, 0.000000000000000000, 0.000000000000000000 ) ) ;
#31593=AXIS2_PLACEMENT_3D ( 'NONE', #20101, #31529, #26097 ) ;
#31594=CARTESIAN_POINT ( 'NONE',  ( 66.99999662536841072, -25.98076211353320275, -9.999999999999998224 ) ) ;
#31595=EDGE_CURVE ( 'NONE', #5465, #5553, #7232, .T. ) ;
#31596=CIRCLE ( 'NONE', #26840, 2.000000000000001776 ) ;
#31597=ORIENTED_EDGE ( 'NONE', *, *, #32722, .F. ) ;
#31599=CARTESIAN_POINT ( 'NONE',  ( -3.374631327851540519E-06, 86.60254037844397601, 17.49999999999999645 ) ) ;
#31600=VERTEX_POINT ( 'NONE', #17539 ) ;
#31601=CIRCLE ( 'NONE', #26822, 2.000000000000000000 ) ;
#31602=ORIENTED_EDGE ( 'NONE', *, *, #20563, .F. ) ;
#31603=ORIENTED_EDGE ( 'NONE', *, *, #20884, .F. ) ;
#31605=DIRECTION ( 'NONE',  ( -1.000000000000000000, 0.000000000000000000, 0.000000000000000000 ) ) ;
#31606=CARTESIAN_POINT ( 'NONE',  ( 42.99999662536848888, -77.94228634059960825, 12.50000000000000000 ) ) ;
#31608=ADVANCED_FACE ( 'NONE', ( #33612 ), #9669, .F. ) ;
#31609=VECTOR ( 'NONE', #8657, 1000.000000000000000 ) ;
#31610=DIRECTION ( 'NONE',  ( -1.000000000000000000, 0.000000000000000000, 0.000000000000000000 ) ) ;
#31611=ORIENTED_EDGE ( 'NONE', *, *, #21359, .T. ) ;
#31613=CYLINDRICAL_SURFACE ( 'NONE', #17936, 2.000000000000000000 ) ;
#31614=VERTEX_POINT ( 'NONE', #24277 ) ;
#31615=AXIS2_PLACEMENT_3D ( 'NONE', #13220, #18847, #10784 ) ;
#31616=AXIS2_PLACEMENT_3D ( 'NONE', #6177, #25514, #36957 ) ;
#31617=FACE_BOUND ( 'NONE', #1182, .T. ) ;
#31618=AXIS2_PLACEMENT_3D ( 'NONE', #13058, #21504, #9867 ) ;
#31619=EDGE_CURVE ( 'NONE', #26391, #13843, #33808, .T. ) ;
#31620=AXIS2_PLACEMENT_3D ( 'NONE', #14452, #34168, #16898 ) ;
#31622=ADVANCED_FACE ( 'NONE', ( #7914 ), #9837, .F. ) ;
#31624=EDGE_CURVE ( 'NONE', #34831, #14526, #251, .T. ) ;
#31625=EDGE_CURVE ( 'NONE', #20160, #36282, #31951, .T. ) ;
#31627=DIRECTION ( 'NONE',  ( 1.000000000000000000, 0.000000000000000000, 0.000000000000000000 ) ) ;
#31628=AXIS2_PLACEMENT_3D ( 'NONE', #31530, #5870, #23100 ) ;
#31629=DIRECTION ( 'NONE',  ( 1.000000000000000000, 0.000000000000000000, 0.000000000000000000 ) ) ;
#31630=CARTESIAN_POINT ( 'NONE',  ( 0.000000000000000000, 0.000000000000000000, -5.000000000000000000 ) ) ;
#31631=VERTEX_POINT ( 'NONE', #21275 ) ;
#31632=DIRECTION ( 'NONE',  ( 0.000000000000000000, 0.000000000000000000, 1.000000000000000000 ) ) ;
#31634=VECTOR ( 'NONE', #48, 1000.000000000000000 ) ;
#31635=CARTESIAN_POINT ( 'NONE',  ( -3.374631334790434423E-06, 69.28203230275516944, -5.000000000000000000 ) ) ;
#31636=ADVANCED_FACE ( 'NONE', ( #1039 ), #7041, .T. ) ;
#31637=EDGE_CURVE ( 'NONE', #30617, #18465, #29577, .T. ) ;
#31638=ORIENTED_EDGE ( 'NONE', *, *, #23180, .T. ) ;
#31639=ORIENTED_EDGE ( 'NONE', *, *, #16543, .F. ) ;
#31640=EDGE_CURVE ( 'NONE', #6520, #30108, #5058, .T. ) ;
#31641=AXIS2_PLACEMENT_3D ( 'NONE', #2621, #30748, #19327 ) ;
#31642=ORIENTED_EDGE ( 'NONE', *, *, #27254, .T. ) ;
#31644=AXIS2_PLACEMENT_3D ( 'NONE', #6098, #34794, #17522 ) ;
#31645=DIRECTION ( 'NONE',  ( 0.000000000000000000, 0.000000000000000000, -1.000000000000000000 ) ) ;
#31646=AXIS2_PLACEMENT_3D ( 'NONE', #34286, #36912, #31106 ) ;
#31647=CARTESIAN_POINT ( 'NONE',  ( -67.00000337463106348, -60.62177826491083010, 17.49999999999999645 ) ) ;
#31649=FACE_OUTER_BOUND ( 'NONE', #2810, .T. ) ;
#31651=EDGE_LOOP ( 'NONE', ( #3260, #31093, #10599, #3664, #8923 ) ) ;
#31652=ORIENTED_EDGE ( 'NONE', *, *, #33725, .F. ) ;
#31653=DIRECTION ( 'NONE',  ( 1.000000000000000000, 0.000000000000000000, 0.000000000000000000 ) ) ;
#31654=EDGE_CURVE ( 'NONE', #11580, #3735, #14623, .T. ) ;
#31655=LINE ( 'NONE', #14586, #19969 ) ;
#31656=EDGE_CURVE ( 'NONE', #4290, #25888, #1435, .T. ) ;
#31657=CARTESIAN_POINT ( 'NONE',  ( 83.47442710120355969, -31.09745072740822991, -5.000000000000011546 ) ) ;
#31658=VERTEX_POINT ( 'NONE', #1401 ) ;
#31659=FACE_BOUND ( 'NONE', #7229, .T. ) ;
#31660=CIRCLE ( 'NONE', #2944, 2.000000000000001776 ) ;
#31661=ORIENTED_EDGE ( 'NONE', *, *, #33769, .T. ) ;
#31662=VERTEX_POINT ( 'NONE', #35729 ) ;
#31663=EDGE_CURVE ( 'NONE', #6793, #3051, #29520, .T. ) ;
#31664=VECTOR ( 'NONE', #4380, 1000.000000000000000 ) ;
#31665=CYLINDRICAL_SURFACE ( 'NONE', #18858, 2.000000000000001776 ) ;
#31666=ORIENTED_EDGE ( 'NONE', *, *, #6085, .T. ) ;
#31667=CARTESIAN_POINT ( 'NONE',  ( -2.000003374631289521, -69.28203230275519786, 17.49999999999999645 ) ) ;
#31669=ORIENTED_EDGE ( 'NONE', *, *, #7511, .F. ) ;
#31670=VERTEX_POINT ( 'NONE', #18276 ) ;
#31671=CIRCLE ( 'NONE', #19732, 2.000000000000001776 ) ;
#31673=ORIENTED_EDGE ( 'NONE', *, *, #25711, .T. ) ;
#31674=EDGE_CURVE ( 'NONE', #22987, #14529, #36776, .T. ) ;
#31675=ORIENTED_EDGE ( 'NONE', *, *, #32065, .F. ) ;
#31676=AXIS2_PLACEMENT_3D ( 'NONE', #34094, #13831, #295 ) ;
#31678=ADVANCED_FACE ( 'NONE', ( #12823 ), #10038, .F. ) ;
#31683=LINE ( 'NONE', #25515, #14519 ) ;
#31684=CARTESIAN_POINT ( 'NONE',  ( 19.99999662536861678, -86.60254037844400443, -5.000000000000000000 ) ) ;
#31685=ORIENTED_EDGE ( 'NONE', *, *, #18105, .T. ) ;
#31686=DIRECTION ( 'NONE',  ( 0.000000000000000000, 0.000000000000000000, 1.000000000000000000 ) ) ;
#31689=DIRECTION ( 'NONE',  ( 0.000000000000000000, 0.000000000000000000, 1.000000000000000000 ) ) ;
#31690=ORIENTED_EDGE ( 'NONE', *, *, #35459, .F. ) ;
#31691=CARTESIAN_POINT ( 'NONE',  ( -35.00000337463116296, -60.62177826491080168, -9.999999999999998224 ) ) ;
#31693=LINE ( 'NONE', #26065, #28551 ) ;
#31694=VERTEX_POINT ( 'NONE', #16735 ) ;
#31695=VERTEX_POINT ( 'NONE', #22526 ) ;
#31698=DIRECTION ( 'NONE',  ( 0.000000000000000000, 0.000000000000000000, -1.000000000000000000 ) ) ;
#31699=CARTESIAN_POINT ( 'NONE',  ( -3.374631334790434423E-06, 69.28203230275516944, -9.999999999999998224 ) ) ;
#31700=ORIENTED_EDGE ( 'NONE', *, *, #17205, .T. ) ;
#31702=EDGE_CURVE ( 'NONE', #9342, #16686, #14012, .T. ) ;
#31706=ORIENTED_EDGE ( 'NONE', *, *, #2624, .T. ) ;
#31707=CARTESIAN_POINT ( 'NONE',  ( -15.00000337463126066, 77.94228634059957983, -5.000000000000000000 ) ) ;
#31708=AXIS2_PLACEMENT_3D ( 'NONE', #30023, #30197, #1515 ) ;
#31710=ORIENTED_EDGE ( 'NONE', *, *, #32082, .T. ) ;
#31711=CARTESIAN_POINT ( 'NONE',  ( -45.00000337463111322, 77.94228634059959404, 12.50000000000000000 ) ) ;
#31713=FACE_OUTER_BOUND ( 'NONE', #518, .T. ) ;
#31714=EDGE_LOOP ( 'NONE', ( #27438, #21428, #2105, #1846, #22567 ) ) ;
#31715=ORIENTED_EDGE ( 'NONE', *, *, #3708, .F. ) ;
#31717=DIRECTION ( 'NONE',  ( 1.000000000000000000, 0.000000000000000000, 0.000000000000000000 ) ) ;
#31718=CARTESIAN_POINT ( 'NONE',  ( -62.00000337463104927, 34.64101615137757051, -5.000000000000000000 ) ) ;
#31720=CARTESIAN_POINT ( 'NONE',  ( -65.00000337463102085, 43.30127018922198801, -9.999999999999998224 ) ) ;
#31721=EDGE_CURVE ( 'NONE', #21374, #10270, #18824, .T. ) ;
#31722=FACE_BOUND ( 'NONE', #37094, .T. ) ;
#31723=CARTESIAN_POINT ( 'NONE',  ( 16.99999662536859901, 77.94228634059957983, -5.000000000000000000 ) ) ;
#31724=DIRECTION ( 'NONE',  ( -0.000000000000000000, -0.000000000000000000, 1.000000000000000000 ) ) ;
#31726=CIRCLE ( 'NONE', #30545, 2.000000000000001776 ) ;
#31728=DIRECTION ( 'NONE',  ( 1.000000000000000000, 0.000000000000000000, 0.000000000000000000 ) ) ;
#31729=CIRCLE ( 'NONE', #2401, 2.000000000000000000 ) ;
#31730=DIRECTION ( 'NONE',  ( 1.000000000000000000, 0.000000000000000000, 0.000000000000000000 ) ) ;
#31731=VERTEX_POINT ( 'NONE', #33784 ) ;
#31732=DIRECTION ( 'NONE',  ( 1.000000000000000000, 0.000000000000000000, 0.000000000000000000 ) ) ;
#31735=CYLINDRICAL_SURFACE ( 'NONE', #14545, 2.000000000000001776 ) ;
#31736=EDGE_LOOP ( 'NONE', ( #5006, #22458 ) ) ;
#31737=EDGE_LOOP ( 'NONE', ( #8122, #20098, #12216, #10913 ) ) ;
#31738=EDGE_LOOP ( 'NONE', ( #24995, #36582, #26924, #17491 ) ) ;
#31740=DIRECTION ( 'NONE',  ( 0.000000000000000000, 0.000000000000000000, -1.000000000000000000 ) ) ;
#31743=ORIENTED_EDGE ( 'NONE', *, *, #13111, .F. ) ;
#31745=DIRECTION ( 'NONE',  ( 0.000000000000000000, 0.000000000000000000, 1.000000000000000000 ) ) ;
#31747=VECTOR ( 'NONE', #622, 1000.000000000000000 ) ;
#31749=EDGE_CURVE ( 'NONE', #2553, #35136, #24847, .T. ) ;
#31751=DIRECTION ( 'NONE',  ( 0.000000000000000000, 0.000000000000000000, -1.000000000000000000 ) ) ;
#31752=EDGE_LOOP ( 'NONE', ( #28486, #1131 ) ) ;
#31754=EDGE_CURVE ( 'NONE', #24605, #15127, #8086, .T. ) ;
#31755=CARTESIAN_POINT ( 'NONE',  ( -44.13139720814380951, 27.50000000000055422, -5.000000000000000000 ) ) ;
#31757=LINE ( 'NONE', #20685, #20073 ) ;
#31759=ORIENTED_EDGE ( 'NONE', *, *, #22294, .T. ) ;
#31761=CYLINDRICAL_SURFACE ( 'NONE', #9310, 33.00000000000001421 ) ;
#31762=DIRECTION ( 'NONE',  ( 1.000000000000000000, 0.000000000000000000, 0.000000000000000000 ) ) ;
#31763=ORIENTED_EDGE ( 'NONE', *, *, #36622, .T. ) ;
#31764=DIRECTION ( 'NONE',  ( 1.000000000000000000, 0.000000000000000000, 0.000000000000000000 ) ) ;
#31767=EDGE_CURVE ( 'NONE', #13910, #6635, #17649, .T. ) ;
#31768=CARTESIAN_POINT ( 'NONE',  ( -3.374631303565411855E-06, -86.60254037844400443, -5.000000000000000000 ) ) ;
#31769=CARTESIAN_POINT ( 'NONE',  ( -82.00000337463096400, -34.64101615137762025, -9.999999999999998224 ) ) ;
#31770=DIRECTION ( 'NONE',  ( 0.000000000000000000, 0.000000000000000000, 1.000000000000000000 ) ) ;
#31772=DIRECTION ( 'NONE',  ( 0.000000000000000000, 0.000000000000000000, 1.000000000000000000 ) ) ;
#31773=ORIENTED_EDGE ( 'NONE', *, *, #22406, .T. ) ;
#31775=CARTESIAN_POINT ( 'NONE',  ( -35.19434990244938888, 52.39915983220783602, 12.49999999999999822 ) ) ;
#31776=ORIENTED_EDGE ( 'NONE', *, *, #19544, .F. ) ;
#31777=ADVANCED_FACE ( 'NONE', ( #13899 ), #33983, .F. ) ;
#31778=VERTEX_POINT ( 'NONE', #8296 ) ;
#31779=ORIENTED_EDGE ( 'NONE', *, *, #36350, .T. ) ;
#31780=ADVANCED_FACE ( 'NONE', ( #31159 ), #5476, .F. ) ;
#31783=DIRECTION ( 'NONE',  ( 0.000000000000000000, 0.000000000000000000, 1.000000000000000000 ) ) ;
#31785=CYLINDRICAL_SURFACE ( 'NONE', #24875, 2.000000000000000000 ) ;
#31786=EDGE_LOOP ( 'NONE', ( #9940, #22171 ) ) ;
#31787=DIRECTION ( 'NONE',  ( 1.000000000000000000, 0.000000000000000000, 0.000000000000000000 ) ) ;
#31789=ORIENTED_EDGE ( 'NONE', *, *, #13699, .F. ) ;
#31790=FACE_BOUND ( 'NONE', #28148, .T. ) ;
#31791=EDGE_CURVE ( 'NONE', #35055, #22308, #2079, .T. ) ;
#31792=DIRECTION ( 'NONE',  ( 1.000000000000000000, 0.000000000000000000, 0.000000000000000000 ) ) ;
#31793=CARTESIAN_POINT ( 'NONE',  ( 79.99999662536833966, 34.64101615137759183, -9.999999999999998224 ) ) ;
#31794=CARTESIAN_POINT ( 'NONE',  ( 79.99999662536833966, -3.469446951953614189E-15, -5.000000000000000000 ) ) ;
#31796=DIRECTION ( 'NONE',  ( 1.000000000000000000, 0.000000000000000000, 0.000000000000000000 ) ) ;
#31798=CARTESIAN_POINT ( 'NONE',  ( 22.99999662536857059, 77.94228634059957983, -5.000000000000000000 ) ) ;
#31799=ORIENTED_EDGE ( 'NONE', *, *, #25511, .T. ) ;
#31802=CARTESIAN_POINT ( 'NONE',  ( -47.00000337463111322, 77.94228634059959404, -9.999999999999998224 ) ) ;
#31803=ORIENTED_EDGE ( 'NONE', *, *, #5333, .F. ) ;
#31804=EDGE_CURVE ( 'NONE', #4245, #12365, #22728, .T. ) ;
#31807=CARTESIAN_POINT ( 'NONE',  ( 6.999996625368645198, 77.94228634059957983, 17.49999999999999645 ) ) ;
#31808=EDGE_CURVE ( 'NONE', #1539, #21899, #12857, .T. ) ;
#31809=DIRECTION ( 'NONE',  ( 0.000000000000000000, 0.000000000000000000, 1.000000000000000000 ) ) ;
#31810=CIRCLE ( 'NONE', #20449, 2.000000000000000000 ) ;
#31812=DIRECTION ( 'NONE',  ( 0.000000000000000000, 0.000000000000000000, 1.000000000000000000 ) ) ;
#31813=CARTESIAN_POINT ( 'NONE',  ( 0.000000000000000000, 0.000000000000000000, -5.000000000000000000 ) ) ;
#31814=CIRCLE ( 'NONE', #30635, 2.000000000000000000 ) ;
#31816=FACE_OUTER_BOUND ( 'NONE', #10880, .T. ) ;
#31817=VERTEX_POINT ( 'NONE', #14626 ) ;
#31819=LINE ( 'NONE', #32203, #896 ) ;
#31820=CARTESIAN_POINT ( 'NONE',  ( 74.99999662536836809, 43.30127018922198801, -9.999999999999998224 ) ) ;
#31821=CARTESIAN_POINT ( 'NONE',  ( 47.99999662536846756, 69.28203230275516944, 17.49999999999999645 ) ) ;
#31823=ADVANCED_FACE ( 'NONE', ( #23072 ), #34521, .F. ) ;
#31824=FACE_BOUND ( 'NONE', #13776, .T. ) ;
#31825=ORIENTED_EDGE ( 'NONE', *, *, #7937, .T. ) ;
#31826=ORIENTED_EDGE ( 'NONE', *, *, #12058, .T. ) ;
#31827=DIRECTION ( 'NONE',  ( 0.4999999999999919509, -0.8660254037844433705, 0.000000000000000000 ) ) ;
#31828=VERTEX_POINT ( 'NONE', #21007 ) ;
#31829=DIRECTION ( 'NONE',  ( 0.000000000000000000, 0.000000000000000000, -1.000000000000000000 ) ) ;
#31830=AXIS2_PLACEMENT_3D ( 'NONE', #30627, #4944, #5131 ) ;
#31831=CYLINDRICAL_SURFACE ( 'NONE', #4144, 2.000000000000001776 ) ;
#31832=ORIENTED_EDGE ( 'NONE', *, *, #35981, .F. ) ;
#31834=ORIENTED_EDGE ( 'NONE', *, *, #2395, .F. ) ;
#31835=ORIENTED_EDGE ( 'NONE', *, *, #4941, .F. ) ;
#31836=EDGE_CURVE ( 'NONE', #23515, #19493, #22421, .T. ) ;
#31837=ORIENTED_EDGE ( 'NONE', *, *, #28005, .F. ) ;
#31838=DIRECTION ( 'NONE',  ( 1.000000000000000000, 0.000000000000000000, 0.000000000000000000 ) ) ;
#31840=EDGE_CURVE ( 'NONE', #20325, #33375, #12220, .T. ) ;
#31841=DIRECTION ( 'NONE',  ( 0.000000000000000000, 0.000000000000000000, 1.000000000000000000 ) ) ;
#31843=DIRECTION ( 'NONE',  ( 1.000000000000000000, 0.000000000000000000, 0.000000000000000000 ) ) ;
#31844=ORIENTED_EDGE ( 'NONE', *, *, #19076, .F. ) ;
#31845=DIRECTION ( 'NONE',  ( 1.000000000000000000, 0.000000000000000000, 0.000000000000000000 ) ) ;
#31846=EDGE_CURVE ( 'NONE', #5584, #11561, #14652, .T. ) ;
#31847=CIRCLE ( 'NONE', #15714, 2.000000000000001776 ) ;
#31848=VECTOR ( 'NONE', #2852, 1000.000000000000000 ) ;
#31849=DIRECTION ( 'NONE',  ( 1.000000000000000000, 0.000000000000000000, 0.000000000000000000 ) ) ;
#31852=CARTESIAN_POINT ( 'NONE',  ( 0.000000000000000000, 0.000000000000000000, 12.49999999999999822 ) ) ;
#31854=FACE_OUTER_BOUND ( 'NONE', #9832, .T. ) ;
#31856=ORIENTED_EDGE ( 'NONE', *, *, #29821, .F. ) ;
#31857=ORIENTED_EDGE ( 'NONE', *, *, #30075, .T. ) ;
#31859=CIRCLE ( 'NONE', #26501, 2.000000000000001776 ) ;
#31860=DIRECTION ( 'NONE',  ( 0.000000000000000000, 0.000000000000000000, 1.000000000000000000 ) ) ;
#31861=DIRECTION ( 'NONE',  ( -1.000000000000000000, 0.000000000000000000, 0.000000000000000000 ) ) ;
#31862=CYLINDRICAL_SURFACE ( 'NONE', #26253, 2.000000000000000000 ) ;
#31864=EDGE_CURVE ( 'NONE', #31828, #36323, #33207, .T. ) ;
#31865=CYLINDRICAL_SURFACE ( 'NONE', #13515, 2.000000000000001776 ) ;
#31868=CARTESIAN_POINT ( 'NONE',  ( -89.42901512340354486, 31.83425564451495404, -4.999999999999997335 ) ) ;
#31869=EDGE_CURVE ( 'NONE', #28166, #25343, #18384, .T. ) ;
#31870=ORIENTED_EDGE ( 'NONE', *, *, #21967, .F. ) ;
#31871=EDGE_CURVE ( 'NONE', #19642, #7368, #26823, .T. ) ;
#31872=DIRECTION ( 'NONE',  ( 1.000000000000000000, 0.000000000000000000, 0.000000000000000000 ) ) ;
#31873=ORIENTED_EDGE ( 'NONE', *, *, #26474, .F. ) ;
#31874=DIRECTION ( 'NONE',  ( 0.000000000000000000, 0.000000000000000000, -1.000000000000000000 ) ) ;
#31875=CIRCLE ( 'NONE', #23529, 2.000000000000001776 ) ;
#31876=DIRECTION ( 'NONE',  ( 0.000000000000000000, 0.000000000000000000, 1.000000000000000000 ) ) ;
#31878=ORIENTED_EDGE ( 'NONE', *, *, #22485, .T. ) ;
#31880=DIRECTION ( 'NONE',  ( -1.000000000000000000, 0.000000000000000000, 0.000000000000000000 ) ) ;
#31881=CARTESIAN_POINT ( 'NONE',  ( 29.97040607558719572, -71.28181339061548272, -5.000000000000000000 ) ) ;
#31882=CARTESIAN_POINT ( 'NONE',  ( 54.99999662536844625, 43.30127018922198801, -9.999999999999998224 ) ) ;
#31885=AXIS2_PLACEMENT_3D ( 'NONE', #28272, #30714, #5034 ) ;
#31886=FACE_BOUND ( 'NONE', #10013, .T. ) ;
#31887=AXIS2_PLACEMENT_3D ( 'NONE', #27814, #16034, #21653 ) ;
#31889=DIRECTION ( 'NONE',  ( -1.000000000000000000, 0.000000000000000000, 0.000000000000000000 ) ) ;
#31890=DIRECTION ( 'NONE',  ( 0.000000000000000000, 0.000000000000000000, -1.000000000000000000 ) ) ;
#31891=FACE_OUTER_BOUND ( 'NONE', #13866, .T. ) ;
#31892=DIRECTION ( 'NONE',  ( 1.000000000000000000, 0.000000000000000000, 0.000000000000000000 ) ) ;
#31894=EDGE_LOOP ( 'NONE', ( #19707, #28892 ) ) ;
#31897=CIRCLE ( 'NONE', #6783, 1.999999999999998224 ) ;
#31899=ORIENTED_EDGE ( 'NONE', *, *, #19030, .T. ) ;
#31900=CIRCLE ( 'NONE', #15766, 2.000000000000001776 ) ;
#31903=CARTESIAN_POINT ( 'NONE',  ( 59.99999662536845335, 34.64101615137759893, 17.49999999999999645 ) ) ;
#31904=CARTESIAN_POINT ( 'NONE',  ( 67.99999662536836809, -51.96152422706639840, -5.000000000000000000 ) ) ;
#31905=CARTESIAN_POINT ( 'NONE',  ( -28.00000337463119493, -69.28203230275522628, 12.50000000000000000 ) ) ;
#31906=EDGE_LOOP ( 'NONE', ( #17868, #20309, #9922, #35893 ) ) ;
#31907=VERTEX_POINT ( 'NONE', #29255 ) ;
#31909=AXIS2_PLACEMENT_3D ( 'NONE', #36087, #18838, #27459 ) ;
#31910=VERTEX_POINT ( 'NONE', #3937 ) ;
#31912=CARTESIAN_POINT ( 'NONE',  ( 89.67878100130370456, -27.78182860042797131, 12.49999999999999822 ) ) ;
#31913=ORIENTED_EDGE ( 'NONE', *, *, #21980, .T. ) ;
#31914=DIRECTION ( 'NONE',  ( 1.000000000000000000, 0.000000000000000000, 0.000000000000000000 ) ) ;
#31915=EDGE_LOOP ( 'NONE', ( #22770, #5657 ) ) ;
#31917=DIRECTION ( 'NONE',  ( 1.000000000000000000, 0.000000000000000000, 0.000000000000000000 ) ) ;
#31918=FACE_BOUND ( 'NONE', #8377, .T. ) ;
#31919=CYLINDRICAL_SURFACE ( 'NONE', #9284, 3.000000000000002665 ) ;
#31920=ORIENTED_EDGE ( 'NONE', *, *, #6602, .F. ) ;
#31921=CARTESIAN_POINT ( 'NONE',  ( 86.99999662536831124, -25.98076211353319565, 12.50000000000000000 ) ) ;
#31923=CARTESIAN_POINT ( 'NONE',  ( 60.93295298011005201, 19.13981058454729123, 12.49999999999999822 ) ) ;
#31924=DIRECTION ( 'NONE',  ( -0.000000000000000000, 0.000000000000000000, -1.000000000000000000 ) ) ;
#31925=CIRCLE ( 'NONE', #16409, 2.000000000000001776 ) ;
#31927=CYLINDRICAL_SURFACE ( 'NONE', #27896, 2.000000000000001776 ) ;
#31928=CYLINDRICAL_SURFACE ( 'NONE', #18576, 2.000000000000001776 ) ;
#31929=ORIENTED_EDGE ( 'NONE', *, *, #35404, .T. ) ;
#31931=CYLINDRICAL_SURFACE ( 'NONE', #5918, 2.000000000000001776 ) ;
#31934=EDGE_CURVE ( 'NONE', #14326, #10243, #35282, .T. ) ;
#31936=AXIS2_PLACEMENT_3D ( 'NONE', #35398, #9505, #12481 ) ;
#31937=DIRECTION ( 'NONE',  ( 0.000000000000000000, 0.000000000000000000, 1.000000000000000000 ) ) ;
#31938=CIRCLE ( 'NONE', #23584, 2.000000000000001776 ) ;
#31939=CARTESIAN_POINT ( 'NONE',  ( 52.99999662536844625, -60.62177826491080168, -9.999999999999998224 ) ) ;
#31940=ORIENTED_EDGE ( 'NONE', *, *, #27768, .F. ) ;
#31942=CARTESIAN_POINT ( 'NONE',  ( -15.00000337463126066, 77.94228634059957983, 12.50000000000000000 ) ) ;
#31943=DIRECTION ( 'NONE',  ( 0.000000000000000000, 0.000000000000000000, 1.000000000000000000 ) ) ;
#31945=EDGE_CURVE ( 'NONE', #21999, #33006, #27822, .T. ) ;
#31946=ORIENTED_EDGE ( 'NONE', *, *, #29334, .T. ) ;
#31947=ORIENTED_EDGE ( 'NONE', *, *, #36128, .T. ) ;
#31949=DIRECTION ( 'NONE',  ( -0.000000000000000000, -0.000000000000000000, 1.000000000000000000 ) ) ;
#31950=DIRECTION ( 'NONE',  ( 0.000000000000000000, 0.000000000000000000, -1.000000000000000000 ) ) ;
#31951=CIRCLE ( 'NONE', #21212, 2.000000000000001776 ) ;
#31952=CARTESIAN_POINT ( 'NONE',  ( -61.06482292022059966, 72.77422209630346117, 12.49999999999999822 ) ) ;
#31953=EDGE_LOOP ( 'NONE', ( #35509, #11878 ) ) ;
#31955=CARTESIAN_POINT ( 'NONE',  ( -22.00000337463124112, -86.60254037844400443, -5.000000000000000000 ) ) ;
#31956=ORIENTED_EDGE ( 'NONE', *, *, #6005, .F. ) ;
#31957=FACE_BOUND ( 'NONE', #18817, .T. ) ;
#31959=LINE ( 'NONE', #35940, #556 ) ;
#31960=CIRCLE ( 'NONE', #21224, 2.000000000000001776 ) ;
#31966=DIRECTION ( 'NONE',  ( 1.000000000000000000, 0.000000000000000000, 0.000000000000000000 ) ) ;
#31968=ADVANCED_FACE ( 'NONE', ( #29434 ), #3753, .F. ) ;
#31969=EDGE_LOOP ( 'NONE', ( #1365, #29739 ) ) ;
#31970=CARTESIAN_POINT ( 'NONE',  ( 44.99999662536851019, 77.94228634059959404, -9.999999999999998224 ) ) ;
#31971=AXIS2_PLACEMENT_3D ( 'NONE', #12712, #21360, #27356 ) ;
#31972=CARTESIAN_POINT ( 'NONE',  ( 36.99999662536855283, 60.62177826491078747, -9.999999999999998224 ) ) ;
#31973=CARTESIAN_POINT ( 'NONE',  ( 54.99999662536846046, -43.30127018922200222, -9.999999999999998224 ) ) ;
#31975=ORIENTED_EDGE ( 'NONE', *, *, #18408, .F. ) ;
#31976=AXIS2_PLACEMENT_3D ( 'NONE', #15189, #24015, #26622 ) ;
#31977=ORIENTED_EDGE ( 'NONE', *, *, #14238, .F. ) ;
#31979=EDGE_CURVE ( 'NONE', #10472, #17978, #11042, .T. ) ;
#31980=DIRECTION ( 'NONE',  ( 1.000000000000000000, 0.000000000000000000, 0.000000000000000000 ) ) ;
#31982=AXIS2_PLACEMENT_3D ( 'NONE', #12890, #21709, #2208 ) ;
#31983=CARTESIAN_POINT ( 'NONE',  ( 71.99999662536838230, -51.96152422706639840, -5.000000000000000000 ) ) ;
#31984=EDGE_CURVE ( 'NONE', #7436, #7675, #7464, .T. ) ;
#31985=AXIS2_PLACEMENT_3D ( 'NONE', #10416, #30492, #4817 ) ;
#31986=CARTESIAN_POINT ( 'NONE',  ( -10.00000337463128730, 69.28203230275516944, 12.50000000000000000 ) ) ;
#31988=CARTESIAN_POINT ( 'NONE',  ( -72.00000337463100664, -2.404119930384582903E-14, -5.000000000000000000 ) ) ;
#31992=DIRECTION ( 'NONE',  ( 0.000000000000000000, 0.000000000000000000, 1.000000000000000000 ) ) ;
#31993=AXIS2_PLACEMENT_3D ( 'NONE', #23259, #11987, #9009 ) ;
#31995=VECTOR ( 'NONE', #1943, 1000.000000000000000 ) ;
#31996=CARTESIAN_POINT ( 'NONE',  ( 62.97617850287784336, 4.279621169095339184, -49.86561046011506448 ) ) ;
#31998=VECTOR ( 'NONE', #17238, 1000.000000000000000 ) ;
#31999=EDGE_CURVE ( 'NONE', #14157, #27148, #33001, .T. ) ;
#32000=FACE_BOUND ( 'NONE', #19996, .T. ) ;
#32001=ORIENTED_EDGE ( 'NONE', *, *, #7736, .F. ) ;
#32002=ORIENTED_EDGE ( 'NONE', *, *, #27653, .T. ) ;
#32006=AXIS2_PLACEMENT_3D ( 'NONE', #30103, #1808, #4429 ) ;
#32008=CIRCLE ( 'NONE', #15881, 27.00000000000001421 ) ;
#32009=CARTESIAN_POINT ( 'NONE',  ( 64.99999662536839651, -43.30127018922199511, -5.000000000000000000 ) ) ;
#32011=DIRECTION ( 'NONE',  ( 1.000000000000000000, 0.000000000000000000, 0.000000000000000000 ) ) ;
#32012=EDGE_CURVE ( 'NONE', #21341, #29683, #17040, .T. ) ;
#32014=ORIENTED_EDGE ( 'NONE', *, *, #14301, .T. ) ;
#32015=EDGE_LOOP ( 'NONE', ( #23844, #9355 ) ) ;
#32016=ORIENTED_EDGE ( 'NONE', *, *, #35454, .F. ) ;
#32017=VERTEX_POINT ( 'NONE', #15750 ) ;
#32018=AXIS2_PLACEMENT_3D ( 'NONE', #13369, #12806, #16382 ) ;
#32019=DIRECTION ( 'NONE',  ( 1.000000000000000000, 0.000000000000000000, 0.000000000000000000 ) ) ;
#32020=CARTESIAN_POINT ( 'NONE',  ( 51.99999662536847467, 69.28203230275516944, -9.999999999999998224 ) ) ;
#32021=ORIENTED_EDGE ( 'NONE', *, *, #7849, .T. ) ;
#32022=CIRCLE ( 'NONE', #12881, 95.00000000000000000 ) ;
#32025=LINE ( 'NONE', #20431, #23143 ) ;
#32028=AXIS2_PLACEMENT_3D ( 'NONE', #17542, #19995, #5749 ) ;
#32029=CYLINDRICAL_SURFACE ( 'NONE', #24233, 1.999999999999998224 ) ;
#32030=CARTESIAN_POINT ( 'NONE',  ( 71.99999662536841072, 51.96152422706640550, 17.49999999999999645 ) ) ;
#32031=ADVANCED_FACE ( 'NONE', ( #4502 ), #15940, .F. ) ;
#32034=DIRECTION ( 'NONE',  ( 0.000000000000000000, 0.000000000000000000, 1.000000000000000000 ) ) ;
#32036=AXIS2_PLACEMENT_3D ( 'NONE', #20942, #24122, #6687 ) ;
#32037=ORIENTED_EDGE ( 'NONE', *, *, #24793, .T. ) ;
#32038=CIRCLE ( 'NONE', #9904, 2.000000000000001776 ) ;
#32039=ORIENTED_EDGE ( 'NONE', *, *, #18401, .F. ) ;
#32041=DIRECTION ( 'NONE',  ( 1.000000000000000000, 0.000000000000000000, 0.000000000000000000 ) ) ;
#32042=CARTESIAN_POINT ( 'NONE',  ( -52.39915983220772233, -35.19434990244957362, 12.49999999999999822 ) ) ;
#32043=DIRECTION ( 'NONE',  ( 1.000000000000000000, 0.000000000000000000, 0.000000000000000000 ) ) ;
#32045=CARTESIAN_POINT ( 'NONE',  ( 67.99999662536838230, -3.224517592124143893E-15, 17.49999999999999645 ) ) ;
#32048=EDGE_CURVE ( 'NONE', #23693, #32859, #15245, .T. ) ;
#32050=ORIENTED_EDGE ( 'NONE', *, *, #2954, .T. ) ;
#32051=EDGE_CURVE ( 'NONE', #12512, #31658, #282, .T. ) ;
#32052=AXIS2_PLACEMENT_3D ( 'NONE', #13514, #33775, #33602 ) ;
#32054=ORIENTED_EDGE ( 'NONE', *, *, #33699, .F. ) ;
#32056=CIRCLE ( 'NONE', #33295, 2.000000000000001776 ) ;
#32057=AXIS2_PLACEMENT_3D ( 'NONE', #27650, #10235, #21662 ) ;
#32058=LINE ( 'NONE', #21196, #1333 ) ;
#32059=EDGE_CURVE ( 'NONE', #20361, #9651, #26031, .T. ) ;
#32060=VECTOR ( 'NONE', #7779, 1000.000000000000000 ) ;
#32061=DIRECTION ( 'NONE',  ( 0.000000000000000000, 0.000000000000000000, 1.000000000000000000 ) ) ;
#32062=FACE_OUTER_BOUND ( 'NONE', #8251, .T. ) ;
#32064=ORIENTED_EDGE ( 'NONE', *, *, #10096, .T. ) ;
#32065=EDGE_CURVE ( 'NONE', #34930, #9326, #12925, .T. ) ;
#32066=AXIS2_PLACEMENT_3D ( 'NONE', #24879, #33870, #36319 ) ;
#32068=EDGE_CURVE ( 'NONE', #4038, #5699, #36015, .T. ) ;
#32070=VECTOR ( 'NONE', #31512, 1000.000000000000000 ) ;
#32072=ORIENTED_EDGE ( 'NONE', *, *, #25934, .F. ) ;
#32074=FACE_BOUND ( 'NONE', #20384, .T. ) ;
#32075=DIRECTION ( 'NONE',  ( 1.000000000000000000, 0.000000000000000000, 0.000000000000000000 ) ) ;
#32077=DIRECTION ( 'NONE',  ( 1.000000000000000000, 0.000000000000000000, 0.000000000000000000 ) ) ;
#32078=EDGE_CURVE ( 'NONE', #18782, #32494, #25426, .T. ) ;
#32081=CIRCLE ( 'NONE', #36293, 2.000000000000000000 ) ;
#32082=EDGE_CURVE ( 'NONE', #17074, #6836, #6306, .T. ) ;
#32084=AXIS2_PLACEMENT_3D ( 'NONE', #5287, #31489, #36960 ) ;
#32088=DIRECTION ( 'NONE',  ( -1.000000000000000000, 0.000000000000000000, 0.000000000000000000 ) ) ;
#32090=FACE_BOUND ( 'NONE', #2010, .T. ) ;
#32091=LINE ( 'NONE', #29297, #10203 ) ;
#32092=CIRCLE ( 'NONE', #3982, 2.000000000000001776 ) ;
#32094=EDGE_LOOP ( 'NONE', ( #27931, #37104 ) ) ;
#32095=AXIS2_PLACEMENT_3D ( 'NONE', #24093, #35539, #33265 ) ;
#32096=ORIENTED_EDGE ( 'NONE', *, *, #33790, .F. ) ;
#32097=AXIS2_PLACEMENT_3D ( 'NONE', #28267, #33723, #18915 ) ;
#32099=DIRECTION ( 'NONE',  ( 1.000000000000000000, 0.000000000000000000, 0.000000000000000000 ) ) ;
#32100=CYLINDRICAL_SURFACE ( 'NONE', #13987, 2.000000000000001776 ) ;
#32101=DIRECTION ( 'NONE',  ( 0.000000000000000000, 0.000000000000000000, -1.000000000000000000 ) ) ;
#32102=VERTEX_POINT ( 'NONE', #1491 ) ;
#32104=ORIENTED_EDGE ( 'NONE', *, *, #6917, .T. ) ;
#32105=CYLINDRICAL_SURFACE ( 'NONE', #35293, 2.000000000000001776 ) ;
#32106=ORIENTED_EDGE ( 'NONE', *, *, #30860, .T. ) ;
#32108=ORIENTED_EDGE ( 'NONE', *, *, #30212, .T. ) ;
#32109=DIRECTION ( 'NONE',  ( -0.5000000000000101030, -0.8660254037844329345, 0.000000000000000000 ) ) ;
#32110=ORIENTED_EDGE ( 'NONE', *, *, #19516, .F. ) ;
#32111=AXIS2_PLACEMENT_3D ( 'NONE', #6218, #29282, #17478 ) ;
#32112=VERTEX_POINT ( 'NONE', #21933 ) ;
#32115=AXIS2_PLACEMENT_3D ( 'NONE', #9565, #20258, #29038 ) ;
#32116=CYLINDRICAL_SURFACE ( 'NONE', #33844, 3.499999999999989342 ) ;
#32117=ORIENTED_EDGE ( 'NONE', *, *, #30332, .T. ) ;
#32118=VERTEX_POINT ( 'NONE', #35833 ) ;
#32121=CIRCLE ( 'NONE', #33945, 2.000000000000000000 ) ;
#32122=VECTOR ( 'NONE', #25424, 1000.000000000000000 ) ;
#32123=VECTOR ( 'NONE', #18985, 1000.000000000000000 ) ;
#32124=CARTESIAN_POINT ( 'NONE',  ( 82.99999662536832545, 8.660254037844394404, -9.999999999999998224 ) ) ;
#32126=AXIS2_PLACEMENT_3D ( 'NONE', #26752, #15874, #20951 ) ;
#32127=EDGE_LOOP ( 'NONE', ( #12337, #3382, #22321, #18593 ) ) ;
#32128=CYLINDRICAL_SURFACE ( 'NONE', #22524, 2.000000000000001776 ) ;
#32129=DIRECTION ( 'NONE',  ( -0.000000000000000000, -0.000000000000000000, -1.000000000000000000 ) ) ;
#32132=DIRECTION ( 'NONE',  ( 1.000000000000000000, 0.000000000000000000, 0.000000000000000000 ) ) ;
#32133=DIRECTION ( 'NONE',  ( 0.000000000000000000, 0.000000000000000000, 1.000000000000000000 ) ) ;
#32136=AXIS2_PLACEMENT_3D ( 'NONE', #20089, #9028, #31872 ) ;
#32137=EDGE_CURVE ( 'NONE', #6269, #30055, #23062, .T. ) ;
#32140=ADVANCED_FACE ( 'NONE', ( #30913 ), #19857, .F. ) ;
#32142=VERTEX_POINT ( 'NONE', #5988 ) ;
#32143=CARTESIAN_POINT ( 'NONE',  ( 42.99999662536850309, -60.62177826491080168, -9.999999999999998224 ) ) ;
#32147=VECTOR ( 'NONE', #36955, 1000.000000000000000 ) ;
#32148=ORIENTED_EDGE ( 'NONE', *, *, #17644, .T. ) ;
#32150=ORIENTED_EDGE ( 'NONE', *, *, #22464, .F. ) ;
#32152=FACE_OUTER_BOUND ( 'NONE', #4818, .T. ) ;
#32154=DIRECTION ( 'NONE',  ( 0.000000000000000000, 0.000000000000000000, 1.000000000000000000 ) ) ;
#32155=CIRCLE ( 'NONE', #12998, 2.000000000000001776 ) ;
#32157=DIRECTION ( 'NONE',  ( 1.000000000000000000, 0.000000000000000000, 0.000000000000000000 ) ) ;
#32159=VERTEX_POINT ( 'NONE', #28466 ) ;
#32160=CARTESIAN_POINT ( 'NONE',  ( -63.00000337463104927, -25.98076211353322051, -9.999999999999998224 ) ) ;
#32161=ORIENTED_EDGE ( 'NONE', *, *, #18319, .F. ) ;
#32162=FACE_BOUND ( 'NONE', #7144, .T. ) ;
#32164=EDGE_CURVE ( 'NONE', #36526, #859, #34127, .T. ) ;
#32165=AXIS2_PLACEMENT_3D ( 'NONE', #29829, #4154, #24595 ) ;
#32166=LINE ( 'NONE', #6297, #5372 ) ;
#32168=CYLINDRICAL_SURFACE ( 'NONE', #31065, 2.000000000000001776 ) ;
#32169=ORIENTED_EDGE ( 'NONE', *, *, #16466, .F. ) ;
#32171=AXIS2_PLACEMENT_3D ( 'NONE', #10571, #14109, #22011 ) ;
#32173=CIRCLE ( 'NONE', #30983, 2.000000000000001776 ) ;
#32174=DIRECTION ( 'NONE',  ( 0.000000000000000000, 0.000000000000000000, 1.000000000000000000 ) ) ;
#32176=CARTESIAN_POINT ( 'NONE',  ( 65.00000000000000000, 0.000000000000000000, 12.49999999999999822 ) ) ;
#32177=DIRECTION ( 'NONE',  ( 0.000000000000000000, 0.000000000000000000, -1.000000000000000000 ) ) ;
#32178=ORIENTED_EDGE ( 'NONE', *, *, #3221, .T. ) ;
#32179=CARTESIAN_POINT ( 'NONE',  ( -88.00000337463090716, -1.040834085586084257E-14, 17.49999999999999645 ) ) ;
#32180=DIRECTION ( 'NONE',  ( -1.000000000000000000, 0.000000000000000000, 0.000000000000000000 ) ) ;
#32181=DIRECTION ( 'NONE',  ( 0.000000000000000000, 0.000000000000000000, 1.000000000000000000 ) ) ;
#32184=AXIS2_PLACEMENT_3D ( 'NONE', #31033, #5713, #25235 ) ;
#32186=EDGE_CURVE ( 'NONE', #23515, #19701, #27378, .T. ) ;
#32187=EDGE_LOOP ( 'NONE', ( #14724, #7336, #33048, #26029, #14084, #2308, #18918, #1291, #3546, #19275 ) ) ;
#32188=DIRECTION ( 'NONE',  ( 0.000000000000000000, 0.000000000000000000, 1.000000000000000000 ) ) ;
#32189=CIRCLE ( 'NONE', #30413, 2.000000000000001776 ) ;
#32190=FACE_OUTER_BOUND ( 'NONE', #19942, .T. ) ;
#32191=DIRECTION ( 'NONE',  ( 1.000000000000000000, 0.000000000000000000, 0.000000000000000000 ) ) ;
#32193=AXIS2_PLACEMENT_3D ( 'NONE', #26642, #20632, #18026 ) ;
#32194=CARTESIAN_POINT ( 'NONE',  ( 16.99999662536859901, 77.94228634059957983, -9.999999999999998224 ) ) ;
#32195=DIRECTION ( 'NONE',  ( 0.000000000000000000, 0.000000000000000000, 1.000000000000000000 ) ) ;
#32196=CIRCLE ( 'NONE', #33400, 3.499999999999991562 ) ;
#32197=AXIS2_PLACEMENT_3D ( 'NONE', #32641, #6966, #18417 ) ;
#32199=DIRECTION ( 'NONE',  ( 0.000000000000000000, 0.000000000000000000, 1.000000000000000000 ) ) ;
#32200=ORIENTED_EDGE ( 'NONE', *, *, #35718, .F. ) ;
#32201=CIRCLE ( 'NONE', #7064, 1.999999999999998224 ) ;
#32203=CARTESIAN_POINT ( 'NONE',  ( -68.00000337463102085, -34.64101615137762025, -9.999999999999998224 ) ) ;
#32204=AXIS2_PLACEMENT_3D ( 'NONE', #34514, #33779, #8090 ) ;
#32205=EDGE_CURVE ( 'NONE', #29268, #33506, #10487, .T. ) ;
#32206=DIRECTION ( 'NONE',  ( 0.000000000000000000, 0.000000000000000000, 1.000000000000000000 ) ) ;
#32207=ORIENTED_EDGE ( 'NONE', *, *, #29228, .F. ) ;
#32208=DIRECTION ( 'NONE',  ( -1.000000000000000000, 1.490577208987477824E-14, 0.000000000000000000 ) ) ;
#32209=ORIENTED_EDGE ( 'NONE', *, *, #26741, .F. ) ;
#32212=FACE_BOUND ( 'NONE', #34961, .T. ) ;
#32213=VERTEX_POINT ( 'NONE', #31112 ) ;
#32214=EDGE_LOOP ( 'NONE', ( #15500, #37087, #9746, #7320 ) ) ;
#32216=DIRECTION ( 'NONE',  ( 0.000000000000000000, 0.000000000000000000, 1.000000000000000000 ) ) ;
#32217=EDGE_LOOP ( 'NONE', ( #36643, #21440 ) ) ;
#32218=VECTOR ( 'NONE', #11397, 1000.000000000000000 ) ;
#32220=EDGE_CURVE ( 'NONE', #31117, #27431, #14065, .T. ) ;
#32221=AXIS2_PLACEMENT_3D ( 'NONE', #16880, #2062, #25156 ) ;
#32222=DIRECTION ( 'NONE',  ( 0.000000000000000000, 0.000000000000000000, -1.000000000000000000 ) ) ;
#32223=CARTESIAN_POINT ( 'NONE',  ( 16.99999662536859901, 77.94228634059957983, 17.49999999999999645 ) ) ;
#32224=ORIENTED_EDGE ( 'NONE', *, *, #26233, .F. ) ;
#32225=ORIENTED_EDGE ( 'NONE', *, *, #17911, .F. ) ;
#32226=CIRCLE ( 'NONE', #30450, 2.000000000000001776 ) ;
#32227=ORIENTED_EDGE ( 'NONE', *, *, #28204, .T. ) ;
#32228=CIRCLE ( 'NONE', #26242, 2.000000000000001776 ) ;
#32229=EDGE_LOOP ( 'NONE', ( #12788, #13725 ) ) ;
#32231=CARTESIAN_POINT ( 'NONE',  ( -72.00000337463102085, -51.96152422706641971, 17.49999999999999645 ) ) ;
#32233=CYLINDRICAL_SURFACE ( 'NONE', #10215, 2.000000000000001776 ) ;
#32234=ORIENTED_EDGE ( 'NONE', *, *, #34671, .F. ) ;
#32235=DIRECTION ( 'NONE',  ( 1.000000000000000000, 0.000000000000000000, 0.000000000000000000 ) ) ;
#32237=DIRECTION ( 'NONE',  ( 0.000000000000000000, 0.000000000000000000, 1.000000000000000000 ) ) ;
#32239=DIRECTION ( 'NONE',  ( 1.000000000000000000, 0.000000000000000000, 0.000000000000000000 ) ) ;
#32241=AXIS2_PLACEMENT_3D ( 'NONE', #5669, #28541, #214 ) ;
#32242=CARTESIAN_POINT ( 'NONE',  ( 32.99999662536855283, -60.62177826491080168, 12.50000000000000000 ) ) ;
#32243=CARTESIAN_POINT ( 'NONE',  ( -37.00000337463116296, 60.62177826491077326, 17.49999999999999645 ) ) ;
#32244=VERTEX_POINT ( 'NONE', #22304 ) ;
#32245=LINE ( 'NONE', #9572, #501 ) ;
#32246=CARTESIAN_POINT ( 'NONE',  ( -56.13646009116099123, 70.47608876694653190, 12.49999999999999822 ) ) ;
#32247=ORIENTED_EDGE ( 'NONE', *, *, #31039, .T. ) ;
#32248=ADVANCED_FACE ( 'NONE', ( #8046 ), #14231, .F. ) ;
#32250=CARTESIAN_POINT ( 'NONE',  ( -63.00000337463104927, -25.98076211353322051, -9.999999999999998224 ) ) ;
#32253=DIRECTION ( 'NONE',  ( 1.000000000000000000, 0.000000000000000000, 0.000000000000000000 ) ) ;
#32254=DIRECTION ( 'NONE',  ( 1.000000000000000000, 0.000000000000000000, 0.000000000000000000 ) ) ;
#32255=CARTESIAN_POINT ( 'NONE',  ( 42.99999662536848888, 60.62177826491077326, -9.999999999999998224 ) ) ;
#32256=ORIENTED_EDGE ( 'NONE', *, *, #11737, .F. ) ;
#32257=CIRCLE ( 'NONE', #32861, 1.999999999999998224 ) ;
#32258=EDGE_CURVE ( 'NONE', #14036, #5415, #7492, .T. ) ;
#32259=DIRECTION ( 'NONE',  ( -1.000000000000000000, 0.000000000000000000, 0.000000000000000000 ) ) ;
#32260=DIRECTION ( 'NONE',  ( 0.000000000000000000, 0.000000000000000000, 1.000000000000000000 ) ) ;
#32262=CIRCLE ( 'NONE', #20904, 2.000000000000001776 ) ;
#32264=CARTESIAN_POINT ( 'NONE',  ( 74.99999662536836809, 43.30127018922198801, -5.000000000000000000 ) ) ;
#32266=CIRCLE ( 'NONE', #18508, 2.000000000000001776 ) ;
#32267=CYLINDRICAL_SURFACE ( 'NONE', #18715, 2.000000000000001776 ) ;
#32268=LINE ( 'NONE', #20835, #30188 ) ;
#32269=AXIS2_PLACEMENT_3D ( 'NONE', #19831, #20192, #5406 ) ;
#32270=ADVANCED_FACE ( 'NONE', ( #145 ), #20029, .F. ) ;
#32271=DIRECTION ( 'NONE',  ( 1.000000000000000000, 0.000000000000000000, 0.000000000000000000 ) ) ;
#32273=VECTOR ( 'NONE', #658, 1000.000000000000000 ) ;
#32274=EDGE_LOOP ( 'NONE', ( #3589, #32933, #12663, #30409 ) ) ;
#32275=CARTESIAN_POINT ( 'NONE',  ( -83.47442710120355969, 31.09745072740822991, 12.49999999999999645 ) ) ;
#32276=DIRECTION ( 'NONE',  ( 1.000000000000000000, 0.000000000000000000, 0.000000000000000000 ) ) ;
#32277=ORIENTED_EDGE ( 'NONE', *, *, #14919, .F. ) ;
#32278=CYLINDRICAL_SURFACE ( 'NONE', #9968, 2.000000000000000000 ) ;
#32280=FACE_BOUND ( 'NONE', #3801, .T. ) ;
#32281=CIRCLE ( 'NONE', #16147, 2.000000000000001776 ) ;
#32282=CYLINDRICAL_SURFACE ( 'NONE', #8842, 3.000000000000005773 ) ;
#32284=DIRECTION ( 'NONE',  ( 0.000000000000000000, 0.000000000000000000, -1.000000000000000000 ) ) ;
#32285=ORIENTED_EDGE ( 'NONE', *, *, #5405, .T. ) ;
#32286=DIRECTION ( 'NONE',  ( 0.000000000000000000, 0.000000000000000000, 1.000000000000000000 ) ) ;
#32287=EDGE_CURVE ( 'NONE', #30934, #19087, #26773, .T. ) ;
#32289=VECTOR ( 'NONE', #30274, 1000.000000000000000 ) ;
#32290=CYLINDRICAL_SURFACE ( 'NONE', #22982, 2.000000000000001776 ) ;
#32291=EDGE_LOOP ( 'NONE', ( #21040, #36195, #6505 ) ) ;
#32294=CARTESIAN_POINT ( 'NONE',  ( -27.78182860042817026, -56.67878100130359087, -4.999999999999997335 ) ) ;
#32295=CIRCLE ( 'NONE', #16742, 2.000000000000000000 ) ;
#32296=ORIENTED_EDGE ( 'NONE', *, *, #31424, .F. ) ;
#32297=EDGE_CURVE ( 'NONE', #19079, #7505, #32636, .T. ) ;
#32298=VERTEX_POINT ( 'NONE', #20403 ) ;
#32299=VECTOR ( 'NONE', #14743, 1000.000000000000000 ) ;
#32302=DIRECTION ( 'NONE',  ( 0.000000000000000000, 0.000000000000000000, 1.000000000000000000 ) ) ;
#32303=CYLINDRICAL_SURFACE ( 'NONE', #7417, 2.000000000000000000 ) ;
#32305=DIRECTION ( 'NONE',  ( 0.000000000000000000, 0.000000000000000000, 1.000000000000000000 ) ) ;
#32306=ORIENTED_EDGE ( 'NONE', *, *, #15587, .F. ) ;
#32307=VERTEX_POINT ( 'NONE', #6333 ) ;
#32308=CIRCLE ( 'NONE', #16161, 1.999999999999998224 ) ;
#32310=DIRECTION ( 'NONE',  ( -1.000000000000000000, 0.000000000000000000, 0.000000000000000000 ) ) ;
#32311=VERTEX_POINT ( 'NONE', #23227 ) ;
#32313=VERTEX_POINT ( 'NONE', #29210 ) ;
#32314=CIRCLE ( 'NONE', #15572, 2.000000000000001776 ) ;
#32316=ORIENTED_EDGE ( 'NONE', *, *, #4360, .F. ) ;
#32317=EDGE_LOOP ( 'NONE', ( #32322, #6540 ) ) ;
#32318=CARTESIAN_POINT ( 'NONE',  ( 64.99999662536839651, 60.62177826491078747, -9.999999999999998224 ) ) ;
#32319=DIRECTION ( 'NONE',  ( 0.000000000000000000, 0.000000000000000000, -1.000000000000000000 ) ) ;
#32320=EDGE_CURVE ( 'NONE', #11272, #7613, #3311, .T. ) ;
#32321=DIRECTION ( 'NONE',  ( 1.000000000000000000, 0.000000000000000000, 0.000000000000000000 ) ) ;
#32322=ORIENTED_EDGE ( 'NONE', *, *, #35551, .F. ) ;
#32323=VERTEX_POINT ( 'NONE', #26577 ) ;
#32324=CARTESIAN_POINT ( 'NONE',  ( 61.99999662536842493, -51.96152422706639840, -9.999999999999998224 ) ) ;
#32326=DIRECTION ( 'NONE',  ( 1.000000000000000000, 0.000000000000000000, 0.000000000000000000 ) ) ;
#32328=ORIENTED_EDGE ( 'NONE', *, *, #36892, .T. ) ;
#32329=DIRECTION ( 'NONE',  ( 0.000000000000000000, 0.000000000000000000, 1.000000000000000000 ) ) ;
#32330=CARTESIAN_POINT ( 'NONE',  ( 72.99999662536835388, -25.98076211353319565, 12.50000000000000000 ) ) ;
#32331=ORIENTED_EDGE ( 'NONE', *, *, #3146, .F. ) ;
#32332=AXIS2_PLACEMENT_3D ( 'NONE', #23867, #32464, #7348 ) ;
#32333=CARTESIAN_POINT ( 'NONE',  ( -63.00000337463102085, 60.62177826491077326, -9.999999999999998224 ) ) ;
#32334=DIRECTION ( 'NONE',  ( 1.000000000000000000, 0.000000000000000000, 0.000000000000000000 ) ) ;
#32335=CIRCLE ( 'NONE', #11355, 2.000000000000001776 ) ;
#32336=DIRECTION ( 'NONE',  ( 0.000000000000000000, 0.000000000000000000, 1.000000000000000000 ) ) ;
#32337=DIRECTION ( 'NONE',  ( 0.000000000000000000, 0.000000000000000000, -1.000000000000000000 ) ) ;
#32341=CARTESIAN_POINT ( 'NONE',  ( 9.999996625368655856, -86.60254037844400443, -9.999999999999998224 ) ) ;
#32343=ADVANCED_FACE ( 'NONE', ( #15330 ), #9329, .F. ) ;
#32344=DIRECTION ( 'NONE',  ( 0.4999999999999919509, -0.8660254037844432595, 0.000000000000000000 ) ) ;
#32345=CIRCLE ( 'NONE', #32943, 2.000000000000001776 ) ;
#32346=DIRECTION ( 'NONE',  ( 0.000000000000000000, 0.000000000000000000, -1.000000000000000000 ) ) ;
#32347=CARTESIAN_POINT ( 'NONE',  ( -25.00000337463120914, 77.94228634059957983, 12.50000000000000000 ) ) ;
#32348=ORIENTED_EDGE ( 'NONE', *, *, #31625, .T. ) ;
#32350=EDGE_LOOP ( 'NONE', ( #5111, #31779 ) ) ;
#32351=ORIENTED_EDGE ( 'NONE', *, *, #21361, .T. ) ;
#32352=CARTESIAN_POINT ( 'NONE',  ( 24.99999662536857059, 77.94228634059957983, 12.50000000000000000 ) ) ;
#32353=DIRECTION ( 'NONE',  ( 0.000000000000000000, 0.000000000000000000, 1.000000000000000000 ) ) ;
#32354=AXIS2_PLACEMENT_3D ( 'NONE', #2431, #4880, #33569 ) ;
#32355=EDGE_CURVE ( 'NONE', #16050, #32632, #31819, .T. ) ;
#32356=DIRECTION ( 'NONE',  ( 1.000000000000000000, 0.000000000000000000, 0.000000000000000000 ) ) ;
#32357=ADVANCED_FACE ( 'NONE', ( #6534 ), #17970, .F. ) ;
#32358=LINE ( 'NONE', #30090, #11918 ) ;
#32359=DIRECTION ( 'NONE',  ( 1.000000000000000000, 0.000000000000000000, 0.000000000000000000 ) ) ;
#32360=ORIENTED_EDGE ( 'NONE', *, *, #1476, .F. ) ;
#32361=AXIS2_PLACEMENT_3D ( 'NONE', #1728, #4350, #24616 ) ;
#32362=CARTESIAN_POINT ( 'NONE',  ( 6.999996625368645198, 77.94228634059957983, -9.999999999999998224 ) ) ;
#32363=ORIENTED_EDGE ( 'NONE', *, *, #1109, .F. ) ;
#32364=FACE_BOUND ( 'NONE', #36103, .T. ) ;
#32365=AXIS2_PLACEMENT_3D ( 'NONE', #6016, #20428, #23253 ) ;
#32366=EDGE_CURVE ( 'NONE', #5185, #7360, #2106, .T. ) ;
#32367=EDGE_CURVE ( 'NONE', #5101, #23102, #11767, .T. ) ;
#32368=CARTESIAN_POINT ( 'NONE',  ( -68.00000337463099243, 17.32050807568877460, -9.999999999999998224 ) ) ;
#32369=EDGE_CURVE ( 'NONE', #21899, #1539, #31436, .T. ) ;
#32370=EDGE_CURVE ( 'NONE', #7742, #28884, #15279, .T. ) ;
#32371=DIRECTION ( 'NONE',  ( -0.000000000000000000, 0.000000000000000000, -1.000000000000000000 ) ) ;
#32372=ORIENTED_EDGE ( 'NONE', *, *, #2904, .F. ) ;
#32373=DIRECTION ( 'NONE',  ( 0.000000000000000000, 0.000000000000000000, 1.000000000000000000 ) ) ;
#32375=FACE_OUTER_BOUND ( 'NONE', #26385, .T. ) ;
#32377=DIRECTION ( 'NONE',  ( 0.000000000000000000, 0.000000000000000000, 1.000000000000000000 ) ) ;
#32378=VERTEX_POINT ( 'NONE', #28831 ) ;
#32379=DIRECTION ( 'NONE',  ( -0.000000000000000000, -0.000000000000000000, 1.000000000000000000 ) ) ;
#32380=DIRECTION ( 'NONE',  ( 1.000000000000000000, 0.000000000000000000, 0.000000000000000000 ) ) ;
#32381=CARTESIAN_POINT ( 'NONE',  ( 14.80603122773118230, -87.83969979969864994, -49.86561046011506448 ) ) ;
#32382=ORIENTED_EDGE ( 'NONE', *, *, #16330, .T. ) ;
#32383=ORIENTED_EDGE ( 'NONE', *, *, #18194, .T. ) ;
#32384=AXIS2_PLACEMENT_3D ( 'NONE', #31448, #2981, #23406 ) ;
#32385=VERTEX_POINT ( 'NONE', #3156 ) ;
#32386=LINE ( 'NONE', #23571, #14152 ) ;
#32388=EDGE_CURVE ( 'NONE', #13513, #19051, #533, .T. ) ;
#32389=CARTESIAN_POINT ( 'NONE',  ( 43.00330684490809574, 60.50675687296563865, -5.000000000000000000 ) ) ;
#32390=DIRECTION ( 'NONE',  ( 1.000000000000000000, 0.000000000000000000, 0.000000000000000000 ) ) ;
#32391=DIRECTION ( 'NONE',  ( 1.000000000000000000, 0.000000000000000000, 0.000000000000000000 ) ) ;
#32392=CARTESIAN_POINT ( 'NONE',  ( -12.00000337463128908, 69.28203230275516944, 12.50000000000000000 ) ) ;
#32393=ORIENTED_EDGE ( 'NONE', *, *, #4384, .F. ) ;
#32394=ORIENTED_EDGE ( 'NONE', *, *, #36146, .F. ) ;
#32395=CARTESIAN_POINT ( 'NONE',  ( 81.99999662536833966, 34.64101615137759183, -9.999999999999998224 ) ) ;
#32396=CARTESIAN_POINT ( 'NONE',  ( 81.99999662536833966, 17.32050807568879236, 12.50000000000000000 ) ) ;
#32397=VERTEX_POINT ( 'NONE', #9141 ) ;
#32399=ORIENTED_EDGE ( 'NONE', *, *, #15234, .T. ) ;
#32400=VECTOR ( 'NONE', #31461, 1000.000000000000000 ) ;
#32401=FACE_BOUND ( 'NONE', #31564, .T. ) ;
#32402=ORIENTED_EDGE ( 'NONE', *, *, #15142, .F. ) ;
#32403=VERTEX_POINT ( 'NONE', #22087 ) ;
#32404=EDGE_CURVE ( 'NONE', #30579, #8438, #24272, .T. ) ;
#32405=DIRECTION ( 'NONE',  ( 0.000000000000000000, 0.000000000000000000, -1.000000000000000000 ) ) ;
#32406=EDGE_LOOP ( 'NONE', ( #18364, #28673 ) ) ;
#32408=DIRECTION ( 'NONE',  ( 1.000000000000000000, 0.000000000000000000, 0.000000000000000000 ) ) ;
#32409=DIRECTION ( 'NONE',  ( 0.000000000000000000, 0.000000000000000000, 1.000000000000000000 ) ) ;
#32410=CARTESIAN_POINT ( 'NONE',  ( 56.99999662536844625, -60.62177826491080168, -9.999999999999998224 ) ) ;
#32411=VERTEX_POINT ( 'NONE', #15890 ) ;
#32412=EDGE_LOOP ( 'NONE', ( #18061, #28968, #22040, #779, #24028, #15995, #16237, #27027, #26512, #30422 ) ) ;
#32413=ORIENTED_EDGE ( 'NONE', *, *, #16234, .T. ) ;
#32414=EDGE_LOOP ( 'NONE', ( #16484, #22140, #30389, #20392 ) ) ;
#32415=ORIENTED_EDGE ( 'NONE', *, *, #8744, .F. ) ;
#32416=CARTESIAN_POINT ( 'NONE',  ( -7.000003374631269537, -77.94228634059960825, 17.49999999999999645 ) ) ;
#32417=CIRCLE ( 'NONE', #19873, 2.000000000000001776 ) ;
#32419=ORIENTED_EDGE ( 'NONE', *, *, #17345, .F. ) ;
#32420=CIRCLE ( 'NONE', #25830, 2.000000000000001776 ) ;
#32421=DIRECTION ( 'NONE',  ( 0.000000000000000000, 0.000000000000000000, -1.000000000000000000 ) ) ;
#32424=ADVANCED_FACE ( 'NONE', ( #4279 ), #18891, .F. ) ;
#32425=VERTEX_POINT ( 'NONE', #21525 ) ;
#32426=CARTESIAN_POINT ( 'NONE',  ( -65.00000337463104927, -43.30127018922202353, -9.999999999999998224 ) ) ;
#32427=EDGE_CURVE ( 'NONE', #32859, #23693, #18302, .T. ) ;
#32429=DIRECTION ( 'NONE',  ( -1.000000000000000000, 0.000000000000000000, -0.000000000000000000 ) ) ;
#32430=ORIENTED_EDGE ( 'NONE', *, *, #36470, .F. ) ;
#32431=CARTESIAN_POINT ( 'NONE',  ( -35.19434990244938888, 52.39915983220783602, -49.22241343995295892 ) ) ;
#32432=ADVANCED_FACE ( 'NONE', ( #9889 ), #18536, .F. ) ;
#32434=ORIENTED_EDGE ( 'NONE', *, *, #34446, .F. ) ;
#32435=EDGE_LOOP ( 'NONE', ( #33127, #4306, #23939, #21896, #13823 ) ) ;
#32437=DIRECTION ( 'NONE',  ( 0.000000000000000000, 0.000000000000000000, 1.000000000000000000 ) ) ;
#32439=LINE ( 'NONE', #26826, #1298 ) ;
#32441=ORIENTED_EDGE ( 'NONE', *, *, #20004, .T. ) ;
#32442=DIRECTION ( 'NONE',  ( 0.000000000000000000, 0.000000000000000000, 1.000000000000000000 ) ) ;
#32443=CYLINDRICAL_SURFACE ( 'NONE', #1542, 1.999999999999998224 ) ;
#32444=EDGE_LOOP ( 'NONE', ( #35335, #31857, #27121, #30334 ) ) ;
#32445=CIRCLE ( 'NONE', #31830, 2.000000000000001776 ) ;
#32446=ADVANCED_FACE ( 'NONE', ( #21325 ), #24143, .T. ) ;
#32447=DIRECTION ( 'NONE',  ( -1.000000000000000000, 0.000000000000000000, -0.000000000000000000 ) ) ;
#32450=CARTESIAN_POINT ( 'NONE',  ( 1.999996625368696490, -86.60254037844400443, -5.000000000000000000 ) ) ;
#32451=CARTESIAN_POINT ( 'NONE',  ( -55.00000337463107059, 43.30127018922197379, -5.000000000000000000 ) ) ;
#32452=VERTEX_POINT ( 'NONE', #24709 ) ;
#32454=DIRECTION ( 'NONE',  ( 0.000000000000000000, 0.000000000000000000, 1.000000000000000000 ) ) ;
#32456=DIRECTION ( 'NONE',  ( 0.000000000000000000, 0.000000000000000000, 1.000000000000000000 ) ) ;
#32457=EDGE_CURVE ( 'NONE', #30617, #182, #24892, .T. ) ;
#32458=FACE_BOUND ( 'NONE', #1427, .T. ) ;
#32459=DIRECTION ( 'NONE',  ( 0.000000000000000000, 0.000000000000000000, -1.000000000000000000 ) ) ;
#32461=DIRECTION ( 'NONE',  ( -1.000000000000000000, 0.000000000000000000, 0.000000000000000000 ) ) ;
#32463=CYLINDRICAL_SURFACE ( 'NONE', #13500, 3.000000000000002665 ) ;
#32464=DIRECTION ( 'NONE',  ( 0.000000000000000000, 0.000000000000000000, -1.000000000000000000 ) ) ;
#32466=CIRCLE ( 'NONE', #28874, 2.000000000000001776 ) ;
#32468=ORIENTED_EDGE ( 'NONE', *, *, #7577, .T. ) ;
#32469=CARTESIAN_POINT ( 'NONE',  ( 58.48108235278871803, 36.97203788308965500, 12.49999999999999645 ) ) ;
#32470=EDGE_CURVE ( 'NONE', #15896, #31042, #2138, .T. ) ;
#32471=CARTESIAN_POINT ( 'NONE',  ( 0.000000000000000000, 0.000000000000000000, 12.49999999999999822 ) ) ;
#32472=CARTESIAN_POINT ( 'NONE',  ( -42.00000337463114164, 69.28203230275516944, -9.999999999999998224 ) ) ;
#32473=ORIENTED_EDGE ( 'NONE', *, *, #5157, .T. ) ;
#32475=EDGE_CURVE ( 'NONE', #33006, #21999, #10514, .T. ) ;
#32477=DIRECTION ( 'NONE',  ( 0.000000000000000000, 0.000000000000000000, 1.000000000000000000 ) ) ;
#32478=CARTESIAN_POINT ( 'NONE',  ( -58.00000337463104216, 51.96152422706639129, -9.999999999999998224 ) ) ;
#32480=EDGE_LOOP ( 'NONE', ( #38, #27835 ) ) ;
#32481=ORIENTED_EDGE ( 'NONE', *, *, #16249, .F. ) ;
#32484=ORIENTED_EDGE ( 'NONE', *, *, #15291, .T. ) ;
#32485=ORIENTED_EDGE ( 'NONE', *, *, #7960, .F. ) ;
#32487=ORIENTED_EDGE ( 'NONE', *, *, #7511, .T. ) ;
#32488=ORIENTED_EDGE ( 'NONE', *, *, #25134, .F. ) ;
#32489=EDGE_CURVE ( 'NONE', #21698, #35086, #29958, .T. ) ;
#32490=FACE_OUTER_BOUND ( 'NONE', #1993, .T. ) ;
#32491=AXIS2_PLACEMENT_3D ( 'NONE', #12069, #31267, #19846 ) ;
#32493=VERTEX_POINT ( 'NONE', #6886 ) ;
#32494=VERTEX_POINT ( 'NONE', #1445 ) ;
#32495=FACE_OUTER_BOUND ( 'NONE', #3054, .T. ) ;
#32498=CARTESIAN_POINT ( 'NONE',  ( 0.000000000000000000, 0.000000000000000000, 17.49999999999999645 ) ) ;
#32499=CARTESIAN_POINT ( 'NONE',  ( 26.99999662536856704, 77.94228634059957983, -9.999999999999998224 ) ) ;
#32500=ORIENTED_EDGE ( 'NONE', *, *, #31836, .F. ) ;
#32501=CARTESIAN_POINT ( 'NONE',  ( 54.99999662536844625, -60.62177826491080168, -9.999999999999998224 ) ) ;
#32502=DIRECTION ( 'NONE',  ( 0.000000000000000000, 0.000000000000000000, 1.000000000000000000 ) ) ;
#32503=ADVANCED_FACE ( 'NONE', ( #18332 ), #29759, .F. ) ;
#32504=VERTEX_POINT ( 'NONE', #16097 ) ;
#32505=CARTESIAN_POINT ( 'NONE',  ( 29.99999662536856349, 69.28203230275518365, -9.999999999999998224 ) ) ;
#32506=DIRECTION ( 'NONE',  ( -1.000000000000000000, 0.000000000000000000, 0.000000000000000000 ) ) ;
#32509=CARTESIAN_POINT ( 'NONE',  ( 56.52018970185258695, -35.83991598322081273, 12.49999999999999822 ) ) ;
#32510=CIRCLE ( 'NONE', #4367, 2.000000000000001776 ) ;
#32511=CARTESIAN_POINT ( 'NONE',  ( 64.99999662536842493, 43.30127018922200222, -9.999999999999998224 ) ) ;
#32513=ORIENTED_EDGE ( 'NONE', *, *, #28434, .F. ) ;
#32514=CARTESIAN_POINT ( 'NONE',  ( 56.67878100130369035, -27.78182860042797131, 12.49999999999999822 ) ) ;
#32515=CARTESIAN_POINT ( 'NONE',  ( 79.99999662536833966, 34.64101615137759183, -5.000000000000000000 ) ) ;
#32516=DIRECTION ( 'NONE',  ( 1.000000000000000000, 0.000000000000000000, 0.000000000000000000 ) ) ;
#32518=ORIENTED_EDGE ( 'NONE', *, *, #18585, .T. ) ;
#32519=ORIENTED_EDGE ( 'NONE', *, *, #3628, .T. ) ;
#32520=EDGE_CURVE ( 'NONE', #21264, #23931, #22506, .T. ) ;
#32521=AXIS2_PLACEMENT_3D ( 'NONE', #16386, #13574, #36463 ) ;
#32522=DIRECTION ( 'NONE',  ( 1.000000000000000000, 0.000000000000000000, 0.000000000000000000 ) ) ;
#32523=CARTESIAN_POINT ( 'NONE',  ( 49.99999662536846756, -69.28203230275519786, -9.999999999999998224 ) ) ;
#32524=DIRECTION ( 'NONE',  ( -1.000000000000000000, 0.000000000000000000, 0.000000000000000000 ) ) ;
#32526=DIRECTION ( 'NONE',  ( 0.000000000000000000, 0.000000000000000000, 1.000000000000000000 ) ) ;
#32527=DIRECTION ( 'NONE',  ( 0.000000000000000000, 0.000000000000000000, 1.000000000000000000 ) ) ;
#32528=ORIENTED_EDGE ( 'NONE', *, *, #3052, .F. ) ;
#32530=ORIENTED_EDGE ( 'NONE', *, *, #9971, .F. ) ;
#32531=FACE_BOUND ( 'NONE', #13719, .T. ) ;
#32534=EDGE_CURVE ( 'NONE', #27413, #5488, #5147, .T. ) ;
#32536=FACE_OUTER_BOUND ( 'NONE', #13458, .T. ) ;
#32537=DIRECTION ( 'NONE',  ( -0.000000000000000000, -0.000000000000000000, 1.000000000000000000 ) ) ;
#32538=EDGE_CURVE ( 'NONE', #34151, #27516, #20094, .T. ) ;
#32539=ORIENTED_EDGE ( 'NONE', *, *, #7466, .T. ) ;
#32540=DIRECTION ( 'NONE',  ( 1.000000000000000000, 0.000000000000000000, 0.000000000000000000 ) ) ;
#32542=ADVANCED_FACE ( 'NONE', ( #8561 ), #31069, .F. ) ;
#32543=CARTESIAN_POINT ( 'NONE',  ( 26.99999662536859546, -77.94228634059960825, -5.000000000000000000 ) ) ;
#32545=DIRECTION ( 'NONE',  ( -1.000000000000000000, 0.000000000000000000, 0.000000000000000000 ) ) ;
#32546=DIRECTION ( 'NONE',  ( -1.000000000000000000, 0.000000000000000000, 0.000000000000000000 ) ) ;
#32547=ORIENTED_EDGE ( 'NONE', *, *, #1790, .T. ) ;
#32548=CARTESIAN_POINT ( 'NONE',  ( -10.00000337463128730, 69.28203230275516944, 17.49999999999999645 ) ) ;
#32549=EDGE_CURVE ( 'NONE', #68, #13800, #11126, .T. ) ;
#32550=CARTESIAN_POINT ( 'NONE',  ( -10.00000337463128197, 86.60254037844397601, 17.49999999999999645 ) ) ;
#32551=DIRECTION ( 'NONE',  ( 1.000000000000000000, 0.000000000000000000, 0.000000000000000000 ) ) ;
#32553=CIRCLE ( 'NONE', #2611, 1.999999999999998224 ) ;
#32554=ORIENTED_EDGE ( 'NONE', *, *, #34300, .T. ) ;
#32556=EDGE_LOOP ( 'NONE', ( #7018, #31482 ) ) ;
#32558=CARTESIAN_POINT ( 'NONE',  ( 14.99999662536863632, -77.94228634059960825, -5.000000000000000000 ) ) ;
#32559=ADVANCED_FACE ( 'NONE', ( #2198 ), #34084, .F. ) ;
#32560=EDGE_CURVE ( 'NONE', #11572, #27066, #24902, .T. ) ;
#32562=CARTESIAN_POINT ( 'NONE',  ( -27.78182860042817026, -56.67878100130359087, 12.49999999999999822 ) ) ;
#32563=EDGE_CURVE ( 'NONE', #36578, #20452, #6931, .T. ) ;
#32564=EDGE_CURVE ( 'NONE', #31600, #13165, #2746, .T. ) ;
#32565=CARTESIAN_POINT ( 'NONE',  ( -27.78182860042817026, -56.67878100130359087, -4.999999999999997335 ) ) ;
#32567=EDGE_CURVE ( 'NONE', #20619, #33480, #30864, .T. ) ;
#32568=DIRECTION ( 'NONE',  ( 0.000000000000000000, 0.000000000000000000, 1.000000000000000000 ) ) ;
#32569=ORIENTED_EDGE ( 'NONE', *, *, #6671, .T. ) ;
#32570=AXIS2_PLACEMENT_3D ( 'NONE', #27187, #4898, #4335 ) ;
#32571=ORIENTED_EDGE ( 'NONE', *, *, #70, .T. ) ;
#32572=CARTESIAN_POINT ( 'NONE',  ( -45.00000337463112743, -60.62177826491080168, -9.999999999999998224 ) ) ;
#32573=AXIS2_PLACEMENT_3D ( 'NONE', #28702, #31689, #22891 ) ;
#32574=DIRECTION ( 'NONE',  ( -0.000000000000000000, 0.000000000000000000, -1.000000000000000000 ) ) ;
#32575=ORIENTED_EDGE ( 'NONE', *, *, #25976, .T. ) ;
#32576=CARTESIAN_POINT ( 'NONE',  ( -65.00000000000000000, 0.000000000000000000, 17.49999999999999645 ) ) ;
#32577=ORIENTED_EDGE ( 'NONE', *, *, #24579, .T. ) ;
#32578=FACE_BOUND ( 'NONE', #10815, .T. ) ;
#32580=EDGE_LOOP ( 'NONE', ( #20097, #17056, #28850, #16850 ) ) ;
#32581=DIRECTION ( 'NONE',  ( 1.000000000000000000, 0.000000000000000000, 0.000000000000000000 ) ) ;
#32582=ORIENTED_EDGE ( 'NONE', *, *, #22761, .F. ) ;
#32585=DIRECTION ( 'NONE',  ( 0.000000000000000000, 0.000000000000000000, 1.000000000000000000 ) ) ;
#32586=CARTESIAN_POINT ( 'NONE',  ( 49.99999662536846756, -69.28203230275519786, -5.000000000000000000 ) ) ;
#32587=CARTESIAN_POINT ( 'NONE',  ( 11.99999662536865763, -86.60254037844400443, -5.000000000000000000 ) ) ;
#32588=ORIENTED_EDGE ( 'NONE', *, *, #29534, .F. ) ;
#32590=VERTEX_POINT ( 'NONE', #5201 ) ;
#32591=VECTOR ( 'NONE', #36944, 1000.000000000000000 ) ;
#32592=AXIS2_PLACEMENT_3D ( 'NONE', #12701, #29405, #9900 ) ;
#32593=EDGE_LOOP ( 'NONE', ( #35428, #20900, #32382, #15644 ) ) ;
#32594=ORIENTED_EDGE ( 'NONE', *, *, #14972, .F. ) ;
#32595=FACE_OUTER_BOUND ( 'NONE', #7991, .T. ) ;
#32596=CIRCLE ( 'NONE', #8650, 2.000000000000001776 ) ;
#32597=CARTESIAN_POINT ( 'NONE',  ( 76.99999662536835388, -43.30127018922199511, -5.000000000000000000 ) ) ;
#32598=ORIENTED_EDGE ( 'NONE', *, *, #34868, .F. ) ;
#32599=CARTESIAN_POINT ( 'NONE',  ( -58.00000337463104216, 51.96152422706639129, 17.49999999999999645 ) ) ;
#32601=CARTESIAN_POINT ( 'NONE',  ( 69.99999662536838230, -51.96152422706639840, -5.000000000000000000 ) ) ;
#32602=ORIENTED_EDGE ( 'NONE', *, *, #16318, .F. ) ;
#32603=LINE ( 'NONE', #18574, #11637 ) ;
#32604=EDGE_CURVE ( 'NONE', #34166, #28642, #29074, .T. ) ;
#32605=DIRECTION ( 'NONE',  ( 0.000000000000000000, 0.000000000000000000, 1.000000000000000000 ) ) ;
#32606=AXIS2_PLACEMENT_3D ( 'NONE', #12349, #31686, #29426 ) ;
#32607=EDGE_CURVE ( 'NONE', #8583, #911, #8724, .T. ) ;
#32609=ORIENTED_EDGE ( 'NONE', *, *, #35042, .T. ) ;
#32610=DIRECTION ( 'NONE',  ( 0.000000000000000000, 0.000000000000000000, 1.000000000000000000 ) ) ;
#32612=LINE ( 'NONE', #18580, #7013 ) ;
#32613=ORIENTED_EDGE ( 'NONE', *, *, #6212, .T. ) ;
#32615=ORIENTED_EDGE ( 'NONE', *, *, #28542, .F. ) ;
#32616=DIRECTION ( 'NONE',  ( 1.000000000000000000, 0.000000000000000000, 0.000000000000000000 ) ) ;
#32617=DIRECTION ( 'NONE',  ( -1.000000000000000000, 0.000000000000000000, 0.000000000000000000 ) ) ;
#32618=DIRECTION ( 'NONE',  ( 0.8660254037844337116, -0.5000000000000084377, 0.000000000000000000 ) ) ;
#32619=CARTESIAN_POINT ( 'NONE',  ( 59.99999662536845335, 34.64101615137759893, -9.999999999999998224 ) ) ;
#32621=CARTESIAN_POINT ( 'NONE',  ( -67.00000337463102085, 25.98076211353317433, 12.50000000000000000 ) ) ;
#32623=DIRECTION ( 'NONE',  ( 1.000000000000000000, 0.000000000000000000, 0.000000000000000000 ) ) ;
#32624=VERTEX_POINT ( 'NONE', #18089 ) ;
#32625=LINE ( 'NONE', #12937, #11217 ) ;
#32626=ORIENTED_EDGE ( 'NONE', *, *, #21291, .T. ) ;
#32627=EDGE_CURVE ( 'NONE', #12872, #14823, #7519, .T. ) ;
#32628=CARTESIAN_POINT ( 'NONE',  ( 52.99999662536844625, -60.62177826491080168, -5.000000000000000000 ) ) ;
#32629=LINE ( 'NONE', #18770, #14605 ) ;
#32631=CARTESIAN_POINT ( 'NONE',  ( -60.00000337463107059, -34.64101615137762025, -5.000000000000000000 ) ) ;
#32632=VERTEX_POINT ( 'NONE', #837 ) ;
#32634=ORIENTED_EDGE ( 'NONE', *, *, #30685, .T. ) ;
#32635=CIRCLE ( 'NONE', #6305, 27.00000000000001776 ) ;
#32636=CIRCLE ( 'NONE', #22477, 2.000000000000001776 ) ;
#32638=VERTEX_POINT ( 'NONE', #17918 ) ;
#32639=CARTESIAN_POINT ( 'NONE',  ( 89.27079897466127534, -32.49191361593859995, -4.999999999999997335 ) ) ;
#32640=FACE_BOUND ( 'NONE', #6457, .T. ) ;
#32641=CARTESIAN_POINT ( 'NONE',  ( 9.999996625368655856, -69.28203230275519786, -9.999999999999998224 ) ) ;
#32642=LINE ( 'NONE', #34920, #12083 ) ;
#32643=VECTOR ( 'NONE', #18097, 1000.000000000000000 ) ;
#32644=CYLINDRICAL_SURFACE ( 'NONE', #17728, 2.000000000000000000 ) ;
#32645=ORIENTED_EDGE ( 'NONE', *, *, #14236, .F. ) ;
#32646=CARTESIAN_POINT ( 'NONE',  ( -25.00000337463120914, 77.94228634059957983, -9.999999999999998224 ) ) ;
#32647=CIRCLE ( 'NONE', #33871, 27.00000000000001421 ) ;
#32648=CIRCLE ( 'NONE', #10524, 2.000000000000001776 ) ;
#32649=CARTESIAN_POINT ( 'NONE',  ( -73.00000337463097821, -8.660254037844422825, -9.999999999999998224 ) ) ;
#32650=EDGE_CURVE ( 'NONE', #20452, #32323, #35685, .T. ) ;
#32651=CARTESIAN_POINT ( 'NONE',  ( -27.78182860042817026, -56.67878100130359087, -4.999999999999997335 ) ) ;
#32652=ORIENTED_EDGE ( 'NONE', *, *, #697, .T. ) ;
#32653=DIRECTION ( 'NONE',  ( 0.000000000000000000, 0.000000000000000000, 1.000000000000000000 ) ) ;
#32654=DIRECTION ( 'NONE',  ( 1.000000000000000000, 0.000000000000000000, 0.000000000000000000 ) ) ;
#32655=DIRECTION ( 'NONE',  ( 0.000000000000000000, 0.000000000000000000, 1.000000000000000000 ) ) ;
#32656=ORIENTED_EDGE ( 'NONE', *, *, #32297, .T. ) ;
#32657=ORIENTED_EDGE ( 'NONE', *, *, #17177, .T. ) ;
#32658=LINE ( 'NONE', #21424, #4954 ) ;
#32659=DIRECTION ( 'NONE',  ( 1.000000000000000000, 0.000000000000000000, 0.000000000000000000 ) ) ;
#32660=AXIS2_PLACEMENT_3D ( 'NONE', #6611, #6224, #17657 ) ;
#32661=CARTESIAN_POINT ( 'NONE',  ( -10.00000337463128730, 69.28203230275516944, 17.49999999999999645 ) ) ;
#32663=VERTEX_POINT ( 'NONE', #663 ) ;
#32664=CIRCLE ( 'NONE', #34472, 2.000000000000001776 ) ;
#32665=ORIENTED_EDGE ( 'NONE', *, *, #20296, .T. ) ;
#32667=VECTOR ( 'NONE', #10789, 1000.000000000000000 ) ;
#32669=CYLINDRICAL_SURFACE ( 'NONE', #6927, 2.000000000000001776 ) ;
#32670=ORIENTED_EDGE ( 'NONE', *, *, #22710, .T. ) ;
#32672=EDGE_LOOP ( 'NONE', ( #28061, #22439 ) ) ;
#32673=CARTESIAN_POINT ( 'NONE',  ( 46.99999662536851019, -60.62177826491080168, -5.000000000000000000 ) ) ;
#32676=VERTEX_POINT ( 'NONE', #9093 ) ;
#32677=AXIS2_PLACEMENT_3D ( 'NONE', #33135, #13267, #17197 ) ;
#32679=CARTESIAN_POINT ( 'NONE',  ( -55.00000337463110611, -43.30127018922202353, -9.999999999999998224 ) ) ;
#32680=VERTEX_POINT ( 'NONE', #23726 ) ;
#32681=ADVANCED_FACE ( 'NONE', ( #23368 ), #14920, .F. ) ;
#32682=ORIENTED_EDGE ( 'NONE', *, *, #3278, .T. ) ;
#32683=CARTESIAN_POINT ( 'NONE',  ( 71.99999662536838230, -51.96152422706639840, -9.999999999999998224 ) ) ;
#32684=DIRECTION ( 'NONE',  ( 1.000000000000000000, 0.000000000000000000, 0.000000000000000000 ) ) ;
#32685=CIRCLE ( 'NONE', #20140, 3.499999999999989342 ) ;
#32687=CARTESIAN_POINT ( 'NONE',  ( 32.99999662536855283, -77.94228634059960825, -9.999999999999998224 ) ) ;
#32689=CIRCLE ( 'NONE', #33289, 2.000000000000000000 ) ;
#32691=CYLINDRICAL_SURFACE ( 'NONE', #14757, 2.000000000000001776 ) ;
#32692=ORIENTED_EDGE ( 'NONE', *, *, #26626, .F. ) ;
#32696=AXIS2_PLACEMENT_3D ( 'NONE', #30007, #15584, #32623 ) ;
#32698=CARTESIAN_POINT ( 'NONE',  ( 74.99999662536836809, 8.660254037844394404, -9.999999999999998224 ) ) ;
#32700=AXIS2_PLACEMENT_3D ( 'NONE', #22454, #33905, #3524 ) ;
#32701=CARTESIAN_POINT ( 'NONE',  ( -33.00000337463116296, 77.94228634059957983, 17.49999999999999645 ) ) ;
#32702=DIRECTION ( 'NONE',  ( 1.000000000000000000, 0.000000000000000000, 0.000000000000000000 ) ) ;
#32703=EDGE_LOOP ( 'NONE', ( #14138, #13177 ) ) ;
#32704=DIRECTION ( 'NONE',  ( 0.000000000000000000, 0.000000000000000000, -1.000000000000000000 ) ) ;
#32705=CARTESIAN_POINT ( 'NONE',  ( -47.04203867989546950, 43.19957991610416315, 12.49999999999999822 ) ) ;
#32706=DIRECTION ( 'NONE',  ( 1.000000000000000000, 0.000000000000000000, 0.000000000000000000 ) ) ;
#32707=ORIENTED_EDGE ( 'NONE', *, *, #22376, .F. ) ;
#32708=AXIS2_PLACEMENT_3D ( 'NONE', #31212, #16957, #16408 ) ;
#32710=ORIENTED_EDGE ( 'NONE', *, *, #3345, .T. ) ;
#32711=VERTEX_POINT ( 'NONE', #9274 ) ;
#32712=CARTESIAN_POINT ( 'NONE',  ( 0.000000000000000000, 0.000000000000000000, 12.49999999999999822 ) ) ;
#32713=DIRECTION ( 'NONE',  ( 0.000000000000000000, 0.000000000000000000, 1.000000000000000000 ) ) ;
#32715=EDGE_LOOP ( 'NONE', ( #31302, #5274 ) ) ;
#32716=AXIS2_PLACEMENT_3D ( 'NONE', #24254, #21639, #21453 ) ;
#32718=LINE ( 'NONE', #21483, #5366 ) ;
#32719=VECTOR ( 'NONE', #33408, 1000.000000000000000 ) ;
#32720=CARTESIAN_POINT ( 'NONE',  ( -58.00000337463107059, -34.64101615137762025, -5.000000000000000000 ) ) ;
#32721=ORIENTED_EDGE ( 'NONE', *, *, #16427, .T. ) ;
#32722=EDGE_CURVE ( 'NONE', #2002, #14001, #8142, .T. ) ;
#32725=VERTEX_POINT ( 'NONE', #29154 ) ;
#32727=FACE_BOUND ( 'NONE', #6376, .T. ) ;
#32728=CIRCLE ( 'NONE', #30928, 2.000000000000001776 ) ;
#32729=AXIS2_PLACEMENT_3D ( 'NONE', #9783, #7534, #4544 ) ;
#32730=AXIS2_PLACEMENT_3D ( 'NONE', #22069, #33510, #7821 ) ;
#32731=CYLINDRICAL_SURFACE ( 'NONE', #23772, 2.000000000000001776 ) ;
#32733=CARTESIAN_POINT ( 'NONE',  ( 1.999996625368696490, -86.60254037844400443, -9.999999999999998224 ) ) ;
#32734=ORIENTED_EDGE ( 'NONE', *, *, #20793, .T. ) ;
#32740=DIRECTION ( 'NONE',  ( 0.000000000000000000, 0.000000000000000000, 1.000000000000000000 ) ) ;
#32741=CYLINDRICAL_SURFACE ( 'NONE', #19745, 2.000000000000001776 ) ;
#32742=ORIENTED_EDGE ( 'NONE', *, *, #15375, .F. ) ;
#32745=DIRECTION ( 'NONE',  ( 0.000000000000000000, 0.000000000000000000, -1.000000000000000000 ) ) ;
#32746=AXIS2_PLACEMENT_3D ( 'NONE', #21960, #28306, #2069 ) ;
#32747=ORIENTED_EDGE ( 'NONE', *, *, #19293, .F. ) ;
#32748=ORIENTED_EDGE ( 'NONE', *, *, #6789, .T. ) ;
#32749=AXIS2_PLACEMENT_3D ( 'NONE', #36369, #2233, #26164 ) ;
#32752=VECTOR ( 'NONE', #33405, 1000.000000000000000 ) ;
#32753=DIRECTION ( 'NONE',  ( -1.047444401652940007E-14, -1.000000000000000000, 0.000000000000000000 ) ) ;
#32754=LINE ( 'NONE', #15879, #14739 ) ;
#32756=AXIS2_PLACEMENT_3D ( 'NONE', #28706, #2845, #34332 ) ;
#32757=CYLINDRICAL_SURFACE ( 'NONE', #18640, 2.000000000000001776 ) ;
#32759=AXIS2_PLACEMENT_3D ( 'NONE', #31231, #34416, #2933 ) ;
#32761=ORIENTED_EDGE ( 'NONE', *, *, #31171, .F. ) ;
#32762=DIRECTION ( 'NONE',  ( 0.000000000000000000, 0.000000000000000000, 1.000000000000000000 ) ) ;
#32764=ADVANCED_FACE ( 'NONE', ( #15275 ), #14537, .F. ) ;
#32766=ORIENTED_EDGE ( 'NONE', *, *, #9771, .F. ) ;
#32767=VECTOR ( 'NONE', #33186, 1000.000000000000000 ) ;
#32768=EDGE_CURVE ( 'NONE', #10304, #24584, #14125, .T. ) ;
#32769=ORIENTED_EDGE ( 'NONE', *, *, #10234, .F. ) ;
#32770=CARTESIAN_POINT ( 'NONE',  ( -50.00000337463109190, 51.96152422706637708, -5.000000000000000000 ) ) ;
#32773=EDGE_CURVE ( 'NONE', #5559, #19449, #22536, .T. ) ;
#32775=ADVANCED_FACE ( 'NONE', ( #10223 ), #15661, .F. ) ;
#32776=ORIENTED_EDGE ( 'NONE', *, *, #28798, .T. ) ;
#32777=CARTESIAN_POINT ( 'NONE',  ( -78.00000337463094979, -2.428612866367529932E-14, 12.50000000000000000 ) ) ;
#32778=CIRCLE ( 'NONE', #20228, 27.00000000000001776 ) ;
#32779=AXIS2_PLACEMENT_3D ( 'NONE', #15832, #13576, #5139 ) ;
#32780=DIRECTION ( 'NONE',  ( -1.000000000000000000, 0.000000000000000000, -0.000000000000000000 ) ) ;
#32781=EDGE_LOOP ( 'NONE', ( #34261, #6720, #12372, #11664 ) ) ;
#32782=ORIENTED_EDGE ( 'NONE', *, *, #24185, .F. ) ;
#32783=DIRECTION ( 'NONE',  ( 1.000000000000000000, 0.000000000000000000, 0.000000000000000000 ) ) ;
#32784=ORIENTED_EDGE ( 'NONE', *, *, #11674, .T. ) ;
#32785=EDGE_CURVE ( 'NONE', #29590, #23780, #1780, .T. ) ;
#32787=CIRCLE ( 'NONE', #4045, 2.000000000000001776 ) ;
#32788=ADVANCED_FACE ( 'NONE', ( #24477 ), #1948, .F. ) ;
#32790=AXIS2_PLACEMENT_3D ( 'NONE', #20887, #32319, #3810 ) ;
#32791=ADVANCED_FACE ( 'NONE', ( #30461 ), #12644, .F. ) ;
#32794=EDGE_LOOP ( 'NONE', ( #31423, #31400 ) ) ;
#32795=DIRECTION ( 'NONE',  ( 0.000000000000000000, 0.000000000000000000, 1.000000000000000000 ) ) ;
#32796=ORIENTED_EDGE ( 'NONE', *, *, #949, .T. ) ;
#32798=ORIENTED_EDGE ( 'NONE', *, *, #30972, .T. ) ;
#32799=CARTESIAN_POINT ( 'NONE',  ( 37.99999662536853151, 69.28203230275518365, -9.999999999999998224 ) ) ;
#32800=CARTESIAN_POINT ( 'NONE',  ( 91.99999662536828282, 0.000000000000000000, 12.50000000000000000 ) ) ;
#32801=ORIENTED_EDGE ( 'NONE', *, *, #17216, .F. ) ;
#32802=AXIS2_PLACEMENT_3D ( 'NONE', #34079, #27684, #22426 ) ;
#32803=AXIS2_PLACEMENT_3D ( 'NONE', #5080, #21768, #16168 ) ;
#32804=DIRECTION ( 'NONE',  ( 0.000000000000000000, 0.000000000000000000, -1.000000000000000000 ) ) ;
#32805=CARTESIAN_POINT ( 'NONE',  ( 67.99999662536836809, -51.96152422706639840, -9.999999999999998224 ) ) ;
#32808=CIRCLE ( 'NONE', #13671, 2.000000000000001776 ) ;
#32809=DIRECTION ( 'NONE',  ( 1.000000000000000000, 0.000000000000000000, 0.000000000000000000 ) ) ;
#32810=EDGE_CURVE ( 'NONE', #30431, #33375, #34499, .T. ) ;
#32812=CARTESIAN_POINT ( 'NONE',  ( -42.00000337463114164, -69.28203230275519786, -9.999999999999998224 ) ) ;
#32813=DIRECTION ( 'NONE',  ( 1.000000000000000000, 0.000000000000000000, 0.000000000000000000 ) ) ;
#32814=ADVANCED_FACE ( 'NONE', ( #7226 ), #4232, .F. ) ;
#32815=FACE_OUTER_BOUND ( 'NONE', #34440, .T. ) ;
#32816=CYLINDRICAL_SURFACE ( 'NONE', #31024, 2.000000000000001776 ) ;
#32817=ORIENTED_EDGE ( 'NONE', *, *, #23763, .T. ) ;
#32818=EDGE_LOOP ( 'NONE', ( #29781, #33558 ) ) ;
#32819=AXIS2_PLACEMENT_3D ( 'NONE', #27170, #35829, #1691 ) ;
#32820=CARTESIAN_POINT ( 'NONE',  ( 74.99999662536836809, 25.98076211353319565, 12.50000000000000000 ) ) ;
#32821=CARTESIAN_POINT ( 'NONE',  ( 26.99999662536856704, 77.94228634059957983, -9.999999999999998224 ) ) ;
#32822=DIRECTION ( 'NONE',  ( 0.000000000000000000, 0.000000000000000000, 1.000000000000000000 ) ) ;
#32823=CARTESIAN_POINT ( 'NONE',  ( 64.99999662536839651, 60.62177826491078747, -5.000000000000000000 ) ) ;
#32825=ORIENTED_EDGE ( 'NONE', *, *, #8535, .T. ) ;
#32827=AXIS2_PLACEMENT_3D ( 'NONE', #23652, #27149, #33353 ) ;
#32828=DIRECTION ( 'NONE',  ( -0.000000000000000000, 0.000000000000000000, -1.000000000000000000 ) ) ;
#32829=CARTESIAN_POINT ( 'NONE',  ( 79.99999662536833966, 34.64101615137759183, 17.49999999999999645 ) ) ;
#32830=AXIS2_PLACEMENT_3D ( 'NONE', #17841, #34908, #29273 ) ;
#32832=AXIS2_PLACEMENT_3D ( 'NONE', #918, #12345, #23813 ) ;
#32833=DIRECTION ( 'NONE',  ( 1.000000000000000000, 0.000000000000000000, 0.000000000000000000 ) ) ;
#32834=EDGE_LOOP ( 'NONE', ( #255, #26168 ) ) ;
#32836=DIRECTION ( 'NONE',  ( 0.000000000000000000, 0.000000000000000000, 1.000000000000000000 ) ) ;
#32837=EDGE_CURVE ( 'NONE', #5148, #4, #18330, .T. ) ;
#32838=CARTESIAN_POINT ( 'NONE',  ( 86.99999662536832545, 8.660254037844394404, 12.50000000000000000 ) ) ;
#32839=AXIS2_PLACEMENT_3D ( 'NONE', #26064, #32034, #15011 ) ;
#32842=EDGE_CURVE ( 'NONE', #3287, #8594, #2165, .T. ) ;
#32843=ORIENTED_EDGE ( 'NONE', *, *, #16279, .F. ) ;
#32844=ORIENTED_EDGE ( 'NONE', *, *, #25267, .F. ) ;
#32845=AXIS2_PLACEMENT_3D ( 'NONE', #14463, #32, #28877 ) ;
#32846=CIRCLE ( 'NONE', #14297, 2.000000000000001776 ) ;
#32847=ORIENTED_EDGE ( 'NONE', *, *, #29905, .T. ) ;
#32849=FACE_BOUND ( 'NONE', #28313, .T. ) ;
#32850=DIRECTION ( 'NONE',  ( 1.000000000000000000, 0.000000000000000000, 0.000000000000000000 ) ) ;
#32851=DIRECTION ( 'NONE',  ( 0.000000000000000000, 0.000000000000000000, 1.000000000000000000 ) ) ;
#32853=VERTEX_POINT ( 'NONE', #12817 ) ;
#32856=CARTESIAN_POINT ( 'NONE',  ( 59.99999662536845335, 34.64101615137759893, -9.999999999999998224 ) ) ;
#32857=AXIS2_PLACEMENT_3D ( 'NONE', #24965, #31130, #33590 ) ;
#32858=FACE_OUTER_BOUND ( 'NONE', #3490, .T. ) ;
#32859=VERTEX_POINT ( 'NONE', #27639 ) ;
#32860=CARTESIAN_POINT ( 'NONE',  ( 62.99999662536842493, 43.30127018922200222, 12.50000000000000000 ) ) ;
#32861=AXIS2_PLACEMENT_3D ( 'NONE', #1758, #4572, #35353 ) ;
#32862=CARTESIAN_POINT ( 'NONE',  ( -52.39915983220772233, -35.19434990244957362, -49.22241343995298024 ) ) ;
#32863=EDGE_CURVE ( 'NONE', #19047, #33610, #15328, .T. ) ;
#32868=LINE ( 'NONE', #3991, #26543 ) ;
#32869=CARTESIAN_POINT ( 'NONE',  ( -68.00000000000000000, 0.000000000000000000, -4.999999999999997335 ) ) ;
#32871=EDGE_LOOP ( 'NONE', ( #36840, #16469, #23851, #8318, #30576, #12750, #2855, #36092, #18662, #24681, #29983, #20292 ) ) ;
#32872=EDGE_LOOP ( 'NONE', ( #36095, #10427, #21879, #14692 ) ) ;
#32873=AXIS2_PLACEMENT_3D ( 'NONE', #23978, #9143, #32208 ) ;
#32874=VECTOR ( 'NONE', #25370, 1000.000000000000000 ) ;
#32875=CARTESIAN_POINT ( 'NONE',  ( -55.88972745734155012, 34.00000000000049027, -4.999999999999997335 ) ) ;
#32879=CARTESIAN_POINT ( 'NONE',  ( -58.00000337463107059, -34.64101615137762025, -9.999999999999998224 ) ) ;
#32880=EDGE_LOOP ( 'NONE', ( #10865, #30751, #35903, #726, #26063 ) ) ;
#32881=ORIENTED_EDGE ( 'NONE', *, *, #150, .T. ) ;
#32882=DIRECTION ( 'NONE',  ( 1.000000000000000000, 0.000000000000000000, 0.000000000000000000 ) ) ;
#32883=CIRCLE ( 'NONE', #15515, 2.000000000000001776 ) ;
#32885=EDGE_CURVE ( 'NONE', #5353, #10671, #15475, .T. ) ;
#32887=VERTEX_POINT ( 'NONE', #4032 ) ;
#32889=CARTESIAN_POINT ( 'NONE',  ( 14.99999662536859901, 77.94228634059957983, 12.50000000000000000 ) ) ;
#32890=DIRECTION ( 'NONE',  ( 0.000000000000000000, 0.000000000000000000, 1.000000000000000000 ) ) ;
#32891=ORIENTED_EDGE ( 'NONE', *, *, #5981, .T. ) ;
#32893=AXIS2_PLACEMENT_3D ( 'NONE', #4047, #15287, #15487 ) ;
#32894=VERTEX_POINT ( 'NONE', #18660 ) ;
#32895=DIRECTION ( 'NONE',  ( 0.000000000000000000, 0.000000000000000000, 1.000000000000000000 ) ) ;
#32896=DIRECTION ( 'NONE',  ( 1.000000000000000000, 0.000000000000000000, 0.000000000000000000 ) ) ;
#32897=CARTESIAN_POINT ( 'NONE',  ( 95.00000000000000000, 1.163414459189985643E-14, 17.49999999999999645 ) ) ;
#32898=DIRECTION ( 'NONE',  ( 0.000000000000000000, 0.000000000000000000, 1.000000000000000000 ) ) ;
#32899=AXIS2_PLACEMENT_3D ( 'NONE', #25990, #5400, #8564 ) ;
#32900=DIRECTION ( 'NONE',  ( 1.000000000000000000, 0.000000000000000000, 0.000000000000000000 ) ) ;
#32904=AXIS2_PLACEMENT_3D ( 'NONE', #21464, #7394, #9657 ) ;
#32905=ORIENTED_EDGE ( 'NONE', *, *, #23329, .T. ) ;
#32906=CARTESIAN_POINT ( 'NONE',  ( 71.99999662536839651, 34.64101615137758472, 12.50000000000000000 ) ) ;
#32907=DIRECTION ( 'NONE',  ( 1.000000000000000000, 0.000000000000000000, 0.000000000000000000 ) ) ;
#32908=DIRECTION ( 'NONE',  ( 0.000000000000000000, 0.000000000000000000, -1.000000000000000000 ) ) ;
#32909=EDGE_CURVE ( 'NONE', #35698, #27018, #21921, .T. ) ;
#32910=VERTEX_POINT ( 'NONE', #30079 ) ;
#32912=ORIENTED_EDGE ( 'NONE', *, *, #717, .T. ) ;
#32913=AXIS2_PLACEMENT_3D ( 'NONE', #3864, #21117, #1426 ) ;
#32914=FACE_OUTER_BOUND ( 'NONE', #34391, .T. ) ;
#32915=DIRECTION ( 'NONE',  ( -1.000000000000000000, 0.000000000000000000, 0.000000000000000000 ) ) ;
#32919=ORIENTED_EDGE ( 'NONE', *, *, #14017, .T. ) ;
#32920=LINE ( 'NONE', #27091, #28097 ) ;
#32921=EDGE_CURVE ( 'NONE', #16940, #13964, #2759, .T. ) ;
#32925=ORIENTED_EDGE ( 'NONE', *, *, #25251, .F. ) ;
#32927=AXIS2_PLACEMENT_3D ( 'NONE', #8152, #22953, #19596 ) ;
#32928=AXIS2_PLACEMENT_3D ( 'NONE', #29176, #15112, #3683 ) ;
#32930=DIRECTION ( 'NONE',  ( 0.000000000000000000, 0.000000000000000000, -1.000000000000000000 ) ) ;
#32931=VECTOR ( 'NONE', #18979, 1000.000000000000000 ) ;
#32932=EDGE_CURVE ( 'NONE', #32411, #13754, #25772, .T. ) ;
#32933=ORIENTED_EDGE ( 'NONE', *, *, #35507, .F. ) ;
#32935=CIRCLE ( 'NONE', #31708, 2.000000000000001776 ) ;
#32937=DIRECTION ( 'NONE',  ( 1.000000000000000000, 0.000000000000000000, 0.000000000000000000 ) ) ;
#32938=CIRCLE ( 'NONE', #34739, 2.000000000000001776 ) ;
#32939=DIRECTION ( 'NONE',  ( 0.000000000000000000, 0.000000000000000000, 1.000000000000000000 ) ) ;
#32940=DIRECTION ( 'NONE',  ( 0.000000000000000000, 0.000000000000000000, -1.000000000000000000 ) ) ;
#32941=EDGE_LOOP ( 'NONE', ( #15107, #30027 ) ) ;
#32943=AXIS2_PLACEMENT_3D ( 'NONE', #5924, #5175, #16612 ) ;
#32944=DIRECTION ( 'NONE',  ( 0.000000000000000000, 0.000000000000000000, 1.000000000000000000 ) ) ;
#32945=DIRECTION ( 'NONE',  ( 1.000000000000000000, 0.000000000000000000, 0.000000000000000000 ) ) ;
#32946=EDGE_CURVE ( 'NONE', #10255, #36868, #33918, .T. ) ;
#32947=VERTEX_POINT ( 'NONE', #31012 ) ;
#32948=EDGE_CURVE ( 'NONE', #21723, #29660, #4559, .T. ) ;
#32950=CARTESIAN_POINT ( 'NONE',  ( 36.99999662536855283, -60.62177826491080168, -9.999999999999998224 ) ) ;
#32955=DIRECTION ( 'NONE',  ( 0.000000000000000000, 0.000000000000000000, 1.000000000000000000 ) ) ;
#32956=CARTESIAN_POINT ( 'NONE',  ( 16.99999662536859901, 77.94228634059957983, -9.999999999999998224 ) ) ;
#32957=EDGE_CURVE ( 'NONE', #5293, #28159, #9327, .T. ) ;
#32960=EDGE_LOOP ( 'NONE', ( #29276, #8428 ) ) ;
#32961=ORIENTED_EDGE ( 'NONE', *, *, #3236, .T. ) ;
#32962=DIRECTION ( 'NONE',  ( 0.000000000000000000, 0.000000000000000000, 1.000000000000000000 ) ) ;
#32963=EDGE_CURVE ( 'NONE', #24230, #28140, #5170, .T. ) ;
#32964=CARTESIAN_POINT ( 'NONE',  ( 9.999996625368618552, 69.28203230275516944, -9.999999999999998224 ) ) ;
#32967=ORIENTED_EDGE ( 'NONE', *, *, #4474, .F. ) ;
#32969=DIRECTION ( 'NONE',  ( 0.000000000000000000, 0.000000000000000000, 1.000000000000000000 ) ) ;
#32970=ORIENTED_EDGE ( 'NONE', *, *, #19858, .T. ) ;
#32972=DIRECTION ( 'NONE',  ( 1.000000000000000000, 0.000000000000000000, 0.000000000000000000 ) ) ;
#32973=EDGE_LOOP ( 'NONE', ( #23420, #35645, #9078, #31803 ) ) ;
#32974=CARTESIAN_POINT ( 'NONE',  ( 0.000000000000000000, 0.000000000000000000, -5.000000000000000000 ) ) ;
#32976=CARTESIAN_POINT ( 'NONE',  ( 59.99999662536842493, -51.96152422706639840, -9.999999999999998224 ) ) ;
#32977=FACE_OUTER_BOUND ( 'NONE', #17272, .T. ) ;
#32978=AXIS2_PLACEMENT_3D ( 'NONE', #29602, #3927, #15371 ) ;
#32979=ORIENTED_EDGE ( 'NONE', *, *, #13642, .F. ) ;
#32980=DIRECTION ( 'NONE',  ( 0.000000000000000000, 0.000000000000000000, 1.000000000000000000 ) ) ;
#32982=ORIENTED_EDGE ( 'NONE', *, *, #16804, .T. ) ;
#32985=VERTEX_POINT ( 'NONE', #19386 ) ;
#32986=DIRECTION ( 'NONE',  ( 0.000000000000000000, 0.000000000000000000, -1.000000000000000000 ) ) ;
#32987=EDGE_CURVE ( 'NONE', #13225, #8340, #34216, .T. ) ;
#32988=CARTESIAN_POINT ( 'NONE',  ( 64.99999662536839651, -43.30127018922199511, -9.999999999999998224 ) ) ;
#32994=DIRECTION ( 'NONE',  ( -1.000000000000000000, 0.000000000000000000, -0.000000000000000000 ) ) ;
#32996=DIRECTION ( 'NONE',  ( -1.000000000000000000, 0.000000000000000000, 0.000000000000000000 ) ) ;
#32997=CARTESIAN_POINT ( 'NONE',  ( -48.00000337463112032, -51.96152422706641971, -9.999999999999998224 ) ) ;
#32998=DIRECTION ( 'NONE',  ( 1.000000000000000000, 0.000000000000000000, 0.000000000000000000 ) ) ;
#32999=ORIENTED_EDGE ( 'NONE', *, *, #10234, .T. ) ;
#33001=LINE ( 'NONE', #24942, #34426 ) ;
#33002=EDGE_CURVE ( 'NONE', #5488, #1395, #23719, .T. ) ;
#33003=CARTESIAN_POINT ( 'NONE',  ( 19.99999662536861678, -86.60254037844400443, 12.50000000000000000 ) ) ;
#33004=DIRECTION ( 'NONE',  ( 0.000000000000000000, 0.000000000000000000, -1.000000000000000000 ) ) ;
#33005=DIRECTION ( 'NONE',  ( 0.000000000000000000, 0.000000000000000000, 1.000000000000000000 ) ) ;
#33006=VERTEX_POINT ( 'NONE', #22025 ) ;
#33007=FACE_OUTER_BOUND ( 'NONE', #20885, .T. ) ;
#33008=CARTESIAN_POINT ( 'NONE',  ( -60.00000337463107059, -34.64101615137762025, 12.50000000000000000 ) ) ;
#33009=DIRECTION ( 'NONE',  ( -0.000000000000000000, -0.000000000000000000, -1.000000000000000000 ) ) ;
#33011=FACE_OUTER_BOUND ( 'NONE', #3638, .T. ) ;
#33012=ORIENTED_EDGE ( 'NONE', *, *, #2027, .T. ) ;
#33013=SURFACE_SIDE_STYLE ('',( #9638 ) ) ;
#33014=DIRECTION ( 'NONE',  ( 0.000000000000000000, 0.000000000000000000, 1.000000000000000000 ) ) ;
#33016=CARTESIAN_POINT ( 'NONE',  ( 47.99999662536848177, -51.96152422706640550, 12.50000000000000000 ) ) ;
#33017=EDGE_CURVE ( 'NONE', #25535, #24313, #4951, .T. ) ;
#33018=CARTESIAN_POINT ( 'NONE',  ( -30.00000337463118427, 69.28203230275516944, -9.999999999999998224 ) ) ;
#33019=ORIENTED_EDGE ( 'NONE', *, *, #1639, .F. ) ;
#33020=EDGE_CURVE ( 'NONE', #28380, #167, #26118, .T. ) ;
#33021=ORIENTED_EDGE ( 'NONE', *, *, #18244, .F. ) ;
#33022=VECTOR ( 'NONE', #33175, 1000.000000000000000 ) ;
#33024=EDGE_LOOP ( 'NONE', ( #31666, #4866 ) ) ;
#33025=CARTESIAN_POINT ( 'NONE',  ( 52.39915983220795681, 35.19434990244919703, 12.49999999999999822 ) ) ;
#33027=ADVANCED_FACE ( 'NONE', ( #5513 ), #28016, .F. ) ;
#33028=CYLINDRICAL_SURFACE ( 'NONE', #2892, 2.000000000000001776 ) ;
#33030=DIRECTION ( 'NONE',  ( 1.000000000000000000, 0.000000000000000000, 0.000000000000000000 ) ) ;
#33031=EDGE_CURVE ( 'NONE', #6351, #2856, #29104, .T. ) ;
#33036=LINE ( 'NONE', #13520, #7655 ) ;
#33039=ORIENTED_EDGE ( 'NONE', *, *, #27532, .T. ) ;
#33040=ADVANCED_FACE ( 'NONE', ( #11120 ), #22569, .F. ) ;
#33041=EDGE_LOOP ( 'NONE', ( #10872, #25389, #28281, #6295 ) ) ;
#33043=CIRCLE ( 'NONE', #15084, 2.000000000000001776 ) ;
#33044=ADVANCED_FACE ( 'NONE', ( #3622, #32090, #11660, #6230, #5890, #9051, #15050, #26665, #18045 ), #23315, .F. ) ;
#33045=DIRECTION ( 'NONE',  ( 0.000000000000000000, 0.000000000000000000, 1.000000000000000000 ) ) ;
#33048=ORIENTED_EDGE ( 'NONE', *, *, #30932, .F. ) ;
#33049=ORIENTED_EDGE ( 'NONE', *, *, #7395, .T. ) ;
#33051=FACE_OUTER_BOUND ( 'NONE', #11617, .T. ) ;
#33053=ORIENTED_EDGE ( 'NONE', *, *, #24026, .F. ) ;
#33054=FACE_BOUND ( 'NONE', #29170, .T. ) ;
#33056=ORIENTED_EDGE ( 'NONE', *, *, #20630, .F. ) ;
#33057=DIRECTION ( 'NONE',  ( 1.000000000000000000, 0.000000000000000000, 0.000000000000000000 ) ) ;
#33058=FACE_OUTER_BOUND ( 'NONE', #2289, .T. ) ;
#33060=ORIENTED_EDGE ( 'NONE', *, *, #25628, .F. ) ;
#33061=CYLINDRICAL_SURFACE ( 'NONE', #1733, 2.000000000000001776 ) ;
#33062=DIRECTION ( 'NONE',  ( 0.000000000000000000, 0.000000000000000000, 1.000000000000000000 ) ) ;
#33066=DIRECTION ( 'NONE',  ( 1.000000000000000000, 0.000000000000000000, 0.000000000000000000 ) ) ;
#33067=CIRCLE ( 'NONE', #16298, 2.000000000000001776 ) ;
#33068=VERTEX_POINT ( 'NONE', #15222 ) ;
#33069=DIRECTION ( 'NONE',  ( 1.000000000000000000, 0.000000000000000000, 0.000000000000000000 ) ) ;
#33070=FACE_OUTER_BOUND ( 'NONE', #4745, .T. ) ;
#33071=DIRECTION ( 'NONE',  ( 0.000000000000000000, 0.000000000000000000, 1.000000000000000000 ) ) ;
#33072=CARTESIAN_POINT ( 'NONE',  ( 47.63139720814400846, -27.50000000000022737, -10.00000000000000000 ) ) ;
#33073=DIRECTION ( 'NONE',  ( 0.000000000000000000, 0.000000000000000000, 1.000000000000000000 ) ) ;
#33075=DIRECTION ( 'NONE',  ( -0.000000000000000000, -0.000000000000000000, 1.000000000000000000 ) ) ;
#33076=EDGE_LOOP ( 'NONE', ( #24194, #33828, #7924, #14054 ) ) ;
#33077=DIRECTION ( 'NONE',  ( -0.000000000000000000, -0.000000000000000000, 1.000000000000000000 ) ) ;
#33078=DIRECTION ( 'NONE',  ( 1.000000000000000000, 0.000000000000000000, 0.000000000000000000 ) ) ;
#33079=CARTESIAN_POINT ( 'NONE',  ( -43.00000337463112743, -60.62177826491080168, 12.50000000000000000 ) ) ;
#33083=EDGE_LOOP ( 'NONE', ( #866, #34456, #13977, #12137 ) ) ;
#33084=EDGE_CURVE ( 'NONE', #23027, #25033, #9428, .T. ) ;
#33086=CYLINDRICAL_SURFACE ( 'NONE', #31615, 2.000000000000000000 ) ;
#33087=EDGE_LOOP ( 'NONE', ( #33154, #34275, #37059, #9091 ) ) ;
#33088=DIRECTION ( 'NONE',  ( 0.000000000000000000, 0.000000000000000000, 1.000000000000000000 ) ) ;
#33090=CYLINDRICAL_SURFACE ( 'NONE', #23716, 1.999999999999998224 ) ;
#33091=VERTEX_POINT ( 'NONE', #786 ) ;
#33092=CIRCLE ( 'NONE', #11537, 2.000000000000001776 ) ;
#33094=VERTEX_POINT ( 'NONE', #25936 ) ;
#33095=FACE_OUTER_BOUND ( 'NONE', #10463, .T. ) ;
#33096=CYLINDRICAL_SURFACE ( 'NONE', #33358, 1.999999999999998224 ) ;
#33097=DIRECTION ( 'NONE',  ( 1.000000000000000000, 0.000000000000000000, 0.000000000000000000 ) ) ;
#33098=DIRECTION ( 'NONE',  ( 1.000000000000000000, 0.000000000000000000, 0.000000000000000000 ) ) ;
#33099=EDGE_LOOP ( 'NONE', ( #4801, #9600, #27079, #6158 ) ) ;
#33100=DIRECTION ( 'NONE',  ( 1.000000000000000000, 0.000000000000000000, 0.000000000000000000 ) ) ;
#33101=EDGE_CURVE ( 'NONE', #23066, #1626, #23747, .T. ) ;
#33103=EDGE_CURVE ( 'NONE', #7750, #22308, #33331, .T. ) ;
#33105=FACE_OUTER_BOUND ( 'NONE', #75, .T. ) ;
#33106=AXIS2_PLACEMENT_3D ( 'NONE', #17823, #20819, #29055 ) ;
#33107=DIRECTION ( 'NONE',  ( 0.000000000000000000, 0.000000000000000000, 1.000000000000000000 ) ) ;
#33108=DIRECTION ( 'NONE',  ( 1.000000000000000000, 0.000000000000000000, 0.000000000000000000 ) ) ;
#33110=DIRECTION ( 'NONE',  ( 0.000000000000000000, 0.000000000000000000, 1.000000000000000000 ) ) ;
#33111=CARTESIAN_POINT ( 'NONE',  ( 4.279621169095998212, -62.97617850287780072, -49.86561046011506448 ) ) ;
#33112=CARTESIAN_POINT ( 'NONE',  ( 36.99999662536853862, 77.94228634059959404, 12.50000000000000000 ) ) ;
#33114=EDGE_LOOP ( 'NONE', ( #4965, #8220, #18636, #18657, #34231 ) ) ;
#33116=ORIENTED_EDGE ( 'NONE', *, *, #32220, .T. ) ;
#33117=DIRECTION ( 'NONE',  ( 0.000000000000000000, 0.000000000000000000, 1.000000000000000000 ) ) ;
#33118=CARTESIAN_POINT ( 'NONE',  ( -45.00000337463111322, 77.94228634059959404, -9.999999999999998224 ) ) ;
#33120=ORIENTED_EDGE ( 'NONE', *, *, #20497, .F. ) ;
#33121=EDGE_CURVE ( 'NONE', #15905, #9326, #8198, .T. ) ;
#33122=DIRECTION ( 'NONE',  ( 0.000000000000000000, 0.000000000000000000, 1.000000000000000000 ) ) ;
#33124=CARTESIAN_POINT ( 'NONE',  ( 34.99999662536855283, -77.94228634059960825, -5.000000000000000000 ) ) ;
#33125=AXIS2_PLACEMENT_3D ( 'NONE', #28565, #16949, #17494 ) ;
#33126=CARTESIAN_POINT ( 'NONE',  ( -73.90204618161054384, 6.988581222280664917, -5.000000000000000000 ) ) ;
#33127=ORIENTED_EDGE ( 'NONE', *, *, #26715, .F. ) ;
#33128=ORIENTED_EDGE ( 'NONE', *, *, #13642, .T. ) ;
#33131=DIRECTION ( 'NONE',  ( 0.000000000000000000, 0.000000000000000000, -1.000000000000000000 ) ) ;
#33132=ORIENTED_EDGE ( 'NONE', *, *, #28335, .T. ) ;
#33133=PLANE ( 'NONE',  #5975 ) ;
#33134=ORIENTED_EDGE ( 'NONE', *, *, #1079, .T. ) ;
#33135=CARTESIAN_POINT ( 'NONE',  ( -35.19434990244938888, 52.39915983220783602, -4.999999999999997335 ) ) ;
#33136=AXIS2_PLACEMENT_3D ( 'NONE', #2596, #17024, #16248 ) ;
#33137=DIRECTION ( 'NONE',  ( 1.000000000000000000, 0.000000000000000000, 0.000000000000000000 ) ) ;
#33138=ORIENTED_EDGE ( 'NONE', *, *, #5717, .T. ) ;
#33139=CIRCLE ( 'NONE', #27755, 2.000000000000001776 ) ;
#33140=EDGE_CURVE ( 'NONE', #12474, #20714, #27352, .T. ) ;
#33141=DIRECTION ( 'NONE',  ( -1.000000000000000000, 0.000000000000000000, 0.000000000000000000 ) ) ;
#33142=ORIENTED_EDGE ( 'NONE', *, *, #2765, .F. ) ;
#33144=VECTOR ( 'NONE', #29155, 1000.000000000000000 ) ;
#33145=CARTESIAN_POINT ( 'NONE',  ( 67.99999662536836809, -34.64101615137759183, 17.49999999999999645 ) ) ;
#33146=CARTESIAN_POINT ( 'NONE',  ( 1.999996625368710257, -69.28203230275519786, -9.999999999999998224 ) ) ;
#33147=DIRECTION ( 'NONE',  ( 0.000000000000000000, 0.000000000000000000, 1.000000000000000000 ) ) ;
#33148=VERTEX_POINT ( 'NONE', #29467 ) ;
#33149=DIRECTION ( 'NONE',  ( 0.5000000000000038858, 0.8660254037844363761, 0.000000000000000000 ) ) ;
#33150=EDGE_CURVE ( 'NONE', #8319, #4953, #28911, .T. ) ;
#33152=DIRECTION ( 'NONE',  ( -1.000000000000000000, 0.000000000000000000, 0.000000000000000000 ) ) ;
#33153=CARTESIAN_POINT ( 'NONE',  ( 31.02796211690949235, -59.29837256189548356, -4.999999999999997335 ) ) ;
#33154=ORIENTED_EDGE ( 'NONE', *, *, #20307, .F. ) ;
#33156=AXIS2_PLACEMENT_3D ( 'NONE', #23407, #4836, #21518 ) ;
#33157=EDGE_CURVE ( 'NONE', #4442, #15311, #5199, .T. ) ;
#33159=DIRECTION ( 'NONE',  ( 1.000000000000000000, 0.000000000000000000, 0.000000000000000000 ) ) ;
#33160=ORIENTED_EDGE ( 'NONE', *, *, #2164, .T. ) ;
#33163=VECTOR ( 'NONE', #4424, 1000.000000000000000 ) ;
#33164=CARTESIAN_POINT ( 'NONE',  ( -70.47608876694631874, -59.13646009116124702, 12.49999999999999822 ) ) ;
#33165=CIRCLE ( 'NONE', #833, 27.00000000000001421 ) ;
#33166=DIRECTION ( 'NONE',  ( 1.000000000000000000, 0.000000000000000000, 0.000000000000000000 ) ) ;
#33168=CARTESIAN_POINT ( 'NONE',  ( -69.13212189986965939, -2.778182860042805125, -4.999999999999997335 ) ) ;
#33169=DIRECTION ( 'NONE',  ( 1.000000000000000000, 0.000000000000000000, 0.000000000000000000 ) ) ;
#33174=CYLINDRICAL_SURFACE ( 'NONE', #169, 2.000000000000001776 ) ;
#33175=DIRECTION ( 'NONE',  ( 0.000000000000000000, 0.000000000000000000, 1.000000000000000000 ) ) ;
#33176=LINE ( 'NONE', #24754, #31076 ) ;
#33179=ADVANCED_FACE ( 'NONE', ( #21419, #21778, #26864, #30412, #18428, #30034, #23875 ), #12597, .F. ) ;
#33180=PLANE ( 'NONE',  #11732 ) ;
#33181=CARTESIAN_POINT ( 'NONE',  ( 56.67878100130369035, -27.78182860042797131, -4.999999999999997335 ) ) ;
#33182=AXIS2_PLACEMENT_3D ( 'NONE', #13984, #25260, #25429 ) ;
#33183=DIRECTION ( 'NONE',  ( 1.000000000000000000, 0.000000000000000000, 0.000000000000000000 ) ) ;
#33184=ORIENTED_EDGE ( 'NONE', *, *, #20128, .F. ) ;
#33185=ADVANCED_FACE ( 'NONE', ( #7179 ), #9975, .F. ) ;
#33186=DIRECTION ( 'NONE',  ( 0.000000000000000000, 0.000000000000000000, 1.000000000000000000 ) ) ;
#33188=DIRECTION ( 'NONE',  ( -1.000000000000000000, 0.000000000000000000, 0.000000000000000000 ) ) ;
#33189=AXIS2_PLACEMENT_3D ( 'NONE', #24030, #12177, #9397 ) ;
#33190=CARTESIAN_POINT ( 'NONE',  ( -82.00000337463094979, 17.32050807568878525, -9.999999999999998224 ) ) ;
#33195=DIRECTION ( 'NONE',  ( 1.000000000000000000, 0.000000000000000000, 0.000000000000000000 ) ) ;
#33196=EDGE_CURVE ( 'NONE', #30803, #8170, #20728, .T. ) ;
#33197=VERTEX_POINT ( 'NONE', #6782 ) ;
#33200=CARTESIAN_POINT ( 'NONE',  ( 76.99999662536835388, -25.98076211353319565, -5.000000000000000000 ) ) ;
#33201=AXIS2_PLACEMENT_3D ( 'NONE', #17993, #9163, #3369 ) ;
#33202=DIRECTION ( 'NONE',  ( 0.000000000000000000, 0.000000000000000000, 1.000000000000000000 ) ) ;
#33205=ORIENTED_EDGE ( 'NONE', *, *, #15246, .F. ) ;
#33207=CIRCLE ( 'NONE', #14037, 2.000000000000001776 ) ;
#33208=DIRECTION ( 'NONE',  ( 1.000000000000000000, 0.000000000000000000, 0.000000000000000000 ) ) ;
#33209=( LENGTH_UNIT ( ) NAMED_UNIT ( * ) SI_UNIT ( .MILLI., .METRE. ) );
#33211=DIRECTION ( 'NONE',  ( -1.000000000000000000, 0.000000000000000000, 0.000000000000000000 ) ) ;
#33212=DIRECTION ( 'NONE',  ( 0.000000000000000000, 0.000000000000000000, -1.000000000000000000 ) ) ;
#33213=AXIS2_PLACEMENT_3D ( 'NONE', #15722, #32585, #18725 ) ;
#33214=ORIENTED_EDGE ( 'NONE', *, *, #12561, .F. ) ;
#33215=AXIS2_PLACEMENT_3D ( 'NONE', #22691, #36747, #11046 ) ;
#33216=AXIS2_PLACEMENT_3D ( 'NONE', #19820, #13822, #37071 ) ;
#33219=AXIS2_PLACEMENT_3D ( 'NONE', #5540, #17165, #5371 ) ;
#33220=FACE_OUTER_BOUND ( 'NONE', #27604, .T. ) ;
#33222=EDGE_CURVE ( 'NONE', #10069, #34770, #2196, .T. ) ;
#33224=ORIENTED_EDGE ( 'NONE', *, *, #30723, .T. ) ;
#33225=EDGE_LOOP ( 'NONE', ( #32485, #25492 ) ) ;
#33226=ORIENTED_EDGE ( 'NONE', *, *, #10352, .T. ) ;
#33227=EDGE_CURVE ( 'NONE', #20954, #28688, #29649, .T. ) ;
#33229=CIRCLE ( 'NONE', #3280, 2.000000000000001776 ) ;
#33230=ORIENTED_EDGE ( 'NONE', *, *, #9420, .T. ) ;
#33231=CIRCLE ( 'NONE', #17642, 1.999999999999998224 ) ;
#33232=EDGE_CURVE ( 'NONE', #14569, #24516, #27939, .T. ) ;
#33233=CARTESIAN_POINT ( 'NONE',  ( 19.99999662536861678, -69.28203230275519786, 17.49999999999999645 ) ) ;
#33236=EDGE_LOOP ( 'NONE', ( #3814, #29103 ) ) ;
#33238=CARTESIAN_POINT ( 'NONE',  ( 0.000000000000000000, 0.000000000000000000, 12.49999999999999822 ) ) ;
#33239=CARTESIAN_POINT ( 'NONE',  ( 0.000000000000000000, 0.000000000000000000, -5.000000000000000000 ) ) ;
#33240=ORIENTED_EDGE ( 'NONE', *, *, #9994, .F. ) ;
#33242=DIRECTION ( 'NONE',  ( 1.000000000000000000, 0.000000000000000000, 0.000000000000000000 ) ) ;
#33243=CYLINDRICAL_SURFACE ( 'NONE', #27935, 2.000000000000001776 ) ;
#33244=ADVANCED_FACE ( 'NONE', ( #29855 ), #18791, .F. ) ;
#33245=CIRCLE ( 'NONE', #16465, 2.000000000000001776 ) ;
#33246=DIRECTION ( 'NONE',  ( 0.000000000000000000, 0.000000000000000000, 1.000000000000000000 ) ) ;
#33247=EDGE_CURVE ( 'NONE', #16797, #5699, #11757, .T. ) ;
#33248=CARTESIAN_POINT ( 'NONE',  ( -5.000003374631269537, -77.94228634059960825, 12.50000000000000000 ) ) ;
#33250=EDGE_LOOP ( 'NONE', ( #28961, #2409 ) ) ;
#33251=DIRECTION ( 'NONE',  ( 0.000000000000000000, 0.000000000000000000, 1.000000000000000000 ) ) ;
#33255=CARTESIAN_POINT ( 'NONE',  ( 24.99999662536859546, -77.94228634059960825, 17.49999999999999645 ) ) ;
#33256=DIRECTION ( 'NONE',  ( 0.000000000000000000, 0.000000000000000000, 1.000000000000000000 ) ) ;
#33257=DIRECTION ( 'NONE',  ( 1.000000000000000000, 0.000000000000000000, 0.000000000000000000 ) ) ;
#33259=DIRECTION ( 'NONE',  ( 1.000000000000000000, 0.000000000000000000, 0.000000000000000000 ) ) ;
#33263=CARTESIAN_POINT ( 'NONE',  ( -10.00000337463125000, -86.60254037844400443, 12.50000000000000000 ) ) ;
#33264=AXIS2_PLACEMENT_3D ( 'NONE', #28550, #31192, #13931 ) ;
#33265=DIRECTION ( 'NONE',  ( 1.000000000000000000, 0.000000000000000000, 0.000000000000000000 ) ) ;
#33267=AXIS2_PLACEMENT_3D ( 'NONE', #13535, #30978, #28169 ) ;
#33268=AXIS2_PLACEMENT_3D ( 'NONE', #29760, #18539, #4097 ) ;
#33269=ORIENTED_EDGE ( 'NONE', *, *, #11812, .F. ) ;
#33270=AXIS2_PLACEMENT_3D ( 'NONE', #4456, #7274, #7091 ) ;
#33271=VERTEX_POINT ( 'NONE', #9618 ) ;
#33272=ADVANCED_FACE ( 'NONE', ( #10346 ), #24220, .F. ) ;
#33273=ORIENTED_EDGE ( 'NONE', *, *, #215, .T. ) ;
#33274=CIRCLE ( 'NONE', #26680, 33.00000000000001421 ) ;
#33277=ORIENTED_EDGE ( 'NONE', *, *, #33421, .T. ) ;
#33279=CIRCLE ( 'NONE', #8731, 95.00000000000000000 ) ;
#33280=CARTESIAN_POINT ( 'NONE',  ( -4.279621169095561228, 62.97617850287782915, 12.49999999999999822 ) ) ;
#33282=ORIENTED_EDGE ( 'NONE', *, *, #25228, .F. ) ;
#33283=DIRECTION ( 'NONE',  ( -1.000000000000000000, 0.000000000000000000, 0.000000000000000000 ) ) ;
#33284=VERTEX_POINT ( 'NONE', #1734 ) ;
#33285=EDGE_CURVE ( 'NONE', #5530, #25623, #13167, .T. ) ;
#33286=FACE_OUTER_BOUND ( 'NONE', #11157, .T. ) ;
#33287=CARTESIAN_POINT ( 'NONE',  ( -40.00000337463113453, 69.28203230275516944, 12.50000000000000000 ) ) ;
#33288=FACE_OUTER_BOUND ( 'NONE', #30235, .T. ) ;
#33289=AXIS2_PLACEMENT_3D ( 'NONE', #14315, #17315, #5132 ) ;
#33290=DIRECTION ( 'NONE',  ( 1.000000000000000000, 0.000000000000000000, 0.000000000000000000 ) ) ;
#33291=CIRCLE ( 'NONE', #24924, 2.000000000000001776 ) ;
#33293=CARTESIAN_POINT ( 'NONE',  ( -56.67878100130369035, 27.78182860042797131, -49.86348611802629449 ) ) ;
#33295=AXIS2_PLACEMENT_3D ( 'NONE', #946, #9756, #758 ) ;
#33296=AXIS2_PLACEMENT_3D ( 'NONE', #19581, #7951, #28366 ) ;
#33298=ADVANCED_FACE ( 'NONE', ( #4743 ), #22339, .F. ) ;
#33299=DIRECTION ( 'NONE',  ( 0.000000000000000000, 0.000000000000000000, 1.000000000000000000 ) ) ;
#33300=VECTOR ( 'NONE', #24731, 1000.000000000000000 ) ;
#33302=VERTEX_POINT ( 'NONE', #28321 ) ;
#33303=CARTESIAN_POINT ( 'NONE',  ( 34.00000000000068923, 58.88972745734143643, -49.22241343995293761 ) ) ;
#33304=CARTESIAN_POINT ( 'NONE',  ( 14.80603122773119118, -87.83969979969866415, 12.49999999999999645 ) ) ;
#33306=ORIENTED_EDGE ( 'NONE', *, *, #15478, .F. ) ;
#33307=DIRECTION ( 'NONE',  ( 1.000000000000000000, 0.000000000000000000, 0.000000000000000000 ) ) ;
#33308=CIRCLE ( 'NONE', #4564, 2.000000000000001776 ) ;
#33309=DIRECTION ( 'NONE',  ( 1.000000000000000000, 0.000000000000000000, 0.000000000000000000 ) ) ;
#33310=DIRECTION ( 'NONE',  ( 3.469446951953612611E-15, 1.000000000000000000, 0.000000000000000000 ) ) ;
#33311=VECTOR ( 'NONE', #21333, 1000.000000000000000 ) ;
#33312=VERTEX_POINT ( 'NONE', #7733 ) ;
#33313=EDGE_LOOP ( 'NONE', ( #4728, #33778 ) ) ;
#33314=LINE ( 'NONE', #32950, #18361 ) ;
#33316=CIRCLE ( 'NONE', #6944, 2.000000000000001776 ) ;
#33317=CARTESIAN_POINT ( 'NONE',  ( 68.19434990244977257, -52.39915983220758022, -49.22241343995298024 ) ) ;
#33319=VERTEX_POINT ( 'NONE', #16899 ) ;
#33321=FACE_OUTER_BOUND ( 'NONE', #20670, .T. ) ;
#33324=DIRECTION ( 'NONE',  ( 0.000000000000000000, 0.000000000000000000, 1.000000000000000000 ) ) ;
#33325=CIRCLE ( 'NONE', #17159, 2.000000000000001776 ) ;
#33326=AXIS2_PLACEMENT_3D ( 'NONE', #19369, #8321, #13751 ) ;
#33328=CIRCLE ( 'NONE', #16548, 2.000000000000001776 ) ;
#33329=EDGE_CURVE ( 'NONE', #27967, #14230, #13722, .T. ) ;
#33330=ORIENTED_EDGE ( 'NONE', *, *, #3960, .T. ) ;
#33331=CIRCLE ( 'NONE', #23150, 33.00000000000001421 ) ;
#33332=VERTEX_POINT ( 'NONE', #16350 ) ;
#33333=CARTESIAN_POINT ( 'NONE',  ( -5.000003374631269537, -77.94228634059960825, -9.999999999999998224 ) ) ;
#33334=CIRCLE ( 'NONE', #11185, 2.000000000000001776 ) ;
#33335=LINE ( 'NONE', #13992, #21269 ) ;
#33336=VERTEX_POINT ( 'NONE', #13521 ) ;
#33338=VERTEX_POINT ( 'NONE', #33418 ) ;
#33340=AXIS2_PLACEMENT_3D ( 'NONE', #17686, #15242, #1001 ) ;
#33342=VERTEX_POINT ( 'NONE', #19346 ) ;
#33344=ORIENTED_EDGE ( 'NONE', *, *, #22291, .T. ) ;
#33348=CIRCLE ( 'NONE', #16593, 2.000000000000001776 ) ;
#33350=CARTESIAN_POINT ( 'NONE',  ( -8.000003374631287301, 69.28203230275516944, -9.999999999999998224 ) ) ;
#33352=ORIENTED_EDGE ( 'NONE', *, *, #2258, .F. ) ;
#33353=DIRECTION ( 'NONE',  ( -1.000000000000000000, 0.000000000000000000, 0.000000000000000000 ) ) ;
#33354=FACE_OUTER_BOUND ( 'NONE', #31121, .T. ) ;
#33355=LINE ( 'NONE', #12184, #14814 ) ;
#33356=DIRECTION ( 'NONE',  ( -0.000000000000000000, -0.000000000000000000, 1.000000000000000000 ) ) ;
#33358=AXIS2_PLACEMENT_3D ( 'NONE', #4807, #24115, #1415 ) ;
#33360=VECTOR ( 'NONE', #11164, 1000.000000000000000 ) ;
#33363=ORIENTED_EDGE ( 'NONE', *, *, #8399, .T. ) ;
#33364=DIRECTION ( 'NONE',  ( 0.000000000000000000, 0.000000000000000000, 1.000000000000000000 ) ) ;
#33365=FACE_OUTER_BOUND ( 'NONE', #25941, .T. ) ;
#33366=AXIS2_PLACEMENT_3D ( 'NONE', #19552, #33998, #10911 ) ;
#33367=DIRECTION ( 'NONE',  ( -1.000000000000000000, 0.000000000000000000, 0.000000000000000000 ) ) ;
#33368=CYLINDRICAL_SURFACE ( 'NONE', #9229, 2.000000000000001776 ) ;
#33369=DIRECTION ( 'NONE',  ( 0.000000000000000000, 0.000000000000000000, 1.000000000000000000 ) ) ;
#33373=ADVANCED_FACE ( 'NONE', ( #24983 ), #2475, .F. ) ;
#33375=VERTEX_POINT ( 'NONE', #36421 ) ;
#33376=CIRCLE ( 'NONE', #17207, 2.000000000000001776 ) ;
#33377=ORIENTED_EDGE ( 'NONE', *, *, #13517, .T. ) ;
#33379=DIRECTION ( 'NONE',  ( 0.000000000000000000, 0.000000000000000000, -1.000000000000000000 ) ) ;
#33380=CARTESIAN_POINT ( 'NONE',  ( -80.00000337463094979, -2.428612866367529932E-14, -9.999999999999998224 ) ) ;
#33381=DIRECTION ( 'NONE',  ( 0.000000000000000000, 0.000000000000000000, 1.000000000000000000 ) ) ;
#33382=ORIENTED_EDGE ( 'NONE', *, *, #35810, .T. ) ;
#33385=DIRECTION ( 'NONE',  ( 1.000000000000000000, 0.000000000000000000, 0.000000000000000000 ) ) ;
#33386=AXIS2_PLACEMENT_3D ( 'NONE', #11145, #17347, #22594 ) ;
#33389=ORIENTED_EDGE ( 'NONE', *, *, #19467, .F. ) ;
#33392=CIRCLE ( 'NONE', #23194, 65.00000000000000000 ) ;
#33393=FILL_AREA_STYLE_COLOUR ( '', #6353 ) ;
#33394=CARTESIAN_POINT ( 'NONE',  ( 81.86307328356784296, -18.04779437809804321, 12.50000000000000000 ) ) ;
#33397=ADVANCED_FACE ( 'NONE', ( #36970 ), #19722, .F. ) ;
#33398=ORIENTED_EDGE ( 'NONE', *, *, #2572, .T. ) ;
#33399=ORIENTED_EDGE ( 'NONE', *, *, #23802, .F. ) ;
#33400=AXIS2_PLACEMENT_3D ( 'NONE', #9282, #5745, #3292 ) ;
#33401=AXIS2_PLACEMENT_3D ( 'NONE', #34197, #6050, #20461 ) ;
#33402=AXIS2_PLACEMENT_3D ( 'NONE', #33417, #4742, #24789 ) ;
#33403=ORIENTED_EDGE ( 'NONE', *, *, #23113, .T. ) ;
#33404=CARTESIAN_POINT ( 'NONE',  ( -67.00000337463102085, 43.30127018922198801, 12.50000000000000000 ) ) ;
#33405=DIRECTION ( 'NONE',  ( 0.000000000000000000, 0.000000000000000000, 1.000000000000000000 ) ) ;
#33406=CARTESIAN_POINT ( 'NONE',  ( -45.00000337463112743, -60.62177826491080168, -5.000000000000000000 ) ) ;
#33407=CARTESIAN_POINT ( 'NONE',  ( -42.00000337463114164, -69.28203230275519786, -5.000000000000000000 ) ) ;
#33408=DIRECTION ( 'NONE',  ( 0.000000000000000000, 0.000000000000000000, 1.000000000000000000 ) ) ;
#33410=CYLINDRICAL_SURFACE ( 'NONE', #17704, 2.000000000000001776 ) ;
#33413=CARTESIAN_POINT ( 'NONE',  ( 67.99999662536838230, 17.32050807568879236, 12.50000000000000000 ) ) ;
#33414=EDGE_CURVE ( 'NONE', #5018, #33284, #14153, .T. ) ;
#33415=CARTESIAN_POINT ( 'NONE',  ( -15.00000337463126066, 77.94228634059957983, -9.999999999999998224 ) ) ;
#33416=ORIENTED_EDGE ( 'NONE', *, *, #13799, .T. ) ;
#33417=CARTESIAN_POINT ( 'NONE',  ( 44.99999662536849598, 60.62177826491077326, 12.50000000000000000 ) ) ;
#33418=CARTESIAN_POINT ( 'NONE',  ( -33.00000337463116296, -60.62177826491080168, -9.999999999999998224 ) ) ;
#33419=AXIS2_PLACEMENT_3D ( 'NONE', #36080, #1213, #10377 ) ;
#33420=ORIENTED_EDGE ( 'NONE', *, *, #34396, .T. ) ;
#33421=EDGE_CURVE ( 'NONE', #10270, #30265, #12970, .T. ) ;
#33422=ORIENTED_EDGE ( 'NONE', *, *, #36750, .F. ) ;
#33423=AXIS2_PLACEMENT_3D ( 'NONE', #4521, #9956, #1330 ) ;
#33424=FACE_OUTER_BOUND ( 'NONE', #2897, .T. ) ;
#33428=ORIENTED_EDGE ( 'NONE', *, *, #23763, .F. ) ;
#33431=CIRCLE ( 'NONE', #14259, 2.000000000000001776 ) ;
#33432=VERTEX_POINT ( 'NONE', #5472 ) ;
#33433=CIRCLE ( 'NONE', #34640, 2.000000000000001776 ) ;
#33434=CARTESIAN_POINT ( 'NONE',  ( -35.00000337463116296, 77.94228634059957983, -5.000000000000000000 ) ) ;
#33435=EDGE_CURVE ( 'NONE', #13680, #3339, #35744, .T. ) ;
#33436=VECTOR ( 'NONE', #3931, 1000.000000000000000 ) ;
#33438=CARTESIAN_POINT ( 'NONE',  ( -45.00000337463111322, 77.94228634059959404, -9.999999999999998224 ) ) ;
#33439=ORIENTED_EDGE ( 'NONE', *, *, #34909, .F. ) ;
#33440=ORIENTED_EDGE ( 'NONE', *, *, #4592, .F. ) ;
#33441=VECTOR ( 'NONE', #30621, 1000.000000000000000 ) ;
#33442=DIRECTION ( 'NONE',  ( 0.000000000000000000, 0.000000000000000000, 1.000000000000000000 ) ) ;
#33443=LINE ( 'NONE', #1754, #17079 ) ;
#33445=VERTEX_POINT ( 'NONE', #27602 ) ;
#33446=CARTESIAN_POINT ( 'NONE',  ( 95.00000000000000000, 1.163414459189985643E-14, 12.49999999999999822 ) ) ;
#33447=AXIS2_PLACEMENT_3D ( 'NONE', #31088, #5771, #5417 ) ;
#33450=DIRECTION ( 'NONE',  ( 1.000000000000000000, 0.000000000000000000, 0.000000000000000000 ) ) ;
#33451=EDGE_CURVE ( 'NONE', #5475, #21277, #24361, .T. ) ;
#33452=EDGE_LOOP ( 'NONE', ( #19095, #3634 ) ) ;
#33453=CARTESIAN_POINT ( 'NONE',  ( -65.00000337463104927, -25.98076211353322051, -9.999999999999998224 ) ) ;
#33454=AXIS2_PLACEMENT_3D ( 'NONE', #19158, #16333, #22319 ) ;
#33455=FACE_BOUND ( 'NONE', #31552, .T. ) ;
#33456=CIRCLE ( 'NONE', #26834, 1.999999999999998224 ) ;
#33457=CARTESIAN_POINT ( 'NONE',  ( 79.99999662536833966, -3.469446951953614189E-15, -9.999999999999998224 ) ) ;
#33458=DIRECTION ( 'NONE',  ( 0.000000000000000000, 0.000000000000000000, -1.000000000000000000 ) ) ;
#33459=DIRECTION ( 'NONE',  ( 1.000000000000000000, 0.000000000000000000, 0.000000000000000000 ) ) ;
#33460=DIRECTION ( 'NONE',  ( 1.000000000000000000, 0.000000000000000000, 0.000000000000000000 ) ) ;
#33461=AXIS2_PLACEMENT_3D ( 'NONE', #655, #15088, #2932 ) ;
#33462=EDGE_CURVE ( 'NONE', #10417, #35979, #17761, .T. ) ;
#33464=CIRCLE ( 'NONE', #17872, 2.000000000000001776 ) ;
#33465=ADVANCED_FACE ( 'NONE', ( #17448 ), #6027, .F. ) ;
#33466=CARTESIAN_POINT ( 'NONE',  ( 33.21453428580180400, -78.84346569788027637, 12.50000000000000000 ) ) ;
#33468=CARTESIAN_POINT ( 'NONE',  ( 69.99999662536839651, 34.64101615137758472, -9.999999999999998224 ) ) ;
#33469=ADVANCED_FACE ( 'NONE', ( #14453 ), #23624, .F. ) ;
#33471=CARTESIAN_POINT ( 'NONE',  ( 67.99999662536838230, -3.224517592124143893E-15, -9.999999999999998224 ) ) ;
#33473=ORIENTED_EDGE ( 'NONE', *, *, #347, .F. ) ;
#33475=VECTOR ( 'NONE', #18251, 1000.000000000000000 ) ;
#33477=ORIENTED_EDGE ( 'NONE', *, *, #32957, .T. ) ;
#33479=DIRECTION ( 'NONE',  ( 0.000000000000000000, 0.000000000000000000, 1.000000000000000000 ) ) ;
#33480=VERTEX_POINT ( 'NONE', #32246 ) ;
#33482=CARTESIAN_POINT ( 'NONE',  ( -15.00000337463125710, -77.94228634059960825, -5.000000000000000000 ) ) ;
#33483=ADVANCED_FACE ( 'NONE', ( #29251 ), #5838, .F. ) ;
#33484=CIRCLE ( 'NONE', #16112, 33.00000000000001421 ) ;
#33485=CARTESIAN_POINT ( 'NONE',  ( -78.00000337463094979, 17.32050807568878525, -9.999999999999998224 ) ) ;
#33486=ORIENTED_EDGE ( 'NONE', *, *, #9337, .F. ) ;
#33487=FACE_OUTER_BOUND ( 'NONE', #2797, .T. ) ;
#33489=AXIS2_PLACEMENT_3D ( 'NONE', #818, #18070, #15252 ) ;
#33490=FACE_BOUND ( 'NONE', #19000, .T. ) ;
#33491=CYLINDRICAL_SURFACE ( 'NONE', #12394, 2.000000000000001776 ) ;
#33492=CYLINDRICAL_SURFACE ( 'NONE', #21526, 2.000000000000000000 ) ;
#33493=AXIS2_PLACEMENT_3D ( 'NONE', #22038, #36100, #10400 ) ;
#33494=CARTESIAN_POINT ( 'NONE',  ( 7.999996625368625658, 86.60254037844397601, -9.999999999999998224 ) ) ;
#33495=ORIENTED_EDGE ( 'NONE', *, *, #34866, .F. ) ;
#33501=AXIS2_PLACEMENT_3D ( 'NONE', #13646, #36537, #19110 ) ;
#33503=ORIENTED_EDGE ( 'NONE', *, *, #28832, .F. ) ;
#33504=DIRECTION ( 'NONE',  ( 0.000000000000000000, 0.000000000000000000, 1.000000000000000000 ) ) ;
#33506=VERTEX_POINT ( 'NONE', #184 ) ;
#33507=EDGE_CURVE ( 'NONE', #8634, #598, #8825, .T. ) ;
#33508=CARTESIAN_POINT ( 'NONE',  ( -80.00000337463094979, 17.32050807568878525, 17.49999999999999645 ) ) ;
#33509=DIRECTION ( 'NONE',  ( 1.000000000000000000, 0.000000000000000000, 0.000000000000000000 ) ) ;
#33510=DIRECTION ( 'NONE',  ( 0.000000000000000000, 0.000000000000000000, -1.000000000000000000 ) ) ;
#33511=ADVANCED_FACE ( 'NONE', ( #12159 ), #6375, .F. ) ;
#33513=ORIENTED_EDGE ( 'NONE', *, *, #7559, .F. ) ;
#33514=CIRCLE ( 'NONE', #11361, 2.000000000000001776 ) ;
#33515=ORIENTED_EDGE ( 'NONE', *, *, #23625, .T. ) ;
#33516=EDGE_CURVE ( 'NONE', #15574, #31133, #27966, .T. ) ;
#33518=LINE ( 'NONE', #4993, #1602 ) ;
#33519=DIRECTION ( 'NONE',  ( -1.000000000000000000, 0.000000000000000000, 0.000000000000000000 ) ) ;
#33520=EDGE_CURVE ( 'NONE', #13843, #26293, #31693, .T. ) ;
#33521=DIRECTION ( 'NONE',  ( -1.000000000000000000, 0.000000000000000000, 0.000000000000000000 ) ) ;
#33522=ORIENTED_EDGE ( 'NONE', *, *, #17202, .T. ) ;
#33523=ORIENTED_EDGE ( 'NONE', *, *, #3048, .F. ) ;
#33524=DIRECTION ( 'NONE',  ( -0.000000000000000000, -0.000000000000000000, 1.000000000000000000 ) ) ;
#33525=DIRECTION ( 'NONE',  ( 0.000000000000000000, 0.000000000000000000, 1.000000000000000000 ) ) ;
#33526=CARTESIAN_POINT ( 'NONE',  ( 67.99999662536838230, -3.224517592124143893E-15, -5.000000000000000000 ) ) ;
#33527=CIRCLE ( 'NONE', #1181, 2.000000000000001776 ) ;
#33528=CARTESIAN_POINT ( 'NONE',  ( -87.00000337463093558, -8.660254037844422825, -9.999999999999998224 ) ) ;
#33529=EDGE_CURVE ( 'NONE', #35441, #28925, #2223, .T. ) ;
#33530=VERTEX_POINT ( 'NONE', #17279 ) ;
#33531=ADVANCED_FACE ( 'NONE', ( #31854 ), #11807, .F. ) ;
#33532=ORIENTED_EDGE ( 'NONE', *, *, #18390, .T. ) ;
#33533=DIRECTION ( 'NONE',  ( 1.000000000000000000, 0.000000000000000000, 0.000000000000000000 ) ) ;
#33534=CIRCLE ( 'NONE', #25155, 2.000000000000001776 ) ;
#33535=ADVANCED_FACE ( 'NONE', ( #6187 ), #747, .F. ) ;
#33536=CARTESIAN_POINT ( 'NONE',  ( 19.99999662536857770, 86.60254037844397601, -9.999999999999998224 ) ) ;
#33537=EDGE_LOOP ( 'NONE', ( #7537, #28030 ) ) ;
#33539=DIRECTION ( 'NONE',  ( 0.000000000000000000, 0.000000000000000000, 1.000000000000000000 ) ) ;
#33540=EDGE_LOOP ( 'NONE', ( #5608, #7118, #6577, #28643 ) ) ;
#33541=CYLINDRICAL_SURFACE ( 'NONE', #15336, 2.000000000000001776 ) ;
#33542=CIRCLE ( 'NONE', #28137, 2.000000000000001776 ) ;
#33543=CARTESIAN_POINT ( 'NONE',  ( 14.99999662536859901, 77.94228634059957983, -5.000000000000000000 ) ) ;
#33544=CIRCLE ( 'NONE', #10782, 2.000000000000001776 ) ;
#33545=AXIS2_PLACEMENT_3D ( 'NONE', #20545, #18305, #26198 ) ;
#33546=DIRECTION ( 'NONE',  ( 0.000000000000000000, 0.000000000000000000, 1.000000000000000000 ) ) ;
#33547=ORIENTED_EDGE ( 'NONE', *, *, #2470, .F. ) ;
#33549=CARTESIAN_POINT ( 'NONE',  ( 56.67878100130369035, -27.78182860042797131, -4.999999999999997335 ) ) ;
#33550=DIRECTION ( 'NONE',  ( -1.000000000000000000, 0.000000000000000000, 0.000000000000000000 ) ) ;
#33552=ORIENTED_EDGE ( 'NONE', *, *, #932, .T. ) ;
#33553=CARTESIAN_POINT ( 'NONE',  ( 74.99999662536835388, -25.98076211353319565, 12.50000000000000000 ) ) ;
#33554=DIRECTION ( 'NONE',  ( 0.000000000000000000, 0.000000000000000000, 1.000000000000000000 ) ) ;
#33556=AXIS2_PLACEMENT_3D ( 'NONE', #24494, #16049, #21487 ) ;
#33557=ORIENTED_EDGE ( 'NONE', *, *, #13552, .F. ) ;
#33558=ORIENTED_EDGE ( 'NONE', *, *, #2444, .F. ) ;
#33560=CYLINDRICAL_SURFACE ( 'NONE', #3623, 3.000000000000002665 ) ;
#33561=ORIENTED_EDGE ( 'NONE', *, *, #29115, .T. ) ;
#33562=CARTESIAN_POINT ( 'NONE',  ( -15.00000337463126066, 77.94228634059957983, -5.000000000000000000 ) ) ;
#33563=CIRCLE ( 'NONE', #23384, 2.000000000000001776 ) ;
#33564=CYLINDRICAL_SURFACE ( 'NONE', #12385, 2.000000000000000000 ) ;
#33565=FACE_OUTER_BOUND ( 'NONE', #23209, .T. ) ;
#33566=AXIS2_PLACEMENT_3D ( 'NONE', #9707, #32568, #7643 ) ;
#33567=CARTESIAN_POINT ( 'NONE',  ( 21.99999662536862033, -86.60254037844400443, 12.50000000000000000 ) ) ;
#33568=DIRECTION ( 'NONE',  ( 0.000000000000000000, 0.000000000000000000, 1.000000000000000000 ) ) ;
#33569=DIRECTION ( 'NONE',  ( 1.000000000000000000, 0.000000000000000000, 0.000000000000000000 ) ) ;
#33570=DIRECTION ( 'NONE',  ( 1.000000000000000000, 0.000000000000000000, 0.000000000000000000 ) ) ;
#33571=FACE_OUTER_BOUND ( 'NONE', #27369, .T. ) ;
#33572=ORIENTED_EDGE ( 'NONE', *, *, #12081, .T. ) ;
#33573=ORIENTED_EDGE ( 'NONE', *, *, #11291, .T. ) ;
#33575=CARTESIAN_POINT ( 'NONE',  ( 36.99999662536855283, 60.62177826491078747, 12.50000000000000000 ) ) ;
#33577=LINE ( 'NONE', #30370, #17436 ) ;
#33578=CIRCLE ( 'NONE', #11396, 27.00000000000001421 ) ;
#33579=CARTESIAN_POINT ( 'NONE',  ( -67.00000337463106348, -60.62177826491083010, -9.999999999999998224 ) ) ;
#33582=CYLINDRICAL_SURFACE ( 'NONE', #13791, 27.00000000000001066 ) ;
#33583=ORIENTED_EDGE ( 'NONE', *, *, #25679, .F. ) ;
#33584=VECTOR ( 'NONE', #28151, 1000.000000000000000 ) ;
#33585=DIRECTION ( 'NONE',  ( 0.000000000000000000, 0.000000000000000000, 1.000000000000000000 ) ) ;
#33586=EDGE_LOOP ( 'NONE', ( #35477, #2739 ) ) ;
#33587=SURFACE_STYLE_USAGE ( .BOTH. , #33013 ) ;
#33588=CARTESIAN_POINT ( 'NONE',  ( 32.99999662536855283, -60.62177826491080168, -9.999999999999998224 ) ) ;
#33590=DIRECTION ( 'NONE',  ( 0.8660254037844347108, -0.5000000000000067724, 0.000000000000000000 ) ) ;
#33591=ORIENTED_EDGE ( 'NONE', *, *, #34659, .T. ) ;
#33592=ORIENTED_EDGE ( 'NONE', *, *, #19474, .F. ) ;
#33594=EDGE_CURVE ( 'NONE', #7804, #30855, #11993, .T. ) ;
#33595=VERTEX_POINT ( 'NONE', #24181 ) ;
#33596=DIRECTION ( 'NONE',  ( 1.000000000000000000, 0.000000000000000000, 0.000000000000000000 ) ) ;
#33597=CARTESIAN_POINT ( 'NONE',  ( -37.00000337463117717, -77.94228634059963667, -5.000000000000000000 ) ) ;
#33598=DIRECTION ( 'NONE',  ( 0.000000000000000000, 0.000000000000000000, 1.000000000000000000 ) ) ;
#33599=FACE_OUTER_BOUND ( 'NONE', #24546, .T. ) ;
#33601=VERTEX_POINT ( 'NONE', #35278 ) ;
#33602=DIRECTION ( 'NONE',  ( 1.000000000000000000, 0.000000000000000000, 0.000000000000000000 ) ) ;
#33603=DIRECTION ( 'NONE',  ( -1.000000000000000000, 0.000000000000000000, 0.000000000000000000 ) ) ;
#33605=CIRCLE ( 'NONE', #21009, 2.000000000000001776 ) ;
#33606=DIRECTION ( 'NONE',  ( 1.000000000000000000, 0.000000000000000000, 0.000000000000000000 ) ) ;
#33607=ORIENTED_EDGE ( 'NONE', *, *, #13537, .F. ) ;
#33608=FACE_OUTER_BOUND ( 'NONE', #16122, .T. ) ;
#33609=CARTESIAN_POINT ( 'NONE',  ( -15.97563234535668109, 90.60231327712331506, 12.49999999999999822 ) ) ;
#33610=VERTEX_POINT ( 'NONE', #35828 ) ;
#33611=ORIENTED_EDGE ( 'NONE', *, *, #9099, .F. ) ;
#33612=FACE_OUTER_BOUND ( 'NONE', #18059, .T. ) ;
#33613=CARTESIAN_POINT ( 'NONE',  ( 27.99999662536855993, 69.28203230275518365, -9.999999999999998224 ) ) ;
#33614=EDGE_CURVE ( 'NONE', #8438, #30579, #17788, .T. ) ;
#33617=ORIENTED_EDGE ( 'NONE', *, *, #37060, .T. ) ;
#33618=ORIENTED_EDGE ( 'NONE', *, *, #25633, .T. ) ;
#33619=DIRECTION ( 'NONE',  ( 0.000000000000000000, 0.000000000000000000, 1.000000000000000000 ) ) ;
#33620=ORIENTED_EDGE ( 'NONE', *, *, #28920, .F. ) ;
#33621=AXIS2_PLACEMENT_3D ( 'NONE', #11998, #26444, #32618 ) ;
#33622=CARTESIAN_POINT ( 'NONE',  ( 32.99999662536855283, -77.94228634059960825, 17.49999999999999645 ) ) ;
#33623=ORIENTED_EDGE ( 'NONE', *, *, #16271, .T. ) ;
#33624=ORIENTED_EDGE ( 'NONE', *, *, #34537, .T. ) ;
#33625=DIRECTION ( 'NONE',  ( -1.000000000000000000, 0.000000000000000000, 0.000000000000000000 ) ) ;
#33626=EDGE_CURVE ( 'NONE', #28925, #31383, #29431, .T. ) ;
#33627=DIRECTION ( 'NONE',  ( 1.000000000000000000, 0.000000000000000000, 0.000000000000000000 ) ) ;
#33628=EDGE_LOOP ( 'NONE', ( #7843, #17564 ) ) ;
#33629=EDGE_LOOP ( 'NONE', ( #1448, #10686, #1740, #19876 ) ) ;
#33630=CARTESIAN_POINT ( 'NONE',  ( 49.99999662536848177, -51.96152422706640550, 17.49999999999999645 ) ) ;
#33631=FACE_OUTER_BOUND ( 'NONE', #31199, .T. ) ;
#33632=CARTESIAN_POINT ( 'NONE',  ( -40.00000337463113453, -69.28203230275519786, -9.999999999999998224 ) ) ;
#33633=DIRECTION ( 'NONE',  ( 0.000000000000000000, 0.000000000000000000, 1.000000000000000000 ) ) ;
#33634=ORIENTED_EDGE ( 'NONE', *, *, #14498, .F. ) ;
#33635=DIRECTION ( 'NONE',  ( 1.000000000000000000, 0.000000000000000000, 0.000000000000000000 ) ) ;
#33638=FACE_BOUND ( 'NONE', #2224, .T. ) ;
#33640=FACE_OUTER_BOUND ( 'NONE', #15452, .T. ) ;
#33642=DIRECTION ( 'NONE',  ( 1.000000000000000000, 0.000000000000000000, 0.000000000000000000 ) ) ;
#33645=ADVANCED_FACE ( 'NONE', ( #6575 ), #21372, .F. ) ;
#33646=CARTESIAN_POINT ( 'NONE',  ( 61.99999662536845335, 34.64101615137759893, -9.999999999999998224 ) ) ;
#33647=ORIENTED_EDGE ( 'NONE', *, *, #9265, .F. ) ;
#33649=AXIS2_PLACEMENT_3D ( 'NONE', #21187, #29056, #26624 ) ;
#33650=DIRECTION ( 'NONE',  ( 0.000000000000000000, 0.000000000000000000, 1.000000000000000000 ) ) ;
#33651=CARTESIAN_POINT ( 'NONE',  ( -78.00000337463096400, -34.64101615137762025, 12.50000000000000000 ) ) ;
#33653=EDGE_LOOP ( 'NONE', ( #9516, #31200, #10404, #26302, #22941, #797 ) ) ;
#33654=VERTEX_POINT ( 'NONE', #6744 ) ;
#33655=DIRECTION ( 'NONE',  ( -1.000000000000000000, 0.000000000000000000, 0.000000000000000000 ) ) ;
#33656=CARTESIAN_POINT ( 'NONE',  ( -85.00000337463092137, 25.98076211353317433, 12.50000000000000000 ) ) ;
#33658=CARTESIAN_POINT ( 'NONE',  ( -77.00000337463097821, -8.660254037844422825, 17.49999999999999645 ) ) ;
#33659=ADVANCED_FACE ( 'NONE', ( #32815 ), #21003, .F. ) ;
#33661=ORIENTED_EDGE ( 'NONE', *, *, #419, .F. ) ;
#33662=DIRECTION ( 'NONE',  ( 0.000000000000000000, 0.000000000000000000, 1.000000000000000000 ) ) ;
#33663=VERTEX_POINT ( 'NONE', #21570 ) ;
#33664=DIRECTION ( 'NONE',  ( 0.000000000000000000, 0.000000000000000000, 1.000000000000000000 ) ) ;
#33665=EDGE_CURVE ( 'NONE', #32142, #8319, #21977, .T. ) ;
#33666=DIRECTION ( 'NONE',  ( 0.000000000000000000, 0.000000000000000000, -1.000000000000000000 ) ) ;
#33667=CARTESIAN_POINT ( 'NONE',  ( -10.00000337463125000, -86.60254037844400443, -9.999999999999998224 ) ) ;
#33670=ORIENTED_EDGE ( 'NONE', *, *, #27718, .F. ) ;
#33671=CARTESIAN_POINT ( 'NONE',  ( -12.00000337463127842, -69.28203230275519786, 12.50000000000000000 ) ) ;
#33672=DIRECTION ( 'NONE',  ( 0.000000000000000000, 0.000000000000000000, 1.000000000000000000 ) ) ;
#33673=CARTESIAN_POINT ( 'NONE',  ( -58.00000337463108480, -51.96152422706641971, 12.50000000000000000 ) ) ;
#33674=ORIENTED_EDGE ( 'NONE', *, *, #14932, .F. ) ;
#33675=CYLINDRICAL_SURFACE ( 'NONE', #23367, 2.000000000000001776 ) ;
#33676=DIRECTION ( 'NONE',  ( 1.000000000000000000, 0.000000000000000000, 0.000000000000000000 ) ) ;
#33677=ORIENTED_EDGE ( 'NONE', *, *, #17151, .F. ) ;
#33679=CARTESIAN_POINT ( 'NONE',  ( 24.99999662536859546, -77.94228634059960825, -5.000000000000000000 ) ) ;
#33680=FACE_OUTER_BOUND ( 'NONE', #25982, .T. ) ;
#33681=DIRECTION ( 'NONE',  ( 1.000000000000000000, 0.000000000000000000, 0.000000000000000000 ) ) ;
#33682=CIRCLE ( 'NONE', #17498, 2.000000000000001776 ) ;
#33684=VERTEX_POINT ( 'NONE', #36010 ) ;
#33685=EDGE_CURVE ( 'NONE', #34111, #5560, #32612, .T. ) ;
#33686=EDGE_LOOP ( 'NONE', ( #32645, #14053, #20974, #32225 ) ) ;
#33688=DIRECTION ( 'NONE',  ( 0.000000000000000000, 0.000000000000000000, -1.000000000000000000 ) ) ;
#33689=DIRECTION ( 'NONE',  ( 0.000000000000000000, 0.000000000000000000, 1.000000000000000000 ) ) ;
#33691=ORIENTED_EDGE ( 'NONE', *, *, #7457, .T. ) ;
#33692=AXIS2_PLACEMENT_3D ( 'NONE', #16890, #33964, #31145 ) ;
#33693=PLANE ( 'NONE',  #8004 ) ;
#33696=ORIENTED_EDGE ( 'NONE', *, *, #37042, .F. ) ;
#33697=EDGE_LOOP ( 'NONE', ( #7989, #12785, #32518, #12267 ) ) ;
#33698=DIRECTION ( 'NONE',  ( 0.000000000000000000, 0.000000000000000000, 1.000000000000000000 ) ) ;
#33699=EDGE_CURVE ( 'NONE', #15126, #33094, #18747, .T. ) ;
#33701=EDGE_LOOP ( 'NONE', ( #3257, #6344, #18265, #18855, #26412, #25094, #14343, #20694, #7049 ) ) ;
#33702=EDGE_CURVE ( 'NONE', #1764, #26494, #26764, .T. ) ;
#33703=FACE_OUTER_BOUND ( 'NONE', #31476, .T. ) ;
#33704=EDGE_LOOP ( 'NONE', ( #24239, #12063, #12995, #2350 ) ) ;
#33705=FACE_BOUND ( 'NONE', #24454, .T. ) ;
#33707=CIRCLE ( 'NONE', #17527, 3.000000000000002665 ) ;
#33708=CYLINDRICAL_SURFACE ( 'NONE', #16715, 2.000000000000001776 ) ;
#33709=EDGE_CURVE ( 'NONE', #4217, #5741, #21736, .T. ) ;
#33711=ORIENTED_EDGE ( 'NONE', *, *, #20335, .T. ) ;
#33713=EDGE_CURVE ( 'NONE', #21017, #19227, #36360, .T. ) ;
#33715=CARTESIAN_POINT ( 'NONE',  ( -35.19434990244938888, 52.39915983220783602, -4.999999999999997335 ) ) ;
#33717=DIRECTION ( 'NONE',  ( -0.000000000000000000, 0.000000000000000000, -1.000000000000000000 ) ) ;
#33718=CARTESIAN_POINT ( 'NONE',  ( 19.99999662536861678, -86.60254037844400443, -9.999999999999998224 ) ) ;
#33719=EDGE_LOOP ( 'NONE', ( #33981, #2315 ) ) ;
#33720=VECTOR ( 'NONE', #16943, 1000.000000000000000 ) ;
#33721=CARTESIAN_POINT ( 'NONE',  ( -73.00000337463097821, 43.30127018922197379, -5.000000000000000000 ) ) ;
#33722=DIRECTION ( 'NONE',  ( 0.000000000000000000, 0.000000000000000000, -1.000000000000000000 ) ) ;
#33723=DIRECTION ( 'NONE',  ( 0.000000000000000000, 0.000000000000000000, -1.000000000000000000 ) ) ;
#33724=EDGE_CURVE ( 'NONE', #29503, #7561, #26618, .T. ) ;
#33725=EDGE_CURVE ( 'NONE', #13179, #20167, #10007, .T. ) ;
#33726=ORIENTED_EDGE ( 'NONE', *, *, #12341, .F. ) ;
#33730=DIRECTION ( 'NONE',  ( -0.000000000000000000, -0.000000000000000000, 1.000000000000000000 ) ) ;
#33731=ORIENTED_EDGE ( 'NONE', *, *, #31274, .T. ) ;
#33733=CARTESIAN_POINT ( 'NONE',  ( -65.00000337463102085, 43.30127018922198801, -5.000000000000000000 ) ) ;
#33735=FACE_OUTER_BOUND ( 'NONE', #14678, .T. ) ;
#33736=AXIS2_PLACEMENT_3D ( 'NONE', #29212, #28833, #25686 ) ;
#33738=CARTESIAN_POINT ( 'NONE',  ( -22.00000337463124112, 69.28203230275516944, 17.49999999999999645 ) ) ;
#33739=CYLINDRICAL_SURFACE ( 'NONE', #9503, 2.000000000000001776 ) ;
#33740=CARTESIAN_POINT ( 'NONE',  ( 81.86307328356785717, -18.04779437809804676, -5.000000000000000000 ) ) ;
#33742=CARTESIAN_POINT ( 'NONE',  ( -75.00000337463100664, -43.30127018922202353, -9.999999999999998224 ) ) ;
#33743=ORIENTED_EDGE ( 'NONE', *, *, #27502, .F. ) ;
#33744=ORIENTED_EDGE ( 'NONE', *, *, #27, .T. ) ;
#33746=AXIS2_PLACEMENT_3D ( 'NONE', #7176, #26305, #35493 ) ;
#33747=LINE ( 'NONE', #11037, #24741 ) ;
#33748=CYLINDRICAL_SURFACE ( 'NONE', #10861, 2.000000000000000000 ) ;
#33749=CARTESIAN_POINT ( 'NONE',  ( -78.00000337463094979, -2.428612866367529932E-14, -9.999999999999998224 ) ) ;
#33751=CYLINDRICAL_SURFACE ( 'NONE', #26366, 2.000000000000001776 ) ;
#33755=AXIS2_PLACEMENT_3D ( 'NONE', #3793, #15795, #628 ) ;
#33756=VERTEX_POINT ( 'NONE', #36375 ) ;
#33757=CARTESIAN_POINT ( 'NONE',  ( 19.99999662536861678, -69.28203230275519786, -5.000000000000000000 ) ) ;
#33759=CARTESIAN_POINT ( 'NONE',  ( 0.000000000000000000, 0.000000000000000000, -5.000000000000000000 ) ) ;
#33761=EDGE_LOOP ( 'NONE', ( #22895, #23962 ) ) ;
#33764=ORIENTED_EDGE ( 'NONE', *, *, #15522, .F. ) ;
#33767=CARTESIAN_POINT ( 'NONE',  ( 72.99999662536836809, -8.660254037844401509, -5.000000000000000000 ) ) ;
#33769=EDGE_CURVE ( 'NONE', #15901, #10971, #8226, .T. ) ;
#33770=LINE ( 'NONE', #19519, #35945 ) ;
#33771=CARTESIAN_POINT ( 'NONE',  ( -77.00000337463097821, -8.660254037844422825, -9.999999999999998224 ) ) ;
#33772=DIRECTION ( 'NONE',  ( 0.000000000000000000, 0.000000000000000000, 1.000000000000000000 ) ) ;
#33773=CARTESIAN_POINT ( 'NONE',  ( 32.99999662536855283, -77.94228634059960825, -9.999999999999998224 ) ) ;
#33775=DIRECTION ( 'NONE',  ( 0.000000000000000000, 0.000000000000000000, 1.000000000000000000 ) ) ;
#33776=DIRECTION ( 'NONE',  ( -0.000000000000000000, -0.000000000000000000, -1.000000000000000000 ) ) ;
#33778=ORIENTED_EDGE ( 'NONE', *, *, #16747, .T. ) ;
#33779=DIRECTION ( 'NONE',  ( 0.000000000000000000, -0.000000000000000000, -1.000000000000000000 ) ) ;
#33780=CARTESIAN_POINT ( 'NONE',  ( -35.19434990244938888, 52.39915983220783602, -49.22241343995295892 ) ) ;
#33781=ORIENTED_EDGE ( 'NONE', *, *, #24113, .T. ) ;
#33782=VECTOR ( 'NONE', #7835, 1000.000000000000000 ) ;
#33783=ORIENTED_EDGE ( 'NONE', *, *, #33157, .T. ) ;
#33784=CARTESIAN_POINT ( 'NONE',  ( 76.99999662536835388, -43.30127018922199511, -9.999999999999998224 ) ) ;
#33785=DIRECTION ( 'NONE',  ( 0.8660254037844415942, 0.4999999999999949485, 0.000000000000000000 ) ) ;
#33786=CARTESIAN_POINT ( 'NONE',  ( -68.00000000000000000, 0.000000000000000000, -49.86348611802629449 ) ) ;
#33790=EDGE_CURVE ( 'NONE', #22817, #24238, #13677, .T. ) ;
#33791=CIRCLE ( 'NONE', #27186, 2.000000000000001776 ) ;
#33792=FACE_BOUND ( 'NONE', #17543, .T. ) ;
#33794=EDGE_LOOP ( 'NONE', ( #9935, #36134, #35884, #3986, #35606 ) ) ;
#33797=ORIENTED_EDGE ( 'NONE', *, *, #8150, .T. ) ;
#33799=DIRECTION ( 'NONE',  ( 1.000000000000000000, 0.000000000000000000, 0.000000000000000000 ) ) ;
#33800=LINE ( 'NONE', #8317, #36427 ) ;
#33801=VERTEX_POINT ( 'NONE', #13473 ) ;
#33802=VECTOR ( 'NONE', #3915, 1000.000000000000000 ) ;
#33803=VERTEX_POINT ( 'NONE', #33168 ) ;
#33804=DIRECTION ( 'NONE',  ( 1.000000000000000000, 0.000000000000000000, 0.000000000000000000 ) ) ;
#33805=CARTESIAN_POINT ( 'NONE',  ( 17.99999662536858125, 86.60254037844397601, -9.999999999999998224 ) ) ;
#33806=CARTESIAN_POINT ( 'NONE',  ( -37.00000337463116296, -60.62177826491080168, -9.999999999999998224 ) ) ;
#33808=CIRCLE ( 'NONE', #15218, 3.000000000000002665 ) ;
#33809=EDGE_LOOP ( 'NONE', ( #1923, #29839, #14055, #3977, #4203, #16901 ) ) ;
#33810=CYLINDRICAL_SURFACE ( 'NONE', #18349, 2.000000000000001776 ) ;
#33812=FACE_BOUND ( 'NONE', #22315, .T. ) ;
#33813=DIRECTION ( 'NONE',  ( 0.000000000000000000, 0.000000000000000000, 1.000000000000000000 ) ) ;
#33814=FACE_OUTER_BOUND ( 'NONE', #1782, .T. ) ;
#33815=DIRECTION ( 'NONE',  ( -1.000000000000000000, 0.000000000000000000, 0.000000000000000000 ) ) ;
#33816=CARTESIAN_POINT ( 'NONE',  ( 79.99999662536833966, -3.469446951953614189E-15, 17.49999999999999645 ) ) ;
#33818=AXIS2_PLACEMENT_3D ( 'NONE', #35607, #29969, #1457 ) ;
#33819=DIRECTION ( 'NONE',  ( 0.000000000000000000, 0.000000000000000000, 1.000000000000000000 ) ) ;
#33820=CIRCLE ( 'NONE', #17631, 2.000000000000000000 ) ;
#33822=EDGE_LOOP ( 'NONE', ( #16449, #5536 ) ) ;
#33824=CARTESIAN_POINT ( 'NONE',  ( 62.97617850287784336, 4.279621169095339184, 12.49999999999999822 ) ) ;
#33825=DIRECTION ( 'NONE',  ( -1.000000000000000000, 0.000000000000000000, 0.000000000000000000 ) ) ;
#33827=ORIENTED_EDGE ( 'NONE', *, *, #33725, .T. ) ;
#33828=ORIENTED_EDGE ( 'NONE', *, *, #9178, .T. ) ;
#33830=EDGE_CURVE ( 'NONE', #14157, #28556, #13623, .T. ) ;
#33831=FACE_OUTER_BOUND ( 'NONE', #25356, .T. ) ;
#33833=AXIS2_PLACEMENT_3D ( 'NONE', #19977, #23163, #2548 ) ;
#33834=ORIENTED_EDGE ( 'NONE', *, *, #10098, .F. ) ;
#33835=ADVANCED_FACE ( 'NONE', ( #7489 ), #7687, .F. ) ;
#33836=AXIS2_PLACEMENT_3D ( 'NONE', #26442, #23453, #6939 ) ;
#33837=CARTESIAN_POINT ( 'NONE',  ( 37.99999662536853151, -69.28203230275519786, -9.999999999999998224 ) ) ;
#33839=CARTESIAN_POINT ( 'NONE',  ( -75.00000337463099243, -25.98076211353322051, -9.999999999999998224 ) ) ;
#33840=EDGE_CURVE ( 'NONE', #15693, #12600, #445, .T. ) ;
#33842=DIRECTION ( 'NONE',  ( 0.000000000000000000, 0.000000000000000000, 1.000000000000000000 ) ) ;
#33843=AXIS2_PLACEMENT_3D ( 'NONE', #25657, #24909, #8018 ) ;
#33844=AXIS2_PLACEMENT_3D ( 'NONE', #6638, #12431, #23343 ) ;
#33847=CARTESIAN_POINT ( 'NONE',  ( 46.99999662536849598, 60.62177826491077326, 12.50000000000000000 ) ) ;
#33848=ORIENTED_EDGE ( 'NONE', *, *, #1611, .F. ) ;
#33849=CARTESIAN_POINT ( 'NONE',  ( -85.00000337463092137, -8.660254037844422825, -9.999999999999998224 ) ) ;
#33850=DIRECTION ( 'NONE',  ( -1.000000000000000000, 0.000000000000000000, 0.000000000000000000 ) ) ;
#33851=CARTESIAN_POINT ( 'NONE',  ( 46.99999662536851019, 77.94228634059959404, -5.000000000000000000 ) ) ;
#33852=ORIENTED_EDGE ( 'NONE', *, *, #6392, .T. ) ;
#33853=DIRECTION ( 'NONE',  ( 0.000000000000000000, -0.000000000000000000, -1.000000000000000000 ) ) ;
#33854=DIRECTION ( 'NONE',  ( 0.000000000000000000, 0.000000000000000000, -1.000000000000000000 ) ) ;
#33856=EDGE_CURVE ( 'NONE', #22350, #24339, #30405, .T. ) ;
#33857=DIRECTION ( 'NONE',  ( 0.000000000000000000, 0.000000000000000000, -1.000000000000000000 ) ) ;
#33859=DIRECTION ( 'NONE',  ( 0.000000000000000000, 0.000000000000000000, -1.000000000000000000 ) ) ;
#33860=CARTESIAN_POINT ( 'NONE',  ( 0.000000000000000000, 0.000000000000000000, -5.000000000000000000 ) ) ;
#33861=VECTOR ( 'NONE', #18998, 1000.000000000000000 ) ;
#33863=FACE_OUTER_BOUND ( 'NONE', #20780, .T. ) ;
#33866=ORIENTED_EDGE ( 'NONE', *, *, #24016, .T. ) ;
#33867=ORIENTED_EDGE ( 'NONE', *, *, #31286, .T. ) ;
#33869=CIRCLE ( 'NONE', #11682, 33.00000000000001421 ) ;
#33870=DIRECTION ( 'NONE',  ( 0.000000000000000000, 0.000000000000000000, 1.000000000000000000 ) ) ;
#33871=AXIS2_PLACEMENT_3D ( 'NONE', #24864, #36303, #10612 ) ;
#33872=EDGE_CURVE ( 'NONE', #7967, #23429, #32787, .T. ) ;
#33873=ORIENTED_EDGE ( 'NONE', *, *, #22291, .F. ) ;
#33874=ORIENTED_EDGE ( 'NONE', *, *, #19544, .T. ) ;
#33877=DIRECTION ( 'NONE',  ( -0.000000000000000000, -0.000000000000000000, -1.000000000000000000 ) ) ;
#33878=CYLINDRICAL_SURFACE ( 'NONE', #881, 2.000000000000001776 ) ;
#33880=EDGE_CURVE ( 'NONE', #25896, #30809, #22126, .T. ) ;
#33882=CARTESIAN_POINT ( 'NONE',  ( -56.13646009116099123, 70.47608876694653190, -49.22241343995295892 ) ) ;
#33883=CIRCLE ( 'NONE', #17698, 2.000000000000000000 ) ;
#33884=CARTESIAN_POINT ( 'NONE',  ( -75.00000337463097821, 8.660254037844374864, -9.999999999999998224 ) ) ;
#33885=EDGE_LOOP ( 'NONE', ( #13789, #21910 ) ) ;
#33886=AXIS2_PLACEMENT_3D ( 'NONE', #17441, #15178, #14448 ) ;
#33888=EDGE_CURVE ( 'NONE', #20625, #14287, #17818, .T. ) ;
#33890=FACE_BOUND ( 'NONE', #7224, .T. ) ;
#33891=CIRCLE ( 'NONE', #24928, 2.000000000000001776 ) ;
#33892=VECTOR ( 'NONE', #22220, 1000.000000000000000 ) ;
#33893=AXIS2_PLACEMENT_3D ( 'NONE', #32770, #30128, #2005 ) ;
#33894=EDGE_CURVE ( 'NONE', #29300, #19586, #18422, .T. ) ;
#33896=VERTEX_POINT ( 'NONE', #9136 ) ;
#33898=AXIS2_PLACEMENT_3D ( 'NONE', #7455, #27694, #30692 ) ;
#33899=DIRECTION ( 'NONE',  ( 1.000000000000000000, 0.000000000000000000, 0.000000000000000000 ) ) ;
#33900=DIRECTION ( 'NONE',  ( 0.4999999999999919509, -0.8660254037844432595, 0.000000000000000000 ) ) ;
#33901=CARTESIAN_POINT ( 'NONE',  ( 95.00000000000001421, 0.000000000000000000, -10.00000000000000000 ) ) ;
#33903=CARTESIAN_POINT ( 'NONE',  ( 37.27962116909601065, -62.97617850287780072, -4.999999999999997335 ) ) ;
#33904=FACE_OUTER_BOUND ( 'NONE', #27744, .T. ) ;
#33905=DIRECTION ( 'NONE',  ( 0.000000000000000000, 0.000000000000000000, 1.000000000000000000 ) ) ;
#33906=EDGE_LOOP ( 'NONE', ( #3088, #36413, #4406, #10221 ) ) ;
#33908=ORIENTED_EDGE ( 'NONE', *, *, #34071, .T. ) ;
#33909=AXIS2_PLACEMENT_3D ( 'NONE', #26105, #34753, #32077 ) ;
#33910=DIRECTION ( 'NONE',  ( 0.000000000000000000, 0.000000000000000000, -1.000000000000000000 ) ) ;
#33911=ORIENTED_EDGE ( 'NONE', *, *, #4256, .T. ) ;
#33913=DIRECTION ( 'NONE',  ( 0.000000000000000000, 0.000000000000000000, 1.000000000000000000 ) ) ;
#33915=CARTESIAN_POINT ( 'NONE',  ( 16.99999662536863454, -77.94228634059960825, -5.000000000000000000 ) ) ;
#33917=ADVANCED_FACE ( 'NONE', ( #23219 ), #17027, .F. ) ;
#33918=CIRCLE ( 'NONE', #21323, 2.000000000000001776 ) ;
#33919=DIRECTION ( 'NONE',  ( 1.000000000000000000, 0.000000000000000000, 0.000000000000000000 ) ) ;
#33920=CYLINDRICAL_SURFACE ( 'NONE', #17053, 2.000000000000001776 ) ;
#33921=ADVANCED_FACE ( 'NONE', ( #31649 ), #14771, .F. ) ;
#33924=EDGE_CURVE ( 'NONE', #31223, #29568, #2848, .T. ) ;
#33926=DIRECTION ( 'NONE',  ( 0.000000000000000000, 0.000000000000000000, -1.000000000000000000 ) ) ;
#33927=EDGE_LOOP ( 'NONE', ( #8960, #34428, #11959, #6189 ) ) ;
#33928=VECTOR ( 'NONE', #31565, 1000.000000000000000 ) ;
#33930=CARTESIAN_POINT ( 'NONE',  ( -18.00000337463123756, -69.28203230275522628, -9.999999999999998224 ) ) ;
#33931=DIRECTION ( 'NONE',  ( 0.000000000000000000, 0.000000000000000000, 1.000000000000000000 ) ) ;
#33932=CARTESIAN_POINT ( 'NONE',  ( 19.99999662536858835, 69.28203230275516944, -5.000000000000000000 ) ) ;
#33933=CARTESIAN_POINT ( 'NONE',  ( 24.99999662536859546, -77.94228634059960825, -9.999999999999998224 ) ) ;
#33934=VERTEX_POINT ( 'NONE', #25680 ) ;
#33936=VECTOR ( 'NONE', #20845, 1000.000000000000000 ) ;
#33937=EDGE_CURVE ( 'NONE', #15730, #31817, #36998, .T. ) ;
#33938=CIRCLE ( 'NONE', #5805, 2.000000000000001776 ) ;
#33939=FACE_BOUND ( 'NONE', #12395, .T. ) ;
#33940=ORIENTED_EDGE ( 'NONE', *, *, #3236, .F. ) ;
#33941=ORIENTED_EDGE ( 'NONE', *, *, #34196, .T. ) ;
#33943=CARTESIAN_POINT ( 'NONE',  ( -15.97563234535668109, 90.60231327712331506, -49.86561046011506448 ) ) ;
#33944=ORIENTED_EDGE ( 'NONE', *, *, #6554, .T. ) ;
#33945=AXIS2_PLACEMENT_3D ( 'NONE', #34744, #14305, #11836 ) ;
#33947=AXIS2_PLACEMENT_3D ( 'NONE', #19983, #31405, #13620 ) ;
#33948=DIRECTION ( 'NONE',  ( 0.000000000000000000, 0.000000000000000000, 1.000000000000000000 ) ) ;
#33949=AXIS2_PLACEMENT_3D ( 'NONE', #1912, #24790, #36223 ) ;
#33950=PLANE ( 'NONE',  #3244 ) ;
#33951=AXIS2_PLACEMENT_3D ( 'NONE', #33860, #16074, #24874 ) ;
#33954=ORIENTED_EDGE ( 'NONE', *, *, #33451, .F. ) ;
#33955=ORIENTED_EDGE ( 'NONE', *, *, #27943, .T. ) ;
#33956=CIRCLE ( 'NONE', #4026, 2.000000000000001776 ) ;
#33957=ORIENTED_EDGE ( 'NONE', *, *, #27873, .F. ) ;
#33958=EDGE_CURVE ( 'NONE', #30809, #9993, #23798, .T. ) ;
#33959=ORIENTED_EDGE ( 'NONE', *, *, #642, .T. ) ;
#33961=DIRECTION ( 'NONE',  ( 1.000000000000000000, 0.000000000000000000, 0.000000000000000000 ) ) ;
#33962=ADVANCED_FACE ( 'NONE', ( #33354 ), #28460, .F. ) ;
#33963=DIRECTION ( 'NONE',  ( 0.000000000000000000, 0.000000000000000000, 1.000000000000000000 ) ) ;
#33964=DIRECTION ( 'NONE',  ( 0.000000000000000000, 0.000000000000000000, 1.000000000000000000 ) ) ;
#33965=DIRECTION ( 'NONE',  ( 1.000000000000000000, 0.000000000000000000, 0.000000000000000000 ) ) ;
#33966=VECTOR ( 'NONE', #17376, 1000.000000000000000 ) ;
#33967=ORIENTED_EDGE ( 'NONE', *, *, #28451, .T. ) ;
#33968=DIRECTION ( 'NONE',  ( 0.000000000000000000, 0.000000000000000000, 1.000000000000000000 ) ) ;
#33969=CIRCLE ( 'NONE', #36964, 2.000000000000001776 ) ;
#33971=AXIS2_PLACEMENT_3D ( 'NONE', #836, #18088, #9485 ) ;
#33972=AXIS2_PLACEMENT_3D ( 'NONE', #30984, #28338, #5316 ) ;
#33974=ORIENTED_EDGE ( 'NONE', *, *, #18253, .F. ) ;
#33976=EDGE_CURVE ( 'NONE', #29874, #25059, #29776, .T. ) ;
#33977=DIRECTION ( 'NONE',  ( -0.000000000000000000, -0.000000000000000000, 1.000000000000000000 ) ) ;
#33978=DIRECTION ( 'NONE',  ( 0.000000000000000000, 0.000000000000000000, 1.000000000000000000 ) ) ;
#33980=AXIS2_PLACEMENT_3D ( 'NONE', #29996, #18008, #15185 ) ;
#33981=ORIENTED_EDGE ( 'NONE', *, *, #27672, .T. ) ;
#33983=CYLINDRICAL_SURFACE ( 'NONE', #9871, 2.000000000000001776 ) ;
#33985=CARTESIAN_POINT ( 'NONE',  ( -20.00000337463124112, 69.28203230275516944, -9.999999999999998224 ) ) ;
#33986=DIRECTION ( 'NONE',  ( 1.000000000000000000, 0.000000000000000000, 0.000000000000000000 ) ) ;
#33987=ORIENTED_EDGE ( 'NONE', *, *, #1219, .T. ) ;
#33988=VERTEX_POINT ( 'NONE', #17575 ) ;
#33989=EDGE_CURVE ( 'NONE', #29105, #32624, #16044, .T. ) ;
#33994=AXIS2_PLACEMENT_3D ( 'NONE', #4195, #32101, #15623 ) ;
#33995=ORIENTED_EDGE ( 'NONE', *, *, #9882, .T. ) ;
#33997=AXIS2_PLACEMENT_3D ( 'NONE', #7023, #7386, #16023 ) ;
#33998=DIRECTION ( 'NONE',  ( 0.000000000000000000, 0.000000000000000000, 1.000000000000000000 ) ) ;
#33999=ORIENTED_EDGE ( 'NONE', *, *, #9041, .T. ) ;
#34000=AXIS2_PLACEMENT_3D ( 'NONE', #27707, #2024, #23653 ) ;
#34001=ORIENTED_EDGE ( 'NONE', *, *, #15653, .T. ) ;
#34002=DIRECTION ( 'NONE',  ( 0.000000000000000000, 0.000000000000000000, 1.000000000000000000 ) ) ;
#34003=CIRCLE ( 'NONE', #33402, 2.000000000000001776 ) ;
#34004=DIRECTION ( 'NONE',  ( 3.491481338843133355E-15, 1.000000000000000000, 0.000000000000000000 ) ) ;
#34005=ORIENTED_EDGE ( 'NONE', *, *, #16403, .F. ) ;
#34006=VERTEX_POINT ( 'NONE', #31988 ) ;
#34007=CARTESIAN_POINT ( 'NONE',  ( -65.00000337463102085, 25.98076211353317433, -9.999999999999998224 ) ) ;
#34008=DIRECTION ( 'NONE',  ( 0.000000000000000000, 0.000000000000000000, 1.000000000000000000 ) ) ;
#34009=CARTESIAN_POINT ( 'NONE',  ( 34.99999662536855283, -77.94228634059960825, 12.50000000000000000 ) ) ;
#34010=CARTESIAN_POINT ( 'NONE',  ( -77.00000337463099243, -25.98076211353322051, -9.999999999999998224 ) ) ;
#34011=AXIS2_PLACEMENT_3D ( 'NONE', #31176, #25007, #33625 ) ;
#34012=ORIENTED_EDGE ( 'NONE', *, *, #13537, .T. ) ;
#34013=LINE ( 'NONE', #17114, #34518 ) ;
#34014=FACE_BOUND ( 'NONE', #22093, .T. ) ;
#34015=CARTESIAN_POINT ( 'NONE',  ( 49.99999662536848177, -51.96152422706640550, -9.999999999999998224 ) ) ;
#34017=AXIS2_PLACEMENT_3D ( 'NONE', #27071, #24083, #21077 ) ;
#34018=CARTESIAN_POINT ( 'NONE',  ( 86.45172111230354517, -31.46585318596159553, 12.49999999999999822 ) ) ;
#34020=CARTESIAN_POINT ( 'NONE',  ( 84.99999662536832545, 25.98076211353319565, -9.999999999999998224 ) ) ;
#34022=DIRECTION ( 'NONE',  ( 1.000000000000000000, 0.000000000000000000, 0.000000000000000000 ) ) ;
#34024=DIRECTION ( 'NONE',  ( 0.000000000000000000, 0.000000000000000000, 1.000000000000000000 ) ) ;
#34026=DIRECTION ( 'NONE',  ( 0.000000000000000000, 0.000000000000000000, 1.000000000000000000 ) ) ;
#34027=CIRCLE ( 'NONE', #9473, 2.000000000000001776 ) ;
#34028=CARTESIAN_POINT ( 'NONE',  ( -40.00000337463113453, -69.28203230275519786, 12.50000000000000000 ) ) ;
#34029=CARTESIAN_POINT ( 'NONE',  ( 4.999996625368676284, -77.94228634059960825, 17.49999999999999645 ) ) ;
#34030=AXIS2_PLACEMENT_3D ( 'NONE', #8955, #9307, #20549 ) ;
#34031=VERTEX_POINT ( 'NONE', #25851 ) ;
#34032=ORIENTED_EDGE ( 'NONE', *, *, #30016, .F. ) ;
#34033=ORIENTED_EDGE ( 'NONE', *, *, #10024, .F. ) ;
#34034=AXIS2_PLACEMENT_3D ( 'NONE', #35670, #21611, #7353 ) ;
#34036=DIRECTION ( 'NONE',  ( 0.000000000000000000, 0.000000000000000000, -1.000000000000000000 ) ) ;
#34037=EDGE_LOOP ( 'NONE', ( #5544, #32881, #19112, #12029 ) ) ;
#34038=AXIS2_PLACEMENT_3D ( 'NONE', #30986, #5115, #33799 ) ;
#34039=CYLINDRICAL_SURFACE ( 'NONE', #26897, 2.000000000000001776 ) ;
#34040=VERTEX_POINT ( 'NONE', #14968 ) ;
#34041=EDGE_CURVE ( 'NONE', #9761, #32663, #14824, .T. ) ;
#34043=ORIENTED_EDGE ( 'NONE', *, *, #32627, .T. ) ;
#34044=DIRECTION ( 'NONE',  ( 0.000000000000000000, 0.000000000000000000, -1.000000000000000000 ) ) ;
#34045=AXIS2_PLACEMENT_3D ( 'NONE', #30150, #10665, #15911 ) ;
#34047=DIRECTION ( 'NONE',  ( 0.000000000000000000, 0.000000000000000000, 1.000000000000000000 ) ) ;
#34049=CIRCLE ( 'NONE', #23240, 2.000000000000001776 ) ;
#34051=DIRECTION ( 'NONE',  ( 1.000000000000000000, 0.000000000000000000, 0.000000000000000000 ) ) ;
#34052=AXIS2_PLACEMENT_3D ( 'NONE', #6734, #22832, #8756 ) ;
#34053=CIRCLE ( 'NONE', #3507, 1.999999999999998224 ) ;
#34054=CYLINDRICAL_SURFACE ( 'NONE', #2737, 2.000000000000001776 ) ;
#34056=CIRCLE ( 'NONE', #18501, 2.000000000000001776 ) ;
#34057=ORIENTED_EDGE ( 'NONE', *, *, #18175, .F. ) ;
#34058=CARTESIAN_POINT ( 'NONE',  ( -75.00000337463099243, -25.98076211353322051, -9.999999999999998224 ) ) ;
#34062=DIRECTION ( 'NONE',  ( -1.000000000000000000, 0.000000000000000000, -0.000000000000000000 ) ) ;
#34063=DIRECTION ( 'NONE',  ( 0.000000000000000000, 0.000000000000000000, 1.000000000000000000 ) ) ;
#34064=EDGE_CURVE ( 'NONE', #30348, #5113, #19015, .T. ) ;
#34065=CIRCLE ( 'NONE', #30463, 2.000000000000001776 ) ;
#34066=ADVANCED_FACE ( 'NONE', ( #11570 ), #8780, .F. ) ;
#34068=CIRCLE ( 'NONE', #13089, 2.000000000000001776 ) ;
#34069=ORIENTED_EDGE ( 'NONE', *, *, #8740, .T. ) ;
#34070=ORIENTED_EDGE ( 'NONE', *, *, #1988, .T. ) ;
#34071=EDGE_CURVE ( 'NONE', #23292, #12699, #3459, .T. ) ;
#34073=DIRECTION ( 'NONE',  ( 0.000000000000000000, 0.000000000000000000, 1.000000000000000000 ) ) ;
#34074=ADVANCED_FACE ( 'NONE', ( #32914 ), #16227, .F. ) ;
#34075=ORIENTED_EDGE ( 'NONE', *, *, #5044, .T. ) ;
#34076=ORIENTED_EDGE ( 'NONE', *, *, #13882, .T. ) ;
#34077=CIRCLE ( 'NONE', #13099, 2.000000000000001776 ) ;
#34078=DIRECTION ( 'NONE',  ( 0.000000000000000000, 0.000000000000000000, -1.000000000000000000 ) ) ;
#34079=CARTESIAN_POINT ( 'NONE',  ( -70.00000337463099243, 51.96152422706637708, -5.000000000000000000 ) ) ;
#34080=VECTOR ( 'NONE', #4212, 1000.000000000000000 ) ;
#34081=DIRECTION ( 'NONE',  ( 0.000000000000000000, 0.000000000000000000, 1.000000000000000000 ) ) ;
#34082=EDGE_LOOP ( 'NONE', ( #29005, #18845, #20747, #3115, #27679, #11805 ) ) ;
#34083=VERTEX_POINT ( 'NONE', #27645 ) ;
#34084=CYLINDRICAL_SURFACE ( 'NONE', #3926, 2.000000000000001776 ) ;
#34085=CARTESIAN_POINT ( 'NONE',  ( -35.00000337463116296, -60.62177826491080168, -9.999999999999998224 ) ) ;
#34086=VERTEX_POINT ( 'NONE', #19045 ) ;
#34087=AXIS2_PLACEMENT_3D ( 'NONE', #36828, #10949, #10787 ) ;
#34088=EDGE_CURVE ( 'NONE', #8936, #7710, #4672, .T. ) ;
#34089=DIRECTION ( 'NONE',  ( 0.000000000000000000, 0.000000000000000000, 1.000000000000000000 ) ) ;
#34091=FACE_BOUND ( 'NONE', #17080, .T. ) ;
#34092=CIRCLE ( 'NONE', #35297, 2.000000000000001776 ) ;
#34093=AXIS2_PLACEMENT_3D ( 'NONE', #1278, #5016, #16451 ) ;
#34094=CARTESIAN_POINT ( 'NONE',  ( -5.000003374631269537, -77.94228634059960825, -9.999999999999998224 ) ) ;
#34095=VECTOR ( 'NONE', #20166, 1000.000000000000000 ) ;
#34096=ORIENTED_EDGE ( 'NONE', *, *, #3033, .T. ) ;
#34098=CARTESIAN_POINT ( 'NONE',  ( -3.000003374631269981, -77.94228634059960825, -9.999999999999998224 ) ) ;
#34099=AXIS2_PLACEMENT_3D ( 'NONE', #18557, #4473, #1108 ) ;
#34100=DIRECTION ( 'NONE',  ( 0.8660254037844413721, 0.4999999999999950595, 0.000000000000000000 ) ) ;
#34101=CARTESIAN_POINT ( 'NONE',  ( -75.00000337463097821, 25.98076211353318854, -5.000000000000000000 ) ) ;
#34102=EDGE_CURVE ( 'NONE', #32493, #5473, #11809, .T. ) ;
#34103=ORIENTED_EDGE ( 'NONE', *, *, #25651, .F. ) ;
#34106=CYLINDRICAL_SURFACE ( 'NONE', #14261, 2.000000000000000000 ) ;
#34108=ORIENTED_EDGE ( 'NONE', *, *, #36428, .F. ) ;
#34109=ORIENTED_EDGE ( 'NONE', *, *, #1709, .T. ) ;
#34111=VERTEX_POINT ( 'NONE', #35728 ) ;
#34113=DIRECTION ( 'NONE',  ( 0.000000000000000000, 0.000000000000000000, 1.000000000000000000 ) ) ;
#34114=CARTESIAN_POINT ( 'NONE',  ( 3.499999999999991562, 55.00000000000000000, -10.00000000000000000 ) ) ;
#34115=CIRCLE ( 'NONE', #37105, 2.000000000000001776 ) ;
#34116=FACE_BOUND ( 'NONE', #35662, .T. ) ;
#34117=AXIS2_PLACEMENT_3D ( 'NONE', #9851, #29726, #35563 ) ;
#34118=EDGE_CURVE ( 'NONE', #34784, #17325, #18666, .T. ) ;
#34120=CIRCLE ( 'NONE', #29305, 2.000000000000001776 ) ;
#34122=CARTESIAN_POINT ( 'NONE',  ( -15.00000337463125710, -77.94228634059960825, -9.999999999999998224 ) ) ;
#34125=ORIENTED_EDGE ( 'NONE', *, *, #8493, .F. ) ;
#34126=ORIENTED_EDGE ( 'NONE', *, *, #35419, .T. ) ;
#34127=LINE ( 'NONE', #11575, #31998 ) ;
#34128=AXIS2_PLACEMENT_3D ( 'NONE', #27294, #13055, #23757 ) ;
#34129=CARTESIAN_POINT ( 'NONE',  ( -83.00000337463092137, 8.660254037844389075, 12.50000000000000000 ) ) ;
#34130=DIRECTION ( 'NONE',  ( 0.000000000000000000, 0.000000000000000000, 1.000000000000000000 ) ) ;
#34131=CARTESIAN_POINT ( 'NONE',  ( 4.279621169095998212, -62.97617850287780072, -4.999999999999997335 ) ) ;
#34133=AXIS2_PLACEMENT_3D ( 'NONE', #8405, #23006, #5965 ) ;
#34135=FACE_BOUND ( 'NONE', #840, .T. ) ;
#34136=EDGE_LOOP ( 'NONE', ( #36385, #14073, #25291, #11423, #12018 ) ) ;
#34137=ORIENTED_EDGE ( 'NONE', *, *, #7736, .T. ) ;
#34139=ORIENTED_EDGE ( 'NONE', *, *, #10867, .T. ) ;
#34141=DIRECTION ( 'NONE',  ( 1.000000000000000000, 0.000000000000000000, 0.000000000000000000 ) ) ;
#34143=DIRECTION ( 'NONE',  ( 1.000000000000000000, 0.000000000000000000, 0.000000000000000000 ) ) ;
#34144=CIRCLE ( 'NONE', #2934, 2.000000000000001776 ) ;
#34145=DIRECTION ( 'NONE',  ( 1.000000000000000000, 0.000000000000000000, 0.000000000000000000 ) ) ;
#34147=CIRCLE ( 'NONE', #23354, 2.000000000000001776 ) ;
#34148=EDGE_LOOP ( 'NONE', ( #18392, #25428, #4302, #25946, #6095, #12110, #12013, #13305, #30941 ) ) ;
#34149=EDGE_LOOP ( 'NONE', ( #6998, #243, #16818 ) ) ;
#34151=VERTEX_POINT ( 'NONE', #21477 ) ;
#34154=CARTESIAN_POINT ( 'NONE',  ( 44.99999662536849598, -77.94228634059960825, -5.000000000000000000 ) ) ;
#34155=AXIS2_PLACEMENT_3D ( 'NONE', #8972, #35231, #6146 ) ;
#34157=CIRCLE ( 'NONE', #9344, 2.000000000000001776 ) ;
#34158=CARTESIAN_POINT ( 'NONE',  ( 0.000000000000000000, 0.000000000000000000, -5.000000000000000000 ) ) ;
#34159=CARTESIAN_POINT ( 'NONE',  ( -55.00000337463109901, -60.62177826491083010, -5.000000000000000000 ) ) ;
#34160=CARTESIAN_POINT ( 'NONE',  ( 90.60231327712337190, 15.97563234535636134, -49.86561046011506448 ) ) ;
#34161=ORIENTED_EDGE ( 'NONE', *, *, #17999, .T. ) ;
#34162=CARTESIAN_POINT ( 'NONE',  ( 7.999996625368618552, 69.28203230275516944, -9.999999999999998224 ) ) ;
#34163=LINE ( 'NONE', #28315, #33584 ) ;
#34164=ADVANCED_FACE ( 'NONE', ( #21658 ), #4794, .F. ) ;
#34166=VERTEX_POINT ( 'NONE', #13027 ) ;
#34167=CIRCLE ( 'NONE', #25785, 2.000000000000000000 ) ;
#34168=DIRECTION ( 'NONE',  ( 0.000000000000000000, 0.000000000000000000, 1.000000000000000000 ) ) ;
#34170=EDGE_LOOP ( 'NONE', ( #18449, #1171, #21656, #5527 ) ) ;
#34171=ORIENTED_EDGE ( 'NONE', *, *, #36839, .F. ) ;
#34172=CARTESIAN_POINT ( 'NONE',  ( -70.00000337463099243, -2.428612866367529932E-14, -9.999999999999998224 ) ) ;
#34173=CARTESIAN_POINT ( 'NONE',  ( 82.99999662536832545, 8.660254037844394404, 12.50000000000000000 ) ) ;
#34174=AXIS2_PLACEMENT_3D ( 'NONE', #24786, #36219, #33603 ) ;
#34175=CARTESIAN_POINT ( 'NONE',  ( 61.99999662536845335, 34.64101615137759893, 17.49999999999999645 ) ) ;
#34176=CARTESIAN_POINT ( 'NONE',  ( -3.374631334790434423E-06, 69.28203230275516944, -9.999999999999998224 ) ) ;
#34177=ORIENTED_EDGE ( 'NONE', *, *, #6127, .T. ) ;
#34179=DIRECTION ( 'NONE',  ( -1.000000000000000000, 0.000000000000000000, 0.000000000000000000 ) ) ;
#34182=VERTEX_POINT ( 'NONE', #10589 ) ;
#34183=EDGE_CURVE ( 'NONE', #30962, #4217, #32092, .T. ) ;
#34184=LINE ( 'NONE', #19739, #21987 ) ;
#34186=VERTEX_POINT ( 'NONE', #21832 ) ;
#34188=DIRECTION ( 'NONE',  ( 1.000000000000000000, 0.000000000000000000, 0.000000000000000000 ) ) ;
#34189=CYLINDRICAL_SURFACE ( 'NONE', #34038, 2.000000000000001776 ) ;
#34190=CARTESIAN_POINT ( 'NONE',  ( 51.99999662536847467, 69.28203230275516944, -5.000000000000000000 ) ) ;
#34192=ORIENTED_EDGE ( 'NONE', *, *, #1103, .F. ) ;
#34193=EDGE_CURVE ( 'NONE', #27668, #35643, #19542, .T. ) ;
#34194=DIRECTION ( 'NONE',  ( 0.000000000000000000, 0.000000000000000000, 1.000000000000000000 ) ) ;
#34195=DIRECTION ( 'NONE',  ( 0.000000000000000000, 0.000000000000000000, 1.000000000000000000 ) ) ;
#34196=EDGE_CURVE ( 'NONE', #29936, #21303, #24958, .T. ) ;
#34197=CARTESIAN_POINT ( 'NONE',  ( -45.00000337463111322, 60.62177826491077326, 17.49999999999999645 ) ) ;
#34198=LINE ( 'NONE', #34010, #35273 ) ;
#34199=ORIENTED_EDGE ( 'NONE', *, *, #34845, .T. ) ;
#34200=CARTESIAN_POINT ( 'NONE',  ( -65.00000337463104927, -43.30127018922202353, -9.999999999999998224 ) ) ;
#34201=AXIS2_PLACEMENT_3D ( 'NONE', #17570, #25845, #29197 ) ;
#34202=FACE_BOUND ( 'NONE', #33586, .T. ) ;
#34203=DIRECTION ( 'NONE',  ( 1.000000000000000000, 0.000000000000000000, 0.000000000000000000 ) ) ;
#34204=DIRECTION ( 'NONE',  ( 0.000000000000000000, 0.000000000000000000, 1.000000000000000000 ) ) ;
#34207=DIRECTION ( 'NONE',  ( 0.000000000000000000, 0.000000000000000000, -1.000000000000000000 ) ) ;
#34208=ADVANCED_FACE ( 'NONE', ( #33831 ), #8346, .F. ) ;
#34211=EDGE_CURVE ( 'NONE', #21629, #28577, #25536, .T. ) ;
#34212=DIRECTION ( 'NONE',  ( 0.000000000000000000, 0.000000000000000000, -1.000000000000000000 ) ) ;
#34213=ORIENTED_EDGE ( 'NONE', *, *, #29868, .T. ) ;
#34216=LINE ( 'NONE', #19774, #6955 ) ;
#34217=DIRECTION ( 'NONE',  ( 1.000000000000000000, 0.000000000000000000, 0.000000000000000000 ) ) ;
#34218=EDGE_LOOP ( 'NONE', ( #20863, #23817, #9183, #3245 ) ) ;
#34219=EDGE_LOOP ( 'NONE', ( #35260, #15400, #24804, #36132 ) ) ;
#34220=ORIENTED_EDGE ( 'NONE', *, *, #21954, .F. ) ;
#34221=CARTESIAN_POINT ( 'NONE',  ( -87.00000337463093558, 25.98076211353317433, 12.50000000000000000 ) ) ;
#34222=CARTESIAN_POINT ( 'NONE',  ( -47.63139720814380951, 27.50000000000055422, -5.000000000000000000 ) ) ;
#34223=DIRECTION ( 'NONE',  ( 0.000000000000000000, 0.000000000000000000, 1.000000000000000000 ) ) ;
#34225=DIRECTION ( 'NONE',  ( 1.000000000000000000, 0.000000000000000000, 0.000000000000000000 ) ) ;
#34226=EDGE_LOOP ( 'NONE', ( #14726, #19404, #31409, #5264 ) ) ;
#34228=ORIENTED_EDGE ( 'NONE', *, *, #15694, .F. ) ;
#34229=FACE_OUTER_BOUND ( 'NONE', #1004, .T. ) ;
#34231=ORIENTED_EDGE ( 'NONE', *, *, #9519, .T. ) ;
#34234=ORIENTED_EDGE ( 'NONE', *, *, #31934, .T. ) ;
#34237=DIRECTION ( 'NONE',  ( 0.000000000000000000, 0.000000000000000000, 1.000000000000000000 ) ) ;
#34241=DIRECTION ( 'NONE',  ( 1.000000000000000000, 0.000000000000000000, 0.000000000000000000 ) ) ;
#34242=CIRCLE ( 'NONE', #18050, 2.000000000000001776 ) ;
#34243=ORIENTED_EDGE ( 'NONE', *, *, #12131, .F. ) ;
#34244=DIRECTION ( 'NONE',  ( 0.000000000000000000, 0.000000000000000000, 1.000000000000000000 ) ) ;
#34245=AXIS2_PLACEMENT_3D ( 'NONE', #9381, #20820, #32254 ) ;
#34246=DIRECTION ( 'NONE',  ( 0.000000000000000000, 0.000000000000000000, 1.000000000000000000 ) ) ;
#34248=CYLINDRICAL_SURFACE ( 'NONE', #33833, 2.000000000000001776 ) ;
#34250=VERTEX_POINT ( 'NONE', #8145 ) ;
#34251=EDGE_CURVE ( 'NONE', #18020, #26782, #23745, .T. ) ;
#34252=ORIENTED_EDGE ( 'NONE', *, *, #23889, .T. ) ;
#34254=CARTESIAN_POINT ( 'NONE',  ( 42.99999662536848888, -77.94228634059960825, -9.999999999999998224 ) ) ;
#34256=ORIENTED_EDGE ( 'NONE', *, *, #3879, .T. ) ;
#34257=CARTESIAN_POINT ( 'NONE',  ( 56.99999662536846046, -43.30127018922200222, 17.49999999999999645 ) ) ;
#34258=DIRECTION ( 'NONE',  ( 1.000000000000000000, 0.000000000000000000, 0.000000000000000000 ) ) ;
#34259=DIRECTION ( 'NONE',  ( 0.000000000000000000, 0.000000000000000000, 1.000000000000000000 ) ) ;
#34261=ORIENTED_EDGE ( 'NONE', *, *, #19810, .F. ) ;
#34263=VERTEX_POINT ( 'NONE', #31368 ) ;
#34264=CARTESIAN_POINT ( 'NONE',  ( -28.00000337463118427, 69.28203230275516944, -9.999999999999998224 ) ) ;
#34266=FACE_BOUND ( 'NONE', #6584, .T. ) ;
#34267=ADVANCED_FACE ( 'NONE', ( #19781 ), #28022, .T. ) ;
#34268=DIRECTION ( 'NONE',  ( -1.000000000000000000, 0.000000000000000000, 0.000000000000000000 ) ) ;
#34269=FACE_BOUND ( 'NONE', #18209, .T. ) ;
#34272=CARTESIAN_POINT ( 'NONE',  ( -15.00000337463126066, 77.94228634059957983, -9.999999999999998224 ) ) ;
#34273=CARTESIAN_POINT ( 'NONE',  ( -58.88972745734203329, -33.99999999999965894, 12.49999999999999822 ) ) ;
#34274=PLANE ( 'NONE',  #2352 ) ;
#34275=ORIENTED_EDGE ( 'NONE', *, *, #11473, .T. ) ;
#34276=DIRECTION ( 'NONE',  ( 1.000000000000000000, 0.000000000000000000, 0.000000000000000000 ) ) ;
#34277=PLANE ( 'NONE',  #16647 ) ;
#34278=DIRECTION ( 'NONE',  ( 0.000000000000000000, 0.000000000000000000, 1.000000000000000000 ) ) ;
#34279=ORIENTED_EDGE ( 'NONE', *, *, #21261, .T. ) ;
#34280=VERTEX_POINT ( 'NONE', #25224 ) ;
#34281=AXIS2_PLACEMENT_3D ( 'NONE', #21208, #30025, #24780 ) ;
#34283=ORIENTED_EDGE ( 'NONE', *, *, #30250, .F. ) ;
#34284=CARTESIAN_POINT ( 'NONE',  ( 39.99999662536853151, 69.28203230275518365, -9.999999999999998224 ) ) ;
#34285=DIRECTION ( 'NONE',  ( 0.000000000000000000, 0.000000000000000000, -1.000000000000000000 ) ) ;
#34286=CARTESIAN_POINT ( 'NONE',  ( -47.63139720814380951, 27.50000000000055422, -10.00000000000000000 ) ) ;
#34287=DIRECTION ( 'NONE',  ( 1.000000000000000000, 0.000000000000000000, 0.000000000000000000 ) ) ;
#34288=CARTESIAN_POINT ( 'NONE',  ( -60.00000337463104216, 34.64101615137757051, -9.999999999999998224 ) ) ;
#34289=DIRECTION ( 'NONE',  ( -1.000000000000000000, 0.000000000000000000, 0.000000000000000000 ) ) ;
#34291=ORIENTED_EDGE ( 'NONE', *, *, #8918, .F. ) ;
#34292=AXIS2_PLACEMENT_3D ( 'NONE', #10353, #26873, #13172 ) ;
#34294=EDGE_CURVE ( 'NONE', #23016, #603, #17734, .T. ) ;
#34296=DIRECTION ( 'NONE',  ( -1.000000000000000000, 0.000000000000000000, 0.000000000000000000 ) ) ;
#34297=DIRECTION ( 'NONE',  ( 0.000000000000000000, 0.000000000000000000, 1.000000000000000000 ) ) ;
#34298=ORIENTED_EDGE ( 'NONE', *, *, #15246, .T. ) ;
#34300=EDGE_CURVE ( 'NONE', #25896, #12555, #14239, .T. ) ;
#34301=FACE_BOUND ( 'NONE', #6496, .T. ) ;
#34302=VERTEX_POINT ( 'NONE', #36474 ) ;
#34304=EDGE_LOOP ( 'NONE', ( #27673, #317 ) ) ;
#34305=CIRCLE ( 'NONE', #13334, 2.000000000000001776 ) ;
#34306=EDGE_CURVE ( 'NONE', #33312, #10163, #1572, .T. ) ;
#34308=VERTEX_POINT ( 'NONE', #8686 ) ;
#34309=FACE_OUTER_BOUND ( 'NONE', #17694, .T. ) ;
#34310=FACE_OUTER_BOUND ( 'NONE', #20890, .T. ) ;
#34311=EDGE_CURVE ( 'NONE', #393, #27431, #25392, .T. ) ;
#34312=DIRECTION ( 'NONE',  ( 0.000000000000000000, 0.000000000000000000, -1.000000000000000000 ) ) ;
#34314=EDGE_LOOP ( 'NONE', ( #3838, #19661, #33617, #5282, #26044 ) ) ;
#34315=VERTEX_POINT ( 'NONE', #34221 ) ;
#34316=ORIENTED_EDGE ( 'NONE', *, *, #7815, .T. ) ;
#34317=AXIS2_PLACEMENT_3D ( 'NONE', #34338, #26443, #189 ) ;
#34318=ORIENTED_EDGE ( 'NONE', *, *, #494, .F. ) ;
#34319=DIRECTION ( 'NONE',  ( 1.000000000000000000, 0.000000000000000000, 0.000000000000000000 ) ) ;
#34320=DIRECTION ( 'NONE',  ( 1.000000000000000000, 0.000000000000000000, 0.000000000000000000 ) ) ;
#34321=DIRECTION ( 'NONE',  ( -1.000000000000000000, 0.000000000000000000, 0.000000000000000000 ) ) ;
#34322=DIRECTION ( 'NONE',  ( -0.000000000000000000, -0.000000000000000000, -1.000000000000000000 ) ) ;
#34323=CARTESIAN_POINT ( 'NONE',  ( -80.00000337463094979, 17.32050807568878525, 12.50000000000000000 ) ) ;
#34324=ORIENTED_EDGE ( 'NONE', *, *, #32367, .T. ) ;
#34325=FACE_OUTER_BOUND ( 'NONE', #5662, .T. ) ;
#34326=ADVANCED_FACE ( 'NONE', ( #11130 ), #5519, .F. ) ;
#34328=VECTOR ( 'NONE', #23364, 1000.000000000000000 ) ;
#34329=CARTESIAN_POINT ( 'NONE',  ( -75.00000337463099243, -25.98076211353322051, 12.50000000000000000 ) ) ;
#34330=VERTEX_POINT ( 'NONE', #22216 ) ;
#34332=DIRECTION ( 'NONE',  ( 1.000000000000000000, 0.000000000000000000, 0.000000000000000000 ) ) ;
#34333=ORIENTED_EDGE ( 'NONE', *, *, #19094, .T. ) ;
#34334=EDGE_CURVE ( 'NONE', #18549, #34302, #28564, .T. ) ;
#34335=EDGE_LOOP ( 'NONE', ( #11295, #2197, #21126 ) ) ;
#34336=DIRECTION ( 'NONE',  ( 0.000000000000000000, 0.000000000000000000, 1.000000000000000000 ) ) ;
#34337=EDGE_CURVE ( 'NONE', #6568, #25502, #35122, .T. ) ;
#34338=CARTESIAN_POINT ( 'NONE',  ( -62.97617850287781494, -4.279621169095772615, -4.999999999999997335 ) ) ;
#34339=CARTESIAN_POINT ( 'NONE',  ( -77.00000337463097821, 8.660254037844374864, 12.50000000000000000 ) ) ;
#34340=DIRECTION ( 'NONE',  ( 1.000000000000000000, 0.000000000000000000, 0.000000000000000000 ) ) ;
#34341=ORIENTED_EDGE ( 'NONE', *, *, #11427, .T. ) ;
#34342=EDGE_LOOP ( 'NONE', ( #17326, #20080, #7665, #5612 ) ) ;
#34343=CIRCLE ( 'NONE', #19355, 2.000000000000001776 ) ;
#34345=CARTESIAN_POINT ( 'NONE',  ( 66.99999662536839651, -43.30127018922199511, -9.999999999999998224 ) ) ;
#34347=AXIS2_PLACEMENT_3D ( 'NONE', #6889, #26962, #10269 ) ;
#34348=ORIENTED_EDGE ( 'NONE', *, *, #23854, .T. ) ;
#34349=CYLINDRICAL_SURFACE ( 'NONE', #32136, 2.000000000000001776 ) ;
#34350=ORIENTED_EDGE ( 'NONE', *, *, #18731, .T. ) ;
#34351=ORIENTED_EDGE ( 'NONE', *, *, #17756, .F. ) ;
#34352=CIRCLE ( 'NONE', #31936, 2.000000000000001776 ) ;
#34353=CARTESIAN_POINT ( 'NONE',  ( 84.99999662536832545, 8.660254037844394404, 12.50000000000000000 ) ) ;
#34354=EDGE_CURVE ( 'NONE', #31383, #31631, #33325, .T. ) ;
#34355=AXIS2_PLACEMENT_3D ( 'NONE', #28908, #31545, #22934 ) ;
#34356=DIRECTION ( 'NONE',  ( 0.000000000000000000, 0.000000000000000000, 1.000000000000000000 ) ) ;
#34358=EDGE_LOOP ( 'NONE', ( #17113, #28560, #17405, #11278 ) ) ;
#34359=CARTESIAN_POINT ( 'NONE',  ( 77.99999662536833966, 17.32050807568879236, 12.50000000000000000 ) ) ;
#34360=VECTOR ( 'NONE', #4033, 1000.000000000000000 ) ;
#34361=DIRECTION ( 'NONE',  ( 0.000000000000000000, 0.000000000000000000, 1.000000000000000000 ) ) ;
#34363=ORIENTED_EDGE ( 'NONE', *, *, #21996, .T. ) ;
#34364=CARTESIAN_POINT ( 'NONE',  ( 69.99999662536839651, -17.32050807568879947, 17.49999999999999645 ) ) ;
#34365=FACE_BOUND ( 'NONE', #34945, .T. ) ;
#34366=CARTESIAN_POINT ( 'NONE',  ( -87.00000337463093558, 8.660254037844389075, 17.49999999999999645 ) ) ;
#34367=DIRECTION ( 'NONE',  ( 1.000000000000000000, 0.000000000000000000, 0.000000000000000000 ) ) ;
#34368=CARTESIAN_POINT ( 'NONE',  ( -18.00000337463123756, -69.28203230275522628, -5.000000000000000000 ) ) ;
#34369=CARTESIAN_POINT ( 'NONE',  ( -82.00000337463094979, -2.404119930384582903E-14, -9.999999999999998224 ) ) ;
#34370=CIRCLE ( 'NONE', #10406, 2.000000000000001776 ) ;
#34371=ADVANCED_FACE ( 'NONE', ( #11668 ), #29303, .F. ) ;
#34373=ORIENTED_EDGE ( 'NONE', *, *, #36493, .T. ) ;
#34374=EDGE_CURVE ( 'NONE', #8594, #3287, #3361, .T. ) ;
#34375=DIRECTION ( 'NONE',  ( 0.000000000000000000, 0.000000000000000000, 1.000000000000000000 ) ) ;
#34377=DIRECTION ( 'NONE',  ( 0.000000000000000000, 0.000000000000000000, 1.000000000000000000 ) ) ;
#34379=ORIENTED_EDGE ( 'NONE', *, *, #31242, .T. ) ;
#34380=EDGE_CURVE ( 'NONE', #25160, #18782, #36329, .T. ) ;
#34381=ORIENTED_EDGE ( 'NONE', *, *, #13014, .T. ) ;
#34382=EDGE_LOOP ( 'NONE', ( #23982, #1837, #28637, #15069, #9251 ) ) ;
#34383=AXIS2_PLACEMENT_3D ( 'NONE', #22719, #20066, #9011 ) ;
#34384=DIRECTION ( 'NONE',  ( 0.000000000000000000, 0.000000000000000000, -1.000000000000000000 ) ) ;
#34385=CARTESIAN_POINT ( 'NONE',  ( 74.99999662536835388, -25.98076211353319565, -9.999999999999998224 ) ) ;
#34386=EDGE_CURVE ( 'NONE', #34851, #18020, #9435, .T. ) ;
#34387=FACE_OUTER_BOUND ( 'NONE', #9113, .T. ) ;
#34389=EDGE_CURVE ( 'NONE', #30855, #15669, #22533, .T. ) ;
#34391=EDGE_LOOP ( 'NONE', ( #10588, #7885, #13460, #18629, #34730 ) ) ;
#34392=DIRECTION ( 'NONE',  ( 1.000000000000000000, 0.000000000000000000, 0.000000000000000000 ) ) ;
#34393=ORIENTED_EDGE ( 'NONE', *, *, #32489, .T. ) ;
#34394=DIRECTION ( 'NONE',  ( -1.000000000000000000, 0.000000000000000000, 0.000000000000000000 ) ) ;
#34395=VERTEX_POINT ( 'NONE', #35328 ) ;
#34396=EDGE_CURVE ( 'NONE', #26676, #13541, #34767, .T. ) ;
#34397=EDGE_LOOP ( 'NONE', ( #7516, #29811 ) ) ;
#34399=VECTOR ( 'NONE', #30771, 1000.000000000000000 ) ;
#34400=DIRECTION ( 'NONE',  ( 0.000000000000000000, 0.000000000000000000, 1.000000000000000000 ) ) ;
#34401=DIRECTION ( 'NONE',  ( 0.000000000000000000, 0.000000000000000000, -1.000000000000000000 ) ) ;
#34402=EDGE_CURVE ( 'NONE', #406, #24516, #12036, .T. ) ;
#34403=DIRECTION ( 'NONE',  ( 1.000000000000000000, 0.000000000000000000, 0.000000000000000000 ) ) ;
#34405=DIRECTION ( 'NONE',  ( 1.000000000000000000, 0.000000000000000000, 0.000000000000000000 ) ) ;
#34406=AXIS2_PLACEMENT_3D ( 'NONE', #23239, #3727, #34692 ) ;
#34407=DIRECTION ( 'NONE',  ( 0.000000000000000000, 0.000000000000000000, 1.000000000000000000 ) ) ;
#34408=CARTESIAN_POINT ( 'NONE',  ( -3.374631289687624047E-06, -69.28203230275519786, -9.999999999999998224 ) ) ;
#34410=CIRCLE ( 'NONE', #9826, 2.000000000000001776 ) ;
#34412=DIRECTION ( 'NONE',  ( 0.000000000000000000, 0.000000000000000000, -1.000000000000000000 ) ) ;
#34413=VERTEX_POINT ( 'NONE', #17493 ) ;
#34415=CARTESIAN_POINT ( 'NONE',  ( -12.00000337463128197, 86.60254037844397601, -9.999999999999998224 ) ) ;
#34416=DIRECTION ( 'NONE',  ( 0.000000000000000000, 0.000000000000000000, 1.000000000000000000 ) ) ;
#34417=CARTESIAN_POINT ( 'NONE',  ( 81.99999662536833966, -3.469446951953614189E-15, -5.000000000000000000 ) ) ;
#34418=EDGE_CURVE ( 'NONE', #7729, #21619, #34580, .T. ) ;
#34421=ADVANCED_FACE ( 'NONE', ( #23322 ), #20666, .F. ) ;
#34422=CIRCLE ( 'NONE', #28985, 2.000000000000001776 ) ;
#34424=DIRECTION ( 'NONE',  ( -1.000000000000000000, 0.000000000000000000, 0.000000000000000000 ) ) ;
#34425=ORIENTED_EDGE ( 'NONE', *, *, #28455, .F. ) ;
#34426=VECTOR ( 'NONE', #13301, 1000.000000000000000 ) ;
#34427=ORIENTED_EDGE ( 'NONE', *, *, #24459, .F. ) ;
#34428=ORIENTED_EDGE ( 'NONE', *, *, #8215, .T. ) ;
#34429=CARTESIAN_POINT ( 'NONE',  ( 49.99999662536846756, -69.28203230275519786, -9.999999999999998224 ) ) ;
#34430=DIRECTION ( 'NONE',  ( 1.000000000000000000, 0.000000000000000000, 0.000000000000000000 ) ) ;
#34431=EDGE_CURVE ( 'NONE', #4753, #31059, #10329, .T. ) ;
#34433=CIRCLE ( 'NONE', #10495, 2.000000000000001776 ) ;
#34434=AXIS2_PLACEMENT_3D ( 'NONE', #32679, #36069, #12790 ) ;
#34435=EDGE_LOOP ( 'NONE', ( #1914, #4378 ) ) ;
#34436=CIRCLE ( 'NONE', #23044, 33.00000000000001421 ) ;
#34437=DIRECTION ( 'NONE',  ( 0.000000000000000000, 0.000000000000000000, 1.000000000000000000 ) ) ;
#34438=ORIENTED_EDGE ( 'NONE', *, *, #15087, .F. ) ;
#34439=FACE_OUTER_BOUND ( 'NONE', #18916, .T. ) ;
#34440=EDGE_LOOP ( 'NONE', ( #29500, #28955, #15695, #21123 ) ) ;
#34441=DIRECTION ( 'NONE',  ( 0.000000000000000000, 0.000000000000000000, -1.000000000000000000 ) ) ;
#34442=EDGE_CURVE ( 'NONE', #17803, #31097, #7928, .T. ) ;
#34444=EDGE_CURVE ( 'NONE', #13283, #22239, #14510, .T. ) ;
#34445=CARTESIAN_POINT ( 'NONE',  ( -43.00000337463111322, -77.94228634059960825, 12.50000000000000000 ) ) ;
#34446=EDGE_CURVE ( 'NONE', #21906, #30228, #35480, .T. ) ;
#34448=FACE_BOUND ( 'NONE', #11588, .T. ) ;
#34449=AXIS2_PLACEMENT_3D ( 'NONE', #36857, #20165, #31592 ) ;
#34451=CIRCLE ( 'NONE', #4527, 33.00000000000001421 ) ;
#34452=VECTOR ( 'NONE', #25304, 1000.000000000000000 ) ;
#34453=DIRECTION ( 'NONE',  ( 0.000000000000000000, 0.000000000000000000, 1.000000000000000000 ) ) ;
#34454=DIRECTION ( 'NONE',  ( 1.000000000000000000, 0.000000000000000000, 0.000000000000000000 ) ) ;
#34455=DIRECTION ( 'NONE',  ( 0.000000000000000000, 0.000000000000000000, 1.000000000000000000 ) ) ;
#34456=ORIENTED_EDGE ( 'NONE', *, *, #27757, .F. ) ;
#34457=DIRECTION ( 'NONE',  ( 0.000000000000000000, 0.000000000000000000, 1.000000000000000000 ) ) ;
#34458=FACE_OUTER_BOUND ( 'NONE', #23545, .T. ) ;
#34459=CIRCLE ( 'NONE', #26066, 2.000000000000001776 ) ;
#34460=DIRECTION ( 'NONE',  ( 0.000000000000000000, 0.000000000000000000, 1.000000000000000000 ) ) ;
#34464=ORIENTED_EDGE ( 'NONE', *, *, #7847, .F. ) ;
#34465=ORIENTED_EDGE ( 'NONE', *, *, #17072, .T. ) ;
#34467=DIRECTION ( 'NONE',  ( 0.000000000000000000, 0.000000000000000000, 1.000000000000000000 ) ) ;
#34468=VECTOR ( 'NONE', #16802, 1000.000000000000000 ) ;
#34469=DIRECTION ( 'NONE',  ( -1.000000000000000000, 0.000000000000000000, -0.000000000000000000 ) ) ;
#34471=DIRECTION ( 'NONE',  ( -1.000000000000000000, 0.000000000000000000, 0.000000000000000000 ) ) ;
#34472=AXIS2_PLACEMENT_3D ( 'NONE', #1265, #13070, #20960 ) ;
#34476=AXIS2_PLACEMENT_3D ( 'NONE', #21102, #9286, #6844 ) ;
#34477=EDGE_LOOP ( 'NONE', ( #8244, #24898, #24383, #24463 ) ) ;
#34478=EDGE_LOOP ( 'NONE', ( #24213, #7446, #24712, #35333 ) ) ;
#34479=DIRECTION ( 'NONE',  ( 0.000000000000000000, 0.000000000000000000, 1.000000000000000000 ) ) ;
#34480=DIRECTION ( 'NONE',  ( -1.000000000000000000, 0.000000000000000000, 0.000000000000000000 ) ) ;
#34481=CARTESIAN_POINT ( 'NONE',  ( -75.00000337463097821, 8.660254037844374864, 17.49999999999999645 ) ) ;
#34482=ORIENTED_EDGE ( 'NONE', *, *, #7847, .T. ) ;
#34485=ORIENTED_EDGE ( 'NONE', *, *, #12686, .F. ) ;
#34488=FACE_OUTER_BOUND ( 'NONE', #22254, .T. ) ;
#34490=AXIS2_PLACEMENT_3D ( 'NONE', #25071, #33853, #14356 ) ;
#34496=VECTOR ( 'NONE', #29946, 1000.000000000000000 ) ;
#34497=ORIENTED_EDGE ( 'NONE', *, *, #9145, .F. ) ;
#34498=CIRCLE ( 'NONE', #2163, 2.000000000000001776 ) ;
#34499=CIRCLE ( 'NONE', #36885, 2.000000000000001776 ) ;
#34500=ORIENTED_EDGE ( 'NONE', *, *, #6074, .F. ) ;
#34501=AXIS2_PLACEMENT_3D ( 'NONE', #31635, #17399, #20014 ) ;
#34502=ORIENTED_EDGE ( 'NONE', *, *, #12075, .T. ) ;
#34503=DIRECTION ( 'NONE',  ( 0.000000000000000000, -0.000000000000000000, -1.000000000000000000 ) ) ;
#34504=CARTESIAN_POINT ( 'NONE',  ( 9.999996625368625658, 86.60254037844397601, -9.999999999999998224 ) ) ;
#34505=FACE_OUTER_BOUND ( 'NONE', #6725, .T. ) ;
#34508=ADVANCED_FACE ( 'NONE', ( #33424 ), #21615, .F. ) ;
#34509=ORIENTED_EDGE ( 'NONE', *, *, #25421, .F. ) ;
#34510=CARTESIAN_POINT ( 'NONE',  ( -31.46585318596190106, -86.45172111230344569, 12.49999999999999822 ) ) ;
#34512=CARTESIAN_POINT ( 'NONE',  ( -2.000003374631334818, 69.28203230275516944, -5.000000000000000000 ) ) ;
#34513=ORIENTED_EDGE ( 'NONE', *, *, #12809, .T. ) ;
#34514=CARTESIAN_POINT ( 'NONE',  ( -19.13981058454750794, 60.93295298010998806, 12.49999999999999822 ) ) ;
#34515=EDGE_CURVE ( 'NONE', #5895, #25177, #3134, .T. ) ;
#34517=ORIENTED_EDGE ( 'NONE', *, *, #36938, .T. ) ;
#34518=VECTOR ( 'NONE', #11309, 1000.000000000000000 ) ;
#34521=CYLINDRICAL_SURFACE ( 'NONE', #6871, 2.000000000000000000 ) ;
#34522=AXIS2_PLACEMENT_3D ( 'NONE', #10521, #7721, #7345 ) ;
#34523=DIRECTION ( 'NONE',  ( 0.000000000000000000, 0.000000000000000000, -1.000000000000000000 ) ) ;
#34528=AXIS2_PLACEMENT_3D ( 'NONE', #19587, #2695, #28202 ) ;
#34529=AXIS2_PLACEMENT_3D ( 'NONE', #6876, #12504, #26949 ) ;
#34530=CIRCLE ( 'NONE', #36332, 2.000000000000001776 ) ;
#34531=CYLINDRICAL_SURFACE ( 'NONE', #29081, 3.000000000000002665 ) ;
#34532=CARTESIAN_POINT ( 'NONE',  ( 59.99999662536842493, 51.96152422706639129, 12.50000000000000000 ) ) ;
#34535=CIRCLE ( 'NONE', #21953, 2.000000000000000000 ) ;
#34537=EDGE_CURVE ( 'NONE', #16351, #25578, #32658, .T. ) ;
#34538=DIRECTION ( 'NONE',  ( 0.000000000000000000, 0.000000000000000000, 1.000000000000000000 ) ) ;
#34539=ORIENTED_EDGE ( 'NONE', *, *, #15546, .F. ) ;
#34540=ORIENTED_EDGE ( 'NONE', *, *, #11690, .F. ) ;
#34541=VECTOR ( 'NONE', #22956, 1000.000000000000000 ) ;
#34542=CYLINDRICAL_SURFACE ( 'NONE', #30164, 2.000000000000001776 ) ;
#34543=CARTESIAN_POINT ( 'NONE',  ( 69.99999662536839651, 17.32050807568879236, 12.50000000000000000 ) ) ;
#34544=ORIENTED_EDGE ( 'NONE', *, *, #1319, .F. ) ;
#34545=ORIENTED_EDGE ( 'NONE', *, *, #22844, .T. ) ;
#34546=CARTESIAN_POINT ( 'NONE',  ( 82.99999662536832545, 25.98076211353319565, -9.999999999999998224 ) ) ;
#34548=EDGE_CURVE ( 'NONE', #27432, #745, #13913, .T. ) ;
#34549=CARTESIAN_POINT ( 'NONE',  ( 67.99999662536839651, 51.96152422706640550, -5.000000000000000000 ) ) ;
#34550=DIRECTION ( 'NONE',  ( 1.000000000000000000, 0.000000000000000000, 0.000000000000000000 ) ) ;
#34551=CIRCLE ( 'NONE', #11771, 2.000000000000001776 ) ;
#34552=ORIENTED_EDGE ( 'NONE', *, *, #4373, .F. ) ;
#34553=FACE_OUTER_BOUND ( 'NONE', #21779, .T. ) ;
#34555=ADVANCED_FACE ( 'NONE', ( #1737 ), #3990, .T. ) ;
#34556=FACE_BOUND ( 'NONE', #14389, .T. ) ;
#34558=CARTESIAN_POINT ( 'NONE',  ( 66.99999662536842493, 43.30127018922200222, 17.49999999999999645 ) ) ;
#34560=CARTESIAN_POINT ( 'NONE',  ( -2.000003374631303732, -86.60254037844400443, -9.999999999999998224 ) ) ;
#34561=AXIS2_PLACEMENT_3D ( 'NONE', #20683, #11511, #26499 ) ;
#34563=ADVANCED_FACE ( 'NONE', ( #4548 ), #15794, .F. ) ;
#34566=AXIS2_PLACEMENT_3D ( 'NONE', #36082, #10379, #36457 ) ;
#34567=DIRECTION ( 'NONE',  ( 0.000000000000000000, 0.000000000000000000, 1.000000000000000000 ) ) ;
#34568=DIRECTION ( 'NONE',  ( 0.000000000000000000, 0.000000000000000000, 1.000000000000000000 ) ) ;
#34569=ORIENTED_EDGE ( 'NONE', *, *, #31595, .T. ) ;
#34571=ADVANCED_FACE ( 'NONE', ( #27605 ), #27217, .F. ) ;
#34572=DIRECTION ( 'NONE',  ( 0.000000000000000000, 0.000000000000000000, 1.000000000000000000 ) ) ;
#34573=DIRECTION ( 'NONE',  ( 0.000000000000000000, 0.000000000000000000, 1.000000000000000000 ) ) ;
#34574=AXIS2_PLACEMENT_3D ( 'NONE', #27111, #16071, #4631 ) ;
#34575=ORIENTED_EDGE ( 'NONE', *, *, #18072, .T. ) ;
#34576=AXIS2_PLACEMENT_3D ( 'NONE', #12173, #17634, #18022 ) ;
#34577=ORIENTED_EDGE ( 'NONE', *, *, #11316, .F. ) ;
#34578=EDGE_LOOP ( 'NONE', ( #2625, #22106, #22090, #17990 ) ) ;
#34579=EDGE_CURVE ( 'NONE', #24524, #14473, #15621, .T. ) ;
#34580=LINE ( 'NONE', #26671, #36094 ) ;
#34582=CARTESIAN_POINT ( 'NONE',  ( 64.99999662536841072, 25.98076211353318854, -9.999999999999998224 ) ) ;
#34583=VERTEX_POINT ( 'NONE', #24226 ) ;
#34584=AXIS2_PLACEMENT_3D ( 'NONE', #15648, #12804, #4023 ) ;
#34585=AXIS2_PLACEMENT_3D ( 'NONE', #6405, #15912, #30151 ) ;
#34586=DIRECTION ( 'NONE',  ( 0.000000000000000000, 0.000000000000000000, 1.000000000000000000 ) ) ;
#34587=AXIS2_PLACEMENT_3D ( 'NONE', #7225, #27461, #21650 ) ;
#34588=ORIENTED_EDGE ( 'NONE', *, *, #35465, .T. ) ;
#34592=ORIENTED_EDGE ( 'NONE', *, *, #15395, .F. ) ;
#34593=EDGE_LOOP ( 'NONE', ( #10883, #35599, #18356, #36682 ) ) ;
#34594=AXIS2_PLACEMENT_3D ( 'NONE', #28110, #30909, #27566 ) ;
#34596=EDGE_CURVE ( 'NONE', #6951, #24986, #31279, .T. ) ;
#34597=CARTESIAN_POINT ( 'NONE',  ( 27.78182860042856461, 56.67878100130339902, -49.86348611802629449 ) ) ;
#34599=ORIENTED_EDGE ( 'NONE', *, *, #16057, .F. ) ;
#34601=AXIS2_PLACEMENT_3D ( 'NONE', #6096, #20906, #11895 ) ;
#34602=EDGE_CURVE ( 'NONE', #21975, #16037, #28862, .T. ) ;
#34603=DIRECTION ( 'NONE',  ( -0.000000000000000000, -0.000000000000000000, -1.000000000000000000 ) ) ;
#34604=CARTESIAN_POINT ( 'NONE',  ( 4.279621169095998212, -62.97617850287780072, 12.49999999999999822 ) ) ;
#34605=ORIENTED_EDGE ( 'NONE', *, *, #18911, .T. ) ;
#34606=CARTESIAN_POINT ( 'NONE',  ( 77.99999662536833966, 34.64101615137759183, 17.49999999999999645 ) ) ;
#34607=CIRCLE ( 'NONE', #458, 2.000000000000000000 ) ;
#34608=DIRECTION ( 'NONE',  ( 0.000000000000000000, 0.000000000000000000, 1.000000000000000000 ) ) ;
#34609=ADVANCED_FACE ( 'NONE', ( #33220 ), #36054, .F. ) ;
#34610=VERTEX_POINT ( 'NONE', #4358 ) ;
#34611=CARTESIAN_POINT ( 'NONE',  ( 22.99999662536857059, 77.94228634059957983, -9.999999999999998224 ) ) ;
#34612=AXIS2_PLACEMENT_3D ( 'NONE', #8385, #31240, #25261 ) ;
#34614=DIRECTION ( 'NONE',  ( 1.000000000000000000, 0.000000000000000000, 0.000000000000000000 ) ) ;
#34615=DIRECTION ( 'NONE',  ( 1.000000000000000000, 0.000000000000000000, 0.000000000000000000 ) ) ;
#34617=AXIS2_PLACEMENT_3D ( 'NONE', #30343, #18732, #13278 ) ;
#34618=CARTESIAN_POINT ( 'NONE',  ( 57.99999662536844625, 34.64101615137759893, -5.000000000000000000 ) ) ;
#34620=VERTEX_POINT ( 'NONE', #7540 ) ;
#34622=DIRECTION ( 'NONE',  ( 1.000000000000000000, 0.000000000000000000, 0.000000000000000000 ) ) ;
#34623=ORIENTED_EDGE ( 'NONE', *, *, #14255, .F. ) ;
#34624=CIRCLE ( 'NONE', #19652, 2.000000000000001776 ) ;
#34625=ORIENTED_EDGE ( 'NONE', *, *, #16391, .T. ) ;
#34626=ORIENTED_EDGE ( 'NONE', *, *, #22975, .T. ) ;
#34627=ADVANCED_FACE ( 'NONE', ( #12602 ), #21981, .F. ) ;
#34629=DIRECTION ( 'NONE',  ( 0.000000000000000000, 0.000000000000000000, 1.000000000000000000 ) ) ;
#34630=CARTESIAN_POINT ( 'NONE',  ( 34.99999662536855283, 60.62177826491078747, 17.49999999999999645 ) ) ;
#34632=AXIS2_PLACEMENT_3D ( 'NONE', #25750, #5320, #8486 ) ;
#34633=CYLINDRICAL_SURFACE ( 'NONE', #32028, 2.000000000000001776 ) ;
#34634=ORIENTED_EDGE ( 'NONE', *, *, #19844, .T. ) ;
#34635=CARTESIAN_POINT ( 'NONE',  ( 86.99999662536832545, 8.660254037844394404, -5.000000000000000000 ) ) ;
#34636=VERTEX_POINT ( 'NONE', #1534 ) ;
#34637=AXIS2_PLACEMENT_3D ( 'NONE', #36098, #36475, #10947 ) ;
#34639=FACE_BOUND ( 'NONE', #3657, .T. ) ;
#34640=AXIS2_PLACEMENT_3D ( 'NONE', #14755, #11747, #23207 ) ;
#34642=CIRCLE ( 'NONE', #34034, 3.000000000000002665 ) ;
#34643=CYLINDRICAL_SURFACE ( 'NONE', #32269, 1.999999999999998224 ) ;
#34645=EDGE_CURVE ( 'NONE', #8370, #9761, #9982, .T. ) ;
#34646=DIRECTION ( 'NONE',  ( 1.000000000000000000, 0.000000000000000000, 0.000000000000000000 ) ) ;
#34648=EDGE_CURVE ( 'NONE', #31778, #17896, #15715, .T. ) ;
#34649=CARTESIAN_POINT ( 'NONE',  ( -45.00000337463111322, 77.94228634059959404, 12.50000000000000000 ) ) ;
#34650=CIRCLE ( 'NONE', #31628, 2.000000000000000000 ) ;
#34651=CARTESIAN_POINT ( 'NONE',  ( -2.778182860043013847, -66.86787810013035482, -49.86348611802629449 ) ) ;
#34652=DIRECTION ( 'NONE',  ( -1.000000000000000000, 0.000000000000000000, -0.000000000000000000 ) ) ;
#34654=CARTESIAN_POINT ( 'NONE',  ( -70.00000337463102085, -34.64101615137762025, 12.50000000000000000 ) ) ;
#34655=EDGE_CURVE ( 'NONE', #23066, #21363, #10736, .T. ) ;
#34656=DIRECTION ( 'NONE',  ( 0.000000000000000000, 0.000000000000000000, -1.000000000000000000 ) ) ;
#34657=AXIS2_PLACEMENT_3D ( 'NONE', #10116, #29979, #21545 ) ;
#34658=DIRECTION ( 'NONE',  ( 1.000000000000000000, 0.000000000000000000, 0.000000000000000000 ) ) ;
#34659=EDGE_CURVE ( 'NONE', #18483, #6666, #30083, .T. ) ;
#34660=ORIENTED_EDGE ( 'NONE', *, *, #10816, .F. ) ;
#34662=VECTOR ( 'NONE', #26841, 1000.000000000000000 ) ;
#34663=VERTEX_POINT ( 'NONE', #33613 ) ;
#34668=DIRECTION ( 'NONE',  ( 0.000000000000000000, 0.000000000000000000, 1.000000000000000000 ) ) ;
#34670=ADVANCED_FACE ( 'NONE', ( #13526 ), #7738, .F. ) ;
#34671=EDGE_CURVE ( 'NONE', #10470, #8482, #9118, .T. ) ;
#34672=CIRCLE ( 'NONE', #22697, 2.000000000000000000 ) ;
#34674=CARTESIAN_POINT ( 'NONE',  ( -5.000003374631307729, 77.94228634059957983, -9.999999999999998224 ) ) ;
#34675=DIRECTION ( 'NONE',  ( 1.000000000000000000, 0.000000000000000000, 0.000000000000000000 ) ) ;
#34676=AXIS2_PLACEMENT_3D ( 'NONE', #25486, #18984, #31283 ) ;
#34678=EDGE_LOOP ( 'NONE', ( #638, #1120, #29978, #34660 ) ) ;
#34679=ORIENTED_EDGE ( 'NONE', *, *, #15694, .T. ) ;
#34680=AXIS2_PLACEMENT_3D ( 'NONE', #14852, #12383, #26292 ) ;
#34681=DIRECTION ( 'NONE',  ( 0.000000000000000000, 0.000000000000000000, 1.000000000000000000 ) ) ;
#34682=DIRECTION ( 'NONE',  ( 0.000000000000000000, 0.000000000000000000, -1.000000000000000000 ) ) ;
#34683=CARTESIAN_POINT ( 'NONE',  ( 52.39915983220795681, 35.19434990244919703, -4.999999999999997335 ) ) ;
#34685=DIRECTION ( 'NONE',  ( 1.000000000000000000, 0.000000000000000000, 0.000000000000000000 ) ) ;
#34687=ORIENTED_EDGE ( 'NONE', *, *, #14181, .T. ) ;
#34688=ORIENTED_EDGE ( 'NONE', *, *, #32320, .T. ) ;
#34689=CIRCLE ( 'NONE', #22722, 2.000000000000001776 ) ;
#34691=ORIENTED_EDGE ( 'NONE', *, *, #1528, .F. ) ;
#34692=DIRECTION ( 'NONE',  ( -1.000000000000000000, 0.000000000000000000, 0.000000000000000000 ) ) ;
#34693=DIRECTION ( 'NONE',  ( 1.000000000000000000, 0.000000000000000000, 0.000000000000000000 ) ) ;
#34694=ORIENTED_EDGE ( 'NONE', *, *, #22958, .T. ) ;
#34695=VERTEX_POINT ( 'NONE', #5097 ) ;
#34696=AXIS2_PLACEMENT_3D ( 'NONE', #23191, #28969, #20932 ) ;
#34699=CIRCLE ( 'NONE', #13736, 2.000000000000001776 ) ;
#34700=VERTEX_POINT ( 'NONE', #16353 ) ;
#34701=DIRECTION ( 'NONE',  ( 1.000000000000000000, 0.000000000000000000, 0.000000000000000000 ) ) ;
#34702=CIRCLE ( 'NONE', #10746, 2.000000000000001776 ) ;
#34703=DIRECTION ( 'NONE',  ( 1.000000000000000000, 0.000000000000000000, 0.000000000000000000 ) ) ;
#34704=DIRECTION ( 'NONE',  ( 0.000000000000000000, 0.000000000000000000, -1.000000000000000000 ) ) ;
#34707=ORIENTED_EDGE ( 'NONE', *, *, #7365, .F. ) ;
#34708=DIRECTION ( 'NONE',  ( -1.000000000000000000, 0.000000000000000000, 0.000000000000000000 ) ) ;
#34709=DIRECTION ( 'NONE',  ( 1.000000000000000000, 0.000000000000000000, 0.000000000000000000 ) ) ;
#34710=AXIS2_PLACEMENT_3D ( 'NONE', #30187, #7707, #19156 ) ;
#34711=AXIS2_PLACEMENT_3D ( 'NONE', #36505, #30496, #16069 ) ;
#34713=DIRECTION ( 'NONE',  ( 1.000000000000000000, 0.000000000000000000, 0.000000000000000000 ) ) ;
#34715=CARTESIAN_POINT ( 'NONE',  ( 46.99999662536851019, -60.62177826491080168, 12.50000000000000000 ) ) ;
#34716=CIRCLE ( 'NONE', #9573, 33.00000000000001421 ) ;
#34717=DIRECTION ( 'NONE',  ( 1.000000000000000000, 0.000000000000000000, 0.000000000000000000 ) ) ;
#34718=ORIENTED_EDGE ( 'NONE', *, *, #15836, .T. ) ;
#34719=ORIENTED_EDGE ( 'NONE', *, *, #20087, .T. ) ;
#34721=CARTESIAN_POINT ( 'NONE',  ( -59.13646009116099833, 70.47608876694653190, 12.49999999999999822 ) ) ;
#34722=DIRECTION ( 'NONE',  ( 0.000000000000000000, 0.000000000000000000, 1.000000000000000000 ) ) ;
#34723=DIRECTION ( 'NONE',  ( 0.000000000000000000, 0.000000000000000000, 1.000000000000000000 ) ) ;
#34724=ORIENTED_EDGE ( 'NONE', *, *, #19239, .T. ) ;
#34725=AXIS2_PLACEMENT_3D ( 'NONE', #5158, #22394, #5704 ) ;
#34726=CARTESIAN_POINT ( 'NONE',  ( -52.39915983220772233, -35.19434990244957362, -49.22241343995298024 ) ) ;
#34728=DIRECTION ( 'NONE',  ( -0.000000000000000000, -0.000000000000000000, 1.000000000000000000 ) ) ;
#34729=CIRCLE ( 'NONE', #14354, 2.000000000000001776 ) ;
#34730=ORIENTED_EDGE ( 'NONE', *, *, #4143, .F. ) ;
#34731=CIRCLE ( 'NONE', #28745, 2.000000000000001776 ) ;
#34732=FACE_OUTER_BOUND ( 'NONE', #10509, .T. ) ;
#34733=AXIS2_PLACEMENT_3D ( 'NONE', #2631, #10887, #10716 ) ;
#34734=VERTEX_POINT ( 'NONE', #24990 ) ;
#34735=ADVANCED_FACE ( 'NONE', ( #11281 ), #27970, .F. ) ;
#34737=DIRECTION ( 'NONE',  ( 0.000000000000000000, 0.000000000000000000, -1.000000000000000000 ) ) ;
#34738=CARTESIAN_POINT ( 'NONE',  ( -70.00000337463102085, -34.64101615137762025, -5.000000000000000000 ) ) ;
#34739=AXIS2_PLACEMENT_3D ( 'NONE', #31225, #34608, #14904 ) ;
#34740=CARTESIAN_POINT ( 'NONE',  ( -57.00000337463109901, -60.62177826491083010, -9.999999999999998224 ) ) ;
#34741=ORIENTED_EDGE ( 'NONE', *, *, #8853, .T. ) ;
#34742=VERTEX_POINT ( 'NONE', #34173 ) ;
#34744=CARTESIAN_POINT ( 'NONE',  ( 9.999996625368625658, 86.60254037844397601, 12.50000000000000000 ) ) ;
#34745=DIRECTION ( 'NONE',  ( 1.000000000000000000, 0.000000000000000000, 0.000000000000000000 ) ) ;
#34746=CARTESIAN_POINT ( 'NONE',  ( 71.99999662536839651, -17.32050807568879947, -9.999999999999998224 ) ) ;
#34747=EDGE_CURVE ( 'NONE', #28991, #27815, #19899, .T. ) ;
#34749=CARTESIAN_POINT ( 'NONE',  ( 44.99999662536851019, -60.62177826491080168, -9.999999999999998224 ) ) ;
#34750=FACE_BOUND ( 'NONE', #32406, .T. ) ;
#34753=DIRECTION ( 'NONE',  ( 0.000000000000000000, 0.000000000000000000, 1.000000000000000000 ) ) ;
#34756=AXIS2_PLACEMENT_3D ( 'NONE', #16725, #8459, #11270 ) ;
#34757=EDGE_CURVE ( 'NONE', #25770, #5185, #21114, .T. ) ;
#34758=CARTESIAN_POINT ( 'NONE',  ( -70.00000337463099243, -2.428612866367529932E-14, -5.000000000000000000 ) ) ;
#34759=ORIENTED_EDGE ( 'NONE', *, *, #6003, .T. ) ;
#34760=CARTESIAN_POINT ( 'NONE',  ( 11.99999662536865763, -86.60254037844400443, -9.999999999999998224 ) ) ;
#34763=CARTESIAN_POINT ( 'NONE',  ( -8.000003374631249997, -86.60254037844400443, -5.000000000000000000 ) ) ;
#34764=VERTEX_POINT ( 'NONE', #26074 ) ;
#34765=ORIENTED_EDGE ( 'NONE', *, *, #36536, .F. ) ;
#34766=ORIENTED_EDGE ( 'NONE', *, *, #20746, .F. ) ;
#34767=LINE ( 'NONE', #9625, #27314 ) ;
#34770=VERTEX_POINT ( 'NONE', #3391 ) ;
#34772=ORIENTED_EDGE ( 'NONE', *, *, #21568, .F. ) ;
#34773=EDGE_CURVE ( 'NONE', #15209, #6733, #939, .T. ) ;
#34774=CARTESIAN_POINT ( 'NONE',  ( 11.99999662536862566, 86.60254037844397601, 17.49999999999999645 ) ) ;
#34775=ORIENTED_EDGE ( 'NONE', *, *, #1776, .T. ) ;
#34776=CARTESIAN_POINT ( 'NONE',  ( -80.00000337463094979, 17.32050807568878525, -9.999999999999998224 ) ) ;
#34778=ORIENTED_EDGE ( 'NONE', *, *, #27644, .T. ) ;
#34779=DIRECTION ( 'NONE',  ( 0.000000000000000000, 0.000000000000000000, 1.000000000000000000 ) ) ;
#34780=CARTESIAN_POINT ( 'NONE',  ( -43.00000337463111322, 60.62177826491077326, -5.000000000000000000 ) ) ;
#34781=DIRECTION ( 'NONE',  ( 1.000000000000000000, 0.000000000000000000, 0.000000000000000000 ) ) ;
#34782=AXIS2_PLACEMENT_3D ( 'NONE', #10857, #30904, #16131 ) ;
#34783=ADVANCED_FACE ( 'NONE', ( #9185 ), #6382, .F. ) ;
#34784=VERTEX_POINT ( 'NONE', #3039 ) ;
#34785=CARTESIAN_POINT ( 'NONE',  ( -58.88972745734203329, -33.99999999999965894, -49.86561046011506448 ) ) ;
#34787=DIRECTION ( 'NONE',  ( 0.000000000000000000, 0.000000000000000000, 1.000000000000000000 ) ) ;
#34788=EDGE_CURVE ( 'NONE', #33480, #12339, #25303, .T. ) ;
#34789=ORIENTED_EDGE ( 'NONE', *, *, #25021, .T. ) ;
#34790=DIRECTION ( 'NONE',  ( 0.000000000000000000, 0.000000000000000000, 1.000000000000000000 ) ) ;
#34791=CARTESIAN_POINT ( 'NONE',  ( -68.66839587347244844, -56.74224907229008608, 12.49999999999999645 ) ) ;
#34793=DIRECTION ( 'NONE',  ( 0.000000000000000000, 0.000000000000000000, 1.000000000000000000 ) ) ;
#34794=DIRECTION ( 'NONE',  ( 0.000000000000000000, 0.000000000000000000, -1.000000000000000000 ) ) ;
#34795=DIRECTION ( 'NONE',  ( 0.000000000000000000, 0.000000000000000000, 1.000000000000000000 ) ) ;
#34797=CARTESIAN_POINT ( 'NONE',  ( 44.99999662536851019, 77.94228634059959404, 17.49999999999999645 ) ) ;
#34798=DIRECTION ( 'NONE',  ( 0.000000000000000000, 0.000000000000000000, 1.000000000000000000 ) ) ;
#34799=ORIENTED_EDGE ( 'NONE', *, *, #32470, .T. ) ;
#34800=DIRECTION ( 'NONE',  ( -0.000000000000000000, -0.000000000000000000, 1.000000000000000000 ) ) ;
#34802=CARTESIAN_POINT ( 'NONE',  ( 46.99999662536851019, -60.62177826491080168, -9.999999999999998224 ) ) ;
#34803=ORIENTED_EDGE ( 'NONE', *, *, #25511, .F. ) ;
#34804=EDGE_CURVE ( 'NONE', #18782, #5564, #22323, .T. ) ;
#34805=ORIENTED_EDGE ( 'NONE', *, *, #3843, .T. ) ;
#34806=EDGE_LOOP ( 'NONE', ( #21376, #7777, #6378, #11986, #7103 ) ) ;
#34809=CARTESIAN_POINT ( 'NONE',  ( 74.99999662536835388, -25.98076211353319565, -5.000000000000000000 ) ) ;
#34810=DIRECTION ( 'NONE',  ( 0.000000000000000000, 0.000000000000000000, 1.000000000000000000 ) ) ;
#34811=EDGE_CURVE ( 'NONE', #2942, #553, #14554, .T. ) ;
#34812=CARTESIAN_POINT ( 'NONE',  ( 9.999996625368618552, 69.28203230275516944, -9.999999999999998224 ) ) ;
#34813=ORIENTED_EDGE ( 'NONE', *, *, #16587, .T. ) ;
#34814=EDGE_CURVE ( 'NONE', #29485, #12595, #4981, .T. ) ;
#34815=CARTESIAN_POINT ( 'NONE',  ( -60.00000337463108480, -51.96152422706641971, -9.999999999999998224 ) ) ;
#34817=FACE_BOUND ( 'NONE', #6362, .T. ) ;
#34818=CYLINDRICAL_SURFACE ( 'NONE', #17353, 2.000000000000000000 ) ;
#34819=CARTESIAN_POINT ( 'NONE',  ( 19.99999662536857770, 86.60254037844397601, -9.999999999999998224 ) ) ;
#34820=ORIENTED_EDGE ( 'NONE', *, *, #11528, .T. ) ;
#34822=CIRCLE ( 'NONE', #13266, 27.00000000000001776 ) ;
#34823=CARTESIAN_POINT ( 'NONE',  ( 59.29837256189581041, 31.02796211690886707, 12.49999999999999822 ) ) ;
#34824=EDGE_CURVE ( 'NONE', #27465, #6217, #28886, .T. ) ;
#34825=CARTESIAN_POINT ( 'NONE',  ( -65.00000337463102085, 60.62177826491077326, -9.999999999999998224 ) ) ;
#34826=CARTESIAN_POINT ( 'NONE',  ( -50.00000337463109190, 69.28203230275518365, 12.50000000000000000 ) ) ;
#34827=VERTEX_POINT ( 'NONE', #8830 ) ;
#34828=FACE_OUTER_BOUND ( 'NONE', #23251, .T. ) ;
#34830=CARTESIAN_POINT ( 'NONE',  ( 61.99999662536843914, -34.64101615137759893, -9.999999999999998224 ) ) ;
#34831=VERTEX_POINT ( 'NONE', #15190 ) ;
#34832=ORIENTED_EDGE ( 'NONE', *, *, #10813, .T. ) ;
#34834=ORIENTED_EDGE ( 'NONE', *, *, #21261, .F. ) ;
#34835=FACE_OUTER_BOUND ( 'NONE', #7075, .T. ) ;
#34837=ADVANCED_FACE ( 'NONE', ( #18013 ), #11814, .T. ) ;
#34839=CARTESIAN_POINT ( 'NONE',  ( -45.00000337463111322, 60.62177826491077326, -5.000000000000000000 ) ) ;
#34841=CIRCLE ( 'NONE', #9690, 2.000000000000001776 ) ;
#34842=CARTESIAN_POINT ( 'NONE',  ( -25.00000337463120914, 77.94228634059957983, -5.000000000000000000 ) ) ;
#34843=CARTESIAN_POINT ( 'NONE',  ( 3.499999999999991562, -55.00000000000000000, -5.000000000000000000 ) ) ;
#34845=EDGE_CURVE ( 'NONE', #21657, #16356, #32510, .T. ) ;
#34846=ORIENTED_EDGE ( 'NONE', *, *, #19894, .T. ) ;
#34847=CARTESIAN_POINT ( 'NONE',  ( -85.00000337463092137, 25.98076211353317433, -5.000000000000000000 ) ) ;
#34849=DIRECTION ( 'NONE',  ( 1.000000000000000000, 0.000000000000000000, 0.000000000000000000 ) ) ;
#34850=EDGE_CURVE ( 'NONE', #1195, #31600, #7364, .T. ) ;
#34851=VERTEX_POINT ( 'NONE', #6193 ) ;
#34852=EDGE_CURVE ( 'NONE', #19680, #15168, #31875, .T. ) ;
#34853=FACE_BOUND ( 'NONE', #11519, .T. ) ;
#34854=EDGE_LOOP ( 'NONE', ( #15076, #24946 ) ) ;
#34857=EDGE_LOOP ( 'NONE', ( #19462, #32383, #12687, #32513, #16270 ) ) ;
#34858=EDGE_CURVE ( 'NONE', #13344, #23066, #29509, .T. ) ;
#34860=ADVANCED_FACE ( 'NONE', ( #751 ), #35076, .F. ) ;
#34861=CARTESIAN_POINT ( 'NONE',  ( -85.00000337463092137, 8.660254037844389075, 12.50000000000000000 ) ) ;
#34862=ADVANCED_FACE ( 'NONE', ( #26623 ), #20077, .F. ) ;
#34864=DIRECTION ( 'NONE',  ( -0.000000000000000000, 0.000000000000000000, -1.000000000000000000 ) ) ;
#34865=CARTESIAN_POINT ( 'NONE',  ( -2.778182860043013847, -66.86787810013035482, 12.49999999999999822 ) ) ;
#34866=EDGE_CURVE ( 'NONE', #22384, #24412, #8567, .T. ) ;
#34867=VERTEX_POINT ( 'NONE', #35284 ) ;
#34868=EDGE_CURVE ( 'NONE', #7368, #10592, #26520, .T. ) ;
#34870=ORIENTED_EDGE ( 'NONE', *, *, #31663, .T. ) ;
#34871=VERTEX_POINT ( 'NONE', #30369 ) ;
#34872=ORIENTED_EDGE ( 'NONE', *, *, #32549, .F. ) ;
#34873=FACE_OUTER_BOUND ( 'NONE', #35172, .T. ) ;
#34878=CARTESIAN_POINT ( 'NONE',  ( 84.99999662536831124, -8.660254037844397956, -5.000000000000000000 ) ) ;
#34879=ORIENTED_EDGE ( 'NONE', *, *, #15939, .F. ) ;
#34880=DIRECTION ( 'NONE',  ( 0.000000000000000000, 0.000000000000000000, -1.000000000000000000 ) ) ;
#34883=VECTOR ( 'NONE', #19727, 1000.000000000000000 ) ;
#34884=CARTESIAN_POINT ( 'NONE',  ( 69.13212189986965939, 2.778182860042805125, -49.86348611802629449 ) ) ;
#34885=CARTESIAN_POINT ( 'NONE',  ( -80.00000337463096400, -34.64101615137762025, -5.000000000000000000 ) ) ;
#34886=EDGE_LOOP ( 'NONE', ( #7150, #32064, #23493, #16554 ) ) ;
#34887=CARTESIAN_POINT ( 'NONE',  ( 54.99999662536846046, -43.30127018922200222, 17.49999999999999645 ) ) ;
#34888=DIRECTION ( 'NONE',  ( 0.000000000000000000, 0.000000000000000000, 1.000000000000000000 ) ) ;
#34889=ORIENTED_EDGE ( 'NONE', *, *, #11484, .F. ) ;
#34890=ORIENTED_EDGE ( 'NONE', *, *, #26567, .F. ) ;
#34891=DIRECTION ( 'NONE',  ( 1.000000000000000000, 0.000000000000000000, 0.000000000000000000 ) ) ;
#34895=CYLINDRICAL_SURFACE ( 'NONE', #19678, 2.000000000000001776 ) ;
#34896=EDGE_LOOP ( 'NONE', ( #36519, #35558 ) ) ;
#34898=CARTESIAN_POINT ( 'NONE',  ( -63.00000337463102085, 43.30127018922198801, -9.999999999999998224 ) ) ;
#34900=ORIENTED_EDGE ( 'NONE', *, *, #21551, .T. ) ;
#34902=VERTEX_POINT ( 'NONE', #7317 ) ;
#34903=DIRECTION ( 'NONE',  ( 0.000000000000000000, 0.000000000000000000, -1.000000000000000000 ) ) ;
#34904=EDGE_CURVE ( 'NONE', #8445, #19786, #16945, .T. ) ;
#34905=CIRCLE ( 'NONE', #1361, 2.000000000000000000 ) ;
#34906=CARTESIAN_POINT ( 'NONE',  ( -68.19171733629717380, 52.81598405851951838, 12.50000000000000000 ) ) ;
#34907=EDGE_CURVE ( 'NONE', #111, #21657, #10360, .T. ) ;
#34908=DIRECTION ( 'NONE',  ( 0.000000000000000000, 0.000000000000000000, 1.000000000000000000 ) ) ;
#34909=EDGE_CURVE ( 'NONE', #32638, #11718, #27719, .T. ) ;
#34910=VERTEX_POINT ( 'NONE', #13132 ) ;
#34911=EDGE_LOOP ( 'NONE', ( #31602, #29761 ) ) ;
#34913=DIRECTION ( 'NONE',  ( 0.000000000000000000, 0.000000000000000000, 1.000000000000000000 ) ) ;
#34915=ORIENTED_EDGE ( 'NONE', *, *, #11731, .F. ) ;
#34916=CARTESIAN_POINT ( 'NONE',  ( -77.00000337463097821, 8.660254037844374864, -5.000000000000000000 ) ) ;
#34917=AXIS2_PLACEMENT_3D ( 'NONE', #12246, #18656, #35913 ) ;
#34918=FACE_BOUND ( 'NONE', #20992, .T. ) ;
#34919=CARTESIAN_POINT ( 'NONE',  ( -73.00000337463097821, 43.30127018922197379, -9.999999999999998224 ) ) ;
#34920=CARTESIAN_POINT ( 'NONE',  ( 66.86787810013036903, -2.778182860042780700, -49.86348611802629449 ) ) ;
#34921=DIRECTION ( 'NONE',  ( 0.000000000000000000, 0.000000000000000000, 1.000000000000000000 ) ) ;
#34922=ORIENTED_EDGE ( 'NONE', *, *, #7435, .T. ) ;
#34924=LINE ( 'NONE', #783, #24776 ) ;
#34925=ORIENTED_EDGE ( 'NONE', *, *, #34972, .T. ) ;
#34926=DIRECTION ( 'NONE',  ( 1.000000000000000000, 0.000000000000000000, 0.000000000000000000 ) ) ;
#34927=DIRECTION ( 'NONE',  ( 0.000000000000000000, 0.000000000000000000, 1.000000000000000000 ) ) ;
#34928=LINE ( 'NONE', #3435, #31747 ) ;
#34929=EDGE_CURVE ( 'NONE', #12570, #31248, #15941, .T. ) ;
#34930=VERTEX_POINT ( 'NONE', #15753 ) ;
#34931=AXIS2_PLACEMENT_3D ( 'NONE', #11768, #23031, #3543 ) ;
#34932=ORIENTED_EDGE ( 'NONE', *, *, #28914, .F. ) ;
#34933=ORIENTED_EDGE ( 'NONE', *, *, #28978, .F. ) ;
#34934=DIRECTION ( 'NONE',  ( 0.000000000000000000, 0.000000000000000000, 1.000000000000000000 ) ) ;
#34935=DIRECTION ( 'NONE',  ( 0.000000000000000000, 0.000000000000000000, 1.000000000000000000 ) ) ;
#34937=ORIENTED_EDGE ( 'NONE', *, *, #29511, .T. ) ;
#34938=ORIENTED_EDGE ( 'NONE', *, *, #5453, .F. ) ;
#34939=VECTOR ( 'NONE', #37048, 1000.000000000000000 ) ;
#34940=EDGE_CURVE ( 'NONE', #30390, #16972, #15577, .T. ) ;
#34941=CARTESIAN_POINT ( 'NONE',  ( 59.99999662536843914, -34.64101615137759893, -9.999999999999998224 ) ) ;
#34942=CIRCLE ( 'NONE', #1399, 2.000000000000001776 ) ;
#34945=EDGE_LOOP ( 'NONE', ( #33573, #1826 ) ) ;
#34946=DIRECTION ( 'NONE',  ( 0.000000000000000000, 0.000000000000000000, 1.000000000000000000 ) ) ;
#34947=EDGE_LOOP ( 'NONE', ( #10580, #13824, #14401, #32528 ) ) ;
#34948=AXIS2_PLACEMENT_3D ( 'NONE', #23170, #2736, #14538 ) ;
#34951=DIRECTION ( 'NONE',  ( 0.000000000000000000, 0.000000000000000000, -1.000000000000000000 ) ) ;
#34954=VERTEX_POINT ( 'NONE', #21008 ) ;
#34955=EDGE_LOOP ( 'NONE', ( #11478, #33911 ) ) ;
#34956=CYLINDRICAL_SURFACE ( 'NONE', #14898, 2.000000000000001776 ) ;
#34957=AXIS2_PLACEMENT_3D ( 'NONE', #15057, #12413, #26484 ) ;
#34958=CARTESIAN_POINT ( 'NONE',  ( -56.29165124598824832, 32.50000000000046896, 12.49999999999999822 ) ) ;
#34959=CARTESIAN_POINT ( 'NONE',  ( -15.97563234535668109, 90.60231327712331506, 12.49999999999999822 ) ) ;
#34960=AXIS2_PLACEMENT_3D ( 'NONE', #30120, #4448, #36135 ) ;
#34961=EDGE_LOOP ( 'NONE', ( #14630, #10040 ) ) ;
#34962=CARTESIAN_POINT ( 'NONE',  ( 46.99999662536849598, -77.94228634059960825, 17.49999999999999645 ) ) ;
#34963=DIRECTION ( 'NONE',  ( 0.000000000000000000, 0.000000000000000000, 1.000000000000000000 ) ) ;
#34964=ORIENTED_EDGE ( 'NONE', *, *, #18867, .T. ) ;
#34966=CYLINDRICAL_SURFACE ( 'NONE', #9502, 2.000000000000001776 ) ;
#34970=DIRECTION ( 'NONE',  ( 0.000000000000000000, 0.000000000000000000, 1.000000000000000000 ) ) ;
#34972=EDGE_CURVE ( 'NONE', #12226, #21994, #9140, .T. ) ;
#34973=CARTESIAN_POINT ( 'NONE',  ( -88.00000337463090716, -1.040834085586084257E-14, -9.999999999999998224 ) ) ;
#34974=ORIENTED_EDGE ( 'NONE', *, *, #34858, .T. ) ;
#34975=CYLINDRICAL_SURFACE ( 'NONE', #7630, 2.000000000000001776 ) ;
#34977=DIRECTION ( 'NONE',  ( -1.000000000000000000, 0.000000000000000000, -0.000000000000000000 ) ) ;
#34978=EDGE_CURVE ( 'NONE', #25502, #6568, #3155, .T. ) ;
#34980=VERTEX_POINT ( 'NONE', #18754 ) ;
#34981=ORIENTED_EDGE ( 'NONE', *, *, #10090, .F. ) ;
#34983=DIRECTION ( 'NONE',  ( 0.000000000000000000, 0.000000000000000000, 1.000000000000000000 ) ) ;
#34984=EDGE_CURVE ( 'NONE', #25888, #17256, #1138, .T. ) ;
#34985=CARTESIAN_POINT ( 'NONE',  ( 76.99999662536835388, -25.98076211353319565, -9.999999999999998224 ) ) ;
#34986=AXIS2_PLACEMENT_3D ( 'NONE', #31321, #28872, #28160 ) ;
#34987=LINE ( 'NONE', #14234, #27019 ) ;
#34989=DIRECTION ( 'NONE',  ( 1.000000000000000000, 0.000000000000000000, 0.000000000000000000 ) ) ;
#34990=VERTEX_POINT ( 'NONE', #7141 ) ;
#34991=CARTESIAN_POINT ( 'NONE',  ( 46.99999662536851019, -60.62177826491080168, -9.999999999999998224 ) ) ;
#34992=VERTEX_POINT ( 'NONE', #1314 ) ;
#34993=FACE_BOUND ( 'NONE', #15629, .T. ) ;
#34996=DIRECTION ( 'NONE',  ( 0.000000000000000000, 0.000000000000000000, 1.000000000000000000 ) ) ;
#34997=ADVANCED_FACE ( 'NONE', ( #7496 ), #33174, .F. ) ;
#34998=ORIENTED_EDGE ( 'NONE', *, *, #7338, .F. ) ;
#34999=CARTESIAN_POINT ( 'NONE',  ( 44.99999662536849598, -77.94228634059960825, 17.49999999999999645 ) ) ;
#35003=DIRECTION ( 'NONE',  ( 0.000000000000000000, 0.000000000000000000, 1.000000000000000000 ) ) ;
#35004=EDGE_LOOP ( 'NONE', ( #20213, #25277 ) ) ;
#35005=CARTESIAN_POINT ( 'NONE',  ( -57.00000337463107059, 43.30127018922197379, -9.999999999999998224 ) ) ;
#35006=CIRCLE ( 'NONE', #9865, 2.000000000000001776 ) ;
#35008=DIRECTION ( 'NONE',  ( 1.000000000000000000, 0.000000000000000000, 0.000000000000000000 ) ) ;
#35009=EDGE_CURVE ( 'NONE', #9788, #12832, #3938, .T. ) ;
#35010=ORIENTED_EDGE ( 'NONE', *, *, #13573, .F. ) ;
#35013=EDGE_CURVE ( 'NONE', #27668, #5018, #3765, .T. ) ;
#35014=ORIENTED_EDGE ( 'NONE', *, *, #9858, .F. ) ;
#35015=DIRECTION ( 'NONE',  ( 0.000000000000000000, 0.000000000000000000, 1.000000000000000000 ) ) ;
#35016=EDGE_CURVE ( 'NONE', #29281, #35919, #15741, .T. ) ;
#35017=CARTESIAN_POINT ( 'NONE',  ( -90.00000337463090716, -1.040834085586084257E-14, 17.49999999999999645 ) ) ;
#35018=ORIENTED_EDGE ( 'NONE', *, *, #26011, .F. ) ;
#35019=AXIS2_PLACEMENT_3D ( 'NONE', #22850, #34285, #8587 ) ;
#35020=DIRECTION ( 'NONE',  ( 1.000000000000000000, 0.000000000000000000, 0.000000000000000000 ) ) ;
#35022=EDGE_CURVE ( 'NONE', #4407, #12415, #6940, .T. ) ;
#35023=FACE_OUTER_BOUND ( 'NONE', #2998, .T. ) ;
#35024=ORIENTED_EDGE ( 'NONE', *, *, #7129, .F. ) ;
#35025=VERTEX_POINT ( 'NONE', #24387 ) ;
#35027=EDGE_CURVE ( 'NONE', #11389, #18782, #10943, .T. ) ;
#35029=ORIENTED_EDGE ( 'NONE', *, *, #11879, .T. ) ;
#35030=VECTOR ( 'NONE', #21080, 1000.000000000000000 ) ;
#35031=DIRECTION ( 'NONE',  ( 1.000000000000000000, 0.000000000000000000, 0.000000000000000000 ) ) ;
#35032=ORIENTED_EDGE ( 'NONE', *, *, #5477, .F. ) ;
#35033=PLANE ( 'NONE',  #1154 ) ;
#35035=EDGE_LOOP ( 'NONE', ( #13863, #35542, #10864 ) ) ;
#35036=LINE ( 'NONE', #6719, #14635 ) ;
#35037=ORIENTED_EDGE ( 'NONE', *, *, #1047, .T. ) ;
#35040=CIRCLE ( 'NONE', #29645, 2.000000000000000000 ) ;
#35041=DIRECTION ( 'NONE',  ( 0.000000000000000000, 0.000000000000000000, 1.000000000000000000 ) ) ;
#35042=EDGE_CURVE ( 'NONE', #23091, #33432, #33747, .T. ) ;
#35043=CARTESIAN_POINT ( 'NONE',  ( -2.000003374631334818, 69.28203230275516944, 12.50000000000000000 ) ) ;
#35044=PLANE ( 'NONE',  #19088 ) ;
#35045=ORIENTED_EDGE ( 'NONE', *, *, #5078, .F. ) ;
#35046=ORIENTED_EDGE ( 'NONE', *, *, #22881, .T. ) ;
#35047=ORIENTED_EDGE ( 'NONE', *, *, #36264, .F. ) ;
#35048=EDGE_CURVE ( 'NONE', #14051, #36367, #33707, .T. ) ;
#35049=ORIENTED_EDGE ( 'NONE', *, *, #17447, .F. ) ;
#35051=AXIS2_PLACEMENT_3D ( 'NONE', #15683, #10059, #21497 ) ;
#35052=CARTESIAN_POINT ( 'NONE',  ( -25.00000337463121980, -77.94228634059963667, -9.999999999999998224 ) ) ;
#35053=EDGE_CURVE ( 'NONE', #10733, #35776, #34905, .T. ) ;
#35054=DIRECTION ( 'NONE',  ( 1.000000000000000000, 0.000000000000000000, 0.000000000000000000 ) ) ;
#35055=VERTEX_POINT ( 'NONE', #34129 ) ;
#35056=VECTOR ( 'NONE', #32286, 1000.000000000000000 ) ;
#35057=EDGE_CURVE ( 'NONE', #9552, #30244, #25140, .T. ) ;
#35058=CARTESIAN_POINT ( 'NONE',  ( -60.00000337463104216, 34.64101615137757051, 17.49999999999999645 ) ) ;
#35060=DIRECTION ( 'NONE',  ( 0.000000000000000000, 0.000000000000000000, 1.000000000000000000 ) ) ;
#35061=CIRCLE ( 'NONE', #21890, 2.000000000000001776 ) ;
#35065=DIRECTION ( 'NONE',  ( 0.000000000000000000, 0.000000000000000000, 1.000000000000000000 ) ) ;
#35066=DIRECTION ( 'NONE',  ( 1.000000000000000000, 0.000000000000000000, 0.000000000000000000 ) ) ;
#35067=VERTEX_POINT ( 'NONE', #33575 ) ;
#35068=DIRECTION ( 'NONE',  ( 0.000000000000000000, 0.000000000000000000, 1.000000000000000000 ) ) ;
#35069=DIRECTION ( 'NONE',  ( 0.000000000000000000, 0.000000000000000000, 1.000000000000000000 ) ) ;
#35070=AXIS2_PLACEMENT_3D ( 'NONE', #21499, #18864, #32937 ) ;
#35072=VECTOR ( 'NONE', #1633, 1000.000000000000000 ) ;
#35075=EDGE_CURVE ( 'NONE', #15938, #2053, #30105, .T. ) ;
#35076=CYLINDRICAL_SURFACE ( 'NONE', #28304, 2.000000000000001776 ) ;
#35077=DIRECTION ( 'NONE',  ( -1.000000000000000000, 0.000000000000000000, 0.000000000000000000 ) ) ;
#35078=FACE_OUTER_BOUND ( 'NONE', #9888, .T. ) ;
#35082=AXIS2_PLACEMENT_3D ( 'NONE', #11483, #30797, #10933 ) ;
#35083=ORIENTED_EDGE ( 'NONE', *, *, #15853, .T. ) ;
#35084=VECTOR ( 'NONE', #11443, 1000.000000000000000 ) ;
#35085=LINE ( 'NONE', #29267, #27947 ) ;
#35086=VERTEX_POINT ( 'NONE', #30915 ) ;
#35087=AXIS2_PLACEMENT_3D ( 'NONE', #34839, #9135, #704 ) ;
#35088=CIRCLE ( 'NONE', #8138, 2.000000000000001776 ) ;
#35090=CARTESIAN_POINT ( 'NONE',  ( -52.39915983220772233, -35.19434990244957362, -4.999999999999997335 ) ) ;
#35091=AXIS2_PLACEMENT_3D ( 'NONE', #5688, #16777, #30636 ) ;
#35094=EDGE_CURVE ( 'NONE', #7314, #13283, #17033, .T. ) ;
#35095=DIRECTION ( 'NONE',  ( 0.000000000000000000, 0.000000000000000000, 1.000000000000000000 ) ) ;
#35096=ORIENTED_EDGE ( 'NONE', *, *, #22290, .F. ) ;
#35098=ORIENTED_EDGE ( 'NONE', *, *, #7277, .F. ) ;
#35099=AXIS2_PLACEMENT_3D ( 'NONE', #1823, #10630, #4994 ) ;
#35100=CARTESIAN_POINT ( 'NONE',  ( -75.00000337463099243, -25.98076211353322051, -9.999999999999998224 ) ) ;
#35102=AXIS2_PLACEMENT_3D ( 'NONE', #15712, #1451, #12884 ) ;
#35103=DIRECTION ( 'NONE',  ( 0.000000000000000000, 0.000000000000000000, 1.000000000000000000 ) ) ;
#35104=EDGE_CURVE ( 'NONE', #19401, #630, #2576, .T. ) ;
#35105=ORIENTED_EDGE ( 'NONE', *, *, #18611, .F. ) ;
#35106=DIRECTION ( 'NONE',  ( 0.000000000000000000, 0.000000000000000000, 1.000000000000000000 ) ) ;
#35107=CARTESIAN_POINT ( 'NONE',  ( 54.99999662536844625, 60.62177826491077326, -9.999999999999998224 ) ) ;
#35108=EDGE_CURVE ( 'NONE', #7505, #34871, #2594, .T. ) ;
#35110=CARTESIAN_POINT ( 'NONE',  ( -4.279621169095561228, 62.97617850287782915, -4.999999999999997335 ) ) ;
#35113=CARTESIAN_POINT ( 'NONE',  ( -59.13646009116099833, 70.47608876694653190, -49.22241343995295892 ) ) ;
#35114=VECTOR ( 'NONE', #32329, 1000.000000000000000 ) ;
#35115=DIRECTION ( 'NONE',  ( 1.000000000000000000, 0.000000000000000000, 0.000000000000000000 ) ) ;
#35117=VERTEX_POINT ( 'NONE', #19315 ) ;
#35118=DIRECTION ( 'NONE',  ( 1.000000000000000000, 0.000000000000000000, 0.000000000000000000 ) ) ;
#35121=CARTESIAN_POINT ( 'NONE',  ( -52.39915983220772233, -35.19434990244957362, 12.49999999999999822 ) ) ;
#35122=CIRCLE ( 'NONE', #28519, 2.000000000000001776 ) ;
#35123=ADVANCED_FACE ( 'NONE', ( #22305 ), #5252, .F. ) ;
#35124=AXIS2_PLACEMENT_3D ( 'NONE', #15315, #15132, #26760 ) ;
#35125=ORIENTED_EDGE ( 'NONE', *, *, #13908, .T. ) ;
#35126=AXIS2_PLACEMENT_3D ( 'NONE', #14071, #31154, #28155 ) ;
#35127=EDGE_CURVE ( 'NONE', #9816, #8706, #28333, .T. ) ;
#35128=VERTEX_POINT ( 'NONE', #27732 ) ;
#35129=VECTOR ( 'NONE', #25970, 1000.000000000000000 ) ;
#35130=VERTEX_POINT ( 'NONE', #2046 ) ;
#35131=EDGE_CURVE ( 'NONE', #11035, #9484, #24765, .T. ) ;
#35132=EDGE_CURVE ( 'NONE', #5473, #32493, #24165, .T. ) ;
#35133=CARTESIAN_POINT ( 'NONE',  ( -75.00000337463097821, 43.30127018922197379, -9.999999999999998224 ) ) ;
#35136=VERTEX_POINT ( 'NONE', #5439 ) ;
#35137=ORIENTED_EDGE ( 'NONE', *, *, #5978, .F. ) ;
#35138=EDGE_LOOP ( 'NONE', ( #22475, #8844, #5446, #14420 ) ) ;
#35139=DIRECTION ( 'NONE',  ( 1.000000000000000000, 0.000000000000000000, 0.000000000000000000 ) ) ;
#35140=ORIENTED_EDGE ( 'NONE', *, *, #24375, .F. ) ;
#35143=CARTESIAN_POINT ( 'NONE',  ( -22.00000337463124112, -69.28203230275522628, -9.999999999999998224 ) ) ;
#35144=ORIENTED_EDGE ( 'NONE', *, *, #30468, .T. ) ;
#35145=VECTOR ( 'NONE', #27800, 1000.000000000000000 ) ;
#35146=EDGE_LOOP ( 'NONE', ( #12054, #7545, #24042, #26560 ) ) ;
#35147=FACE_OUTER_BOUND ( 'NONE', #14592, .T. ) ;
#35148=DIRECTION ( 'NONE',  ( 1.000000000000000000, 0.000000000000000000, 0.000000000000000000 ) ) ;
#35150=EDGE_LOOP ( 'NONE', ( #22661, #9360, #34126, #30101 ) ) ;
#35151=EDGE_LOOP ( 'NONE', ( #5455, #26421, #3299 ) ) ;
#35155=AXIS2_PLACEMENT_3D ( 'NONE', #12679, #4640, #7077 ) ;
#35156=EDGE_CURVE ( 'NONE', #35412, #18409, #16865, .T. ) ;
#35158=CARTESIAN_POINT ( 'NONE',  ( -40.00000337463113453, 69.28203230275516944, -5.000000000000000000 ) ) ;
#35159=CARTESIAN_POINT ( 'NONE',  ( 4.999996625368676284, -77.94228634059960825, -9.999999999999998224 ) ) ;
#35160=CIRCLE ( 'NONE', #7017, 2.000000000000001776 ) ;
#35161=ORIENTED_EDGE ( 'NONE', *, *, #24113, .F. ) ;
#35162=CARTESIAN_POINT ( 'NONE',  ( 1.999996625368672287, 86.60254037844397601, 17.49999999999999645 ) ) ;
#35164=EDGE_LOOP ( 'NONE', ( #20788, #30605 ) ) ;
#35165=DIRECTION ( 'NONE',  ( 1.000000000000000000, 0.000000000000000000, 0.000000000000000000 ) ) ;
#35166=DIRECTION ( 'NONE',  ( 1.000000000000000000, 0.000000000000000000, 0.000000000000000000 ) ) ;
#35167=CARTESIAN_POINT ( 'NONE',  ( -87.00000337463093558, -8.660254037844422825, -5.000000000000000000 ) ) ;
#35169=VECTOR ( 'NONE', #18594, 1000.000000000000000 ) ;
#35170=DIRECTION ( 'NONE',  ( 1.000000000000000000, 0.000000000000000000, 0.000000000000000000 ) ) ;
#35171=DIRECTION ( 'NONE',  ( 1.000000000000000000, 0.000000000000000000, 0.000000000000000000 ) ) ;
#35172=EDGE_LOOP ( 'NONE', ( #17251, #736, #30546, #17007 ) ) ;
#35174=AXIS2_PLACEMENT_3D ( 'NONE', #13613, #33859, #2379 ) ;
#35176=CARTESIAN_POINT ( 'NONE',  ( 62.33939050065184517, -13.89091430021398565, 12.49999999999999822 ) ) ;
#35177=AXIS2_PLACEMENT_3D ( 'NONE', #10438, #33324, #4647 ) ;
#35178=AXIS2_PLACEMENT_3D ( 'NONE', #4904, #10517, #30754 ) ;
#35179=ORIENTED_EDGE ( 'NONE', *, *, #2958, .F. ) ;
#35180=ORIENTED_EDGE ( 'NONE', *, *, #31984, .F. ) ;
#35181=EDGE_LOOP ( 'NONE', ( #6792, #11414, #29412, #31319 ) ) ;
#35182=AXIS2_PLACEMENT_3D ( 'NONE', #29514, #27080, #23533 ) ;
#35184=CARTESIAN_POINT ( 'NONE',  ( 54.99999662536844625, -60.62177826491080168, -5.000000000000000000 ) ) ;
#35185=CARTESIAN_POINT ( 'NONE',  ( -60.00000337463107059, -34.64101615137762025, -9.999999999999998224 ) ) ;
#35187=CARTESIAN_POINT ( 'NONE',  ( 67.99999662536838230, -17.32050807568879947, -5.000000000000000000 ) ) ;
#35189=DIRECTION ( 'NONE',  ( 0.000000000000000000, 0.000000000000000000, 1.000000000000000000 ) ) ;
#35191=VERTEX_POINT ( 'NONE', #13302 ) ;
#35192=DIRECTION ( 'NONE',  ( 0.000000000000000000, 0.000000000000000000, 1.000000000000000000 ) ) ;
#35193=ORIENTED_EDGE ( 'NONE', *, *, #1192, .F. ) ;
#35194=FACE_BOUND ( 'NONE', #27006, .T. ) ;
#35195=VECTOR ( 'NONE', #17560, 1000.000000000000000 ) ;
#35197=AXIS2_PLACEMENT_3D ( 'NONE', #13631, #25780, #3082 ) ;
#35200=FACE_OUTER_BOUND ( 'NONE', #20463, .T. ) ;
#35201=CIRCLE ( 'NONE', #7062, 33.00000000000002132 ) ;
#35203=EDGE_CURVE ( 'NONE', #30254, #1072, #5007, .T. ) ;
#35205=EDGE_CURVE ( 'NONE', #31374, #6244, #30127, .T. ) ;
#35206=AXIS2_PLACEMENT_3D ( 'NONE', #31261, #128, #22656 ) ;
#35207=CARTESIAN_POINT ( 'NONE',  ( 82.99999662536832545, 25.98076211353319565, 17.49999999999999645 ) ) ;
#35208=CIRCLE ( 'NONE', #23822, 2.000000000000001776 ) ;
#35209=CYLINDRICAL_SURFACE ( 'NONE', #14956, 3.499999999999989342 ) ;
#35210=CARTESIAN_POINT ( 'NONE',  ( -65.00000337463106348, -60.62177826491083010, -9.999999999999998224 ) ) ;
#35213=DIRECTION ( 'NONE',  ( 1.000000000000000000, 0.000000000000000000, 0.000000000000000000 ) ) ;
#35216=VECTOR ( 'NONE', #20868, 1000.000000000000000 ) ;
#35217=EDGE_LOOP ( 'NONE', ( #3412, #21091, #20448, #16272, #7619, #28240, #15516, #7956, #14087, #29960, #22500, #25148, #11920 ) ) ;
#35218=CIRCLE ( 'NONE', #23210, 33.00000000000001421 ) ;
#35220=ORIENTED_EDGE ( 'NONE', *, *, #34102, .F. ) ;
#35224=CARTESIAN_POINT ( 'NONE',  ( 56.52018970185260116, -35.83991598322081273, -4.999999999999997335 ) ) ;
#35225=AXIS2_PLACEMENT_3D ( 'NONE', #11301, #22750, #33627 ) ;
#35226=ADVANCED_FACE ( 'NONE', ( #20404 ), #17972, .F. ) ;
#35227=DIRECTION ( 'NONE',  ( 0.000000000000000000, 0.000000000000000000, 1.000000000000000000 ) ) ;
#35228=DIRECTION ( 'NONE',  ( 0.000000000000000000, 0.000000000000000000, 1.000000000000000000 ) ) ;
#35230=AXIS2_PLACEMENT_3D ( 'NONE', #21407, #21602, #24210 ) ;
#35231=DIRECTION ( 'NONE',  ( 0.000000000000000000, 0.000000000000000000, 1.000000000000000000 ) ) ;
#35232=ORIENTED_EDGE ( 'NONE', *, *, #34648, .F. ) ;
#35233=CIRCLE ( 'NONE', #37022, 2.000000000000001776 ) ;
#35234=ORIENTED_EDGE ( 'NONE', *, *, #18065, .F. ) ;
#35236=VECTOR ( 'NONE', #19720, 1000.000000000000000 ) ;
#35237=DIRECTION ( 'NONE',  ( -0.8660254037844449249, -0.4999999999999888978, 0.000000000000000000 ) ) ;
#35238=VERTEX_POINT ( 'NONE', #23415 ) ;
#35240=VERTEX_POINT ( 'NONE', #6152 ) ;
#35241=AXIS2_PLACEMENT_3D ( 'NONE', #30169, #21572, #32998 ) ;
#35242=FACE_BOUND ( 'NONE', #20953, .T. ) ;
#35243=ORIENTED_EDGE ( 'NONE', *, *, #9288, .F. ) ;
#35244=VERTEX_POINT ( 'NONE', #2802 ) ;
#35245=EDGE_CURVE ( 'NONE', #12872, #26254, #17549, .T. ) ;
#35252=VECTOR ( 'NONE', #20585, 1000.000000000000000 ) ;
#35254=LINE ( 'NONE', #32410, #36481 ) ;
#35255=ORIENTED_EDGE ( 'NONE', *, *, #27718, .T. ) ;
#35256=ORIENTED_EDGE ( 'NONE', *, *, #31274, .F. ) ;
#35259=ORIENTED_EDGE ( 'NONE', *, *, #155, .F. ) ;
#35260=ORIENTED_EDGE ( 'NONE', *, *, #28573, .F. ) ;
#35261=EDGE_CURVE ( 'NONE', #10755, #2344, #12746, .T. ) ;
#35262=AXIS2_PLACEMENT_3D ( 'NONE', #31986, #35227, #32390 ) ;
#35264=CARTESIAN_POINT ( 'NONE',  ( -65.00000337463106348, -60.62177826491083010, 12.50000000000000000 ) ) ;
#35265=CARTESIAN_POINT ( 'NONE',  ( -30.89873480577614018, 67.49533652152319974, -5.000000000000000000 ) ) ;
#35266=ORIENTED_EDGE ( 'NONE', *, *, #4165, .F. ) ;
#35267=DIRECTION ( 'NONE',  ( -1.000000000000000000, 0.000000000000000000, 0.000000000000000000 ) ) ;
#35269=CARTESIAN_POINT ( 'NONE',  ( -55.00000337463109901, -60.62177826491083010, 12.50000000000000000 ) ) ;
#35271=ORIENTED_EDGE ( 'NONE', *, *, #29672, .T. ) ;
#35273=VECTOR ( 'NONE', #8323, 1000.000000000000000 ) ;
#35274=DIRECTION ( 'NONE',  ( 0.000000000000000000, 0.000000000000000000, 1.000000000000000000 ) ) ;
#35276=VERTEX_POINT ( 'NONE', #17416 ) ;
#35277=CARTESIAN_POINT ( 'NONE',  ( -85.00000337463092137, 8.660254037844389075, -9.999999999999998224 ) ) ;
#35278=CARTESIAN_POINT ( 'NONE',  ( -22.00000337463124112, -69.28203230275522628, -9.999999999999998224 ) ) ;
#35279=VERTEX_POINT ( 'NONE', #17582 ) ;
#35281=EDGE_CURVE ( 'NONE', #29968, #13826, #31655, .T. ) ;
#35282=LINE ( 'NONE', #32250, #5085 ) ;
#35283=AXIS2_PLACEMENT_3D ( 'NONE', #33718, #24726, #25282 ) ;
#35284=CARTESIAN_POINT ( 'NONE',  ( -72.00000337463100664, 34.64101615137758472, -5.000000000000000000 ) ) ;
#35285=CYLINDRICAL_SURFACE ( 'NONE', #9060, 2.000000000000001776 ) ;
#35286=FACE_OUTER_BOUND ( 'NONE', #10392, .T. ) ;
#35287=VERTEX_POINT ( 'NONE', #22860 ) ;
#35288=AXIS2_PLACEMENT_3D ( 'NONE', #3265, #29324, #17695 ) ;
#35289=ADVANCED_FACE ( 'NONE', ( #29008 ), #2994, .T. ) ;
#35292=ORIENTED_EDGE ( 'NONE', *, *, #21431, .F. ) ;
#35293=AXIS2_PLACEMENT_3D ( 'NONE', #34941, #14134, #19949 ) ;
#35294=EDGE_CURVE ( 'NONE', #5247, #26842, #23551, .T. ) ;
#35296=EDGE_LOOP ( 'NONE', ( #19973, #12186 ) ) ;
#35297=AXIS2_PLACEMENT_3D ( 'NONE', #9333, #23784, #3343 ) ;
#35298=DIRECTION ( 'NONE',  ( 0.000000000000000000, 0.000000000000000000, 1.000000000000000000 ) ) ;
#35299=CARTESIAN_POINT ( 'NONE',  ( -56.13646009116099123, 70.47608876694653190, -4.999999999999997335 ) ) ;
#35301=DIRECTION ( 'NONE',  ( 0.000000000000000000, 0.000000000000000000, 1.000000000000000000 ) ) ;
#35302=EDGE_LOOP ( 'NONE', ( #14372, #18161, #22284, #23250 ) ) ;
#35303=CIRCLE ( 'NONE', #23325, 1.999999999999998224 ) ;
#35304=ORIENTED_EDGE ( 'NONE', *, *, #5477, .T. ) ;
#35305=DIRECTION ( 'NONE',  ( -1.000000000000000000, 0.000000000000000000, 0.000000000000000000 ) ) ;
#35307=ORIENTED_EDGE ( 'NONE', *, *, #1528, .T. ) ;
#35310=DIRECTION ( 'NONE',  ( 1.000000000000000000, 0.000000000000000000, 0.000000000000000000 ) ) ;
#35311=AXIS2_PLACEMENT_3D ( 'NONE', #24159, #34864, #35610 ) ;
#35312=CARTESIAN_POINT ( 'NONE',  ( -50.00000337463109190, 69.28203230275518365, -9.999999999999998224 ) ) ;
#35314=CYLINDRICAL_SURFACE ( 'NONE', #6347, 2.000000000000001776 ) ;
#35315=ORIENTED_EDGE ( 'NONE', *, *, #29334, .F. ) ;
#35316=FACE_OUTER_BOUND ( 'NONE', #25312, .T. ) ;
#35318=DIRECTION ( 'NONE',  ( -0.000000000000000000, -0.000000000000000000, 1.000000000000000000 ) ) ;
#35319=VERTEX_POINT ( 'NONE', #14233 ) ;
#35320=DIRECTION ( 'NONE',  ( 0.000000000000000000, 0.000000000000000000, 1.000000000000000000 ) ) ;
#35323=AXIS2_PLACEMENT_3D ( 'NONE', #26370, #3298, #676 ) ;
#35324=ORIENTED_EDGE ( 'NONE', *, *, #17662, .F. ) ;
#35325=ORIENTED_EDGE ( 'NONE', *, *, #16130, .F. ) ;
#35327=ADVANCED_FACE ( 'NONE', ( #8598 ), #11962, .F. ) ;
#35328=CARTESIAN_POINT ( 'NONE',  ( -13.00000337463125710, -77.94228634059960825, 12.50000000000000000 ) ) ;
#35329=DIRECTION ( 'NONE',  ( 0.000000000000000000, 0.000000000000000000, 1.000000000000000000 ) ) ;
#35330=EDGE_CURVE ( 'NONE', #35136, #2553, #11565, .T. ) ;
#35331=CYLINDRICAL_SURFACE ( 'NONE', #7058, 2.000000000000000000 ) ;
#35332=ORIENTED_EDGE ( 'NONE', *, *, #32457, .F. ) ;
#35333=ORIENTED_EDGE ( 'NONE', *, *, #2470, .T. ) ;
#35335=ORIENTED_EDGE ( 'NONE', *, *, #10615, .F. ) ;
#35337=DIRECTION ( 'NONE',  ( 1.000000000000000000, 0.000000000000000000, 0.000000000000000000 ) ) ;
#35339=ORIENTED_EDGE ( 'NONE', *, *, #33702, .T. ) ;
#35341=EDGE_LOOP ( 'NONE', ( #20711, #35503 ) ) ;
#35342=EDGE_CURVE ( 'NONE', #34186, #35276, #15167, .T. ) ;
#35343=CIRCLE ( 'NONE', #23335, 2.000000000000001776 ) ;
#35344=DIRECTION ( 'NONE',  ( 0.000000000000000000, 0.000000000000000000, 1.000000000000000000 ) ) ;
#35345=EDGE_LOOP ( 'NONE', ( #27574, #1804 ) ) ;
#35346=ADVANCED_FACE ( 'NONE', ( #710 ), #12120, .F. ) ;
#35347=ORIENTED_EDGE ( 'NONE', *, *, #21976, .T. ) ;
#35348=( NAMED_UNIT ( * ) SI_UNIT ( $, .STERADIAN. ) SOLID_ANGLE_UNIT ( ) );
#35349=CARTESIAN_POINT ( 'NONE',  ( 0.000000000000000000, 0.000000000000000000, -5.000000000000000000 ) ) ;
#35350=DIRECTION ( 'NONE',  ( 1.000000000000000000, 0.000000000000000000, 0.000000000000000000 ) ) ;
#35351=ORIENTED_EDGE ( 'NONE', *, *, #16523, .T. ) ;
#35352=ORIENTED_EDGE ( 'NONE', *, *, #21621, .T. ) ;
#35353=DIRECTION ( 'NONE',  ( 1.000000000000000000, 0.000000000000000000, 0.000000000000000000 ) ) ;
#35356=EDGE_CURVE ( 'NONE', #25432, #26711, #36142, .T. ) ;
#35358=ADVANCED_FACE ( 'NONE', ( #9890 ), #21328, .T. ) ;
#35361=ORIENTED_EDGE ( 'NONE', *, *, #7290, .F. ) ;
#35362=DIRECTION ( 'NONE',  ( 0.000000000000000000, 0.000000000000000000, 1.000000000000000000 ) ) ;
#35363=CARTESIAN_POINT ( 'NONE',  ( -47.63139720814438505, -27.49999999999955591, -10.00000000000000178 ) ) ;
#35364=EDGE_CURVE ( 'NONE', #18749, #7366, #36726, .T. ) ;
#35365=ORIENTED_EDGE ( 'NONE', *, *, #22406, .F. ) ;
#35368=EDGE_CURVE ( 'NONE', #36249, #7111, #6786, .T. ) ;
#35369=CARTESIAN_POINT ( 'NONE',  ( 36.99999662536855283, -60.62177826491080168, -9.999999999999998224 ) ) ;
#35370=AXIS2_PLACEMENT_3D ( 'NONE', #3371, #359, #29238 ) ;
#35371=DIRECTION ( 'NONE',  ( 1.000000000000000000, 0.000000000000000000, 0.000000000000000000 ) ) ;
#35373=CYLINDRICAL_SURFACE ( 'NONE', #17914, 2.000000000000000000 ) ;
#35374=CIRCLE ( 'NONE', #19193, 2.000000000000001776 ) ;
#35376=EDGE_LOOP ( 'NONE', ( #35837, #10015 ) ) ;
#35377=DIRECTION ( 'NONE',  ( -0.000000000000000000, -0.000000000000000000, 1.000000000000000000 ) ) ;
#35378=AXIS2_PLACEMENT_3D ( 'NONE', #30299, #21858, #1813 ) ;
#35380=CARTESIAN_POINT ( 'NONE',  ( 54.99999662536844625, 60.62177826491077326, 12.50000000000000000 ) ) ;
#35381=ORIENTED_EDGE ( 'NONE', *, *, #22571, .T. ) ;
#35383=ORIENTED_EDGE ( 'NONE', *, *, #3231, .F. ) ;
#35384=DIRECTION ( 'NONE',  ( 0.000000000000000000, 0.000000000000000000, 1.000000000000000000 ) ) ;
#35385=DIRECTION ( 'NONE',  ( 0.000000000000000000, 0.000000000000000000, 1.000000000000000000 ) ) ;
#35386=AXIS2_PLACEMENT_3D ( 'NONE', #26666, #981, #17668 ) ;
#35388=DIRECTION ( 'NONE',  ( 1.000000000000000000, 0.000000000000000000, 0.000000000000000000 ) ) ;
#35389=DIRECTION ( 'NONE',  ( 1.000000000000000000, 0.000000000000000000, 0.000000000000000000 ) ) ;
#35392=CARTESIAN_POINT ( 'NONE',  ( 49.99999662536846756, 69.28203230275516944, 12.50000000000000000 ) ) ;
#35393=VERTEX_POINT ( 'NONE', #1271 ) ;
#35394=FACE_BOUND ( 'NONE', #10421, .T. ) ;
#35395=AXIS2_PLACEMENT_3D ( 'NONE', #15919, #21725, #7481 ) ;
#35396=FACE_OUTER_BOUND ( 'NONE', #2195, .T. ) ;
#35397=CARTESIAN_POINT ( 'NONE',  ( 52.99999662536846046, -43.30127018922200222, -9.999999999999998224 ) ) ;
#35398=CARTESIAN_POINT ( 'NONE',  ( 54.99999662536844625, -60.62177826491080168, 12.50000000000000000 ) ) ;
#35399=ORIENTED_EDGE ( 'NONE', *, *, #16332, .F. ) ;
#35400=DIRECTION ( 'NONE',  ( 0.000000000000000000, 0.000000000000000000, 1.000000000000000000 ) ) ;
#35401=CARTESIAN_POINT ( 'NONE',  ( -65.00000337463106348, -60.62177826491083010, 17.49999999999999645 ) ) ;
#35402=DIRECTION ( 'NONE',  ( 0.000000000000000000, -0.000000000000000000, -1.000000000000000000 ) ) ;
#35403=CARTESIAN_POINT ( 'NONE',  ( 49.99999662536846756, -69.28203230275519786, -5.000000000000000000 ) ) ;
#35404=EDGE_CURVE ( 'NONE', #28909, #19957, #22349, .T. ) ;
#35405=ORIENTED_EDGE ( 'NONE', *, *, #2676, .T. ) ;
#35407=DIRECTION ( 'NONE',  ( 0.000000000000000000, 0.000000000000000000, -1.000000000000000000 ) ) ;
#35408=LINE ( 'NONE', #29940, #30931 ) ;
#35410=ORIENTED_EDGE ( 'NONE', *, *, #8603, .T. ) ;
#35411=AXIS2_PLACEMENT_3D ( 'NONE', #36559, #22463, #16475 ) ;
#35412=VERTEX_POINT ( 'NONE', #4280 ) ;
#35413=DIRECTION ( 'NONE',  ( 1.000000000000000000, 0.000000000000000000, 0.000000000000000000 ) ) ;
#35414=CARTESIAN_POINT ( 'NONE',  ( 57.99999662536842493, 51.96152422706639129, 17.49999999999999645 ) ) ;
#35415=DIRECTION ( 'NONE',  ( 0.000000000000000000, 0.000000000000000000, 1.000000000000000000 ) ) ;
#35416=DIRECTION ( 'NONE',  ( 0.000000000000000000, 0.000000000000000000, -1.000000000000000000 ) ) ;
#35417=DIRECTION ( 'NONE',  ( 0.8660254037844344888, -0.5000000000000071054, 0.000000000000000000 ) ) ;
#35418=DIRECTION ( 'NONE',  ( 1.000000000000000000, 0.000000000000000000, 0.000000000000000000 ) ) ;
#35419=EDGE_CURVE ( 'NONE', #26119, #26245, #199, .T. ) ;
#35420=ORIENTED_EDGE ( 'NONE', *, *, #37020, .F. ) ;
#35421=EDGE_LOOP ( 'NONE', ( #19103, #21684, #7840, #28471 ) ) ;
#35422=CARTESIAN_POINT ( 'NONE',  ( 64.99999662536839651, 60.62177826491078747, 12.50000000000000000 ) ) ;
#35423=CARTESIAN_POINT ( 'NONE',  ( -2.000003374631303732, -86.60254037844400443, -9.999999999999998224 ) ) ;
#35424=EDGE_LOOP ( 'NONE', ( #21531, #28282 ) ) ;
#35425=CYLINDRICAL_SURFACE ( 'NONE', #37082, 2.000000000000001776 ) ;
#35426=EDGE_LOOP ( 'NONE', ( #7177, #34719, #740, #10983 ) ) ;
#35427=CARTESIAN_POINT ( 'NONE',  ( 56.99999662536846046, -43.30127018922200222, -9.999999999999998224 ) ) ;
#35428=ORIENTED_EDGE ( 'NONE', *, *, #10600, .F. ) ;
#35433=DIRECTION ( 'NONE',  ( 1.000000000000000000, 0.000000000000000000, 0.000000000000000000 ) ) ;
#35434=DIRECTION ( 'NONE',  ( 0.000000000000000000, 0.000000000000000000, 1.000000000000000000 ) ) ;
#35435=DIRECTION ( 'NONE',  ( -1.000000000000000000, 0.000000000000000000, 0.000000000000000000 ) ) ;
#35437=EDGE_LOOP ( 'NONE', ( #22976, #16433, #17782, #10749 ) ) ;
#35438=EDGE_LOOP ( 'NONE', ( #9642, #28411, #15732, #19730 ) ) ;
#35439=ORIENTED_EDGE ( 'NONE', *, *, #19763, .T. ) ;
#35441=VERTEX_POINT ( 'NONE', #24338 ) ;
#35442=VERTEX_POINT ( 'NONE', #35423 ) ;
#35443=CARTESIAN_POINT ( 'NONE',  ( 0.000000000000000000, 0.000000000000000000, -5.000000000000000000 ) ) ;
#35444=AXIS2_PLACEMENT_3D ( 'NONE', #31579, #3097, #19967 ) ;
#35445=CARTESIAN_POINT ( 'NONE',  ( 69.99999662536839651, -3.469446951953614189E-15, 12.50000000000000000 ) ) ;
#35446=ORIENTED_EDGE ( 'NONE', *, *, #33150, .T. ) ;
#35447=CIRCLE ( 'NONE', #28253, 2.000000000000001776 ) ;
#35448=LINE ( 'NONE', #3919, #4715 ) ;
#35449=CARTESIAN_POINT ( 'NONE',  ( 64.99999662536839651, -43.30127018922199511, 12.50000000000000000 ) ) ;
#35450=DIRECTION ( 'NONE',  ( 0.000000000000000000, 0.000000000000000000, 1.000000000000000000 ) ) ;
#35451=VERTEX_POINT ( 'NONE', #12690 ) ;
#35452=DIRECTION ( 'NONE',  ( 0.000000000000000000, 0.000000000000000000, 1.000000000000000000 ) ) ;
#35454=EDGE_CURVE ( 'NONE', #16972, #11035, #35561, .T. ) ;
#35455=DIRECTION ( 'NONE',  ( 0.000000000000000000, 0.000000000000000000, 1.000000000000000000 ) ) ;
#35457=DIRECTION ( 'NONE',  ( 0.000000000000000000, 0.000000000000000000, 1.000000000000000000 ) ) ;
#35459=EDGE_CURVE ( 'NONE', #4910, #10671, #31900, .T. ) ;
#35460=ORIENTED_EDGE ( 'NONE', *, *, #25866, .F. ) ;
#35461=EDGE_LOOP ( 'NONE', ( #31639, #2622, #16102, #35049 ) ) ;
#35462=DIRECTION ( 'NONE',  ( 1.000000000000000000, 0.000000000000000000, 0.000000000000000000 ) ) ;
#35463=DIRECTION ( 'NONE',  ( 0.000000000000000000, 0.000000000000000000, -1.000000000000000000 ) ) ;
#35465=EDGE_CURVE ( 'NONE', #18462, #8511, #4397, .T. ) ;
#35466=ORIENTED_EDGE ( 'NONE', *, *, #18603, .F. ) ;
#35467=CARTESIAN_POINT ( 'NONE',  ( 43.19957991610432657, 47.04203867989531318, 12.49999999999999822 ) ) ;
#35468=CARTESIAN_POINT ( 'NONE',  ( -75.00000337463097821, -8.660254037844422825, -9.999999999999998224 ) ) ;
#35469=EDGE_CURVE ( 'NONE', #1395, #12727, #34451, .T. ) ;
#35471=AXIS2_PLACEMENT_3D ( 'NONE', #26852, #12588, #17654 ) ;
#35472=PLANE ( 'NONE',  #14191 ) ;
#35473=ORIENTED_EDGE ( 'NONE', *, *, #10536, .F. ) ;
#35474=CARTESIAN_POINT ( 'NONE',  ( 27.78182860042856461, 56.67878100130339902, 12.49999999999999822 ) ) ;
#35475=CARTESIAN_POINT ( 'NONE',  ( 4.279621169095998212, -62.97617850287780072, -4.999999999999997335 ) ) ;
#35476=LINE ( 'NONE', #15594, #34662 ) ;
#35477=ORIENTED_EDGE ( 'NONE', *, *, #21533, .T. ) ;
#35478=VERTEX_POINT ( 'NONE', #32396 ) ;
#35479=EDGE_CURVE ( 'NONE', #28847, #31817, #15277, .T. ) ;
#35480=CIRCLE ( 'NONE', #18716, 2.000000000000001776 ) ;
#35481=VERTEX_POINT ( 'NONE', #15531 ) ;
#35482=DIRECTION ( 'NONE',  ( 0.000000000000000000, 0.000000000000000000, -1.000000000000000000 ) ) ;
#35483=DIRECTION ( 'NONE',  ( 0.000000000000000000, 0.000000000000000000, 1.000000000000000000 ) ) ;
#35484=DIRECTION ( 'NONE',  ( 1.000000000000000000, 0.000000000000000000, 0.000000000000000000 ) ) ;
#35485=CARTESIAN_POINT ( 'NONE',  ( 9.999996625368655856, -69.28203230275519786, -5.000000000000000000 ) ) ;
#35486=CARTESIAN_POINT ( 'NONE',  ( -50.00000337463109190, 51.96152422706637708, -9.999999999999998224 ) ) ;
#35487=ORIENTED_EDGE ( 'NONE', *, *, #7349, .F. ) ;
#35488=CARTESIAN_POINT ( 'NONE',  ( -37.00000337463117717, -77.94228634059963667, -9.999999999999998224 ) ) ;
#35489=EDGE_CURVE ( 'NONE', #9206, #12265, #27849, .T. ) ;
#35490=DIRECTION ( 'NONE',  ( -0.000000000000000000, -0.000000000000000000, -1.000000000000000000 ) ) ;
#35491=CIRCLE ( 'NONE', #25313, 2.000000000000001776 ) ;
#35493=DIRECTION ( 'NONE',  ( 1.000000000000000000, 0.000000000000000000, 0.000000000000000000 ) ) ;
#35494=ORIENTED_EDGE ( 'NONE', *, *, #8729, .T. ) ;
#35496=DIRECTION ( 'NONE',  ( 1.000000000000000000, 0.000000000000000000, 0.000000000000000000 ) ) ;
#35497=CYLINDRICAL_SURFACE ( 'NONE', #35386, 2.000000000000001776 ) ;
#35498=EDGE_LOOP ( 'NONE', ( #12646, #10942, #34316, #23145 ) ) ;
#35499=ORIENTED_EDGE ( 'NONE', *, *, #10042, .F. ) ;
#35500=DIRECTION ( 'NONE',  ( -1.000000000000000000, 0.000000000000000000, 0.000000000000000000 ) ) ;
#35501=CYLINDRICAL_SURFACE ( 'NONE', #14573, 2.000000000000001776 ) ;
#35503=ORIENTED_EDGE ( 'NONE', *, *, #11592, .F. ) ;
#35504=ORIENTED_EDGE ( 'NONE', *, *, #24056, .F. ) ;
#35505=VERTEX_POINT ( 'NONE', #1447 ) ;
#35506=CARTESIAN_POINT ( 'NONE',  ( 74.99999662536835388, -25.98076211353319565, 12.50000000000000000 ) ) ;
#35507=EDGE_CURVE ( 'NONE', #33684, #8634, #5700, .T. ) ;
#35508=ORIENTED_EDGE ( 'NONE', *, *, #14570, .T. ) ;
#35509=ORIENTED_EDGE ( 'NONE', *, *, #3107, .T. ) ;
#35510=CARTESIAN_POINT ( 'NONE',  ( -70.00000337463099243, 51.96152422706637708, -5.000000000000000000 ) ) ;
#35513=CIRCLE ( 'NONE', #13948, 2.000000000000000000 ) ;
#35515=ORIENTED_EDGE ( 'NONE', *, *, #9869, .F. ) ;
#35517=ORIENTED_EDGE ( 'NONE', *, *, #18943, .T. ) ;
#35520=CARTESIAN_POINT ( 'NONE',  ( 34.99999662536855283, 60.62177826491078747, -9.999999999999998224 ) ) ;
#35521=DIRECTION ( 'NONE',  ( 0.000000000000000000, 0.000000000000000000, 1.000000000000000000 ) ) ;
#35523=VERTEX_POINT ( 'NONE', #2200 ) ;
#35524=LINE ( 'NONE', #15459, #14731 ) ;
#35526=EDGE_CURVE ( 'NONE', #11341, #23693, #33335, .T. ) ;
#35529=DIRECTION ( 'NONE',  ( 1.000000000000000000, 0.000000000000000000, 0.000000000000000000 ) ) ;
#35530=DIRECTION ( 'NONE',  ( 1.000000000000000000, 0.000000000000000000, 0.000000000000000000 ) ) ;
#35531=EDGE_CURVE ( 'NONE', #20921, #5470, #18270, .T. ) ;
#35532=AXIS2_PLACEMENT_3D ( 'NONE', #23272, #12361, #3586 ) ;
#35533=DIRECTION ( 'NONE',  ( 0.4999999999999922839, -0.8660254037844431485, 0.000000000000000000 ) ) ;
#35534=ADVANCED_FACE ( 'NONE', ( #13825 ), #36877, .F. ) ;
#35537=CARTESIAN_POINT ( 'NONE',  ( 42.99999662536848888, -77.94228634059960825, 17.49999999999999645 ) ) ;
#35538=ADVANCED_FACE ( 'NONE', ( #19271 ), #11186, .T. ) ;
#35539=DIRECTION ( 'NONE',  ( 0.000000000000000000, 0.000000000000000000, 1.000000000000000000 ) ) ;
#35540=CARTESIAN_POINT ( 'NONE',  ( 4.279621169095998212, -62.97617850287780072, -4.999999999999997335 ) ) ;
#35541=ADVANCED_FACE ( 'NONE', ( #22089 ), #25269, .F. ) ;
#35542=ORIENTED_EDGE ( 'NONE', *, *, #33989, .T. ) ;
#35543=ORIENTED_EDGE ( 'NONE', *, *, #16860, .T. ) ;
#35544=EDGE_LOOP ( 'NONE', ( #35876, #30848, #11183, #7648 ) ) ;
#35547=CARTESIAN_POINT ( 'NONE',  ( 86.99999662536832545, 25.98076211353319565, -9.999999999999998224 ) ) ;
#35548=FACE_OUTER_BOUND ( 'NONE', #25022, .T. ) ;
#35550=EDGE_CURVE ( 'NONE', #7036, #29469, #25479, .T. ) ;
#35551=EDGE_CURVE ( 'NONE', #24428, #18343, #29041, .T. ) ;
#35553=DIRECTION ( 'NONE',  ( 0.000000000000000000, 0.000000000000000000, 1.000000000000000000 ) ) ;
#35554=EDGE_CURVE ( 'NONE', #14334, #21168, #1510, .T. ) ;
#35555=CARTESIAN_POINT ( 'NONE',  ( 36.99999662536855283, 60.62177826491078747, -5.000000000000000000 ) ) ;
#35556=ORIENTED_EDGE ( 'NONE', *, *, #16243, .F. ) ;
#35558=ORIENTED_EDGE ( 'NONE', *, *, #27046, .F. ) ;
#35559=DIRECTION ( 'NONE',  ( 1.000000000000000000, 0.000000000000000000, 0.000000000000000000 ) ) ;
#35560=AXIS2_PLACEMENT_3D ( 'NONE', #19538, #36230, #10535 ) ;
#35561=CIRCLE ( 'NONE', #6171, 3.000000000000007105 ) ;
#35562=DIRECTION ( 'NONE',  ( 0.000000000000000000, 0.000000000000000000, 1.000000000000000000 ) ) ;
#35563=DIRECTION ( 'NONE',  ( -1.000000000000000000, 0.000000000000000000, 0.000000000000000000 ) ) ;
#35565=ORIENTED_EDGE ( 'NONE', *, *, #25146, .T. ) ;
#35566=FACE_OUTER_BOUND ( 'NONE', #20432, .T. ) ;
#35568=CARTESIAN_POINT ( 'NONE',  ( 84.99999662536831124, -25.98076211353319565, 12.50000000000000000 ) ) ;
#35569=ADVANCED_FACE ( 'NONE', ( #7842 ), #10993, .F. ) ;
#35570=CIRCLE ( 'NONE', #28954, 2.000000000000001776 ) ;
#35571=CARTESIAN_POINT ( 'NONE',  ( 77.99999662536833966, -3.224517592124143893E-15, -9.999999999999998224 ) ) ;
#35572=DIRECTION ( 'NONE',  ( 0.000000000000000000, 0.000000000000000000, 1.000000000000000000 ) ) ;
#35573=ORIENTED_EDGE ( 'NONE', *, *, #26626, .T. ) ;
#35576=DIRECTION ( 'NONE',  ( 0.000000000000000000, 0.000000000000000000, 1.000000000000000000 ) ) ;
#35578=AXIS2_PLACEMENT_3D ( 'NONE', #12073, #12645, #27082 ) ;
#35580=ORIENTED_EDGE ( 'NONE', *, *, #1412, .T. ) ;
#35581=ORIENTED_EDGE ( 'NONE', *, *, #24114, .F. ) ;
#35583=PLANE ( 'NONE',  #14179 ) ;
#35584=CARTESIAN_POINT ( 'NONE',  ( 69.99999662536839651, 34.64101615137758472, -9.999999999999998224 ) ) ;
#35585=AXIS2_PLACEMENT_3D ( 'NONE', #10083, #32762, #27122 ) ;
#35587=ORIENTED_EDGE ( 'NONE', *, *, #29987, .T. ) ;
#35588=DIRECTION ( 'NONE',  ( -1.000000000000000000, 0.000000000000000000, -0.000000000000000000 ) ) ;
#35589=DIRECTION ( 'NONE',  ( 0.000000000000000000, 0.000000000000000000, 1.000000000000000000 ) ) ;
#35590=DIRECTION ( 'NONE',  ( 0.000000000000000000, 0.000000000000000000, 1.000000000000000000 ) ) ;
#35591=EDGE_CURVE ( 'NONE', #2878, #26137, #12278, .T. ) ;
#35592=ORIENTED_EDGE ( 'NONE', *, *, #5786, .T. ) ;
#35595=VERTEX_POINT ( 'NONE', #31070 ) ;
#35596=CARTESIAN_POINT ( 'NONE',  ( 17.99999662536861678, -86.60254037844400443, -9.999999999999998224 ) ) ;
#35597=EDGE_CURVE ( 'NONE', #1926, #9828, #23682, .T. ) ;
#35598=DIRECTION ( 'NONE',  ( 1.000000000000000000, 0.000000000000000000, 0.000000000000000000 ) ) ;
#35599=ORIENTED_EDGE ( 'NONE', *, *, #32567, .T. ) ;
#35600=ADVANCED_FACE ( 'NONE', ( #1836 ), #10445, .F. ) ;
#35602=ORIENTED_EDGE ( 'NONE', *, *, #2482, .T. ) ;
#35604=CARTESIAN_POINT ( 'NONE',  ( 41.99999662536853151, -69.28203230275519786, -9.999999999999998224 ) ) ;
#35605=ORIENTED_EDGE ( 'NONE', *, *, #7581, .T. ) ;
#35606=ORIENTED_EDGE ( 'NONE', *, *, #25001, .F. ) ;
#35607=CARTESIAN_POINT ( 'NONE',  ( 0.000000000000000000, 0.000000000000000000, -5.000000000000000000 ) ) ;
#35610=DIRECTION ( 'NONE',  ( -1.047444401652940007E-14, -1.000000000000000000, 0.000000000000000000 ) ) ;
#35611=DIRECTION ( 'NONE',  ( -1.000000000000000000, 0.000000000000000000, 0.000000000000000000 ) ) ;
#35612=ORIENTED_EDGE ( 'NONE', *, *, #14403, .T. ) ;
#35613=ORIENTED_EDGE ( 'NONE', *, *, #32388, .F. ) ;
#35614=EDGE_CURVE ( 'NONE', #5261, #27815, #8691, .T. ) ;
#35615=CIRCLE ( 'NONE', #11049, 2.000000000000001776 ) ;
#35616=AXIS2_PLACEMENT_3D ( 'NONE', #24347, #32405, #35794 ) ;
#35620=CARTESIAN_POINT ( 'NONE',  ( -70.00000337463102085, -51.96152422706641971, -9.999999999999998224 ) ) ;
#35621=ORIENTED_EDGE ( 'NONE', *, *, #25645, .F. ) ;
#35622=CARTESIAN_POINT ( 'NONE',  ( -50.00000337463109190, 51.96152422706637708, -9.999999999999998224 ) ) ;
#35623=CARTESIAN_POINT ( 'NONE',  ( 3.499999999999987566, 55.00000000000000000, -10.00000000000000178 ) ) ;
#35624=ORIENTED_EDGE ( 'NONE', *, *, #15843, .T. ) ;
#35625=CARTESIAN_POINT ( 'NONE',  ( -85.00000337463092137, -25.98076211353322051, -9.999999999999998224 ) ) ;
#35626=DIRECTION ( 'NONE',  ( 0.000000000000000000, 0.000000000000000000, 1.000000000000000000 ) ) ;
#35627=VECTOR ( 'NONE', #6506, 1000.000000000000000 ) ;
#35629=DIRECTION ( 'NONE',  ( 0.000000000000000000, 0.000000000000000000, 1.000000000000000000 ) ) ;
#35630=DIRECTION ( 'NONE',  ( 0.000000000000000000, 0.000000000000000000, 1.000000000000000000 ) ) ;
#35633=CARTESIAN_POINT ( 'NONE',  ( -55.00000337463110611, -43.30127018922202353, 12.50000000000000000 ) ) ;
#35634=CARTESIAN_POINT ( 'NONE',  ( -30.00000337463119848, -69.28203230275522628, -5.000000000000000000 ) ) ;
#35635=EDGE_CURVE ( 'NONE', #5095, #33663, #29632, .T. ) ;
#35636=CARTESIAN_POINT ( 'NONE',  ( -80.69570745083950669, 15.44540918807064500, -5.000000000000000000 ) ) ;
#35637=DIRECTION ( 'NONE',  ( 0.5000000000000039968, 0.8660254037844363761, 0.000000000000000000 ) ) ;
#35639=AXIS2_PLACEMENT_3D ( 'NONE', #2411, #11007, #22447 ) ;
#35640=CARTESIAN_POINT ( 'NONE',  ( 57.99999662536844625, 34.64101615137759893, -9.999999999999998224 ) ) ;
#35641=CIRCLE ( 'NONE', #29021, 33.00000000000001421 ) ;
#35643=VERTEX_POINT ( 'NONE', #31952 ) ;
#35644=CARTESIAN_POINT ( 'NONE',  ( -87.83969979969870678, -14.80603122773086966, -49.86561046011506448 ) ) ;
#35645=ORIENTED_EDGE ( 'NONE', *, *, #15370, .T. ) ;
#35647=LINE ( 'NONE', #35847, #1443 ) ;
#35648=AXIS2_PLACEMENT_3D ( 'NONE', #1421, #10244, #29929 ) ;
#35650=ORIENTED_EDGE ( 'NONE', *, *, #9239, .T. ) ;
#35651=VERTEX_POINT ( 'NONE', #28619 ) ;
#35652=ADVANCED_FACE ( 'NONE', ( #2951 ), #31785, .F. ) ;
#35653=VECTOR ( 'NONE', #34437, 1000.000000000000000 ) ;
#35654=EDGE_LOOP ( 'NONE', ( #4638, #349 ) ) ;
#35655=CYLINDRICAL_SURFACE ( 'NONE', #23172, 2.000000000000000000 ) ;
#35656=DIRECTION ( 'NONE',  ( -0.000000000000000000, -0.000000000000000000, 1.000000000000000000 ) ) ;
#35657=EDGE_CURVE ( 'NONE', #28819, #24755, #22474, .T. ) ;
#35658=DIRECTION ( 'NONE',  ( 1.000000000000000000, 0.000000000000000000, 0.000000000000000000 ) ) ;
#35660=AXIS2_PLACEMENT_3D ( 'NONE', #3842, #15285, #26723 ) ;
#35661=CARTESIAN_POINT ( 'NONE',  ( -59.29837256189559724, -31.02796211690927919, -49.86561046011506448 ) ) ;
#35662=EDGE_LOOP ( 'NONE', ( #35690, #3273 ) ) ;
#35663=DIRECTION ( 'NONE',  ( 1.000000000000000000, 0.000000000000000000, 0.000000000000000000 ) ) ;
#35664=VECTOR ( 'NONE', #33672, 1000.000000000000000 ) ;
#35665=AXIS2_PLACEMENT_3D ( 'NONE', #386, #11820, #583 ) ;
#35666=CARTESIAN_POINT ( 'NONE',  ( -73.00000337463097821, 8.660254037844374864, 12.50000000000000000 ) ) ;
#35667=ADVANCED_FACE ( 'NONE', ( #28967 ), #6292, .F. ) ;
#35668=DIRECTION ( 'NONE',  ( 0.000000000000000000, 0.000000000000000000, 1.000000000000000000 ) ) ;
#35669=ORIENTED_EDGE ( 'NONE', *, *, #337, .T. ) ;
#35670=CARTESIAN_POINT ( 'NONE',  ( 70.47608876694671665, 59.13646009116074964, -4.999999999999997335 ) ) ;
#35671=DIRECTION ( 'NONE',  ( 0.000000000000000000, 0.000000000000000000, 1.000000000000000000 ) ) ;
#35672=ORIENTED_EDGE ( 'NONE', *, *, #9971, .T. ) ;
#35673=ORIENTED_EDGE ( 'NONE', *, *, #6677, .F. ) ;
#35674=CIRCLE ( 'NONE', #6947, 27.00000000000001776 ) ;
#35676=EDGE_CURVE ( 'NONE', #33091, #15386, #14733, .T. ) ;
#35677=CARTESIAN_POINT ( 'NONE',  ( 9.999996625368655856, -69.28203230275519786, -9.999999999999998224 ) ) ;
#35678=AXIS2_PLACEMENT_3D ( 'NONE', #11652, #26657, #23483 ) ;
#35679=CARTESIAN_POINT ( 'NONE',  ( -17.14523346298279449, 93.36492675454785228, 12.49999999999999822 ) ) ;
#35681=ORIENTED_EDGE ( 'NONE', *, *, #7833, .T. ) ;
#35682=CIRCLE ( 'NONE', #26086, 2.000000000000001776 ) ;
#35683=ORIENTED_EDGE ( 'NONE', *, *, #23866, .F. ) ;
#35685=CIRCLE ( 'NONE', #16515, 2.000000000000001776 ) ;
#35689=DIRECTION ( 'NONE',  ( -1.000000000000000000, 0.000000000000000000, 0.000000000000000000 ) ) ;
#35690=ORIENTED_EDGE ( 'NONE', *, *, #15087, .T. ) ;
#35691=ORIENTED_EDGE ( 'NONE', *, *, #22906, .T. ) ;
#35692=EDGE_CURVE ( 'NONE', #21307, #27070, #32635, .T. ) ;
#35693=VECTOR ( 'NONE', #4850, 1000.000000000000000 ) ;
#35694=CYLINDRICAL_SURFACE ( 'NONE', #446, 2.000000000000001776 ) ;
#35695=EDGE_CURVE ( 'NONE', #35086, #11321, #27263, .T. ) ;
#35696=CYLINDRICAL_SURFACE ( 'NONE', #34434, 2.000000000000001776 ) ;
#35697=ORIENTED_EDGE ( 'NONE', *, *, #27011, .T. ) ;
#35698=VERTEX_POINT ( 'NONE', #11377 ) ;
#35699=DIRECTION ( 'NONE',  ( 1.000000000000000000, 0.000000000000000000, 0.000000000000000000 ) ) ;
#35700=DIRECTION ( 'NONE',  ( -1.000000000000000000, 0.000000000000000000, 0.000000000000000000 ) ) ;
#35702=DIRECTION ( 'NONE',  ( 0.000000000000000000, 0.000000000000000000, 1.000000000000000000 ) ) ;
#35703=DIRECTION ( 'NONE',  ( 1.000000000000000000, 0.000000000000000000, 0.000000000000000000 ) ) ;
#35704=ORIENTED_EDGE ( 'NONE', *, *, #22776, .T. ) ;
#35705=DIRECTION ( 'NONE',  ( 1.000000000000000000, 0.000000000000000000, 0.000000000000000000 ) ) ;
#35706=VERTEX_POINT ( 'NONE', #11540 ) ;
#35707=DIRECTION ( 'NONE',  ( 1.000000000000000000, 0.000000000000000000, 0.000000000000000000 ) ) ;
#35708=ADVANCED_FACE ( 'NONE', ( #29169 ), #5563, .F. ) ;
#35713=CYLINDRICAL_SURFACE ( 'NONE', #3946, 2.000000000000001776 ) ;
#35714=CIRCLE ( 'NONE', #1574, 2.000000000000001776 ) ;
#35717=DIRECTION ( 'NONE',  ( 1.000000000000000000, 0.000000000000000000, 0.000000000000000000 ) ) ;
#35718=EDGE_CURVE ( 'NONE', #9542, #10851, #14934, .T. ) ;
#35719=DIRECTION ( 'NONE',  ( 0.000000000000000000, 0.000000000000000000, 1.000000000000000000 ) ) ;
#35720=ORIENTED_EDGE ( 'NONE', *, *, #5057, .F. ) ;
#35721=DIRECTION ( 'NONE',  ( -1.000000000000000000, 0.000000000000000000, 0.000000000000000000 ) ) ;
#35722=DIRECTION ( 'NONE',  ( 0.000000000000000000, -0.000000000000000000, -1.000000000000000000 ) ) ;
#35723=FACE_OUTER_BOUND ( 'NONE', #6137, .T. ) ;
#35725=CIRCLE ( 'NONE', #6370, 2.000000000000001776 ) ;
#35727=ORIENTED_EDGE ( 'NONE', *, *, #13095, .T. ) ;
#35728=CARTESIAN_POINT ( 'NONE',  ( 57.99999662536842493, -51.96152422706639840, -9.999999999999998224 ) ) ;
#35729=CARTESIAN_POINT ( 'NONE',  ( -22.00000337463124112, -69.28203230275522628, 17.49999999999999645 ) ) ;
#35730=DIRECTION ( 'NONE',  ( 1.000000000000000000, 0.000000000000000000, 0.000000000000000000 ) ) ;
#35731=ORIENTED_EDGE ( 'NONE', *, *, #14853, .F. ) ;
#35733=CARTESIAN_POINT ( 'NONE',  ( -15.00000337463126066, 77.94228634059957983, -9.999999999999998224 ) ) ;
#35734=ADVANCED_FACE ( 'NONE', ( #8392 ), #23187, .F. ) ;
#35735=CIRCLE ( 'NONE', #15977, 2.000000000000001776 ) ;
#35737=ORIENTED_EDGE ( 'NONE', *, *, #17143, .F. ) ;
#35740=CARTESIAN_POINT ( 'NONE',  ( 44.99999662536851019, 77.94228634059959404, 12.50000000000000000 ) ) ;
#35741=VECTOR ( 'NONE', #21067, 1000.000000000000000 ) ;
#35742=CIRCLE ( 'NONE', #2815, 2.000000000000001776 ) ;
#35743=ADVANCED_FACE ( 'NONE', ( #16999 ), #34633, .F. ) ;
#35744=CIRCLE ( 'NONE', #3401, 2.000000000000000000 ) ;
#35745=AXIS2_PLACEMENT_3D ( 'NONE', #27300, #9868, #20744 ) ;
#35747=DIRECTION ( 'NONE',  ( 0.000000000000000000, 0.000000000000000000, 1.000000000000000000 ) ) ;
#35748=EDGE_CURVE ( 'NONE', #2363, #10643, #20530, .T. ) ;
#35750=ORIENTED_EDGE ( 'NONE', *, *, #31522, .T. ) ;
#35751=DIRECTION ( 'NONE',  ( 0.000000000000000000, 0.000000000000000000, 1.000000000000000000 ) ) ;
#35752=CIRCLE ( 'NONE', #17198, 33.00000000000001421 ) ;
#35753=CARTESIAN_POINT ( 'NONE',  ( -68.17080498304596858, 51.15280100851584422, 12.50000000000000000 ) ) ;
#35754=CARTESIAN_POINT ( 'NONE',  ( 10.21421739743242618, 84.61404610869705323, -5.000000000000000000 ) ) ;
#35755=CARTESIAN_POINT ( 'NONE',  ( 64.99999662536839651, -60.62177826491080168, 17.49999999999999645 ) ) ;
#35757=DIRECTION ( 'NONE',  ( -1.000000000000000000, 0.000000000000000000, 0.000000000000000000 ) ) ;
#35759=DIRECTION ( 'NONE',  ( 0.000000000000000000, 0.000000000000000000, 1.000000000000000000 ) ) ;
#35760=CIRCLE ( 'NONE', #20196, 27.00000000000001776 ) ;
#35761=ORIENTED_EDGE ( 'NONE', *, *, #14432, .F. ) ;
#35762=EDGE_CURVE ( 'NONE', #3917, #13513, #36856, .T. ) ;
#35763=AXIS2_PLACEMENT_3D ( 'NONE', #23925, #17917, #26354 ) ;
#35764=VERTEX_POINT ( 'NONE', #17729 ) ;
#35765=DIRECTION ( 'NONE',  ( 0.000000000000000000, 0.000000000000000000, -1.000000000000000000 ) ) ;
#35766=CARTESIAN_POINT ( 'NONE',  ( -80.00000337463094979, -17.32050807568882078, -9.999999999999998224 ) ) ;
#35767=AXIS2_PLACEMENT_3D ( 'NONE', #17815, #3581, #26439 ) ;
#35768=CARTESIAN_POINT ( 'NONE',  ( -33.00000337463116296, 60.62177826491077326, -5.000000000000000000 ) ) ;
#35769=AXIS2_PLACEMENT_3D ( 'NONE', #11356, #14362, #17523 ) ;
#35770=ORIENTED_EDGE ( 'NONE', *, *, #35022, .T. ) ;
#35771=CYLINDRICAL_SURFACE ( 'NONE', #9195, 3.499999999999991562 ) ;
#35772=DIRECTION ( 'NONE',  ( 0.000000000000000000, 0.000000000000000000, 1.000000000000000000 ) ) ;
#35774=AXIS2_PLACEMENT_3D ( 'NONE', #21120, #13057, #35757 ) ;
#35775=CYLINDRICAL_SURFACE ( 'NONE', #26801, 2.000000000000001776 ) ;
#35776=VERTEX_POINT ( 'NONE', #3123 ) ;
#35777=AXIS2_PLACEMENT_3D ( 'NONE', #24196, #27012, #15399 ) ;
#35779=DIRECTION ( 'NONE',  ( 0.000000000000000000, 0.000000000000000000, 1.000000000000000000 ) ) ;
#35781=DIRECTION ( 'NONE',  ( 0.000000000000000000, 0.000000000000000000, -1.000000000000000000 ) ) ;
#35782=ORIENTED_EDGE ( 'NONE', *, *, #23944, .F. ) ;
#35784=CARTESIAN_POINT ( 'NONE',  ( -72.00000337463100664, 17.32050807568877460, -5.000000000000000000 ) ) ;
#35785=ORIENTED_EDGE ( 'NONE', *, *, #15939, .T. ) ;
#35787=VECTOR ( 'NONE', #36163, 1000.000000000000000 ) ;
#35788=EDGE_CURVE ( 'NONE', #35651, #29261, #12915, .T. ) ;
#35789=AXIS2_PLACEMENT_3D ( 'NONE', #16349, #7178, #18618 ) ;
#35790=DIRECTION ( 'NONE',  ( 1.000000000000000000, 0.000000000000000000, 0.000000000000000000 ) ) ;
#35792=ORIENTED_EDGE ( 'NONE', *, *, #11367, .F. ) ;
#35793=EDGE_CURVE ( 'NONE', #21238, #13993, #30875, .T. ) ;
#35794=DIRECTION ( 'NONE',  ( -1.000000000000000000, 0.000000000000000000, -0.000000000000000000 ) ) ;
#35796=EDGE_CURVE ( 'NONE', #6603, #182, #1543, .T. ) ;
#35799=AXIS2_PLACEMENT_3D ( 'NONE', #36097, #1956, #7231 ) ;
#35800=CARTESIAN_POINT ( 'NONE',  ( 62.99999662536839651, -43.30127018922199511, 12.50000000000000000 ) ) ;
#35801=CIRCLE ( 'NONE', #33386, 2.000000000000001776 ) ;
#35803=DIRECTION ( 'NONE',  ( 0.000000000000000000, 0.000000000000000000, 1.000000000000000000 ) ) ;
#35804=EDGE_LOOP ( 'NONE', ( #28518, #32487 ) ) ;
#35805=DIRECTION ( 'NONE',  ( 0.000000000000000000, 0.000000000000000000, -1.000000000000000000 ) ) ;
#35806=DIRECTION ( 'NONE',  ( 0.000000000000000000, 0.000000000000000000, -1.000000000000000000 ) ) ;
#35807=CIRCLE ( 'NONE', #4080, 3.000000000000006661 ) ;
#35809=VERTEX_POINT ( 'NONE', #27275 ) ;
#35810=EDGE_CURVE ( 'NONE', #10952, #16326, #2757, .T. ) ;
#35811=VERTEX_POINT ( 'NONE', #15288 ) ;
#35812=VERTEX_POINT ( 'NONE', #26921 ) ;
#35813=EDGE_CURVE ( 'NONE', #7555, #9227, #6330, .T. ) ;
#35814=CARTESIAN_POINT ( 'NONE',  ( -70.00000337463099243, 17.32050807568877460, -5.000000000000000000 ) ) ;
#35815=AXIS2_PLACEMENT_3D ( 'NONE', #2902, #629, #37028 ) ;
#35816=EDGE_CURVE ( 'NONE', #27142, #7889, #956, .T. ) ;
#35817=CARTESIAN_POINT ( 'NONE',  ( -63.00000337463104927, -43.30127018922202353, 17.49999999999999645 ) ) ;
#35818=ORIENTED_EDGE ( 'NONE', *, *, #36270, .F. ) ;
#35819=AXIS2_PLACEMENT_3D ( 'NONE', #7085, #35228, #32391 ) ;
#35820=AXIS2_PLACEMENT_3D ( 'NONE', #6772, #12954, #23859 ) ;
#35822=DIRECTION ( 'NONE',  ( 1.000000000000000000, 0.000000000000000000, 0.000000000000000000 ) ) ;
#35823=VERTEX_POINT ( 'NONE', #18100 ) ;
#35825=CARTESIAN_POINT ( 'NONE',  ( -53.00000337463106348, 43.30127018922197379, -9.999999999999998224 ) ) ;
#35826=CARTESIAN_POINT ( 'NONE',  ( -50.00000337463109190, 69.28203230275518365, 17.49999999999999645 ) ) ;
#35828=CARTESIAN_POINT ( 'NONE',  ( -48.00000337463112032, -51.96152422706641971, 12.50000000000000000 ) ) ;
#35829=DIRECTION ( 'NONE',  ( 0.000000000000000000, 0.000000000000000000, -1.000000000000000000 ) ) ;
#35831=VERTEX_POINT ( 'NONE', #12654 ) ;
#35832=VECTOR ( 'NONE', #2434, 1000.000000000000000 ) ;
#35833=CARTESIAN_POINT ( 'NONE',  ( -67.00000337463104927, -43.30127018922202353, 12.50000000000000000 ) ) ;
#35834=CARTESIAN_POINT ( 'NONE',  ( 59.99999662536842493, 51.96152422706639129, 12.50000000000000000 ) ) ;
#35835=CARTESIAN_POINT ( 'NONE',  ( 0.000000000000000000, 0.000000000000000000, 12.49999999999999822 ) ) ;
#35836=DIRECTION ( 'NONE',  ( 0.000000000000000000, 0.000000000000000000, 1.000000000000000000 ) ) ;
#35837=ORIENTED_EDGE ( 'NONE', *, *, #2829, .T. ) ;
#35838=VECTOR ( 'NONE', #32795, 1000.000000000000000 ) ;
#35839=CARTESIAN_POINT ( 'NONE',  ( 1.999996625368710257, -69.28203230275519786, -5.000000000000000000 ) ) ;
#35840=CARTESIAN_POINT ( 'NONE',  ( 27.99999662536857414, -69.28203230275519786, 12.50000000000000000 ) ) ;
#35842=CIRCLE ( 'NONE', #10085, 2.000000000000001776 ) ;
#35844=ORIENTED_EDGE ( 'NONE', *, *, #9131, .T. ) ;
#35845=AXIS2_PLACEMENT_3D ( 'NONE', #17705, #26156, #20908 ) ;
#35846=DIRECTION ( 'NONE',  ( -0.4999999999999980016, 0.8660254037844398178, 0.000000000000000000 ) ) ;
#35847=CARTESIAN_POINT ( 'NONE',  ( 46.99999662536849598, -77.94228634059960825, -9.999999999999998224 ) ) ;
#35852=VECTOR ( 'NONE', #8492, 1000.000000000000000 ) ;
#35853=ORIENTED_EDGE ( 'NONE', *, *, #673, .T. ) ;
#35855=ADVANCED_FACE ( 'NONE', ( #18284 ), #27093, .F. ) ;
#35856=FACE_BOUND ( 'NONE', #30924, .T. ) ;
#35857=DIRECTION ( 'NONE',  ( 0.000000000000000000, 0.000000000000000000, 1.000000000000000000 ) ) ;
#35858=DIRECTION ( 'NONE',  ( 0.000000000000000000, 0.000000000000000000, 1.000000000000000000 ) ) ;
#35859=CARTESIAN_POINT ( 'NONE',  ( 52.99999662536844625, 60.62177826491077326, -9.999999999999998224 ) ) ;
#35860=EDGE_LOOP ( 'NONE', ( #14337, #24435, #34, #34707 ) ) ;
#35862=DIRECTION ( 'NONE',  ( 0.000000000000000000, -0.000000000000000000, -1.000000000000000000 ) ) ;
#35864=DIRECTION ( 'NONE',  ( 0.000000000000000000, 0.000000000000000000, 1.000000000000000000 ) ) ;
#35870=ORIENTED_EDGE ( 'NONE', *, *, #14686, .F. ) ;
#35871=DIRECTION ( 'NONE',  ( 0.000000000000000000, 0.000000000000000000, 1.000000000000000000 ) ) ;
#35872=CARTESIAN_POINT ( 'NONE',  ( -18.00000337463124467, 69.28203230275516944, -9.999999999999998224 ) ) ;
#35874=ORIENTED_EDGE ( 'NONE', *, *, #23643, .F. ) ;
#35875=ORIENTED_EDGE ( 'NONE', *, *, #26535, .F. ) ;
#35876=ORIENTED_EDGE ( 'NONE', *, *, #18119, .F. ) ;
#35879=EDGE_CURVE ( 'NONE', #17794, #12035, #11707, .T. ) ;
#35881=DIRECTION ( 'NONE',  ( 1.000000000000000000, 0.000000000000000000, 0.000000000000000000 ) ) ;
#35882=AXIS2_PLACEMENT_3D ( 'NONE', #30330, #4667, #1843 ) ;
#35883=VERTEX_POINT ( 'NONE', #32720 ) ;
#35884=ORIENTED_EDGE ( 'NONE', *, *, #34757, .F. ) ;
#35885=FACE_BOUND ( 'NONE', #10586, .T. ) ;
#35886=EDGE_LOOP ( 'NONE', ( #16813, #18883 ) ) ;
#35887=ORIENTED_EDGE ( 'NONE', *, *, #12860, .T. ) ;
#35888=ADVANCED_FACE ( 'NONE', ( #17930 ), #4049, .F. ) ;
#35889=EDGE_CURVE ( 'NONE', #11035, #21946, #29072, .T. ) ;
#35890=DIRECTION ( 'NONE',  ( -1.000000000000000000, 0.000000000000000000, 0.000000000000000000 ) ) ;
#35892=DIRECTION ( 'NONE',  ( 1.000000000000000000, 0.000000000000000000, 0.000000000000000000 ) ) ;
#35893=ORIENTED_EDGE ( 'NONE', *, *, #24225, .F. ) ;
#35895=CARTESIAN_POINT ( 'NONE',  ( -12.00000337463128908, 69.28203230275516944, -9.999999999999998224 ) ) ;
#35896=AXIS2_PLACEMENT_3D ( 'NONE', #34007, #19750, #33804 ) ;
#35897=DIRECTION ( 'NONE',  ( -0.000000000000000000, -0.000000000000000000, 1.000000000000000000 ) ) ;
#35899=LINE ( 'NONE', #16016, #33441 ) ;
#35901=CARTESIAN_POINT ( 'NONE',  ( 9.999996625368618552, 69.28203230275516944, -9.999999999999998224 ) ) ;
#35903=ORIENTED_EDGE ( 'NONE', *, *, #4007, .F. ) ;
#35904=EDGE_CURVE ( 'NONE', #21552, #25354, #15671, .T. ) ;
#35905=CARTESIAN_POINT ( 'NONE',  ( -68.00000337463099243, -2.428612866367529932E-14, 12.50000000000000000 ) ) ;
#35906=DIRECTION ( 'NONE',  ( -1.000000000000000000, 0.000000000000000000, -0.000000000000000000 ) ) ;
#35907=CARTESIAN_POINT ( 'NONE',  ( 27.99999662536857414, -69.28203230275519786, 17.49999999999999645 ) ) ;
#35908=CARTESIAN_POINT ( 'NONE',  ( 84.99999662536832545, 8.660254037844394404, -9.999999999999998224 ) ) ;
#35909=AXIS2_PLACEMENT_3D ( 'NONE', #2402, #28425, #2753 ) ;
#35910=DIRECTION ( 'NONE',  ( -1.000000000000000000, 0.000000000000000000, 0.000000000000000000 ) ) ;
#35911=AXIS2_PLACEMENT_3D ( 'NONE', #7420, #18860, #30283 ) ;
#35912=DIRECTION ( 'NONE',  ( 1.000000000000000000, 0.000000000000000000, 0.000000000000000000 ) ) ;
#35913=DIRECTION ( 'NONE',  ( 1.000000000000000000, 0.000000000000000000, 0.000000000000000000 ) ) ;
#35914=AXIS2_PLACEMENT_3D ( 'NONE', #8332, #22017, #5681 ) ;
#35915=ORIENTED_EDGE ( 'NONE', *, *, #1129, .T. ) ;
#35918=CYLINDRICAL_SURFACE ( 'NONE', #27117, 2.000000000000001776 ) ;
#35919=VERTEX_POINT ( 'NONE', #35555 ) ;
#35920=ORIENTED_EDGE ( 'NONE', *, *, #25367, .T. ) ;
#35921=ORIENTED_EDGE ( 'NONE', *, *, #4995, .F. ) ;
#35922=AXIS2_PLACEMENT_3D ( 'NONE', #34826, #9120, #14953 ) ;
#35926=AXIS2_PLACEMENT_3D ( 'NONE', #304, #8574, #34454 ) ;
#35927=ORIENTED_EDGE ( 'NONE', *, *, #15047, .T. ) ;
#35928=EDGE_CURVE ( 'NONE', #12074, #20954, #24300, .T. ) ;
#35929=CYLINDRICAL_SURFACE ( 'NONE', #32893, 2.000000000000001776 ) ;
#35930=DIRECTION ( 'NONE',  ( 1.000000000000000000, 0.000000000000000000, 0.000000000000000000 ) ) ;
#35931=ORIENTED_EDGE ( 'NONE', *, *, #4844, .T. ) ;
#35932=CARTESIAN_POINT ( 'NONE',  ( 49.99999662536848177, -51.96152422706640550, -9.999999999999998224 ) ) ;
#35934=VERTEX_POINT ( 'NONE', #29525 ) ;
#35935=DIRECTION ( 'NONE',  ( 0.000000000000000000, 0.000000000000000000, -1.000000000000000000 ) ) ;
#35936=AXIS2_PLACEMENT_3D ( 'NONE', #26682, #20676, #26131 ) ;
#35938=EDGE_CURVE ( 'NONE', #8999, #4753, #26728, .T. ) ;
#35939=CARTESIAN_POINT ( 'NONE',  ( 74.99999662536836809, -8.660254037844401509, 12.50000000000000000 ) ) ;
#35940=CARTESIAN_POINT ( 'NONE',  ( -27.00000337463121625, -77.94228634059963667, -9.999999999999998224 ) ) ;
#35941=DIRECTION ( 'NONE',  ( 0.8660254037844337116, -0.5000000000000084377, 0.000000000000000000 ) ) ;
#35942=CIRCLE ( 'NONE', #32332, 2.000000000000001776 ) ;
#35945=VECTOR ( 'NONE', #28143, 1000.000000000000000 ) ;
#35948=CARTESIAN_POINT ( 'NONE',  ( 4.279621169095998212, -62.97617850287780072, 12.49999999999999822 ) ) ;
#35949=CIRCLE ( 'NONE', #4793, 2.000000000000001776 ) ;
#35950=FACE_OUTER_BOUND ( 'NONE', #34218, .T. ) ;
#35951=CARTESIAN_POINT ( 'NONE',  ( -32.00000337463119848, -69.28203230275522628, -5.000000000000000000 ) ) ;
#35952=EDGE_LOOP ( 'NONE', ( #7514, #25040 ) ) ;
#35953=DIRECTION ( 'NONE',  ( 1.000000000000000000, 0.000000000000000000, 0.000000000000000000 ) ) ;
#35954=CIRCLE ( 'NONE', #29346, 2.000000000000001776 ) ;
#35955=DIRECTION ( 'NONE',  ( 1.000000000000000000, 0.000000000000000000, 0.000000000000000000 ) ) ;
#35956=DIRECTION ( 'NONE',  ( 1.000000000000000000, 0.000000000000000000, 0.000000000000000000 ) ) ;
#35958=ORIENTED_EDGE ( 'NONE', *, *, #884, .T. ) ;
#35960=AXIS2_PLACEMENT_3D ( 'NONE', #22938, #34377, #28197 ) ;
#35961=CARTESIAN_POINT ( 'NONE',  ( -19.13981058454750794, 60.93295298010998806, 12.49999999999999822 ) ) ;
#35962=DIRECTION ( 'NONE',  ( 0.000000000000000000, 0.000000000000000000, 1.000000000000000000 ) ) ;
#35964=DIRECTION ( 'NONE',  ( 1.000000000000000000, 0.000000000000000000, 0.000000000000000000 ) ) ;
#35965=ORIENTED_EDGE ( 'NONE', *, *, #14997, .T. ) ;
#35966=EDGE_CURVE ( 'NONE', #11272, #6451, #31513, .T. ) ;
#35967=AXIS2_PLACEMENT_3D ( 'NONE', #29646, #35490, #27410 ) ;
#35968=CARTESIAN_POINT ( 'NONE',  ( 74.99999662536835388, -25.98076211353319565, 17.49999999999999645 ) ) ;
#35969=CARTESIAN_POINT ( 'NONE',  ( 46.99999662536851019, 77.94228634059959404, 12.50000000000000000 ) ) ;
#35970=CARTESIAN_POINT ( 'NONE',  ( -73.00000337463099243, -25.98076211353322051, 12.50000000000000000 ) ) ;
#35971=AXIS2_PLACEMENT_3D ( 'NONE', #36554, #13115, #30349 ) ;
#35976=DIRECTION ( 'NONE',  ( 0.000000000000000000, 0.000000000000000000, 1.000000000000000000 ) ) ;
#35977=ORIENTED_EDGE ( 'NONE', *, *, #34602, .T. ) ;
#35979=VERTEX_POINT ( 'NONE', #13390 ) ;
#35980=DIRECTION ( 'NONE',  ( 1.000000000000000000, 0.000000000000000000, 0.000000000000000000 ) ) ;
#35981=EDGE_CURVE ( 'NONE', #35025, #4037, #7963, .T. ) ;
#35982=CARTESIAN_POINT ( 'NONE',  ( 29.99999662536856349, 69.28203230275518365, -9.999999999999998224 ) ) ;
#35983=EDGE_LOOP ( 'NONE', ( #3784, #1380 ) ) ;
#35985=EDGE_LOOP ( 'NONE', ( #30988, #17372 ) ) ;
#35987=DIRECTION ( 'NONE',  ( 0.000000000000000000, 0.000000000000000000, 1.000000000000000000 ) ) ;
#35988=DIRECTION ( 'NONE',  ( -1.000000000000000000, 1.798972493605576793E-15, 0.000000000000000000 ) ) ;
#35989=AXIS2_PLACEMENT_3D ( 'NONE', #4877, #5239, #16676 ) ;
#35991=DIRECTION ( 'NONE',  ( 1.000000000000000000, 0.000000000000000000, 0.000000000000000000 ) ) ;
#35992=DIRECTION ( 'NONE',  ( 0.000000000000000000, 0.000000000000000000, 1.000000000000000000 ) ) ;
#35993=CARTESIAN_POINT ( 'NONE',  ( 37.27962116909601065, -62.97617850287780072, -49.86561046011506448 ) ) ;
#35995=EDGE_LOOP ( 'NONE', ( #24867, #16323, #30585, #6211 ) ) ;
#35996=EDGE_CURVE ( 'NONE', #26912, #902, #16404, .T. ) ;
#35997=ORIENTED_EDGE ( 'NONE', *, *, #19426, .T. ) ;
#35998=PLANE ( 'NONE',  #26027 ) ;
#35999=DIRECTION ( 'NONE',  ( 0.000000000000000000, 0.000000000000000000, 1.000000000000000000 ) ) ;
#36000=EDGE_CURVE ( 'NONE', #7804, #2324, #27289, .T. ) ;
#36001=ORIENTED_EDGE ( 'NONE', *, *, #28659, .T. ) ;
#36002=CARTESIAN_POINT ( 'NONE',  ( -73.00000337463099243, -25.98076211353322051, -9.999999999999998224 ) ) ;
#36003=FACE_OUTER_BOUND ( 'NONE', #10720, .T. ) ;
#36004=LINE ( 'NONE', #10298, #17639 ) ;
#36005=EDGE_CURVE ( 'NONE', #21455, #6156, #2136, .T. ) ;
#36006=FACE_OUTER_BOUND ( 'NONE', #30056, .T. ) ;
#36007=DIRECTION ( 'NONE',  ( 0.000000000000000000, 0.000000000000000000, 1.000000000000000000 ) ) ;
#36008=CARTESIAN_POINT ( 'NONE',  ( 87.99999662536828282, 2.449293598294703949E-16, 12.50000000000000000 ) ) ;
#36009=ADVANCED_FACE ( 'NONE', ( #7597 ), #16594, .F. ) ;
#36010=CARTESIAN_POINT ( 'NONE',  ( 11.99999662536861855, 69.28203230275516944, -9.999999999999998224 ) ) ;
#36011=EDGE_CURVE ( 'NONE', #30228, #21906, #23090, .T. ) ;
#36012=PLANE ( 'NONE',  #32819 ) ;
#36013=ORIENTED_EDGE ( 'NONE', *, *, #11358, .F. ) ;
#36014=ORIENTED_EDGE ( 'NONE', *, *, #31749, .F. ) ;
#36015=LINE ( 'NONE', #7140, #24240 ) ;
#36017=DIRECTION ( 'NONE',  ( -1.000000000000000000, 0.000000000000000000, 0.000000000000000000 ) ) ;
#36018=CARTESIAN_POINT ( 'NONE',  ( 84.99999662536831124, -25.98076211353319565, -9.999999999999998224 ) ) ;
#36019=ORIENTED_EDGE ( 'NONE', *, *, #17401, .F. ) ;
#36020=ADVANCED_FACE ( 'NONE', ( #18852 ), #33090, .F. ) ;
#36021=LINE ( 'NONE', #9755, #15956 ) ;
#36023=DIRECTION ( 'NONE',  ( 1.000000000000000000, 0.000000000000000000, 0.000000000000000000 ) ) ;
#36024=ADVANCED_FACE ( 'NONE', ( #25229 ), #8646, .F. ) ;
#36026=ORIENTED_EDGE ( 'NONE', *, *, #33247, .T. ) ;
#36028=CARTESIAN_POINT ( 'NONE',  ( 4.999996625368676284, -77.94228634059960825, -9.999999999999998224 ) ) ;
#36029=ORIENTED_EDGE ( 'NONE', *, *, #6046, .T. ) ;
#36030=DIRECTION ( 'NONE',  ( 0.000000000000000000, 0.000000000000000000, 1.000000000000000000 ) ) ;
#36032=DIRECTION ( 'NONE',  ( 0.000000000000000000, 0.000000000000000000, 1.000000000000000000 ) ) ;
#36033=EDGE_LOOP ( 'NONE', ( #25905, #5923, #12461, #22111 ) ) ;
#36035=AXIS2_PLACEMENT_3D ( 'NONE', #27175, #21936, #27733 ) ;
#36036=LINE ( 'NONE', #18967, #2407 ) ;
#36037=ADVANCED_FACE ( 'NONE', ( #13224 ), #24671, .F. ) ;
#36040=FACE_OUTER_BOUND ( 'NONE', #27101, .T. ) ;
#36041=CARTESIAN_POINT ( 'NONE',  ( -55.00000337463110611, -43.30127018922202353, 17.49999999999999645 ) ) ;
#36043=LINE ( 'NONE', #24781, #30894 ) ;
#36045=DIRECTION ( 'NONE',  ( 0.000000000000000000, 0.000000000000000000, -1.000000000000000000 ) ) ;
#36046=DIRECTION ( 'NONE',  ( 1.000000000000000000, 0.000000000000000000, 0.000000000000000000 ) ) ;
#36047=DIRECTION ( 'NONE',  ( 0.000000000000000000, 0.000000000000000000, -1.000000000000000000 ) ) ;
#36048=EDGE_LOOP ( 'NONE', ( #13463, #27476, #16344 ) ) ;
#36049=DIRECTION ( 'NONE',  ( 1.000000000000000000, 0.000000000000000000, 0.000000000000000000 ) ) ;
#36050=CARTESIAN_POINT ( 'NONE',  ( -65.00000337463104927, -43.30127018922202353, -5.000000000000000000 ) ) ;
#36051=VERTEX_POINT ( 'NONE', #19050 ) ;
#36053=AXIS2_PLACEMENT_3D ( 'NONE', #20896, #24077, #32326 ) ;
#36054=CYLINDRICAL_SURFACE ( 'NONE', #34292, 2.000000000000001776 ) ;
#36055=FACE_OUTER_BOUND ( 'NONE', #19053, .T. ) ;
#36056=DIRECTION ( 'NONE',  ( -1.000000000000000000, 0.000000000000000000, 0.000000000000000000 ) ) ;
#36057=ORIENTED_EDGE ( 'NONE', *, *, #28400, .T. ) ;
#36058=ORIENTED_EDGE ( 'NONE', *, *, #10289, .T. ) ;
#36059=EDGE_LOOP ( 'NONE', ( #26264, #27303, #33389, #24707, #33477, #2390, #23175, #31878, #11147, #22996, #14705, #15044, #3911, #1, #32844, #12291, #24502, #35232, #35255, #21620, #18271, #4751, #33532, #36514 ) ) ;
#36060=ADVANCED_FACE ( 'NONE', ( #4800 ), #10596, .T. ) ;
#36061=DIRECTION ( 'NONE',  ( 0.000000000000000000, 0.000000000000000000, 1.000000000000000000 ) ) ;
#36062=EDGE_CURVE ( 'NONE', #22987, #29936, #30646, .T. ) ;
#36063=ORIENTED_EDGE ( 'NONE', *, *, #25666, .F. ) ;
#36064=EDGE_CURVE ( 'NONE', #16030, #24141, #24901, .T. ) ;
#36065=DIRECTION ( 'NONE',  ( -1.000000000000000000, 0.000000000000000000, 0.000000000000000000 ) ) ;
#36067=EDGE_LOOP ( 'NONE', ( #19987, #4562, #34192, #23666, #3083, #5138 ) ) ;
#36068=CARTESIAN_POINT ( 'NONE',  ( 34.99999662536853862, 77.94228634059959404, 17.49999999999999645 ) ) ;
#36069=DIRECTION ( 'NONE',  ( 0.000000000000000000, 0.000000000000000000, 1.000000000000000000 ) ) ;
#36071=ORIENTED_EDGE ( 'NONE', *, *, #1175, .T. ) ;
#36073=CARTESIAN_POINT ( 'NONE',  ( -20.00000337463122690, 86.60254037844397601, -9.999999999999998224 ) ) ;
#36074=DIRECTION ( 'NONE',  ( 1.000000000000000000, 0.000000000000000000, 0.000000000000000000 ) ) ;
#36075=CARTESIAN_POINT ( 'NONE',  ( 37.99999662536853151, 69.28203230275518365, 12.50000000000000000 ) ) ;
#36076=EDGE_LOOP ( 'NONE', ( #3886, #26231 ) ) ;
#36077=DIRECTION ( 'NONE',  ( 0.000000000000000000, 0.000000000000000000, 1.000000000000000000 ) ) ;
#36079=VERTEX_POINT ( 'NONE', #12002 ) ;
#36080=CARTESIAN_POINT ( 'NONE',  ( 33.99999999999986500, -58.88972745734191250, 12.49999999999999822 ) ) ;
#36082=CARTESIAN_POINT ( 'NONE',  ( 89.99999662536828282, 0.000000000000000000, -5.000000000000000000 ) ) ;
#36083=DIRECTION ( 'NONE',  ( -1.000000000000000000, 0.000000000000000000, 0.000000000000000000 ) ) ;
#36084=EDGE_CURVE ( 'NONE', #11718, #32638, #13505, .T. ) ;
#36085=DIRECTION ( 'NONE',  ( 0.000000000000000000, 0.000000000000000000, 1.000000000000000000 ) ) ;
#36086=CARTESIAN_POINT ( 'NONE',  ( 1.999996625368672287, 86.60254037844397601, -9.999999999999998224 ) ) ;
#36087=CARTESIAN_POINT ( 'NONE',  ( 29.99999662536856349, 69.28203230275518365, -9.999999999999998224 ) ) ;
#36088=VERTEX_POINT ( 'NONE', #757 ) ;
#36089=DIRECTION ( 'NONE',  ( -1.000000000000000000, 0.000000000000000000, 0.000000000000000000 ) ) ;
#36090=DIRECTION ( 'NONE',  ( 0.000000000000000000, 0.000000000000000000, 1.000000000000000000 ) ) ;
#36091=DIRECTION ( 'NONE',  ( 0.000000000000000000, 0.000000000000000000, -1.000000000000000000 ) ) ;
#36092=ORIENTED_EDGE ( 'NONE', *, *, #34655, .F. ) ;
#36094=VECTOR ( 'NONE', #23494, 1000.000000000000000 ) ;
#36095=ORIENTED_EDGE ( 'NONE', *, *, #20590, .F. ) ;
#36096=VERTEX_POINT ( 'NONE', #23460 ) ;
#36097=CARTESIAN_POINT ( 'NONE',  ( -45.00000337463112743, -60.62177826491080168, -9.999999999999998224 ) ) ;
#36098=CARTESIAN_POINT ( 'NONE',  ( -3.374631303565411855E-06, -86.60254037844400443, 12.50000000000000000 ) ) ;
#36099=ORIENTED_EDGE ( 'NONE', *, *, #33285, .F. ) ;
#36100=DIRECTION ( 'NONE',  ( 0.000000000000000000, 0.000000000000000000, 1.000000000000000000 ) ) ;
#36101=AXIS2_PLACEMENT_3D ( 'NONE', #20802, #26054, #6566 ) ;
#36102=DIRECTION ( 'NONE',  ( 0.000000000000000000, 0.000000000000000000, 1.000000000000000000 ) ) ;
#36103=EDGE_LOOP ( 'NONE', ( #16717, #22720 ) ) ;
#36105=AXIS2_PLACEMENT_3D ( 'NONE', #24659, #36091, #10388 ) ;
#36107=VERTEX_POINT ( 'NONE', #17459 ) ;
#36110=DIRECTION ( 'NONE',  ( 0.000000000000000000, 0.000000000000000000, 1.000000000000000000 ) ) ;
#36111=CYLINDRICAL_SURFACE ( 'NONE', #3798, 2.000000000000001776 ) ;
#36113=CARTESIAN_POINT ( 'NONE',  ( -85.00000337463092137, -8.660254037844422825, -9.999999999999998224 ) ) ;
#36114=DIRECTION ( 'NONE',  ( -1.000000000000000000, 0.000000000000000000, 0.000000000000000000 ) ) ;
#36116=AXIS2_PLACEMENT_3D ( 'NONE', #7693, #28286, #2247 ) ;
#36117=EDGE_LOOP ( 'NONE', ( #8768, #14973 ) ) ;
#36120=ORIENTED_EDGE ( 'NONE', *, *, #27169, .T. ) ;
#36122=DIRECTION ( 'NONE',  ( 0.000000000000000000, 0.000000000000000000, 1.000000000000000000 ) ) ;
#36123=PLANE ( 'NONE',  #8777 ) ;
#36124=EDGE_CURVE ( 'NONE', #8997, #15428, #35714, .T. ) ;
#36125=VERTEX_POINT ( 'NONE', #15195 ) ;
#36126=AXIS2_PLACEMENT_3D ( 'NONE', #15271, #10025, #1223 ) ;
#36127=VERTEX_POINT ( 'NONE', #29062 ) ;
#36128=EDGE_CURVE ( 'NONE', #15570, #2260, #3203, .T. ) ;
#36130=CARTESIAN_POINT ( 'NONE',  ( -42.00000337463114164, -69.28203230275519786, 17.49999999999999645 ) ) ;
#36132=ORIENTED_EDGE ( 'NONE', *, *, #30860, .F. ) ;
#36133=EDGE_CURVE ( 'NONE', #29875, #12814, #26079, .T. ) ;
#36134=ORIENTED_EDGE ( 'NONE', *, *, #19432, .T. ) ;
#36135=DIRECTION ( 'NONE',  ( -1.000000000000000000, -1.798972493605577187E-15, 0.000000000000000000 ) ) ;
#36137=CARTESIAN_POINT ( 'NONE',  ( -60.00000337463107059, -34.64101615137762025, -5.000000000000000000 ) ) ;
#36140=ORIENTED_EDGE ( 'NONE', *, *, #8299, .T. ) ;
#36141=ORIENTED_EDGE ( 'NONE', *, *, #12809, .F. ) ;
#36142=CIRCLE ( 'NONE', #13372, 2.000000000000001776 ) ;
#36144=DIRECTION ( 'NONE',  ( 1.000000000000000000, 0.000000000000000000, 0.000000000000000000 ) ) ;
#36145=ORIENTED_EDGE ( 'NONE', *, *, #11886, .T. ) ;
#36146=EDGE_CURVE ( 'NONE', #23895, #26782, #8837, .T. ) ;
#36147=CARTESIAN_POINT ( 'NONE',  ( 86.99999662536831124, -8.660254037844397956, 12.50000000000000000 ) ) ;
#36149=DIRECTION ( 'NONE',  ( 1.000000000000000000, 0.000000000000000000, 0.000000000000000000 ) ) ;
#36151=ORIENTED_EDGE ( 'NONE', *, *, #22724, .T. ) ;
#36152=CIRCLE ( 'NONE', #19981, 2.000000000000000000 ) ;
#36157=FACE_OUTER_BOUND ( 'NONE', #32672, .T. ) ;
#36158=LINE ( 'NONE', #7854, #25754 ) ;
#36159=CARTESIAN_POINT ( 'NONE',  ( 19.99999662536861678, -86.60254037844400443, -5.000000000000000000 ) ) ;
#36160=ADVANCED_FACE ( 'NONE', ( #26275 ), #21014, .F. ) ;
#36162=CARTESIAN_POINT ( 'NONE',  ( 76.99999662536836809, 8.660254037844394404, -5.000000000000000000 ) ) ;
#36163=DIRECTION ( 'NONE',  ( 0.000000000000000000, 0.000000000000000000, 1.000000000000000000 ) ) ;
#36164=CARTESIAN_POINT ( 'NONE',  ( 4.999996625368645198, 77.94228634059957983, -9.999999999999998224 ) ) ;
#36165=ORIENTED_EDGE ( 'NONE', *, *, #35597, .F. ) ;
#36167=ORIENTED_EDGE ( 'NONE', *, *, #2186, .T. ) ;
#36168=AXIS2_PLACEMENT_3D ( 'NONE', #37068, #28413, #16990 ) ;
#36170=DIRECTION ( 'NONE',  ( 0.000000000000000000, 0.000000000000000000, 1.000000000000000000 ) ) ;
#36171=VERTEX_POINT ( 'NONE', #15389 ) ;
#36172=EDGE_CURVE ( 'NONE', #3095, #18828, #36021, .T. ) ;
#36173=CARTESIAN_POINT ( 'NONE',  ( -59.29837256189559724, -31.02796211690927919, 12.49999999999999822 ) ) ;
#36174=CARTESIAN_POINT ( 'NONE',  ( 67.99999662536838230, 17.32050807568879236, -5.000000000000000000 ) ) ;
#36175=VECTOR ( 'NONE', #20290, 1000.000000000000000 ) ;
#36177=ADVANCED_FACE ( 'NONE', ( #7322 ), #33180, .F. ) ;
#36178=VECTOR ( 'NONE', #14274, 1000.000000000000000 ) ;
#36179=DIRECTION ( 'NONE',  ( -0.000000000000000000, -0.000000000000000000, 1.000000000000000000 ) ) ;
#36183=CARTESIAN_POINT ( 'NONE',  ( -68.00000337463102085, -34.64101615137762025, -9.999999999999998224 ) ) ;
#36186=CARTESIAN_POINT ( 'NONE',  ( -3.374631327851540519E-06, 86.60254037844397601, -9.999999999999998224 ) ) ;
#36188=CARTESIAN_POINT ( 'NONE',  ( -53.00000337463110611, -43.30127018922202353, 17.49999999999999645 ) ) ;
#36189=LINE ( 'NONE', #21937, #15502 ) ;
#36190=ORIENTED_EDGE ( 'NONE', *, *, #6901, .T. ) ;
#36191=CYLINDRICAL_SURFACE ( 'NONE', #28488, 2.000000000000001776 ) ;
#36192=AXIS2_PLACEMENT_3D ( 'NONE', #25818, #20524, #23373 ) ;
#36193=EDGE_CURVE ( 'NONE', #26406, #9668, #19545, .T. ) ;
#36194=DIRECTION ( 'NONE',  ( 0.000000000000000000, 0.000000000000000000, -1.000000000000000000 ) ) ;
#36195=ORIENTED_EDGE ( 'NONE', *, *, #2, .T. ) ;
#36197=EDGE_LOOP ( 'NONE', ( #26978, #18903, #26856, #33116 ) ) ;
#36199=AXIS2_PLACEMENT_3D ( 'NONE', #35475, #14643, #18025 ) ;
#36200=EDGE_CURVE ( 'NONE', #11967, #7273, #15758, .T. ) ;
#36201=CARTESIAN_POINT ( 'NONE',  ( 72.77422209630368855, 61.06482292022033675, -5.000000000000000000 ) ) ;
#36203=CARTESIAN_POINT ( 'NONE',  ( -72.00000337463102085, -34.64101615137762025, -5.000000000000000000 ) ) ;
#36204=EDGE_CURVE ( 'NONE', #35706, #7403, #24929, .T. ) ;
#36205=ORIENTED_EDGE ( 'NONE', *, *, #31123, .T. ) ;
#36206=EDGE_LOOP ( 'NONE', ( #17047, #27934, #27828, #14342 ) ) ;
#36207=EDGE_CURVE ( 'NONE', #9828, #1926, #30320, .T. ) ;
#36208=ORIENTED_EDGE ( 'NONE', *, *, #3807, .T. ) ;
#36210=DIRECTION ( 'NONE',  ( 1.000000000000000000, 0.000000000000000000, 0.000000000000000000 ) ) ;
#36211=DIRECTION ( 'NONE',  ( 0.000000000000000000, 0.000000000000000000, -1.000000000000000000 ) ) ;
#36212=CIRCLE ( 'NONE', #30198, 2.000000000000001776 ) ;
#36213=DIRECTION ( 'NONE',  ( 0.000000000000000000, 0.000000000000000000, 1.000000000000000000 ) ) ;
#36214=CARTESIAN_POINT ( 'NONE',  ( 56.99999662536846046, -43.30127018922200222, -5.000000000000000000 ) ) ;
#36215=DIRECTION ( 'NONE',  ( 0.000000000000000000, 0.000000000000000000, 1.000000000000000000 ) ) ;
#36216=VERTEX_POINT ( 'NONE', #27179 ) ;
#36218=AXIS2_PLACEMENT_3D ( 'NONE', #20076, #34336, #36778 ) ;
#36219=DIRECTION ( 'NONE',  ( 0.000000000000000000, 0.000000000000000000, -1.000000000000000000 ) ) ;
#36220=EDGE_CURVE ( 'NONE', #5553, #21436, #5169, .T. ) ;
#36221=ORIENTED_EDGE ( 'NONE', *, *, #19233, .T. ) ;
#36223=DIRECTION ( 'NONE',  ( 1.000000000000000000, 0.000000000000000000, 0.000000000000000000 ) ) ;
#36225=VERTEX_POINT ( 'NONE', #24393 ) ;
#36228=ORIENTED_EDGE ( 'NONE', *, *, #10098, .T. ) ;
#36229=CARTESIAN_POINT ( 'NONE',  ( 0.000000000000000000, 0.000000000000000000, -5.000000000000000000 ) ) ;
#36230=DIRECTION ( 'NONE',  ( 0.000000000000000000, 0.000000000000000000, 1.000000000000000000 ) ) ;
#36231=DIRECTION ( 'NONE',  ( 0.000000000000000000, 0.000000000000000000, 1.000000000000000000 ) ) ;
#36232=VERTEX_POINT ( 'NONE', #35839 ) ;
#36233=EDGE_LOOP ( 'NONE', ( #36657, #2873 ) ) ;
#36234=ORIENTED_EDGE ( 'NONE', *, *, #7039, .F. ) ;
#36235=CARTESIAN_POINT ( 'NONE',  ( -20.00000337463122690, 86.60254037844397601, -9.999999999999998224 ) ) ;
#36238=ORIENTED_EDGE ( 'NONE', *, *, #15861, .T. ) ;
#36239=EDGE_CURVE ( 'NONE', #31490, #29904, #984, .T. ) ;
#36240=VECTOR ( 'NONE', #19425, 1000.000000000000000 ) ;
#36241=FACE_BOUND ( 'NONE', #4117, .T. ) ;
#36244=EDGE_CURVE ( 'NONE', #14173, #6793, #8165, .T. ) ;
#36245=AXIS2_PLACEMENT_3D ( 'NONE', #32572, #17415, #3887 ) ;
#36247=FACE_OUTER_BOUND ( 'NONE', #20587, .T. ) ;
#36248=VERTEX_POINT ( 'NONE', #27380 ) ;
#36249=VERTEX_POINT ( 'NONE', #7501 ) ;
#36250=ADVANCED_FACE ( 'NONE', ( #33007 ), #30374, .T. ) ;
#36251=DIRECTION ( 'NONE',  ( 0.000000000000000000, 0.000000000000000000, 1.000000000000000000 ) ) ;
#36252=CYLINDRICAL_SURFACE ( 'NONE', #2787, 2.000000000000001776 ) ;
#36254=CIRCLE ( 'NONE', #12863, 2.000000000000001776 ) ;
#36255=DIRECTION ( 'NONE',  ( 1.000000000000000000, 0.000000000000000000, 0.000000000000000000 ) ) ;
#36256=CIRCLE ( 'NONE', #36836, 2.000000000000001776 ) ;
#36257=CARTESIAN_POINT ( 'NONE',  ( 59.99999662536843914, -34.64101615137759893, -9.999999999999998224 ) ) ;
#36258=VERTEX_POINT ( 'NONE', #32621 ) ;
#36260=FACE_BOUND ( 'NONE', #3762, .T. ) ;
#36261=CARTESIAN_POINT ( 'NONE',  ( 71.99999662536839651, 17.32050807568879236, 12.50000000000000000 ) ) ;
#36262=LINE ( 'NONE', #7388, #5815 ) ;
#36263=CARTESIAN_POINT ( 'NONE',  ( -83.00000337463092137, 25.98076211353317433, -9.999999999999998224 ) ) ;
#36264=EDGE_CURVE ( 'NONE', #33803, #28072, #29102, .T. ) ;
#36265=DIRECTION ( 'NONE',  ( 1.000000000000000000, 0.000000000000000000, 0.000000000000000000 ) ) ;
#36266=EDGE_CURVE ( 'NONE', #30829, #9726, #12334, .T. ) ;
#36267=CYLINDRICAL_SURFACE ( 'NONE', #25768, 2.000000000000001776 ) ;
#36268=ADVANCED_FACE ( 'NONE', ( #4079 ), #318, .F. ) ;
#36270=EDGE_CURVE ( 'NONE', #34308, #20758, #33328, .T. ) ;
#36271=DIRECTION ( 'NONE',  ( 1.000000000000000000, 0.000000000000000000, 0.000000000000000000 ) ) ;
#36273=DIRECTION ( 'NONE',  ( 1.000000000000000000, 0.000000000000000000, 0.000000000000000000 ) ) ;
#36276=DIRECTION ( 'NONE',  ( 0.000000000000000000, 0.000000000000000000, -1.000000000000000000 ) ) ;
#36277=CIRCLE ( 'NONE', #13504, 2.000000000000000000 ) ;
#36278=AXIS2_PLACEMENT_3D ( 'NONE', #22039, #7792, #19234 ) ;
#36279=VERTEX_POINT ( 'NONE', #21129 ) ;
#36280=AXIS2_PLACEMENT_3D ( 'NONE', #33333, #10443, #13077 ) ;
#36281=ORIENTED_EDGE ( 'NONE', *, *, #659, .T. ) ;
#36282=VERTEX_POINT ( 'NONE', #6875 ) ;
#36286=VECTOR ( 'NONE', #4996, 1000.000000000000000 ) ;
#36287=CARTESIAN_POINT ( 'NONE',  ( -25.00000337463121980, -77.94228634059963667, -5.000000000000000000 ) ) ;
#36289=EDGE_LOOP ( 'NONE', ( #1202, #10790 ) ) ;
#36290=LINE ( 'NONE', #7599, #15582 ) ;
#36292=FACE_BOUND ( 'NONE', #28426, .T. ) ;
#36293=AXIS2_PLACEMENT_3D ( 'NONE', #7569, #36077, #1566 ) ;
#36295=DIRECTION ( 'NONE',  ( 1.000000000000000000, 0.000000000000000000, 0.000000000000000000 ) ) ;
#36296=VECTOR ( 'NONE', #610, 1000.000000000000000 ) ;
#36297=CARTESIAN_POINT ( 'NONE',  ( -2.000003374631289521, -69.28203230275519786, -9.999999999999998224 ) ) ;
#36300=DIRECTION ( 'NONE',  ( 1.000000000000000000, 0.000000000000000000, 0.000000000000000000 ) ) ;
#36301=AXIS2_PLACEMENT_3D ( 'NONE', #6945, #4150, #9943 ) ;
#36303=DIRECTION ( 'NONE',  ( -0.000000000000000000, -0.000000000000000000, 1.000000000000000000 ) ) ;
#36304=LINE ( 'NONE', #16417, #8069 ) ;
#36305=AXIS2_PLACEMENT_3D ( 'NONE', #6406, #26462, #23654 ) ;
#36306=ORIENTED_EDGE ( 'NONE', *, *, #12116, .F. ) ;
#36307=DIRECTION ( 'NONE',  ( 0.000000000000000000, 0.000000000000000000, -1.000000000000000000 ) ) ;
#36308=DIRECTION ( 'NONE',  ( 1.000000000000000000, 0.000000000000000000, 0.000000000000000000 ) ) ;
#36309=ORIENTED_EDGE ( 'NONE', *, *, #21590, .T. ) ;
#36311=PLANE ( 'NONE',  #20862 ) ;
#36312=DIRECTION ( 'NONE',  ( 0.000000000000000000, 0.000000000000000000, -1.000000000000000000 ) ) ;
#36314=AXIS2_PLACEMENT_3D ( 'NONE', #8750, #34441, #31075 ) ;
#36315=EDGE_LOOP ( 'NONE', ( #31015, #33377 ) ) ;
#36319=DIRECTION ( 'NONE',  ( 1.000000000000000000, 0.000000000000000000, 0.000000000000000000 ) ) ;
#36320=CIRCLE ( 'NONE', #26724, 2.000000000000001776 ) ;
#36321=CARTESIAN_POINT ( 'NONE',  ( -68.00000337463099243, 34.64101615137758472, -9.999999999999998224 ) ) ;
#36322=ORIENTED_EDGE ( 'NONE', *, *, #32059, .F. ) ;
#36323=VERTEX_POINT ( 'NONE', #29744 ) ;
#36325=LINE ( 'NONE', #27863, #33782 ) ;
#36326=CARTESIAN_POINT ( 'NONE',  ( -65.00000337463106348, -60.62177826491083010, -5.000000000000000000 ) ) ;
#36329=CIRCLE ( 'NONE', #2191, 2.000000000000001776 ) ;
#36330=AXIS2_PLACEMENT_3D ( 'NONE', #25755, #17645, #36997 ) ;
#36332=AXIS2_PLACEMENT_3D ( 'NONE', #35939, #29924, #4618 ) ;
#36333=ORIENTED_EDGE ( 'NONE', *, *, #3445, .F. ) ;
#36335=EDGE_LOOP ( 'NONE', ( #6293, #14669 ) ) ;
#36336=DIRECTION ( 'NONE',  ( 0.000000000000000000, 0.000000000000000000, 1.000000000000000000 ) ) ;
#36337=CIRCLE ( 'NONE', #13570, 2.000000000000001776 ) ;
#36338=DIRECTION ( 'NONE',  ( 0.000000000000000000, 0.000000000000000000, 1.000000000000000000 ) ) ;
#36339=ORIENTED_EDGE ( 'NONE', *, *, #6085, .F. ) ;
#36340=CARTESIAN_POINT ( 'NONE',  ( -60.00000337463104216, 34.64101615137757051, -9.999999999999998224 ) ) ;
#36341=ORIENTED_EDGE ( 'NONE', *, *, #16973, .T. ) ;
#36342=DIRECTION ( 'NONE',  ( 0.000000000000000000, 0.000000000000000000, 1.000000000000000000 ) ) ;
#36343=EDGE_CURVE ( 'NONE', #29568, #31223, #20123, .T. ) ;
#36347=CARTESIAN_POINT ( 'NONE',  ( 21.99999662536857770, 86.60254037844397601, -9.999999999999998224 ) ) ;
#36348=EDGE_LOOP ( 'NONE', ( #8636, #34373, #20132, #34517, #19662, #19784, #13176, #9016 ) ) ;
#36349=CARTESIAN_POINT ( 'NONE',  ( 59.99999662536843914, -34.64101615137759893, -9.999999999999998224 ) ) ;
#36350=EDGE_CURVE ( 'NONE', #36323, #31828, #34498, .T. ) ;
#36351=AXIS2_PLACEMENT_3D ( 'NONE', #10297, #24369, #21729 ) ;
#36352=CARTESIAN_POINT ( 'NONE',  ( -30.00000337463118427, 69.28203230275516944, -5.000000000000000000 ) ) ;
#36353=CARTESIAN_POINT ( 'NONE',  ( -75.00000337463097821, 43.30127018922197379, 17.49999999999999645 ) ) ;
#36354=EDGE_LOOP ( 'NONE', ( #18569, #36888 ) ) ;
#36355=CARTESIAN_POINT ( 'NONE',  ( 47.99999662536846756, -69.28203230275519786, -9.999999999999998224 ) ) ;
#36356=DIRECTION ( 'NONE',  ( 1.000000000000000000, 0.000000000000000000, 0.000000000000000000 ) ) ;
#36357=DIRECTION ( 'NONE',  ( 0.000000000000000000, 0.000000000000000000, 1.000000000000000000 ) ) ;
#36358=VERTEX_POINT ( 'NONE', #31807 ) ;
#36359=VECTOR ( 'NONE', #24498, 1000.000000000000000 ) ;
#36360=CIRCLE ( 'NONE', #33980, 2.000000000000001776 ) ;
#36361=ORIENTED_EDGE ( 'NONE', *, *, #15153, .T. ) ;
#36362=AXIS2_PLACEMENT_3D ( 'NONE', #36137, #24705, #21695 ) ;
#36365=EDGE_CURVE ( 'NONE', #34263, #32378, #6141, .T. ) ;
#36366=CARTESIAN_POINT ( 'NONE',  ( 74.99999662536835388, -43.30127018922199511, -9.999999999999998224 ) ) ;
#36367=VERTEX_POINT ( 'NONE', #3327 ) ;
#36369=CARTESIAN_POINT ( 'NONE',  ( -85.00000337463092137, 8.660254037844389075, 12.50000000000000000 ) ) ;
#36370=CIRCLE ( 'NONE', #1610, 2.000000000000001776 ) ;
#36371=DIRECTION ( 'NONE',  ( 1.000000000000000000, 0.000000000000000000, 0.000000000000000000 ) ) ;
#36375=CARTESIAN_POINT ( 'NONE',  ( 31.99999662536857770, -69.28203230275519786, -9.999999999999998224 ) ) ;
#36376=CARTESIAN_POINT ( 'NONE',  ( -10.00000337463127842, -69.28203230275519786, 17.49999999999999645 ) ) ;
#36378=AXIS2_PLACEMENT_3D ( 'NONE', #24609, #27590, #6769 ) ;
#36379=ORIENTED_EDGE ( 'NONE', *, *, #34402, .F. ) ;
#36380=DIRECTION ( 'NONE',  ( 0.000000000000000000, 0.000000000000000000, 1.000000000000000000 ) ) ;
#36383=CYLINDRICAL_SURFACE ( 'NONE', #14442, 2.000000000000001776 ) ;
#36385=ORIENTED_EDGE ( 'NONE', *, *, #16650, .F. ) ;
#36386=AXIS2_PLACEMENT_3D ( 'NONE', #23340, #9247, #6255 ) ;
#36388=CARTESIAN_POINT ( 'NONE',  ( 72.99999662536835388, -25.98076211353319565, -9.999999999999998224 ) ) ;
#36389=VECTOR ( 'NONE', #28218, 1000.000000000000000 ) ;
#36390=CARTESIAN_POINT ( 'NONE',  ( 69.99999662536839651, 34.64101615137758472, 17.49999999999999645 ) ) ;
#36391=ORIENTED_EDGE ( 'NONE', *, *, #2176, .F. ) ;
#36392=EDGE_CURVE ( 'NONE', #6626, #7555, #26563, .T. ) ;
#36393=DIRECTION ( 'NONE',  ( 0.000000000000000000, 0.000000000000000000, 1.000000000000000000 ) ) ;
#36395=AXIS2_PLACEMENT_3D ( 'NONE', #30302, #26940, #33307 ) ;
#36396=DIRECTION ( 'NONE',  ( 1.000000000000000000, 0.000000000000000000, 0.000000000000000000 ) ) ;
#36397=CARTESIAN_POINT ( 'NONE',  ( 84.99999662536831124, -25.98076211353319565, 17.49999999999999645 ) ) ;
#36398=DIRECTION ( 'NONE',  ( -1.000000000000000000, 0.000000000000000000, 0.000000000000000000 ) ) ;
#36399=EDGE_CURVE ( 'NONE', #30228, #26119, #522, .T. ) ;
#36400=CIRCLE ( 'NONE', #4057, 2.000000000000000000 ) ;
#36401=DIRECTION ( 'NONE',  ( -1.000000000000000000, 0.000000000000000000, 0.000000000000000000 ) ) ;
#36402=VERTEX_POINT ( 'NONE', #9316 ) ;
#36403=ORIENTED_EDGE ( 'NONE', *, *, #22280, .T. ) ;
#36404=CIRCLE ( 'NONE', #23812, 33.00000000000001421 ) ;
#36405=VECTOR ( 'NONE', #33598, 1000.000000000000000 ) ;
#36406=AXIS2_PLACEMENT_3D ( 'NONE', #19919, #28894, #3223 ) ;
#36407=VECTOR ( 'NONE', #26477, 1000.000000000000000 ) ;
#36408=ORIENTED_EDGE ( 'NONE', *, *, #13435, .F. ) ;
#36409=DIRECTION ( 'NONE',  ( 0.000000000000000000, 0.000000000000000000, 1.000000000000000000 ) ) ;
#36410=CARTESIAN_POINT ( 'NONE',  ( -83.47442710120355969, 31.09745072740822991, -49.86348611802629449 ) ) ;
#36412=DIRECTION ( 'NONE',  ( 1.000000000000000000, 0.000000000000000000, 0.000000000000000000 ) ) ;
#36413=ORIENTED_EDGE ( 'NONE', *, *, #34071, .F. ) ;
#36415=CIRCLE ( 'NONE', #16687, 2.999999999999999556 ) ;
#36416=ADVANCED_FACE ( 'NONE', ( #34835 ), #6699, .F. ) ;
#36417=CARTESIAN_POINT ( 'NONE',  ( -5.000003374631269537, -77.94228634059960825, -9.999999999999998224 ) ) ;
#36418=DIRECTION ( 'NONE',  ( 0.000000000000000000, 0.000000000000000000, 1.000000000000000000 ) ) ;
#36419=ORIENTED_EDGE ( 'NONE', *, *, #11721, .T. ) ;
#36420=FACE_OUTER_BOUND ( 'NONE', #28840, .T. ) ;
#36421=CARTESIAN_POINT ( 'NONE',  ( 78.38501592334911550, 33.46125459406803060, -5.000000000000000000 ) ) ;
#36422=AXIS2_PLACEMENT_3D ( 'NONE', #2378, #17171, #22240 ) ;
#36423=ORIENTED_EDGE ( 'NONE', *, *, #1074, .F. ) ;
#36424=EDGE_CURVE ( 'NONE', #27540, #11751, #20727, .T. ) ;
#36425=ORIENTED_EDGE ( 'NONE', *, *, #31654, .T. ) ;
#36426=CARTESIAN_POINT ( 'NONE',  ( 19.99999662536861678, -86.60254037844400443, -9.999999999999998224 ) ) ;
#36427=VECTOR ( 'NONE', #8112, 1000.000000000000000 ) ;
#36428=EDGE_CURVE ( 'NONE', #9125, #4, #32386, .T. ) ;
#36429=DIRECTION ( 'NONE',  ( 1.000000000000000000, 0.000000000000000000, 0.000000000000000000 ) ) ;
#36433=ORIENTED_EDGE ( 'NONE', *, *, #5491, .T. ) ;
#36434=AXIS2_PLACEMENT_3D ( 'NONE', #25329, #21962, #36764 ) ;
#36435=CIRCLE ( 'NONE', #21433, 2.000000000000001776 ) ;
#36436=CYLINDRICAL_SURFACE ( 'NONE', #20672, 2.000000000000001776 ) ;
#36437=VERTEX_POINT ( 'NONE', #20751 ) ;
#36438=DIRECTION ( 'NONE',  ( 1.000000000000000000, 0.000000000000000000, -0.000000000000000000 ) ) ;
#36439=ORIENTED_EDGE ( 'NONE', *, *, #29809, .T. ) ;
#36441=DIRECTION ( 'NONE',  ( 0.000000000000000000, 0.000000000000000000, 1.000000000000000000 ) ) ;
#36443=CARTESIAN_POINT ( 'NONE',  ( 0.000000000000000000, 0.000000000000000000, 12.49999999999999822 ) ) ;
#36444=ORIENTED_EDGE ( 'NONE', *, *, #2045, .T. ) ;
#36445=ORIENTED_EDGE ( 'NONE', *, *, #11688, .F. ) ;
#36446=DIRECTION ( 'NONE',  ( 1.000000000000000000, 0.000000000000000000, 0.000000000000000000 ) ) ;
#36447=AXIS2_PLACEMENT_3D ( 'NONE', #8852, #8661, #2667 ) ;
#36448=CYLINDRICAL_SURFACE ( 'NONE', #27315, 2.000000000000001776 ) ;
#36449=CARTESIAN_POINT ( 'NONE',  ( 46.99999662536849598, -77.94228634059960825, -5.000000000000000000 ) ) ;
#36450=CARTESIAN_POINT ( 'NONE',  ( -85.00000337463092137, 25.98076211353317433, 12.50000000000000000 ) ) ;
#36451=ORIENTED_EDGE ( 'NONE', *, *, #4497, .F. ) ;
#36452=CYLINDRICAL_SURFACE ( 'NONE', #6377, 2.000000000000001776 ) ;
#36453=VECTOR ( 'NONE', #28484, 1000.000000000000000 ) ;
#36454=FACE_BOUND ( 'NONE', #37100, .T. ) ;
#36456=CARTESIAN_POINT ( 'NONE',  ( 82.99999662536831124, -8.660254037844397956, 12.50000000000000000 ) ) ;
#36457=DIRECTION ( 'NONE',  ( -1.000000000000000000, 0.000000000000000000, 0.000000000000000000 ) ) ;
#36458=LINE ( 'NONE', #15823, #36846 ) ;
#36460=EDGE_CURVE ( 'NONE', #20259, #15438, #11153, .T. ) ;
#36461=LINE ( 'NONE', #28008, #27553 ) ;
#36463=DIRECTION ( 'NONE',  ( 1.000000000000000000, 0.000000000000000000, 0.000000000000000000 ) ) ;
#36464=VERTEX_POINT ( 'NONE', #23963 ) ;
#36466=DIRECTION ( 'NONE',  ( 0.000000000000000000, 0.000000000000000000, 1.000000000000000000 ) ) ;
#36467=DIRECTION ( 'NONE',  ( 0.000000000000000000, 0.000000000000000000, 1.000000000000000000 ) ) ;
#36468=DIRECTION ( 'NONE',  ( 0.000000000000000000, 0.000000000000000000, 1.000000000000000000 ) ) ;
#36469=ORIENTED_EDGE ( 'NONE', *, *, #32842, .T. ) ;
#36470=EDGE_CURVE ( 'NONE', #12555, #9993, #15878, .T. ) ;
#36471=AXIS2_PLACEMENT_3D ( 'NONE', #26099, #11839, #966 ) ;
#36474=CARTESIAN_POINT ( 'NONE',  ( 12.99999662536859901, 77.94228634059957983, 17.49999999999999645 ) ) ;
#36475=DIRECTION ( 'NONE',  ( 0.000000000000000000, 0.000000000000000000, 1.000000000000000000 ) ) ;
#36478=ADVANCED_FACE ( 'NONE', ( #18878 ), #21869, .F. ) ;
#36480=DIRECTION ( 'NONE',  ( 0.000000000000000000, 0.000000000000000000, 1.000000000000000000 ) ) ;
#36481=VECTOR ( 'NONE', #1288, 1000.000000000000000 ) ;
#36482=CARTESIAN_POINT ( 'NONE',  ( -47.00000337463111322, -77.94228634059960825, -9.999999999999998224 ) ) ;
#36483=VERTEX_POINT ( 'NONE', #30309 ) ;
#36486=CIRCLE ( 'NONE', #18522, 2.000000000000001776 ) ;
#36487=CARTESIAN_POINT ( 'NONE',  ( -67.00000337463104927, -43.30127018922202353, -9.999999999999998224 ) ) ;
#36488=EDGE_CURVE ( 'NONE', #8851, #36088, #3397, .T. ) ;
#36490=DIRECTION ( 'NONE',  ( 0.000000000000000000, 0.000000000000000000, 1.000000000000000000 ) ) ;
#36492=ADVANCED_FACE ( 'NONE', ( #16079 ), #30116, .T. ) ;
#36493=EDGE_CURVE ( 'NONE', #26110, #9484, #22073, .T. ) ;
#36496=ADVANCED_FACE ( 'NONE', ( #21311 ), #35583, .F. ) ;
#36497=VERTEX_POINT ( 'NONE', #10076 ) ;
#36498=CYLINDRICAL_SURFACE ( 'NONE', #18293, 2.000000000000001776 ) ;
#36499=CIRCLE ( 'NONE', #552, 2.000000000000001776 ) ;
#36500=DIRECTION ( 'NONE',  ( 0.000000000000000000, 0.000000000000000000, -1.000000000000000000 ) ) ;
#36501=CARTESIAN_POINT ( 'NONE',  ( -10.00000337463127842, -69.28203230275519786, -9.999999999999998224 ) ) ;
#36502=AXIS2_PLACEMENT_3D ( 'NONE', #14038, #11421, #28290 ) ;
#36503=ORIENTED_EDGE ( 'NONE', *, *, #35676, .T. ) ;
#36504=DIRECTION ( 'NONE',  ( 1.000000000000000000, 0.000000000000000000, 0.000000000000000000 ) ) ;
#36505=CARTESIAN_POINT ( 'NONE',  ( 49.99999662536846756, 51.96152422706637708, -9.999999999999998224 ) ) ;
#36507=AXIS2_PLACEMENT_3D ( 'NONE', #23530, #15654, #13013 ) ;
#36509=DIRECTION ( 'NONE',  ( 0.000000000000000000, 0.000000000000000000, 1.000000000000000000 ) ) ;
#36510=DIRECTION ( 'NONE',  ( 0.8660254037844344888, -0.5000000000000069944, 0.000000000000000000 ) ) ;
#36511=CIRCLE ( 'NONE', #2382, 2.000000000000001776 ) ;
#36514=ORIENTED_EDGE ( 'NONE', *, *, #33002, .F. ) ;
#36515=AXIS2_PLACEMENT_3D ( 'NONE', #32976, #30147, #19116 ) ;
#36516=CARTESIAN_POINT ( 'NONE',  ( 0.000000000000000000, 0.000000000000000000, -5.000000000000000000 ) ) ;
#36517=DIRECTION ( 'NONE',  ( 1.000000000000000000, 0.000000000000000000, 0.000000000000000000 ) ) ;
#36518=CARTESIAN_POINT ( 'NONE',  ( -89.27079897466127534, 32.49191361593859995, -5.000000000000000000 ) ) ;
#36519=ORIENTED_EDGE ( 'NONE', *, *, #37103, .F. ) ;
#36526=VERTEX_POINT ( 'NONE', #10629 ) ;
#36527=CARTESIAN_POINT ( 'NONE',  ( 84.99999662536831124, -25.98076211353319565, -9.999999999999998224 ) ) ;
#36528=CIRCLE ( 'NONE', #8966, 3.000000000000002665 ) ;
#36529=CARTESIAN_POINT ( 'NONE',  ( 29.99999662536856349, 69.28203230275518365, -5.000000000000000000 ) ) ;
#36531=AXIS2_PLACEMENT_3D ( 'NONE', #15610, #6972, #33208 ) ;
#36532=DIRECTION ( 'NONE',  ( 0.000000000000000000, 0.000000000000000000, 1.000000000000000000 ) ) ;
#36533=EDGE_LOOP ( 'NONE', ( #18996, #22432, #2356, #4155 ) ) ;
#36534=DIRECTION ( 'NONE',  ( 1.000000000000000000, 0.000000000000000000, 0.000000000000000000 ) ) ;
#36536=EDGE_CURVE ( 'NONE', #4653, #22919, #6981, .T. ) ;
#36537=DIRECTION ( 'NONE',  ( 0.000000000000000000, 0.000000000000000000, -1.000000000000000000 ) ) ;
#36538=AXIS2_PLACEMENT_3D ( 'NONE', #15261, #26698, #12061 ) ;
#36539=EDGE_CURVE ( 'NONE', #21337, #31907, #27118, .T. ) ;
#36540=AXIS2_PLACEMENT_3D ( 'NONE', #9510, #17556, #29541 ) ;
#36541=CARTESIAN_POINT ( 'NONE',  ( -17.00000337463125533, -77.94228634059960825, -9.999999999999998224 ) ) ;
#36542=ORIENTED_EDGE ( 'NONE', *, *, #10615, .T. ) ;
#36545=DIRECTION ( 'NONE',  ( 0.000000000000000000, 0.000000000000000000, 1.000000000000000000 ) ) ;
#36546=DIRECTION ( 'NONE',  ( 0.000000000000000000, 0.000000000000000000, -1.000000000000000000 ) ) ;
#36548=DIRECTION ( 'NONE',  ( 0.000000000000000000, 0.000000000000000000, 1.000000000000000000 ) ) ;
#36549=DIRECTION ( 'NONE',  ( 1.000000000000000000, 0.000000000000000000, 0.000000000000000000 ) ) ;
#36550=LINE ( 'NONE', #7861, #24932 ) ;
#36551=AXIS2_PLACEMENT_3D ( 'NONE', #31209, #7966, #25591 ) ;
#36552=ORIENTED_EDGE ( 'NONE', *, *, #14752, .F. ) ;
#36554=CARTESIAN_POINT ( 'NONE',  ( 0.000000000000000000, 0.000000000000000000, -5.000000000000000000 ) ) ;
#36555=ORIENTED_EDGE ( 'NONE', *, *, #17941, .F. ) ;
#36556=CARTESIAN_POINT ( 'NONE',  ( -65.00000337463104927, -25.98076211353322051, -9.999999999999998224 ) ) ;
#36557=DIRECTION ( 'NONE',  ( -0.000000000000000000, -0.000000000000000000, -1.000000000000000000 ) ) ;
#36558=EDGE_CURVE ( 'NONE', #32142, #1362, #33314, .T. ) ;
#36559=CARTESIAN_POINT ( 'NONE',  ( -35.19434990244938888, 52.39915983220783602, 12.49999999999999822 ) ) ;
#36560=CIRCLE ( 'NONE', #9597, 27.00000000000001421 ) ;
#36562=CARTESIAN_POINT ( 'NONE',  ( 49.99999662536846756, -69.28203230275519786, -9.999999999999998224 ) ) ;
#36565=DIRECTION ( 'NONE',  ( 0.000000000000000000, 0.000000000000000000, 1.000000000000000000 ) ) ;
#36566=ORIENTED_EDGE ( 'NONE', *, *, #7335, .F. ) ;
#36567=VERTEX_POINT ( 'NONE', #1627 ) ;
#36568=ADVANCED_FACE ( 'NONE', ( #7632 ), #13063, .F. ) ;
#36570=CARTESIAN_POINT ( 'NONE',  ( -57.00000337463107059, 60.62177826491078747, -9.999999999999998224 ) ) ;
#36571=DIRECTION ( 'NONE',  ( 1.000000000000000000, -0.000000000000000000, 0.000000000000000000 ) ) ;
#36572=CIRCLE ( 'NONE', #26364, 2.000000000000001776 ) ;
#36573=CARTESIAN_POINT ( 'NONE',  ( 46.74665512060159500, 61.59603906214631763, 12.50000000000000000 ) ) ;
#36574=ORIENTED_EDGE ( 'NONE', *, *, #25000, .F. ) ;
#36576=DIRECTION ( 'NONE',  ( -1.000000000000000000, 0.000000000000000000, 0.000000000000000000 ) ) ;
#36577=ORIENTED_EDGE ( 'NONE', *, *, #31258, .T. ) ;
#36578=VERTEX_POINT ( 'NONE', #7263 ) ;
#36580=ADVANCED_FACE ( 'NONE', ( #4830 ), #24316, .T. ) ;
#36581=DIRECTION ( 'NONE',  ( 1.000000000000000000, 0.000000000000000000, 0.000000000000000000 ) ) ;
#36582=ORIENTED_EDGE ( 'NONE', *, *, #31871, .T. ) ;
#36584=DIRECTION ( 'NONE',  ( 0.000000000000000000, 0.000000000000000000, -1.000000000000000000 ) ) ;
#36585=DIRECTION ( 'NONE',  ( 0.000000000000000000, 0.000000000000000000, -1.000000000000000000 ) ) ;
#36587=ORIENTED_EDGE ( 'NONE', *, *, #14222, .F. ) ;
#36588=ORIENTED_EDGE ( 'NONE', *, *, #15111, .T. ) ;
#36589=ORIENTED_EDGE ( 'NONE', *, *, #16986, .T. ) ;
#36590=DIRECTION ( 'NONE',  ( 0.000000000000000000, 0.000000000000000000, -1.000000000000000000 ) ) ;
#36591=EDGE_CURVE ( 'NONE', #691, #6247, #33518, .T. ) ;
#36593=LINE ( 'NONE', #24973, #464 ) ;
#36594=CARTESIAN_POINT ( 'NONE',  ( 24.99999662536859546, -77.94228634059960825, 12.50000000000000000 ) ) ;
#36595=DIRECTION ( 'NONE',  ( 0.000000000000000000, 0.000000000000000000, 1.000000000000000000 ) ) ;
#36596=EDGE_CURVE ( 'NONE', #2284, #3385, #14765, .T. ) ;
#36597=ORIENTED_EDGE ( 'NONE', *, *, #20734, .T. ) ;
#36598=CARTESIAN_POINT ( 'NONE',  ( 0.000000000000000000, 0.000000000000000000, 12.49999999999999822 ) ) ;
#36599=DIRECTION ( 'NONE',  ( -1.000000000000000000, 0.000000000000000000, 0.000000000000000000 ) ) ;
#36600=AXIS2_PLACEMENT_3D ( 'NONE', #4490, #26814, #32809 ) ;
#36601=FACE_OUTER_BOUND ( 'NONE', #29192, .T. ) ;
#36603=DIRECTION ( 'NONE',  ( -0.000000000000000000, -0.000000000000000000, 1.000000000000000000 ) ) ;
#36606=ORIENTED_EDGE ( 'NONE', *, *, #30519, .T. ) ;
#36607=ORIENTED_EDGE ( 'NONE', *, *, #7147, .F. ) ;
#36609=DIRECTION ( 'NONE',  ( -1.000000000000000000, 0.000000000000000000, 0.000000000000000000 ) ) ;
#36613=ORIENTED_EDGE ( 'NONE', *, *, #475, .F. ) ;
#36614=EDGE_LOOP ( 'NONE', ( #19384, #32847, #13170, #11079 ) ) ;
#36615=DIRECTION ( 'NONE',  ( 1.000000000000000000, 0.000000000000000000, 0.000000000000000000 ) ) ;
#36616=ORIENTED_EDGE ( 'NONE', *, *, #23047, .T. ) ;
#36618=CIRCLE ( 'NONE', #6686, 2.000000000000001776 ) ;
#36619=DIRECTION ( 'NONE',  ( 0.000000000000000000, 0.000000000000000000, 1.000000000000000000 ) ) ;
#36620=ORIENTED_EDGE ( 'NONE', *, *, #11316, .T. ) ;
#36621=EDGE_LOOP ( 'NONE', ( #69, #597 ) ) ;
#36622=EDGE_CURVE ( 'NONE', #27142, #4841, #22814, .T. ) ;
#36624=FACE_OUTER_BOUND ( 'NONE', #30647, .T. ) ;
#36625=ORIENTED_EDGE ( 'NONE', *, *, #4999, .T. ) ;
#36626=VERTEX_POINT ( 'NONE', #27854 ) ;
#36627=CARTESIAN_POINT ( 'NONE',  ( 3.499999999999991562, 55.00000000000000000, -5.000000000000000000 ) ) ;
#36628=DIRECTION ( 'NONE',  ( 0.000000000000000000, 0.000000000000000000, 1.000000000000000000 ) ) ;
#36629=EDGE_CURVE ( 'NONE', #1500, #575, #2179, .T. ) ;
#36631=CYLINDRICAL_SURFACE ( 'NONE', #10713, 2.000000000000001776 ) ;
#36632=EDGE_LOOP ( 'NONE', ( #5204, #25079, #6706, #13579, #7094 ) ) ;
#36633=DIRECTION ( 'NONE',  ( 0.000000000000000000, 0.000000000000000000, 1.000000000000000000 ) ) ;
#36634=EDGE_CURVE ( 'NONE', #25705, #8997, #29134, .T. ) ;
#36635=FACE_BOUND ( 'NONE', #11137, .T. ) ;
#36636=CARTESIAN_POINT ( 'NONE',  ( 9.999996625368625658, 86.60254037844397601, -5.000000000000000000 ) ) ;
#36637=DIRECTION ( 'NONE',  ( 0.000000000000000000, 0.000000000000000000, -1.000000000000000000 ) ) ;
#36639=CYLINDRICAL_SURFACE ( 'NONE', #36852, 2.000000000000001776 ) ;
#36640=CARTESIAN_POINT ( 'NONE',  ( -50.00000337463109190, 51.96152422706637708, -9.999999999999998224 ) ) ;
#36641=AXIS2_PLACEMENT_3D ( 'NONE', #35520, #35702, #9646 ) ;
#36642=DIRECTION ( 'NONE',  ( 0.000000000000000000, 0.000000000000000000, 1.000000000000000000 ) ) ;
#36643=ORIENTED_EDGE ( 'NONE', *, *, #26774, .T. ) ;
#36646=CARTESIAN_POINT ( 'NONE',  ( 14.99999662536859901, 77.94228634059957983, -9.999999999999998224 ) ) ;
#36648=VERTEX_POINT ( 'NONE', #5738 ) ;
#36649=ORIENTED_EDGE ( 'NONE', *, *, #15831, .F. ) ;
#36652=DIRECTION ( 'NONE',  ( -0.5000000000000094369, -0.8660254037844332675, 0.000000000000000000 ) ) ;
#36653=CYLINDRICAL_SURFACE ( 'NONE', #1083, 2.000000000000001776 ) ;
#36654=EDGE_LOOP ( 'NONE', ( #21050, #19148 ) ) ;
#36655=CARTESIAN_POINT ( 'NONE',  ( -68.66839587347244844, -56.74224907229007187, -49.22241343995298024 ) ) ;
#36656=DIRECTION ( 'NONE',  ( 0.000000000000000000, 0.000000000000000000, 1.000000000000000000 ) ) ;
#36657=ORIENTED_EDGE ( 'NONE', *, *, #2088, .T. ) ;
#36658=CARTESIAN_POINT ( 'NONE',  ( 86.99999662536831124, -25.98076211353319565, 17.49999999999999645 ) ) ;
#36659=ORIENTED_EDGE ( 'NONE', *, *, #19497, .F. ) ;
#36660=DIRECTION ( 'NONE',  ( 1.000000000000000000, 0.000000000000000000, 0.000000000000000000 ) ) ;
#36661=ADVANCED_FACE ( 'NONE', ( #8727 ), #22984, .T. ) ;
#36662=DIRECTION ( 'NONE',  ( 0.4999999999999919509, -0.8660254037844432595, 0.000000000000000000 ) ) ;
#36667=CARTESIAN_POINT ( 'NONE',  ( -78.00000337463094979, -17.32050807568882078, 12.50000000000000000 ) ) ;
#36668=DIRECTION ( 'NONE',  ( -1.000000000000000000, 0.000000000000000000, 0.000000000000000000 ) ) ;
#36669=VERTEX_POINT ( 'NONE', #7992 ) ;
#36670=DIRECTION ( 'NONE',  ( 0.000000000000000000, 0.000000000000000000, -1.000000000000000000 ) ) ;
#36673=ORIENTED_EDGE ( 'NONE', *, *, #3928, .T. ) ;
#36675=ADVANCED_FACE ( 'NONE', ( #30849 ), #36683, .F. ) ;
#36676=CARTESIAN_POINT ( 'NONE',  ( 34.99999662536853862, 77.94228634059959404, 12.50000000000000000 ) ) ;
#36677=CARTESIAN_POINT ( 'NONE',  ( -3.374631303565411855E-06, -86.60254037844400443, 17.49999999999999645 ) ) ;
#36679=CIRCLE ( 'NONE', #22130, 33.00000000000001421 ) ;
#36680=AXIS2_PLACEMENT_3D ( 'NONE', #36977, #30602, #33785 ) ;
#36681=EDGE_LOOP ( 'NONE', ( #25625, #17134, #14536, #6578, #36616 ) ) ;
#36682=ORIENTED_EDGE ( 'NONE', *, *, #18911, .F. ) ;
#36683=CYLINDRICAL_SURFACE ( 'NONE', #25566, 2.000000000000001776 ) ;
#36684=DIRECTION ( 'NONE',  ( 1.000000000000000000, 0.000000000000000000, 0.000000000000000000 ) ) ;
#36685=ORIENTED_EDGE ( 'NONE', *, *, #17656, .F. ) ;
#36686=ORIENTED_EDGE ( 'NONE', *, *, #26583, .F. ) ;
#36688=AXIS2_PLACEMENT_3D ( 'NONE', #14268, #3183, #8624 ) ;
#36691=LINE ( 'NONE', #11538, #33966 ) ;
#36692=ORIENTED_EDGE ( 'NONE', *, *, #17611, .T. ) ;
#36693=ORIENTED_EDGE ( 'NONE', *, *, #28199, .F. ) ;
#36695=DIRECTION ( 'NONE',  ( 1.000000000000000000, 0.000000000000000000, 0.000000000000000000 ) ) ;
#36698=CARTESIAN_POINT ( 'NONE',  ( -18.00000337463123756, -86.60254037844400443, -9.999999999999998224 ) ) ;
#36699=EDGE_LOOP ( 'NONE', ( #32979, #18103, #20104, #18718, #2450, #24068 ) ) ;
#36700=FACE_BOUND ( 'NONE', #36832, .T. ) ;
#36701=VECTOR ( 'NONE', #19683, 1000.000000000000000 ) ;
#36702=EDGE_CURVE ( 'NONE', #4841, #2089, #17760, .T. ) ;
#36703=CARTESIAN_POINT ( 'NONE',  ( -57.00000337463107059, 60.62177826491078747, -9.999999999999998224 ) ) ;
#36705=ORIENTED_EDGE ( 'NONE', *, *, #19830, .F. ) ;
#36708=AXIS2_PLACEMENT_3D ( 'NONE', #7678, #10125, #21558 ) ;
#36709=DIRECTION ( 'NONE',  ( -1.000000000000000000, 0.000000000000000000, 0.000000000000000000 ) ) ;
#36710=LINE ( 'NONE', #33350, #1137 ) ;
#36711=ORIENTED_EDGE ( 'NONE', *, *, #30212, .F. ) ;
#36712=CIRCLE ( 'NONE', #12733, 27.00000000000001421 ) ;
#36713=CARTESIAN_POINT ( 'NONE',  ( 21.99999662536859191, 69.28203230275516944, 17.49999999999999645 ) ) ;
#36714=EDGE_CURVE ( 'NONE', #29900, #9542, #35742, .T. ) ;
#36715=FACE_OUTER_BOUND ( 'NONE', #35985, .T. ) ;
#36716=CARTESIAN_POINT ( 'NONE',  ( -58.00000337463108480, -51.96152422706641971, -9.999999999999998224 ) ) ;
#36717=ORIENTED_EDGE ( 'NONE', *, *, #18094, .F. ) ;
#36718=ORIENTED_EDGE ( 'NONE', *, *, #31134, .T. ) ;
#36721=CARTESIAN_POINT ( 'NONE',  ( -33.99999999999945288, 58.88972745734214698, -49.86561046011506448 ) ) ;
#36722=AXIS2_PLACEMENT_3D ( 'NONE', #34222, #14130, #20482 ) ;
#36723=DIRECTION ( 'NONE',  ( 1.000000000000000000, 0.000000000000000000, 0.000000000000000000 ) ) ;
#36724=ADVANCED_FACE ( 'NONE', ( #27098 ), #32731, .F. ) ;
#36725=ADVANCED_FACE ( 'NONE', ( #35396 ), #33096, .F. ) ;
#36726=CIRCLE ( 'NONE', #2004, 3.000000000000005773 ) ;
#36728=EDGE_CURVE ( 'NONE', #20625, #13035, #7243, .T. ) ;
#36731=CARTESIAN_POINT ( 'NONE',  ( -35.00000337463116296, 60.62177826491077326, -9.999999999999998224 ) ) ;
#36737=DIRECTION ( 'NONE',  ( 0.000000000000000000, 0.000000000000000000, 1.000000000000000000 ) ) ;
#36738=CIRCLE ( 'NONE', #28927, 2.000000000000001776 ) ;
#36739=DIRECTION ( 'NONE',  ( 0.000000000000000000, 0.000000000000000000, 1.000000000000000000 ) ) ;
#36740=FACE_OUTER_BOUND ( 'NONE', #8451, .T. ) ;
#36741=DIRECTION ( 'NONE',  ( -0.000000000000000000, -0.000000000000000000, 1.000000000000000000 ) ) ;
#36742=EDGE_LOOP ( 'NONE', ( #18160, #8806, #34778, #18558 ) ) ;
#36743=CARTESIAN_POINT ( 'NONE',  ( -30.00000337463118427, 69.28203230275516944, -9.999999999999998224 ) ) ;
#36745=ORIENTED_EDGE ( 'NONE', *, *, #36207, .F. ) ;
#36747=DIRECTION ( 'NONE',  ( 0.000000000000000000, 0.000000000000000000, 1.000000000000000000 ) ) ;
#36749=VERTEX_POINT ( 'NONE', #19056 ) ;
#36750=EDGE_CURVE ( 'NONE', #34871, #30085, #13566, .T. ) ;
#36753=CARTESIAN_POINT ( 'NONE',  ( 0.000000000000000000, 0.000000000000000000, -5.000000000000000000 ) ) ;
#36754=DIRECTION ( 'NONE',  ( 0.000000000000000000, 0.000000000000000000, 1.000000000000000000 ) ) ;
#36755=VERTEX_POINT ( 'NONE', #15857 ) ;
#36756=ORIENTED_EDGE ( 'NONE', *, *, #3906, .F. ) ;
#36757=ORIENTED_EDGE ( 'NONE', *, *, #13155, .F. ) ;
#36762=COLOUR_RGB ( '', 0.72549020, 0.75294118, 0.79215686) ;
#36764=DIRECTION ( 'NONE',  ( 1.000000000000000000, 0.000000000000000000, 0.000000000000000000 ) ) ;
#36767=ORIENTED_EDGE ( 'NONE', *, *, #28255, .F. ) ;
#36768=CARTESIAN_POINT ( 'NONE',  ( -65.00000337463102085, 43.30127018922198801, -9.999999999999998224 ) ) ;
#36769=CARTESIAN_POINT ( 'NONE',  ( 0.000000000000000000, 55.00000000000000000, -10.00000000000000000 ) ) ;
#36771=DIRECTION ( 'NONE',  ( 0.000000000000000000, 0.000000000000000000, 1.000000000000000000 ) ) ;
#36774=CARTESIAN_POINT ( 'NONE',  ( 58.88972745734226066, 33.99999999999924682, 12.49999999999999822 ) ) ;
#36775=ORIENTED_EDGE ( 'NONE', *, *, #14156, .F. ) ;
#36776=CIRCLE ( 'NONE', #20581, 2.000000000000001776 ) ;
#36777=ORIENTED_EDGE ( 'NONE', *, *, #4143, .T. ) ;
#36778=DIRECTION ( 'NONE',  ( 1.000000000000000000, 0.000000000000000000, 0.000000000000000000 ) ) ;
#36782=VERTEX_POINT ( 'NONE', #21288 ) ;
#36784=VECTOR ( 'NONE', #16156, 1000.000000000000000 ) ;
#36785=DIRECTION ( 'NONE',  ( 0.000000000000000000, 0.000000000000000000, -1.000000000000000000 ) ) ;
#36786=CIRCLE ( 'NONE', #11630, 2.000000000000001776 ) ;
#36787=ORIENTED_EDGE ( 'NONE', *, *, #36488, .F. ) ;
#36788=CARTESIAN_POINT ( 'NONE',  ( 66.99999662536841072, 25.98076211353318854, 17.49999999999999645 ) ) ;
#36792=LINE ( 'NONE', #22544, #28025 ) ;
#36793=CYLINDRICAL_SURFACE ( 'NONE', #7673, 2.000000000000001776 ) ;
#36794=ORIENTED_EDGE ( 'NONE', *, *, #6827, .T. ) ;
#36795=AXIS2_PLACEMENT_3D ( 'NONE', #35814, #10121, #7298 ) ;
#36797=DIRECTION ( 'NONE',  ( 0.000000000000000000, 0.000000000000000000, 1.000000000000000000 ) ) ;
#36799=DIRECTION ( 'NONE',  ( 1.000000000000000000, 0.000000000000000000, 0.000000000000000000 ) ) ;
#36800=FACE_OUTER_BOUND ( 'NONE', #4161, .T. ) ;
#36801=AXIS2_PLACEMENT_3D ( 'NONE', #32820, #36380, #21740 ) ;
#36802=EDGE_CURVE ( 'NONE', #33338, #5117, #10054, .T. ) ;
#36804=DIRECTION ( 'NONE',  ( 0.000000000000000000, 0.000000000000000000, 1.000000000000000000 ) ) ;
#36805=FACE_BOUND ( 'NONE', #31752, .T. ) ;
#36807=PLANE ( 'NONE',  #31265 ) ;
#36809=DIRECTION ( 'NONE',  ( 1.000000000000000000, 0.000000000000000000, 0.000000000000000000 ) ) ;
#36810=AXIS2_PLACEMENT_3D ( 'NONE', #17009, #22836, #31255 ) ;
#36811=VECTOR ( 'NONE', #17250, 1000.000000000000000 ) ;
#36812=PLANE ( 'NONE',  #29927 ) ;
#36816=ORIENTED_EDGE ( 'NONE', *, *, #13468, .F. ) ;
#36819=CARTESIAN_POINT ( 'NONE',  ( 86.45172111230354517, -31.46585318596159553, -49.86348611802629449 ) ) ;
#36820=ORIENTED_EDGE ( 'NONE', *, *, #121, .T. ) ;
#36821=ORIENTED_EDGE ( 'NONE', *, *, #7392, .F. ) ;
#36822=ORIENTED_EDGE ( 'NONE', *, *, #18620, .F. ) ;
#36823=CIRCLE ( 'NONE', #9269, 2.000000000000001776 ) ;
#36824=DIRECTION ( 'NONE',  ( 0.000000000000000000, 0.000000000000000000, 1.000000000000000000 ) ) ;
#36825=DIRECTION ( 'NONE',  ( 1.000000000000000000, 0.000000000000000000, 0.000000000000000000 ) ) ;
#36826=EDGE_LOOP ( 'NONE', ( #14581, #5778, #7863, #12711 ) ) ;
#36828=CARTESIAN_POINT ( 'NONE',  ( 74.99999662536836809, -8.660254037844401509, -5.000000000000000000 ) ) ;
#36829=ORIENTED_EDGE ( 'NONE', *, *, #21980, .F. ) ;
#36830=EDGE_CURVE ( 'NONE', #29836, #5293, #34530, .T. ) ;
#36831=DIRECTION ( 'NONE',  ( 0.000000000000000000, 0.000000000000000000, 1.000000000000000000 ) ) ;
#36832=EDGE_LOOP ( 'NONE', ( #2513, #25917 ) ) ;
#36833=DIRECTION ( 'NONE',  ( -1.000000000000000000, 0.000000000000000000, 0.000000000000000000 ) ) ;
#36836=AXIS2_PLACEMENT_3D ( 'NONE', #3263, #449, #7007 ) ;
#36837=LINE ( 'NONE', #11144, #29166 ) ;
#36838=CARTESIAN_POINT ( 'NONE',  ( -80.00000337463094979, 17.32050807568878525, -5.000000000000000000 ) ) ;
#36839=EDGE_CURVE ( 'NONE', #32311, #34910, #27936, .T. ) ;
#36840=ORIENTED_EDGE ( 'NONE', *, *, #16537, .F. ) ;
#36841=DIRECTION ( 'NONE',  ( 0.000000000000000000, 0.000000000000000000, 1.000000000000000000 ) ) ;
#36843=CARTESIAN_POINT ( 'NONE',  ( 74.99999662536836809, 25.98076211353319565, 17.49999999999999645 ) ) ;
#36844=DIRECTION ( 'NONE',  ( 0.000000000000000000, 0.000000000000000000, 1.000000000000000000 ) ) ;
#36845=EDGE_CURVE ( 'NONE', #34930, #16912, #32728, .T. ) ;
#36846=VECTOR ( 'NONE', #32898, 1000.000000000000000 ) ;
#36847=ORIENTED_EDGE ( 'NONE', *, *, #29216, .T. ) ;
#36848=CYLINDRICAL_SURFACE ( 'NONE', #21569, 1.999999999999998224 ) ;
#36849=CARTESIAN_POINT ( 'NONE',  ( -12.00000337463125000, -86.60254037844400443, 17.49999999999999645 ) ) ;
#36850=ORIENTED_EDGE ( 'NONE', *, *, #24767, .T. ) ;
#36851=FACE_OUTER_BOUND ( 'NONE', #29581, .T. ) ;
#36852=AXIS2_PLACEMENT_3D ( 'NONE', #19929, #31005, #36809 ) ;
#36853=DIRECTION ( 'NONE',  ( 0.000000000000000000, 0.000000000000000000, -1.000000000000000000 ) ) ;
#36854=CARTESIAN_POINT ( 'NONE',  ( 51.99999662536847467, 69.28203230275516944, 17.49999999999999645 ) ) ;
#36856=CIRCLE ( 'NONE', #21298, 3.000000000000002665 ) ;
#36857=CARTESIAN_POINT ( 'NONE',  ( 56.67878100130369035, -27.78182860042797131, 12.49999999999999822 ) ) ;
#36858=AXIS2_PLACEMENT_3D ( 'NONE', #10831, #5562, #22261 ) ;
#36859=EDGE_LOOP ( 'NONE', ( #32207, #33428, #37101, #36013 ) ) ;
#36860=EDGE_LOOP ( 'NONE', ( #19515, #26999 ) ) ;
#36861=CARTESIAN_POINT ( 'NONE',  ( -78.00000337463096400, -34.64101615137762025, -9.999999999999998224 ) ) ;
#36862=CYLINDRICAL_SURFACE ( 'NONE', #5019, 2.000000000000000000 ) ;
#36867=ORIENTED_EDGE ( 'NONE', *, *, #32768, .F. ) ;
#36868=VERTEX_POINT ( 'NONE', #1799 ) ;
#36869=CARTESIAN_POINT ( 'NONE',  ( -48.00000337463112032, -51.96152422706641971, -5.000000000000000000 ) ) ;
#36872=ORIENTED_EDGE ( 'NONE', *, *, #18175, .T. ) ;
#36873=EDGE_CURVE ( 'NONE', #8103, #6603, #1042, .T. ) ;
#36874=ORIENTED_EDGE ( 'NONE', *, *, #7466, .F. ) ;
#36875=CARTESIAN_POINT ( 'NONE',  ( 74.99999662536835388, -43.30127018922199511, -9.999999999999998224 ) ) ;
#36876=AXIS2_PLACEMENT_3D ( 'NONE', #8330, #16933, #28358 ) ;
#36877=CYLINDRICAL_SURFACE ( 'NONE', #30261, 2.000000000000001776 ) ;
#36878=VERTEX_POINT ( 'NONE', #24676 ) ;
#36880=CARTESIAN_POINT ( 'NONE',  ( -3.374631334790434423E-06, 69.28203230275516944, -9.999999999999998224 ) ) ;
#36882=FACE_BOUND ( 'NONE', #21540, .T. ) ;
#36885=AXIS2_PLACEMENT_3D ( 'NONE', #32515, #13213, #7032 ) ;
#36887=CIRCLE ( 'NONE', #22512, 2.000000000000001776 ) ;
#36888=ORIENTED_EDGE ( 'NONE', *, *, #29935, .T. ) ;
#36890=AXIS2_PLACEMENT_3D ( 'NONE', #2359, #11141, #4971 ) ;
#36891=FACE_OUTER_BOUND ( 'NONE', #26817, .T. ) ;
#36892=EDGE_CURVE ( 'NONE', #21874, #725, #32155, .T. ) ;
#36893=DIRECTION ( 'NONE',  ( 0.000000000000000000, 0.000000000000000000, 1.000000000000000000 ) ) ;
#36894=FACE_OUTER_BOUND ( 'NONE', #22924, .T. ) ;
#36895=ORIENTED_EDGE ( 'NONE', *, *, #32837, .T. ) ;
#36896=DIRECTION ( 'NONE',  ( 1.000000000000000000, 0.000000000000000000, 0.000000000000000000 ) ) ;
#36897=CARTESIAN_POINT ( 'NONE',  ( -68.00000337463099243, 51.96152422706637708, -9.999999999999998224 ) ) ;
#36898=LINE ( 'NONE', #16294, #33300 ) ;
#36899=AXIS2_PLACEMENT_3D ( 'NONE', #8713, #8539, #20157 ) ;
#36901=ORIENTED_EDGE ( 'NONE', *, *, #15591, .F. ) ;
#36902=ORIENTED_EDGE ( 'NONE', *, *, #7055, .F. ) ;
#36903=FACE_OUTER_BOUND ( 'NONE', #22504, .T. ) ;
#36904=FACE_OUTER_BOUND ( 'NONE', #30775, .T. ) ;
#36905=VECTOR ( 'NONE', #19206, 1000.000000000000000 ) ;
#36907=AXIS2_PLACEMENT_3D ( 'NONE', #1529, #21042, #15788 ) ;
#36908=CARTESIAN_POINT ( 'NONE',  ( 61.99999662536845335, 34.64101615137759893, -9.999999999999998224 ) ) ;
#36909=CIRCLE ( 'NONE', #25509, 2.000000000000001776 ) ;
#36910=EDGE_CURVE ( 'NONE', #3771, #12599, #22794, .T. ) ;
#36912=DIRECTION ( 'NONE',  ( -0.000000000000000000, -0.000000000000000000, -1.000000000000000000 ) ) ;
#36914=ADVANCED_FACE ( 'NONE', ( #8156 ), #7970, .F. ) ;
#36915=DIRECTION ( 'NONE',  ( 0.000000000000000000, 0.000000000000000000, 1.000000000000000000 ) ) ;
#36916=DIRECTION ( 'NONE',  ( -1.051347561198064495E-14, -1.000000000000000000, 0.000000000000000000 ) ) ;
#36917=ORIENTED_EDGE ( 'NONE', *, *, #25976, .F. ) ;
#36918=CIRCLE ( 'NONE', #20736, 2.000000000000001776 ) ;
#36920=ORIENTED_EDGE ( 'NONE', *, *, #17239, .F. ) ;
#36922=DIRECTION ( 'NONE',  ( 0.000000000000000000, 0.000000000000000000, -1.000000000000000000 ) ) ;
#36924=CYLINDRICAL_SURFACE ( 'NONE', #34676, 2.000000000000001776 ) ;
#36926=ORIENTED_EDGE ( 'NONE', *, *, #11710, .T. ) ;
#36928=EDGE_CURVE ( 'NONE', #26778, #11374, #25597, .T. ) ;
#36929=AXIS2_PLACEMENT_3D ( 'NONE', #31186, #2502, #13924 ) ;
#36931=FACE_BOUND ( 'NONE', #20952, .T. ) ;
#36932=VERTEX_POINT ( 'NONE', #30653 ) ;
#36933=ORIENTED_EDGE ( 'NONE', *, *, #36084, .T. ) ;
#36935=FACE_OUTER_BOUND ( 'NONE', #4714, .T. ) ;
#36937=CIRCLE ( 'NONE', #20753, 27.00000000000001421 ) ;
#36938=EDGE_CURVE ( 'NONE', #32397, #34636, #8224, .T. ) ;
#36941=DIRECTION ( 'NONE',  ( 0.000000000000000000, 0.000000000000000000, -1.000000000000000000 ) ) ;
#36943=ADVANCED_FACE ( 'NONE', ( #10958 ), #2154, .F. ) ;
#36944=DIRECTION ( 'NONE',  ( 0.000000000000000000, 0.000000000000000000, 1.000000000000000000 ) ) ;
#36945=VECTOR ( 'NONE', #4072, 1000.000000000000000 ) ;
#36946=EDGE_CURVE ( 'NONE', #357, #245, #31032, .T. ) ;
#36948=ADVANCED_FACE ( 'NONE', ( #19959 ), #33491, .F. ) ;
#36949=VERTEX_POINT ( 'NONE', #28033 ) ;
#36951=VERTEX_POINT ( 'NONE', #25404 ) ;
#36952=CIRCLE ( 'NONE', #24996, 27.00000000000001421 ) ;
#36953=VERTEX_POINT ( 'NONE', #22398 ) ;
#36955=DIRECTION ( 'NONE',  ( 0.000000000000000000, 0.000000000000000000, 1.000000000000000000 ) ) ;
#36956=CARTESIAN_POINT ( 'NONE',  ( 19.99999662536861678, -69.28203230275519786, 12.50000000000000000 ) ) ;
#36957=DIRECTION ( 'NONE',  ( -1.000000000000000000, 0.000000000000000000, 0.000000000000000000 ) ) ;
#36958=AXIS2_PLACEMENT_3D ( 'NONE', #14360, #28600, #20507 ) ;
#36959=CYLINDRICAL_SURFACE ( 'NONE', #16928, 2.000000000000001776 ) ;
#36960=DIRECTION ( 'NONE',  ( -1.000000000000000000, 0.000000000000000000, 0.000000000000000000 ) ) ;
#36961=CIRCLE ( 'NONE', #6403, 2.000000000000001776 ) ;
#36962=ORIENTED_EDGE ( 'NONE', *, *, #23295, .F. ) ;
#36963=LINE ( 'NONE', #2837, #35084 ) ;
#36964=AXIS2_PLACEMENT_3D ( 'NONE', #22325, #22509, #33596 ) ;
#36966=CIRCLE ( 'NONE', #35763, 27.00000000000001421 ) ;
#36967=DIRECTION ( 'NONE',  ( 0.000000000000000000, 0.000000000000000000, 1.000000000000000000 ) ) ;
#36968=ORIENTED_EDGE ( 'NONE', *, *, #2414, .F. ) ;
#36969=DIRECTION ( 'NONE',  ( -1.000000000000000000, 0.000000000000000000, 0.000000000000000000 ) ) ;
#36970=FACE_OUTER_BOUND ( 'NONE', #4803, .T. ) ;
#36971=AXIS2_PLACEMENT_3D ( 'NONE', #15496, #12659, #21493 ) ;
#36972=VERTEX_POINT ( 'NONE', #5364 ) ;
#36974=EDGE_LOOP ( 'NONE', ( #22525, #29453, #22000, #31320, #27110, #17486 ) ) ;
#36975=AXIS2_PLACEMENT_3D ( 'NONE', #2122, #21643, #25210 ) ;
#36976=DIRECTION ( 'NONE',  ( -0.5000000000000098810, -0.8660254037844328234, 0.000000000000000000 ) ) ;
#36977=CARTESIAN_POINT ( 'NONE',  ( -60.93295298010992411, -19.13981058454771755, 12.49999999999999822 ) ) ;
#36980=ORIENTED_EDGE ( 'NONE', *, *, #2801, .F. ) ;
#36981=ORIENTED_EDGE ( 'NONE', *, *, #36845, .F. ) ;
#36982=CARTESIAN_POINT ( 'NONE',  ( -72.28378166042018904, -61.53067111003240797, -49.22241343995298024 ) ) ;
#36983=CIRCLE ( 'NONE', #31583, 3.000000000000002665 ) ;
#36984=ORIENTED_EDGE ( 'NONE', *, *, #7262, .F. ) ;
#36986=CYLINDRICAL_SURFACE ( 'NONE', #33366, 2.000000000000001776 ) ;
#36987=EDGE_LOOP ( 'NONE', ( #19283, #25253 ) ) ;
#36988=CIRCLE ( 'NONE', #29831, 2.000000000000001776 ) ;
#36989=ORIENTED_EDGE ( 'NONE', *, *, #32810, .T. ) ;
#36990=CARTESIAN_POINT ( 'NONE',  ( -25.00000337463121980, -77.94228634059963667, 17.49999999999999645 ) ) ;
#36991=DIRECTION ( 'NONE',  ( 0.000000000000000000, 0.000000000000000000, 1.000000000000000000 ) ) ;
#36992=FACE_BOUND ( 'NONE', #33452, .T. ) ;
#36994=ORIENTED_EDGE ( 'NONE', *, *, #32773, .T. ) ;
#36995=ORIENTED_EDGE ( 'NONE', *, *, #4034, .T. ) ;
#36996=CYLINDRICAL_SURFACE ( 'NONE', #23935, 27.00000000000001066 ) ;
#36997=DIRECTION ( 'NONE',  ( -1.000000000000000000, 0.000000000000000000, 0.000000000000000000 ) ) ;
#36998=CIRCLE ( 'NONE', #5257, 33.00000000000001421 ) ;
#36999=CARTESIAN_POINT ( 'NONE',  ( 72.99999662536835388, -25.98076211353319565, -5.000000000000000000 ) ) ;
#37000=CARTESIAN_POINT ( 'NONE',  ( 12.99999662536863632, -77.94228634059960825, -9.999999999999998224 ) ) ;
#37001=CIRCLE ( 'NONE', #22622, 2.000000000000001776 ) ;
#37002=ORIENTED_EDGE ( 'NONE', *, *, #20004, .F. ) ;
#37003=CYLINDRICAL_SURFACE ( 'NONE', #16563, 2.000000000000001776 ) ;
#37004=FACE_BOUND ( 'NONE', #32960, .T. ) ;
#37005=CARTESIAN_POINT ( 'NONE',  ( -18.00000337463123756, -69.28203230275522628, 12.50000000000000000 ) ) ;
#37006=CARTESIAN_POINT ( 'NONE',  ( 74.99999662536836809, 43.30127018922198801, 12.50000000000000000 ) ) ;
#37007=AXIS2_PLACEMENT_3D ( 'NONE', #17905, #17703, #97 ) ;
#37013=CARTESIAN_POINT ( 'NONE',  ( -85.00000337463092137, -8.660254037844422825, -5.000000000000000000 ) ) ;
#37015=DIRECTION ( 'NONE',  ( 1.000000000000000000, 0.000000000000000000, 0.000000000000000000 ) ) ;
#37016=CIRCLE ( 'NONE', #4061, 1.999999999999998224 ) ;
#37017=CIRCLE ( 'NONE', #12447, 2.000000000000001776 ) ;
#37020=EDGE_CURVE ( 'NONE', #111, #28932, #36837, .T. ) ;
#37021=ADVANCED_FACE ( 'NONE', ( #22593 ), #8357, .F. ) ;
#37022=AXIS2_PLACEMENT_3D ( 'NONE', #8222, #33554, #7860 ) ;
#37023=ORIENTED_EDGE ( 'NONE', *, *, #16020, .F. ) ;
#37024=ORIENTED_EDGE ( 'NONE', *, *, #17191, .F. ) ;
#37025=ORIENTED_EDGE ( 'NONE', *, *, #32366, .T. ) ;
#37028=DIRECTION ( 'NONE',  ( -0.8660254037844449249, -0.4999999999999888423, 0.000000000000000000 ) ) ;
#37030=LINE ( 'NONE', #11333, #14905 ) ;
#37031=EDGE_CURVE ( 'NONE', #28688, #24619, #23796, .T. ) ;
#37032=ORIENTED_EDGE ( 'NONE', *, *, #16503, .F. ) ;
#37033=CARTESIAN_POINT ( 'NONE',  ( -43.00331345287344931, -60.50675932581249583, 12.50000000000000000 ) ) ;
#37035=DIRECTION ( 'NONE',  ( -0.000000000000000000, -0.000000000000000000, 1.000000000000000000 ) ) ;
#37036=CIRCLE ( 'NONE', #32827, 2.000000000000001776 ) ;
#37037=ORIENTED_EDGE ( 'NONE', *, *, #23918, .T. ) ;
#37038=VERTEX_POINT ( 'NONE', #31755 ) ;
#37040=DIRECTION ( 'NONE',  ( -1.000000000000000000, 0.000000000000000000, 0.000000000000000000 ) ) ;
#37041=CIRCLE ( 'NONE', #32857, 3.000000000000003997 ) ;
#37042=EDGE_CURVE ( 'NONE', #27070, #36437, #17346, .T. ) ;
#37043=ORIENTED_EDGE ( 'NONE', *, *, #36270, .T. ) ;
#37044=CARTESIAN_POINT ( 'NONE',  ( 67.99999662536838230, 17.32050807568879236, -9.999999999999998224 ) ) ;
#37045=AXIS2_PLACEMENT_3D ( 'NONE', #34158, #8454, #10 ) ;
#37046=AXIS2_PLACEMENT_3D ( 'NONE', #19423, #30842, #13410 ) ;
#37048=DIRECTION ( 'NONE',  ( 0.000000000000000000, 0.000000000000000000, 1.000000000000000000 ) ) ;
#37049=ORIENTED_EDGE ( 'NONE', *, *, #8831, .T. ) ;
#37051=CARTESIAN_POINT ( 'NONE',  ( 42.99999662536850309, -60.62177826491080168, 17.49999999999999645 ) ) ;
#37053=CARTESIAN_POINT ( 'NONE',  ( 29.99999662536857770, -69.28203230275519786, -5.000000000000000000 ) ) ;
#37054=CYLINDRICAL_SURFACE ( 'NONE', #23877, 2.000000000000001776 ) ;
#37056=AXIS2_PLACEMENT_3D ( 'NONE', #31699, #34723, #26271 ) ;
#37058=AXIS2_PLACEMENT_3D ( 'NONE', #17476, #28350, #14482 ) ;
#37059=ORIENTED_EDGE ( 'NONE', *, *, #24071, .T. ) ;
#37060=EDGE_CURVE ( 'NONE', #19941, #2260, #7634, .T. ) ;
#37061=EDGE_LOOP ( 'NONE', ( #12978, #21223, #8901, #2590 ) ) ;
#37063=FACE_OUTER_BOUND ( 'NONE', #23223, .T. ) ;
#37068=CARTESIAN_POINT ( 'NONE',  ( 79.99999662536833966, 34.64101615137759183, 17.49999999999999645 ) ) ;
#37069=DIRECTION ( 'NONE',  ( -1.000000000000000000, 0.000000000000000000, 0.000000000000000000 ) ) ;
#37070=ADVANCED_FACE ( 'NONE', ( #17508 ), #25955, .F. ) ;
#37071=DIRECTION ( 'NONE',  ( -1.000000000000000000, 0.000000000000000000, 0.000000000000000000 ) ) ;
#37072=ORIENTED_EDGE ( 'NONE', *, *, #2128, .F. ) ;
#37075=EDGE_CURVE ( 'NONE', #35191, #8606, #26175, .T. ) ;
#37079=CARTESIAN_POINT ( 'NONE',  ( -3.000003374631269981, -77.94228634059960825, -9.999999999999998224 ) ) ;
#37080=ORIENTED_EDGE ( 'NONE', *, *, #5717, .F. ) ;
#37081=DIRECTION ( 'NONE',  ( 0.000000000000000000, 0.000000000000000000, 1.000000000000000000 ) ) ;
#37082=AXIS2_PLACEMENT_3D ( 'NONE', #6153, #18336, #1273 ) ;
#37083=CIRCLE ( 'NONE', #24507, 2.000000000000000000 ) ;
#37084=CARTESIAN_POINT ( 'NONE',  ( 4.279621169095998212, -62.97617850287780072, -4.999999999999997335 ) ) ;
#37085=CARTESIAN_POINT ( 'NONE',  ( -55.00000337463109901, -60.62177826491083010, -9.999999999999998224 ) ) ;
#37087=ORIENTED_EDGE ( 'NONE', *, *, #13044, .F. ) ;
#37089=DIRECTION ( 'NONE',  ( -0.000000000000000000, -0.000000000000000000, 1.000000000000000000 ) ) ;
#37091=AXIS2_PLACEMENT_3D ( 'NONE', #22065, #10420, #7429 ) ;
#37092=CARTESIAN_POINT ( 'NONE',  ( -3.374631289687624047E-06, -69.28203230275519786, 12.50000000000000000 ) ) ;
#37093=DIRECTION ( 'NONE',  ( 0.000000000000000000, 0.000000000000000000, 1.000000000000000000 ) ) ;
#37094=EDGE_LOOP ( 'NONE', ( #19391, #6984 ) ) ;
#37095=CARTESIAN_POINT ( 'NONE',  ( 42.99999662536848888, 60.62177826491077326, 12.50000000000000000 ) ) ;
#37097=LINE ( 'NONE', #31972, #468 ) ;
#37098=CYLINDRICAL_SURFACE ( 'NONE', #2168, 2.000000000000001776 ) ;
#37099=ADVANCED_FACE ( 'NONE', ( #640 ), #14892, .F. ) ;
#37100=EDGE_LOOP ( 'NONE', ( #18708, #4286 ) ) ;
#37101=ORIENTED_EDGE ( 'NONE', *, *, #9673, .T. ) ;
#37102=CIRCLE ( 'NONE', #29888, 2.000000000000000000 ) ;
#37103=EDGE_CURVE ( 'NONE', #19005, #21830, #15416, .T. ) ;
#37104=ORIENTED_EDGE ( 'NONE', *, *, #9061, .T. ) ;
#37105=AXIS2_PLACEMENT_3D ( 'NONE', #8935, #495, #31787 ) ;
#37106=FACE_OUTER_BOUND ( 'NONE', #5351, .T. ) ;
ENDSEC;
END-ISO-10303-21;
